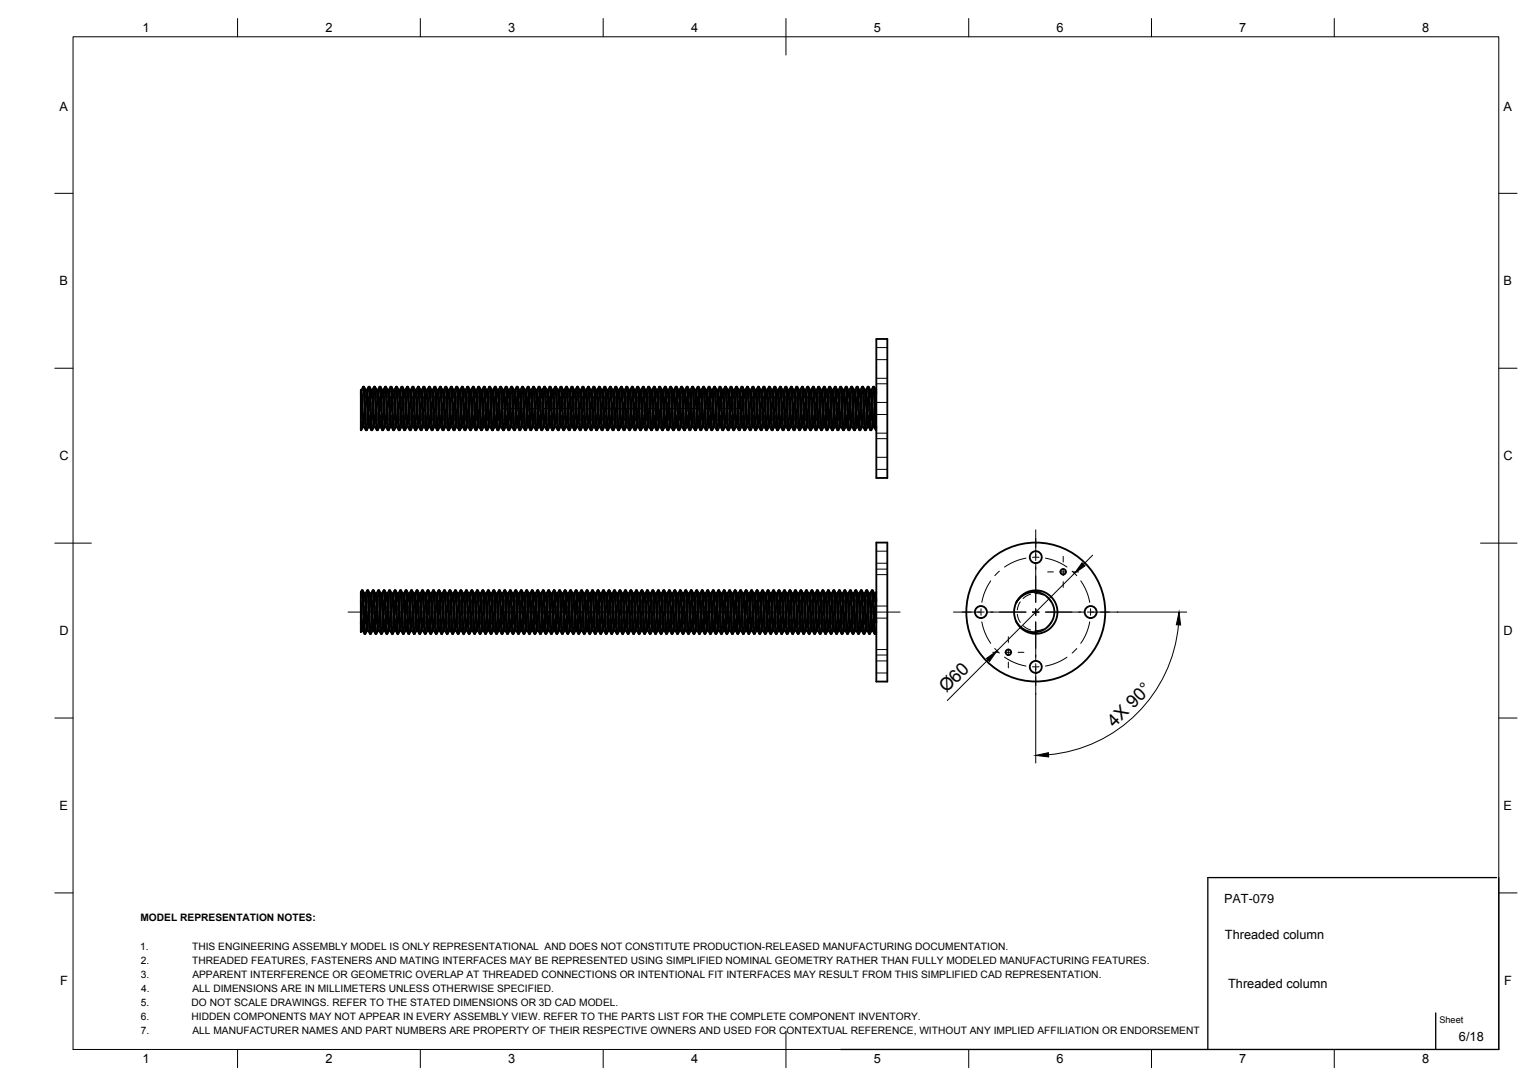
ISO-10303-21;
HEADER;
/* Generated by software containing ST-Developer
 * from STEP Tools, Inc. (www.steptools.com) 
 */

FILE_DESCRIPTION(
/* description */ ('Pipe clamp stand with threaded column'),
/* implementation_level */ '2;1');

FILE_NAME(
/* name */ 'Threaded column.step',
/* time_stamp */ '2026-10-27T10:55:48-07:00',
/* author */ (''),
/* organization */ (''),
/* preprocessor_version */ 'ST-DEVELOPER v20.2',
/* originating_system */ 'Autodesk Translation Framework v15.17.0.0',
/* authorisation */ '');

FILE_SCHEMA (('AUTOMOTIVE_DESIGN { 1 0 10303 214 3 1 1 }'));
ENDSEC;

DATA;
#10=MECHANICAL_DESIGN_GEOMETRIC_PRESENTATION_REPRESENTATION('',(#742),#34433);
#207=B_SPLINE_SURFACE_WITH_KNOTS('',3,3,((#22386,#22387,#22388,#22389,#22390,
#22391,#22392,#22393,#22394,#22395,#22396,#22397,#22398,#22399,#22400,#22401,
#22402,#22403,#22404,#22405,#22406,#22407,#22408,#22409,#22410,#22411,#22412,
#22413,#22414,#22415,#22416,#22417,#22418,#22419,#22420,#22421,#22422,#22423,
#22424,#22425,#22426,#22427,#22428,#22429,#22430,#22431,#22432,#22433,#22434,
#22435,#22436,#22437,#22438,#22439,#22440,#22441,#22442,#22443,#22444,#22445,
#22446,#22447,#22448,#22449,#22450,#22451,#22452,#22453,#22454,#22455,#22456,
#22457,#22458,#22459,#22460,#22461,#22462,#22463,#22464,#22465,#22466,#22467,
#22468,#22469,#22470,#22471,#22472,#22473,#22474,#22475,#22476,#22477,#22478,
#22479,#22480,#22481,#22482,#22483,#22484,#22485,#22486,#22487,#22488,#22489,
#22490,#22491,#22492,#22493,#22494,#22495,#22496,#22497,#22498,#22499,#22500,
#22501,#22502,#22503,#22504,#22505,#22506,#22507,#22508,#22509,#22510,#22511,
#22512,#22513,#22514,#22515,#22516,#22517,#22518,#22519,#22520,#22521,#22522,
#22523,#22524,#22525,#22526,#22527,#22528,#22529,#22530,#22531,#22532,#22533,
#22534,#22535,#22536,#22537,#22538,#22539,#22540,#22541,#22542,#22543,#22544,
#22545,#22546,#22547,#22548,#22549,#22550,#22551,#22552,#22553,#22554,#22555,
#22556,#22557,#22558,#22559,#22560,#22561,#22562,#22563,#22564,#22565,#22566,
#22567,#22568,#22569,#22570,#22571,#22572,#22573,#22574,#22575,#22576,#22577,
#22578,#22579,#22580,#22581,#22582,#22583,#22584,#22585,#22586,#22587,#22588,
#22589,#22590,#22591,#22592,#22593,#22594,#22595,#22596,#22597,#22598,#22599,
#22600,#22601,#22602,#22603,#22604,#22605,#22606,#22607,#22608,#22609,#22610,
#22611,#22612,#22613,#22614,#22615,#22616,#22617,#22618,#22619,#22620,#22621,
#22622,#22623,#22624,#22625,#22626,#22627,#22628,#22629,#22630,#22631,#22632,
#22633,#22634,#22635,#22636,#22637,#22638,#22639,#22640,#22641,#22642,#22643,
#22644,#22645,#22646,#22647,#22648,#22649,#22650,#22651,#22652,#22653,#22654,
#22655,#22656,#22657,#22658,#22659,#22660,#22661,#22662,#22663,#22664,#22665,
#22666,#22667,#22668,#22669,#22670,#22671,#22672,#22673,#22674,#22675,#22676,
#22677,#22678,#22679,#22680,#22681,#22682,#22683,#22684,#22685,#22686,#22687,
#22688,#22689,#22690,#22691,#22692,#22693,#22694,#22695,#22696,#22697,#22698,
#22699,#22700,#22701,#22702,#22703,#22704,#22705,#22706,#22707,#22708,#22709,
#22710,#22711,#22712,#22713,#22714,#22715,#22716,#22717,#22718,#22719,#22720,
#22721,#22722,#22723,#22724,#22725,#22726,#22727,#22728,#22729,#22730,#22731,
#22732,#22733,#22734,#22735,#22736,#22737,#22738,#22739,#22740,#22741,#22742,
#22743,#22744,#22745,#22746,#22747,#22748,#22749,#22750,#22751,#22752,#22753,
#22754,#22755,#22756,#22757,#22758,#22759,#22760,#22761,#22762,#22763,#22764,
#22765,#22766,#22767,#22768,#22769,#22770,#22771,#22772,#22773,#22774,#22775,
#22776,#22777,#22778,#22779,#22780,#22781,#22782,#22783,#22784,#22785,#22786,
#22787,#22788,#22789,#22790,#22791,#22792,#22793,#22794,#22795,#22796,#22797,
#22798,#22799,#22800,#22801,#22802,#22803,#22804,#22805,#22806,#22807,#22808,
#22809,#22810,#22811,#22812,#22813,#22814,#22815,#22816,#22817,#22818,#22819,
#22820,#22821,#22822,#22823,#22824,#22825,#22826,#22827,#22828,#22829,#22830,
#22831,#22832,#22833,#22834,#22835,#22836,#22837,#22838,#22839,#22840,#22841,
#22842,#22843,#22844,#22845,#22846,#22847,#22848,#22849,#22850,#22851,#22852,
#22853,#22854,#22855,#22856,#22857,#22858,#22859,#22860,#22861,#22862,#22863,
#22864,#22865,#22866,#22867,#22868,#22869,#22870,#22871,#22872,#22873,#22874,
#22875,#22876,#22877,#22878,#22879,#22880,#22881,#22882,#22883,#22884,#22885,
#22886,#22887,#22888,#22889,#22890,#22891,#22892,#22893,#22894,#22895,#22896,
#22897,#22898,#22899,#22900,#22901,#22902,#22903,#22904,#22905,#22906,#22907,
#22908,#22909,#22910,#22911,#22912,#22913,#22914,#22915,#22916,#22917,#22918,
#22919,#22920,#22921,#22922,#22923,#22924,#22925,#22926,#22927,#22928,#22929,
#22930,#22931,#22932,#22933,#22934,#22935,#22936,#22937,#22938,#22939,#22940,
#22941,#22942,#22943,#22944,#22945,#22946,#22947,#22948,#22949,#22950,#22951,
#22952,#22953,#22954,#22955,#22956,#22957,#22958,#22959,#22960,#22961,#22962,
#22963,#22964,#22965,#22966,#22967,#22968,#22969,#22970,#22971,#22972,#22973,
#22974,#22975,#22976,#22977,#22978,#22979,#22980,#22981,#22982,#22983,#22984,
#22985,#22986,#22987,#22988,#22989,#22990,#22991,#22992,#22993,#22994,#22995,
#22996,#22997,#22998,#22999,#23000,#23001,#23002,#23003,#23004,#23005,#23006,
#23007,#23008,#23009,#23010,#23011,#23012,#23013,#23014,#23015,#23016,#23017,
#23018,#23019,#23020,#23021,#23022,#23023,#23024,#23025,#23026,#23027,#23028,
#23029,#23030,#23031,#23032,#23033,#23034,#23035,#23036,#23037,#23038,#23039,
#23040,#23041,#23042,#23043,#23044,#23045,#23046,#23047,#23048,#23049,#23050,
#23051,#23052,#23053,#23054,#23055,#23056,#23057,#23058,#23059,#23060,#23061,
#23062,#23063,#23064,#23065,#23066,#23067),(#23068,#23069,#23070,#23071,
#23072,#23073,#23074,#23075,#23076,#23077,#23078,#23079,#23080,#23081,#23082,
#23083,#23084,#23085,#23086,#23087,#23088,#23089,#23090,#23091,#23092,#23093,
#23094,#23095,#23096,#23097,#23098,#23099,#23100,#23101,#23102,#23103,#23104,
#23105,#23106,#23107,#23108,#23109,#23110,#23111,#23112,#23113,#23114,#23115,
#23116,#23117,#23118,#23119,#23120,#23121,#23122,#23123,#23124,#23125,#23126,
#23127,#23128,#23129,#23130,#23131,#23132,#23133,#23134,#23135,#23136,#23137,
#23138,#23139,#23140,#23141,#23142,#23143,#23144,#23145,#23146,#23147,#23148,
#23149,#23150,#23151,#23152,#23153,#23154,#23155,#23156,#23157,#23158,#23159,
#23160,#23161,#23162,#23163,#23164,#23165,#23166,#23167,#23168,#23169,#23170,
#23171,#23172,#23173,#23174,#23175,#23176,#23177,#23178,#23179,#23180,#23181,
#23182,#23183,#23184,#23185,#23186,#23187,#23188,#23189,#23190,#23191,#23192,
#23193,#23194,#23195,#23196,#23197,#23198,#23199,#23200,#23201,#23202,#23203,
#23204,#23205,#23206,#23207,#23208,#23209,#23210,#23211,#23212,#23213,#23214,
#23215,#23216,#23217,#23218,#23219,#23220,#23221,#23222,#23223,#23224,#23225,
#23226,#23227,#23228,#23229,#23230,#23231,#23232,#23233,#23234,#23235,#23236,
#23237,#23238,#23239,#23240,#23241,#23242,#23243,#23244,#23245,#23246,#23247,
#23248,#23249,#23250,#23251,#23252,#23253,#23254,#23255,#23256,#23257,#23258,
#23259,#23260,#23261,#23262,#23263,#23264,#23265,#23266,#23267,#23268,#23269,
#23270,#23271,#23272,#23273,#23274,#23275,#23276,#23277,#23278,#23279,#23280,
#23281,#23282,#23283,#23284,#23285,#23286,#23287,#23288,#23289,#23290,#23291,
#23292,#23293,#23294,#23295,#23296,#23297,#23298,#23299,#23300,#23301,#23302,
#23303,#23304,#23305,#23306,#23307,#23308,#23309,#23310,#23311,#23312,#23313,
#23314,#23315,#23316,#23317,#23318,#23319,#23320,#23321,#23322,#23323,#23324,
#23325,#23326,#23327,#23328,#23329,#23330,#23331,#23332,#23333,#23334,#23335,
#23336,#23337,#23338,#23339,#23340,#23341,#23342,#23343,#23344,#23345,#23346,
#23347,#23348,#23349,#23350,#23351,#23352,#23353,#23354,#23355,#23356,#23357,
#23358,#23359,#23360,#23361,#23362,#23363,#23364,#23365,#23366,#23367,#23368,
#23369,#23370,#23371,#23372,#23373,#23374,#23375,#23376,#23377,#23378,#23379,
#23380,#23381,#23382,#23383,#23384,#23385,#23386,#23387,#23388,#23389,#23390,
#23391,#23392,#23393,#23394,#23395,#23396,#23397,#23398,#23399,#23400,#23401,
#23402,#23403,#23404,#23405,#23406,#23407,#23408,#23409,#23410,#23411,#23412,
#23413,#23414,#23415,#23416,#23417,#23418,#23419,#23420,#23421,#23422,#23423,
#23424,#23425,#23426,#23427,#23428,#23429,#23430,#23431,#23432,#23433,#23434,
#23435,#23436,#23437,#23438,#23439,#23440,#23441,#23442,#23443,#23444,#23445,
#23446,#23447,#23448,#23449,#23450,#23451,#23452,#23453,#23454,#23455,#23456,
#23457,#23458,#23459,#23460,#23461,#23462,#23463,#23464,#23465,#23466,#23467,
#23468,#23469,#23470,#23471,#23472,#23473,#23474,#23475,#23476,#23477,#23478,
#23479,#23480,#23481,#23482,#23483,#23484,#23485,#23486,#23487,#23488,#23489,
#23490,#23491,#23492,#23493,#23494,#23495,#23496,#23497,#23498,#23499,#23500,
#23501,#23502,#23503,#23504,#23505,#23506,#23507,#23508,#23509,#23510,#23511,
#23512,#23513,#23514,#23515,#23516,#23517,#23518,#23519,#23520,#23521,#23522,
#23523,#23524,#23525,#23526,#23527,#23528,#23529,#23530,#23531,#23532,#23533,
#23534,#23535,#23536,#23537,#23538,#23539,#23540,#23541,#23542,#23543,#23544,
#23545,#23546,#23547,#23548,#23549,#23550,#23551,#23552,#23553,#23554,#23555,
#23556,#23557,#23558,#23559,#23560,#23561,#23562,#23563,#23564,#23565,#23566,
#23567,#23568,#23569,#23570,#23571,#23572,#23573,#23574,#23575,#23576,#23577,
#23578,#23579,#23580,#23581,#23582,#23583,#23584,#23585,#23586,#23587,#23588,
#23589,#23590,#23591,#23592,#23593,#23594,#23595,#23596,#23597,#23598,#23599,
#23600,#23601,#23602,#23603,#23604,#23605,#23606,#23607,#23608,#23609,#23610,
#23611,#23612,#23613,#23614,#23615,#23616,#23617,#23618,#23619,#23620,#23621,
#23622,#23623,#23624,#23625,#23626,#23627,#23628,#23629,#23630,#23631,#23632,
#23633,#23634,#23635,#23636,#23637,#23638,#23639,#23640,#23641,#23642,#23643,
#23644,#23645,#23646,#23647,#23648,#23649,#23650,#23651,#23652,#23653,#23654,
#23655,#23656,#23657,#23658,#23659,#23660,#23661,#23662,#23663,#23664,#23665,
#23666,#23667,#23668,#23669,#23670,#23671,#23672,#23673,#23674,#23675,#23676,
#23677,#23678,#23679,#23680,#23681,#23682,#23683,#23684,#23685,#23686,#23687,
#23688,#23689,#23690,#23691,#23692,#23693,#23694,#23695,#23696,#23697,#23698,
#23699,#23700,#23701,#23702,#23703,#23704,#23705,#23706,#23707,#23708,#23709,
#23710,#23711,#23712,#23713,#23714,#23715,#23716,#23717,#23718,#23719,#23720,
#23721,#23722,#23723,#23724,#23725,#23726,#23727,#23728,#23729,#23730,#23731,
#23732,#23733,#23734,#23735,#23736,#23737,#23738,#23739,#23740,#23741,#23742,
#23743,#23744,#23745,#23746,#23747,#23748,#23749),(#23750,#23751,#23752,
#23753,#23754,#23755,#23756,#23757,#23758,#23759,#23760,#23761,#23762,#23763,
#23764,#23765,#23766,#23767,#23768,#23769,#23770,#23771,#23772,#23773,#23774,
#23775,#23776,#23777,#23778,#23779,#23780,#23781,#23782,#23783,#23784,#23785,
#23786,#23787,#23788,#23789,#23790,#23791,#23792,#23793,#23794,#23795,#23796,
#23797,#23798,#23799,#23800,#23801,#23802,#23803,#23804,#23805,#23806,#23807,
#23808,#23809,#23810,#23811,#23812,#23813,#23814,#23815,#23816,#23817,#23818,
#23819,#23820,#23821,#23822,#23823,#23824,#23825,#23826,#23827,#23828,#23829,
#23830,#23831,#23832,#23833,#23834,#23835,#23836,#23837,#23838,#23839,#23840,
#23841,#23842,#23843,#23844,#23845,#23846,#23847,#23848,#23849,#23850,#23851,
#23852,#23853,#23854,#23855,#23856,#23857,#23858,#23859,#23860,#23861,#23862,
#23863,#23864,#23865,#23866,#23867,#23868,#23869,#23870,#23871,#23872,#23873,
#23874,#23875,#23876,#23877,#23878,#23879,#23880,#23881,#23882,#23883,#23884,
#23885,#23886,#23887,#23888,#23889,#23890,#23891,#23892,#23893,#23894,#23895,
#23896,#23897,#23898,#23899,#23900,#23901,#23902,#23903,#23904,#23905,#23906,
#23907,#23908,#23909,#23910,#23911,#23912,#23913,#23914,#23915,#23916,#23917,
#23918,#23919,#23920,#23921,#23922,#23923,#23924,#23925,#23926,#23927,#23928,
#23929,#23930,#23931,#23932,#23933,#23934,#23935,#23936,#23937,#23938,#23939,
#23940,#23941,#23942,#23943,#23944,#23945,#23946,#23947,#23948,#23949,#23950,
#23951,#23952,#23953,#23954,#23955,#23956,#23957,#23958,#23959,#23960,#23961,
#23962,#23963,#23964,#23965,#23966,#23967,#23968,#23969,#23970,#23971,#23972,
#23973,#23974,#23975,#23976,#23977,#23978,#23979,#23980,#23981,#23982,#23983,
#23984,#23985,#23986,#23987,#23988,#23989,#23990,#23991,#23992,#23993,#23994,
#23995,#23996,#23997,#23998,#23999,#24000,#24001,#24002,#24003,#24004,#24005,
#24006,#24007,#24008,#24009,#24010,#24011,#24012,#24013,#24014,#24015,#24016,
#24017,#24018,#24019,#24020,#24021,#24022,#24023,#24024,#24025,#24026,#24027,
#24028,#24029,#24030,#24031,#24032,#24033,#24034,#24035,#24036,#24037,#24038,
#24039,#24040,#24041,#24042,#24043,#24044,#24045,#24046,#24047,#24048,#24049,
#24050,#24051,#24052,#24053,#24054,#24055,#24056,#24057,#24058,#24059,#24060,
#24061,#24062,#24063,#24064,#24065,#24066,#24067,#24068,#24069,#24070,#24071,
#24072,#24073,#24074,#24075,#24076,#24077,#24078,#24079,#24080,#24081,#24082,
#24083,#24084,#24085,#24086,#24087,#24088,#24089,#24090,#24091,#24092,#24093,
#24094,#24095,#24096,#24097,#24098,#24099,#24100,#24101,#24102,#24103,#24104,
#24105,#24106,#24107,#24108,#24109,#24110,#24111,#24112,#24113,#24114,#24115,
#24116,#24117,#24118,#24119,#24120,#24121,#24122,#24123,#24124,#24125,#24126,
#24127,#24128,#24129,#24130,#24131,#24132,#24133,#24134,#24135,#24136,#24137,
#24138,#24139,#24140,#24141,#24142,#24143,#24144,#24145,#24146,#24147,#24148,
#24149,#24150,#24151,#24152,#24153,#24154,#24155,#24156,#24157,#24158,#24159,
#24160,#24161,#24162,#24163,#24164,#24165,#24166,#24167,#24168,#24169,#24170,
#24171,#24172,#24173,#24174,#24175,#24176,#24177,#24178,#24179,#24180,#24181,
#24182,#24183,#24184,#24185,#24186,#24187,#24188,#24189,#24190,#24191,#24192,
#24193,#24194,#24195,#24196,#24197,#24198,#24199,#24200,#24201,#24202,#24203,
#24204,#24205,#24206,#24207,#24208,#24209,#24210,#24211,#24212,#24213,#24214,
#24215,#24216,#24217,#24218,#24219,#24220,#24221,#24222,#24223,#24224,#24225,
#24226,#24227,#24228,#24229,#24230,#24231,#24232,#24233,#24234,#24235,#24236,
#24237,#24238,#24239,#24240,#24241,#24242,#24243,#24244,#24245,#24246,#24247,
#24248,#24249,#24250,#24251,#24252,#24253,#24254,#24255,#24256,#24257,#24258,
#24259,#24260,#24261,#24262,#24263,#24264,#24265,#24266,#24267,#24268,#24269,
#24270,#24271,#24272,#24273,#24274,#24275,#24276,#24277,#24278,#24279,#24280,
#24281,#24282,#24283,#24284,#24285,#24286,#24287,#24288,#24289,#24290,#24291,
#24292,#24293,#24294,#24295,#24296,#24297,#24298,#24299,#24300,#24301,#24302,
#24303,#24304,#24305,#24306,#24307,#24308,#24309,#24310,#24311,#24312,#24313,
#24314,#24315,#24316,#24317,#24318,#24319,#24320,#24321,#24322,#24323,#24324,
#24325,#24326,#24327,#24328,#24329,#24330,#24331,#24332,#24333,#24334,#24335,
#24336,#24337,#24338,#24339,#24340,#24341,#24342,#24343,#24344,#24345,#24346,
#24347,#24348,#24349,#24350,#24351,#24352,#24353,#24354,#24355,#24356,#24357,
#24358,#24359,#24360,#24361,#24362,#24363,#24364,#24365,#24366,#24367,#24368,
#24369,#24370,#24371,#24372,#24373,#24374,#24375,#24376,#24377,#24378,#24379,
#24380,#24381,#24382,#24383,#24384,#24385,#24386,#24387,#24388,#24389,#24390,
#24391,#24392,#24393,#24394,#24395,#24396,#24397,#24398,#24399,#24400,#24401,
#24402,#24403,#24404,#24405,#24406,#24407,#24408,#24409,#24410,#24411,#24412,
#24413,#24414,#24415,#24416,#24417,#24418,#24419,#24420,#24421,#24422,#24423,
#24424,#24425,#24426,#24427,#24428,#24429,#24430,#24431),(#24432,#24433,
#24434,#24435,#24436,#24437,#24438,#24439,#24440,#24441,#24442,#24443,#24444,
#24445,#24446,#24447,#24448,#24449,#24450,#24451,#24452,#24453,#24454,#24455,
#24456,#24457,#24458,#24459,#24460,#24461,#24462,#24463,#24464,#24465,#24466,
#24467,#24468,#24469,#24470,#24471,#24472,#24473,#24474,#24475,#24476,#24477,
#24478,#24479,#24480,#24481,#24482,#24483,#24484,#24485,#24486,#24487,#24488,
#24489,#24490,#24491,#24492,#24493,#24494,#24495,#24496,#24497,#24498,#24499,
#24500,#24501,#24502,#24503,#24504,#24505,#24506,#24507,#24508,#24509,#24510,
#24511,#24512,#24513,#24514,#24515,#24516,#24517,#24518,#24519,#24520,#24521,
#24522,#24523,#24524,#24525,#24526,#24527,#24528,#24529,#24530,#24531,#24532,
#24533,#24534,#24535,#24536,#24537,#24538,#24539,#24540,#24541,#24542,#24543,
#24544,#24545,#24546,#24547,#24548,#24549,#24550,#24551,#24552,#24553,#24554,
#24555,#24556,#24557,#24558,#24559,#24560,#24561,#24562,#24563,#24564,#24565,
#24566,#24567,#24568,#24569,#24570,#24571,#24572,#24573,#24574,#24575,#24576,
#24577,#24578,#24579,#24580,#24581,#24582,#24583,#24584,#24585,#24586,#24587,
#24588,#24589,#24590,#24591,#24592,#24593,#24594,#24595,#24596,#24597,#24598,
#24599,#24600,#24601,#24602,#24603,#24604,#24605,#24606,#24607,#24608,#24609,
#24610,#24611,#24612,#24613,#24614,#24615,#24616,#24617,#24618,#24619,#24620,
#24621,#24622,#24623,#24624,#24625,#24626,#24627,#24628,#24629,#24630,#24631,
#24632,#24633,#24634,#24635,#24636,#24637,#24638,#24639,#24640,#24641,#24642,
#24643,#24644,#24645,#24646,#24647,#24648,#24649,#24650,#24651,#24652,#24653,
#24654,#24655,#24656,#24657,#24658,#24659,#24660,#24661,#24662,#24663,#24664,
#24665,#24666,#24667,#24668,#24669,#24670,#24671,#24672,#24673,#24674,#24675,
#24676,#24677,#24678,#24679,#24680,#24681,#24682,#24683,#24684,#24685,#24686,
#24687,#24688,#24689,#24690,#24691,#24692,#24693,#24694,#24695,#24696,#24697,
#24698,#24699,#24700,#24701,#24702,#24703,#24704,#24705,#24706,#24707,#24708,
#24709,#24710,#24711,#24712,#24713,#24714,#24715,#24716,#24717,#24718,#24719,
#24720,#24721,#24722,#24723,#24724,#24725,#24726,#24727,#24728,#24729,#24730,
#24731,#24732,#24733,#24734,#24735,#24736,#24737,#24738,#24739,#24740,#24741,
#24742,#24743,#24744,#24745,#24746,#24747,#24748,#24749,#24750,#24751,#24752,
#24753,#24754,#24755,#24756,#24757,#24758,#24759,#24760,#24761,#24762,#24763,
#24764,#24765,#24766,#24767,#24768,#24769,#24770,#24771,#24772,#24773,#24774,
#24775,#24776,#24777,#24778,#24779,#24780,#24781,#24782,#24783,#24784,#24785,
#24786,#24787,#24788,#24789,#24790,#24791,#24792,#24793,#24794,#24795,#24796,
#24797,#24798,#24799,#24800,#24801,#24802,#24803,#24804,#24805,#24806,#24807,
#24808,#24809,#24810,#24811,#24812,#24813,#24814,#24815,#24816,#24817,#24818,
#24819,#24820,#24821,#24822,#24823,#24824,#24825,#24826,#24827,#24828,#24829,
#24830,#24831,#24832,#24833,#24834,#24835,#24836,#24837,#24838,#24839,#24840,
#24841,#24842,#24843,#24844,#24845,#24846,#24847,#24848,#24849,#24850,#24851,
#24852,#24853,#24854,#24855,#24856,#24857,#24858,#24859,#24860,#24861,#24862,
#24863,#24864,#24865,#24866,#24867,#24868,#24869,#24870,#24871,#24872,#24873,
#24874,#24875,#24876,#24877,#24878,#24879,#24880,#24881,#24882,#24883,#24884,
#24885,#24886,#24887,#24888,#24889,#24890,#24891,#24892,#24893,#24894,#24895,
#24896,#24897,#24898,#24899,#24900,#24901,#24902,#24903,#24904,#24905,#24906,
#24907,#24908,#24909,#24910,#24911,#24912,#24913,#24914,#24915,#24916,#24917,
#24918,#24919,#24920,#24921,#24922,#24923,#24924,#24925,#24926,#24927,#24928,
#24929,#24930,#24931,#24932,#24933,#24934,#24935,#24936,#24937,#24938,#24939,
#24940,#24941,#24942,#24943,#24944,#24945,#24946,#24947,#24948,#24949,#24950,
#24951,#24952,#24953,#24954,#24955,#24956,#24957,#24958,#24959,#24960,#24961,
#24962,#24963,#24964,#24965,#24966,#24967,#24968,#24969,#24970,#24971,#24972,
#24973,#24974,#24975,#24976,#24977,#24978,#24979,#24980,#24981,#24982,#24983,
#24984,#24985,#24986,#24987,#24988,#24989,#24990,#24991,#24992,#24993,#24994,
#24995,#24996,#24997,#24998,#24999,#25000,#25001,#25002,#25003,#25004,#25005,
#25006,#25007,#25008,#25009,#25010,#25011,#25012,#25013,#25014,#25015,#25016,
#25017,#25018,#25019,#25020,#25021,#25022,#25023,#25024,#25025,#25026,#25027,
#25028,#25029,#25030,#25031,#25032,#25033,#25034,#25035,#25036,#25037,#25038,
#25039,#25040,#25041,#25042,#25043,#25044,#25045,#25046,#25047,#25048,#25049,
#25050,#25051,#25052,#25053,#25054,#25055,#25056,#25057,#25058,#25059,#25060,
#25061,#25062,#25063,#25064,#25065,#25066,#25067,#25068,#25069,#25070,#25071,
#25072,#25073,#25074,#25075,#25076,#25077,#25078,#25079,#25080,#25081,#25082,
#25083,#25084,#25085,#25086,#25087,#25088,#25089,#25090,#25091,#25092,#25093,
#25094,#25095,#25096,#25097,#25098,#25099,#25100,#25101,#25102,#25103,#25104,
#25105,#25106,#25107,#25108,#25109,#25110,#25111,#25112,#25113)),
 .UNSPECIFIED.,.F.,.F.,.F.,(4,4),(4,1,1,1,1,1,1,1,1,1,1,1,1,1,1,1,1,1,1,
1,1,1,1,1,1,1,1,1,1,1,1,1,1,1,1,1,1,1,1,1,1,1,1,1,1,1,1,1,1,1,1,1,1,1,1,
1,1,1,1,1,1,1,1,1,1,1,1,1,1,1,1,1,1,1,1,1,1,1,1,1,1,1,1,1,1,1,1,1,1,1,1,
1,1,1,1,1,1,1,1,1,1,1,1,1,1,1,1,1,1,1,1,1,1,1,1,1,1,1,1,1,1,1,1,1,1,1,1,
1,1,1,1,1,1,1,1,1,1,1,1,1,1,1,1,1,1,1,1,1,1,1,1,1,1,1,1,1,1,1,1,1,1,1,1,
1,1,1,1,1,1,1,1,1,1,1,1,1,1,1,1,1,1,1,1,1,1,1,1,1,1,1,1,1,1,1,1,1,1,1,1,
1,1,1,1,1,1,1,1,1,1,1,1,1,1,1,1,1,1,1,1,1,1,1,1,1,1,1,1,1,1,1,1,1,1,1,1,
1,1,1,1,1,1,1,1,1,1,1,1,1,1,1,1,1,1,1,1,1,1,1,1,1,1,1,1,1,1,1,1,1,1,1,1,
1,1,1,1,1,1,1,1,1,1,1,1,1,1,1,1,1,1,1,1,1,1,1,1,1,1,1,1,1,1,1,1,1,1,1,1,
1,1,1,1,1,1,1,1,1,1,1,1,1,1,1,1,1,1,1,1,1,1,1,1,1,1,1,1,1,1,1,1,1,1,1,1,
1,1,1,1,1,1,1,1,1,1,1,1,1,1,1,1,1,1,1,1,1,1,1,1,1,1,1,1,1,1,1,1,1,1,1,1,
1,1,1,1,1,1,1,1,1,1,1,1,1,1,1,1,1,1,1,1,1,1,1,1,1,1,1,1,1,1,1,1,1,1,1,1,
1,1,1,1,1,1,1,1,1,1,1,1,1,1,1,1,1,1,1,1,1,1,1,1,1,1,1,1,1,1,1,1,1,1,1,1,
1,1,1,1,1,1,1,1,1,1,1,1,1,1,1,1,1,1,1,1,1,1,1,1,1,1,1,1,1,1,1,1,1,1,1,1,
1,1,1,1,1,1,1,1,1,1,1,1,1,1,1,1,1,1,1,1,1,1,1,1,1,1,1,1,1,1,1,1,1,1,1,1,
1,1,1,1,1,1,1,1,1,1,1,1,1,1,1,1,1,1,1,1,1,1,1,1,1,1,1,1,1,1,1,1,1,1,1,1,
1,1,1,1,1,1,1,1,1,1,1,1,1,1,1,1,1,1,1,1,1,1,1,1,1,1,1,1,1,1,1,1,1,1,1,1,
1,1,1,1,1,1,1,1,1,1,1,1,1,1,1,1,1,1,1,1,1,1,1,1,1,1,1,1,1,1,1,1,1,1,1,1,
1,1,1,1,1,1,1,1,1,1,1,1,1,1,1,1,1,1,1,1,1,1,1,1,1,1,1,1,1,1,1,1,1,1,1,1,
1,1,1,1,1,1,1,1,1,1,1,1,4),(0.,0.198319817466637),(8.29931545526329,8.79905931626407,
9.29880317726486,10.2982908992664,11.297778621268,12.2972663432696,12.7970102042703,
13.2967540652711,14.2962417872727,15.2957295092743,16.2952172312758,17.2947049532774,
18.294192675279,18.7939365362798,19.2936803972805,20.2931681192821,21.2926558412837,
22.2921435632852,23.2916312852868,24.2911190072884,25.2906067292899,25.7903505902907,
26.2900944512915,27.2895821732931,28.2890698952946,29.2885576172962,30.2880453392978,
31.2875330612993,32.2870207833009,32.7867646443017,33.2865085053025,34.2859962273041,
35.2854839493056,36.2849716713072,37.2844593933088,38.2839471153103,39.2834348373119,
39.7831786983127,40.2829225593135,41.282410281315,42.2818980033166,43.2813857253182,
44.2808734473197,45.2803611693213,46.2798488913229,46.7795927523237,47.2793366133244,
48.278824335326,49.2783120573276,50.2777997793291,51.2772875013307,52.2767752233323,
53.2762629453338,53.7760068063346,54.2757506673354,55.275238389337,56.2747261113385,
57.2742138333401,58.2737015553417,59.2731892773432,60.2726769993448,60.7724208603456,
61.2721647213464,62.2716524433479,63.2711401653495,64.2706278873511,65.2701156093526,
66.2696033313542,67.2690910533558,67.7688349143566,68.2685787753574,69.2680664973589,
70.2675542193605,71.2670419413621,72.2665296633636,73.2660173853652,74.2655051073667,
74.7652489683675,75.2649928293683,76.2644805513699,77.2639682733715,78.263455995373,
79.2629437173746,80.2624314393762,81.2619191613777,81.7616630223785,82.2614068833793,
83.2608946053809,84.2603823273824,85.259870049384,86.2593577713856,87.2588454933872,
88.2583332153887,88.7580770763895,89.2578209373903,90.2573086593918,91.2567963813934,
92.256284103395,93.2557718253966,94.2552595473981,95.2547472693997,95.7544911304005,
96.2542349914013,97.2537227134028,98.2532104354044,99.2526981574059,100.252185879408,
101.251673601409,102.251161323411,102.750905184411,103.250649045412,104.250136767414,
105.249624489415,106.249112211417,107.248599933418,108.24808765542,109.247575377422,
109.747319238422,110.247063099423,111.246550821425,112.246038543426,113.245526265428,
114.245013987429,115.244501709431,116.243989431433,116.743733292433,117.243477153434,
118.242964875436,119.242452597437,120.241940319439,121.24142804144,122.240915763442,
123.240403485444,123.740147346444,124.239891207445,125.239378929447,126.238866651448,
127.23835437345,128.237842095451,129.237329817453,130.236817539455,130.736561400455,
131.236305261456,132.235792983458,133.235280705459,134.234768427461,135.234256149462,
136.233743871464,137.233231593466,137.732975454466,138.232719315467,139.232207037469,
140.23169475947,141.231182481472,142.230670203473,143.230157925475,144.229645647477,
144.729389508477,145.229133369478,146.22862109148,147.228108813481,148.227596535483,
149.227084257484,150.226571979486,151.226059701487,151.725803562488,152.225547423489,
153.225035145491,154.224522867492,155.224010589494,156.223498311495,157.222986033497,
158.222473755498,158.722217616499,159.2219614775,160.221449199502,161.220936921503,
162.220424643505,163.219912365506,164.219400087508,165.218887809509,165.71863167051,
166.218375531511,167.217863253513,168.217350975514,169.216838697516,170.216326419517,
171.215814141519,172.21530186352,172.715045724521,173.214789585522,174.214277307524,
175.213765029525,176.213252751527,177.212740473528,178.21222819553,179.211715917531,
179.711459778532,180.211203639533,181.210691361535,182.210179083536,183.209666805538,
184.209154527539,185.208642249541,186.208129971542,186.707873832543,187.207617693544,
188.207105415545,189.206593137547,190.206080859549,191.20556858155,192.205056303552,
193.204544025553,193.704287886554,194.204031747555,195.203519469556,196.203007191558,
197.20249491356,198.201982635561,199.201470357563,200.200958079564,200.700701940565,
201.200445801566,202.199933523567,203.199421245569,204.198908967571,205.198396689572,
206.197884411574,207.197372133575,207.697115994576,208.196859855577,209.196347577578,
210.19583529958,211.195323021582,212.194810743583,213.194298465585,214.193786187586,
214.693530048587,215.193273909588,216.192761631589,217.192249353591,218.191737075593,
219.191224797594,220.190712519596,221.190200241597,221.689944102598,222.189687963599,
223.1891756856,224.188663407602,225.188151129604,226.187638851605,227.187126573607,
228.186614295608,228.686358156609,229.18610201761,230.185589739611,231.185077461613,
232.184565183614,233.184052905616,234.183540627618,235.183028349619,235.68277221062,
236.182516071621,237.182003793622,238.181491515624,239.180979237625,240.180466959627,
241.179954681629,242.17944240363,242.679186264631,243.178930125632,244.178417847633,
245.177905569635,246.177393291636,247.176881013638,248.17636873564,249.175856457641,
249.675600318642,250.175344179643,251.174831901644,252.174319623646,253.173807345647,
254.173295067649,255.172782789651,256.172270511652,256.672014372653,257.171758233654,
258.171245955655,259.170733677657,260.170221399658,261.16970912166,262.169196843661,
263.168684565663,263.668428426664,264.168172287665,265.167660009666,266.167147731668,
267.166635453669,268.166123175671,269.165610897672,270.165098619674,270.664842480675,
271.164586341676,272.164074063677,273.163561785679,274.16304950768,275.162537229682,
276.162024951683,277.161512673685,277.661256534686,278.161000395687,279.160488117688,
280.15997583969,281.159463561691,282.158951283693,283.158439005694,284.157926727696,
284.657670588697,285.157414449698,286.156902171699,287.156389893701,288.155877615702,
289.155365337704,290.154853059705,291.154340781707,291.654084642708,292.153828503709,
293.15331622571,294.152803947712,295.152291669713,296.151779391715,297.151267113716,
298.150754835718,298.650498696719,299.15024255772,300.149730279721,301.149218001723,
302.148705723724,303.148193445726,304.147681167727,305.147168889729,306.146656611731,
307.146144333732,308.145632055734,309.145119777735,310.144607499737,310.644351360738,
311.144095221738,312.14358294374,313.143070665741,314.142558387743,315.142046109745,
316.141533831746,317.141021553748,317.640765414749,318.140509275749,319.139996997751,
320.139484719752,321.138972441754,322.138460163756,323.137947885757,324.137435607759,
324.63717946876,325.13692332976,326.136411051762,327.135898773763,328.135386495765,
329.134874217767,330.134361939768,331.13384966177,331.63359352277,332.133337383771,
333.132825105773,334.132312827774,335.131800549776,336.131288271778,337.130775993779,
338.130263715781,338.630007576781,339.129751437782,340.129239159784,341.128726881785,
342.128214603787,343.127702325789,344.12719004779,345.126677769792,345.626421630792,
346.126165491793,347.125653213795,348.125140935796,349.124628657798,350.124116379799,
351.123604101801,352.123091823803,352.622835684803,353.122579545804,354.122067267806,
355.121554989807,356.121042711809,357.12053043381,358.120018155812,359.119505877814,
359.619249738814,360.118993599815,361.118481321817,362.117969043818,363.11745676582,
364.116944487821,365.116432209823,366.115919931825,366.615663792825,367.115407653826,
368.114895375828,369.114383097829,370.113870819831,371.113358541832,372.112846263834,
373.112333985836,373.612077846836,374.111821707837,375.111309429839,376.11079715184,
377.110284873842,378.109772595843,379.109260317845,380.108748039846,380.608491900847,
381.108235761848,382.10772348385,383.107211205851,384.106698927853,385.106186649854,
386.105674371856,387.105162093857,387.604905954858,388.104649815859,389.104137537861,
390.103625259862,391.103112981864,392.102600703865,393.102088425867,394.101576147868,
394.601320008869,395.10106386987,396.100551591872,397.100039313873,398.099527035875,
399.099014757876,400.098502479878,401.097990201879,401.59773406288,402.097477923881,
403.096965645883,404.096453367884,405.095941089886,406.095428811887,407.094916533889,
408.09440425589,408.594148116891,409.093891977892,410.093379699894,411.092867421895,
412.092355143897,413.091842865898,414.0913305879,415.090818309901,415.590562170902,
416.090306031903,417.089793753905,418.089281475906,419.088769197908,420.088256919909,
421.087744641911,422.087232363912,422.586976224913,423.086720085914,424.086207807916,
425.085695529917,426.085183251919,427.08467097392,428.084158695922,429.083646417923,
429.583390278924,430.083134139925,431.082621861926,432.082109583928,433.08159730593,
434.081085027931,435.080572749933,436.080060471934,436.579804332935,437.079548193936,
438.079035915937,439.078523637939,440.078011359941,441.077499081942,442.076986803944,
443.076474525945,443.576218386946,444.075962247947,445.075449969948,446.07493769195,
447.074425413952,448.073913135953,449.073400857955,450.072888579956,450.572632440957,
451.072376301958,452.071864023959,453.071351745961,454.070839467963,455.070327189964,
456.069814911966,457.069302633967,457.569046494968,458.068790355969,459.06827807797,
460.067765799972,461.067253521973,462.066741243975,463.066228965977,464.065716687978,
464.565460548979,465.06520440998,466.064692131981,467.064179853983,468.063667575984,
469.063155297986,470.062643019988,471.062130741989,471.56187460299,472.061618463991,
473.061106185992,474.060593907994,475.060081629995,476.059569351997,477.059057073999,
478.058544796,478.558288657001,479.058032518002,480.057520240003,481.057007962005,
482.056495684006,483.055983406008,484.05547112801,485.054958850011,485.554702711012,
486.054446572013,487.053934294014,488.053422016016,489.052909738017,490.052397460019,
491.051885182021,492.051372904022,492.551116765023,493.050860626024,494.050348348025,
495.049836070027,496.049323792028,497.04881151403,498.048299236031,499.047786958033,
499.547530819034,500.047274680035,501.046762402036,502.046250124038,503.045737846039,
504.045225568041,505.044713290042,506.044201012044,506.543944873045,507.043688734046,
508.043176456047,509.042664178049,510.04215190005,511.041639622052,512.041127344053,
513.040615066055,513.540358927056,514.040102788057,515.039590510058,516.03907823206,
517.038565954061,518.038053676063,519.037541398064,520.037029120066,520.536772981067,
521.036516842067,522.036004564069,523.035492286071,524.034980008072,525.034467730074,
526.033955452075,527.033443174077,527.533187035078,528.032930896078,529.03241861808,
530.031906340082,531.031394062083,532.030881784085,533.030369506086,534.029857228088,
534.529601089089,535.029344950089,536.028832672091,537.028320394093,538.027808116094,
539.027295838096,540.026783560097,541.026271282099,541.5260151431,542.0257590041,
543.025246726102,544.024734448104,545.024222170105,546.023709892107,547.023197614108,
548.02268533611,548.522429197111,549.022173058111,550.021660780113,551.021148502115,
552.020636224116,553.020123946118,554.019611668119,555.019099390121,555.518843251122,
556.018587112122,557.018074834124,558.017562556126,559.017050278127,560.016538000129,
561.01602572213,562.015513444132,562.515257305133,563.015001166133,564.014488888135,
565.013976610137,566.013464332138,567.01295205414,568.012439776141,569.011927498143,
569.511671359144,570.011415220144,571.010902942146,572.010390664148,573.009878386149,
574.009366108151,575.008853830152,576.008341552154,576.508085413155,577.007829274155,
578.007316996157,579.006804718158,580.00629244016,581.005780162162,582.005267884163,
583.004755606165,583.504499467165,584.004243328166,585.003731050168,586.003218772169,
587.002706494171,588.002194216173,589.001681938174,590.001169660176,590.500913521176,
591.000657382177,592.000145104179,592.99963282618,593.999120548182,594.998608270183,
595.998095992185,596.497839853186,596.997583714187,597.997071436188,598.99655915819,
599.996046880191,600.495790741192,600.995534602193),.UNSPECIFIED.);
#208=B_SPLINE_SURFACE_WITH_KNOTS('',3,3,((#25249,#25250,#25251,#25252,#25253,
#25254,#25255,#25256,#25257,#25258,#25259,#25260,#25261,#25262,#25263,#25264,
#25265,#25266,#25267,#25268,#25269,#25270,#25271,#25272,#25273,#25274,#25275,
#25276,#25277,#25278,#25279,#25280,#25281,#25282,#25283,#25284,#25285,#25286,
#25287,#25288,#25289,#25290,#25291,#25292,#25293,#25294,#25295,#25296,#25297,
#25298,#25299,#25300,#25301,#25302,#25303,#25304,#25305,#25306,#25307,#25308,
#25309,#25310,#25311,#25312,#25313,#25314,#25315,#25316,#25317,#25318,#25319,
#25320,#25321,#25322,#25323,#25324,#25325,#25326,#25327,#25328,#25329,#25330,
#25331,#25332,#25333,#25334,#25335,#25336,#25337,#25338,#25339,#25340,#25341,
#25342,#25343,#25344,#25345,#25346,#25347,#25348,#25349,#25350,#25351,#25352,
#25353,#25354,#25355,#25356,#25357,#25358,#25359,#25360,#25361,#25362,#25363,
#25364,#25365,#25366,#25367,#25368,#25369,#25370,#25371,#25372,#25373,#25374,
#25375,#25376,#25377,#25378,#25379,#25380,#25381,#25382,#25383,#25384,#25385,
#25386,#25387,#25388,#25389,#25390,#25391,#25392,#25393,#25394,#25395,#25396,
#25397,#25398,#25399,#25400,#25401,#25402,#25403,#25404,#25405,#25406,#25407,
#25408,#25409,#25410,#25411,#25412,#25413,#25414,#25415,#25416,#25417,#25418,
#25419,#25420,#25421,#25422,#25423,#25424,#25425,#25426,#25427,#25428,#25429,
#25430,#25431,#25432,#25433,#25434,#25435,#25436,#25437,#25438,#25439,#25440,
#25441,#25442,#25443,#25444,#25445,#25446,#25447,#25448,#25449,#25450,#25451,
#25452,#25453,#25454,#25455,#25456,#25457,#25458,#25459,#25460,#25461,#25462,
#25463,#25464,#25465,#25466,#25467,#25468,#25469,#25470,#25471,#25472,#25473,
#25474,#25475,#25476,#25477,#25478,#25479,#25480,#25481,#25482,#25483,#25484,
#25485,#25486,#25487,#25488,#25489,#25490,#25491,#25492,#25493,#25494,#25495,
#25496,#25497,#25498,#25499,#25500,#25501,#25502,#25503,#25504,#25505,#25506,
#25507,#25508,#25509,#25510,#25511,#25512,#25513,#25514,#25515,#25516,#25517,
#25518,#25519,#25520,#25521,#25522,#25523,#25524,#25525,#25526,#25527,#25528,
#25529,#25530,#25531,#25532,#25533,#25534,#25535,#25536,#25537,#25538,#25539,
#25540,#25541,#25542,#25543,#25544,#25545,#25546,#25547,#25548,#25549,#25550,
#25551,#25552,#25553,#25554,#25555,#25556,#25557,#25558,#25559,#25560,#25561,
#25562,#25563,#25564,#25565,#25566,#25567,#25568,#25569,#25570,#25571,#25572,
#25573,#25574,#25575,#25576,#25577,#25578,#25579,#25580,#25581,#25582,#25583,
#25584,#25585,#25586,#25587,#25588,#25589,#25590,#25591,#25592,#25593,#25594,
#25595,#25596,#25597,#25598,#25599,#25600,#25601,#25602,#25603,#25604,#25605,
#25606,#25607,#25608,#25609,#25610,#25611,#25612,#25613,#25614,#25615,#25616,
#25617,#25618,#25619,#25620,#25621,#25622,#25623,#25624,#25625,#25626,#25627,
#25628,#25629,#25630,#25631,#25632,#25633,#25634,#25635,#25636,#25637,#25638,
#25639,#25640,#25641,#25642,#25643,#25644,#25645,#25646,#25647,#25648,#25649,
#25650,#25651,#25652,#25653,#25654,#25655,#25656,#25657,#25658,#25659,#25660,
#25661,#25662,#25663,#25664,#25665,#25666,#25667,#25668,#25669,#25670,#25671,
#25672,#25673,#25674,#25675,#25676,#25677,#25678,#25679,#25680,#25681,#25682,
#25683,#25684,#25685,#25686,#25687,#25688,#25689,#25690,#25691,#25692,#25693,
#25694,#25695,#25696,#25697,#25698,#25699,#25700,#25701,#25702,#25703,#25704,
#25705,#25706,#25707,#25708,#25709,#25710,#25711,#25712,#25713,#25714,#25715,
#25716,#25717,#25718,#25719,#25720,#25721,#25722,#25723,#25724,#25725,#25726,
#25727,#25728,#25729,#25730,#25731,#25732,#25733,#25734,#25735,#25736,#25737,
#25738,#25739,#25740,#25741,#25742,#25743,#25744,#25745,#25746,#25747,#25748,
#25749,#25750,#25751,#25752,#25753,#25754,#25755,#25756,#25757,#25758,#25759,
#25760,#25761,#25762,#25763,#25764,#25765,#25766,#25767,#25768,#25769,#25770,
#25771,#25772,#25773,#25774,#25775,#25776,#25777,#25778,#25779,#25780,#25781,
#25782,#25783,#25784,#25785,#25786,#25787,#25788,#25789,#25790,#25791,#25792,
#25793,#25794,#25795,#25796,#25797,#25798,#25799,#25800,#25801,#25802,#25803,
#25804,#25805,#25806,#25807,#25808,#25809,#25810,#25811,#25812,#25813,#25814,
#25815,#25816,#25817,#25818,#25819,#25820,#25821,#25822,#25823,#25824,#25825,
#25826,#25827,#25828,#25829,#25830,#25831,#25832,#25833,#25834,#25835,#25836,
#25837,#25838,#25839,#25840,#25841,#25842,#25843,#25844,#25845,#25846,#25847,
#25848,#25849,#25850,#25851,#25852,#25853,#25854,#25855,#25856,#25857,#25858,
#25859,#25860,#25861,#25862,#25863,#25864,#25865,#25866,#25867,#25868,#25869,
#25870,#25871,#25872,#25873,#25874,#25875,#25876,#25877,#25878,#25879,#25880,
#25881,#25882,#25883,#25884,#25885,#25886,#25887,#25888,#25889,#25890,#25891,
#25892,#25893,#25894,#25895,#25896,#25897,#25898,#25899,#25900,#25901,#25902,
#25903,#25904,#25905,#25906,#25907,#25908,#25909,#25910,#25911,#25912,#25913,
#25914,#25915,#25916,#25917,#25918,#25919,#25920,#25921,#25922,#25923,#25924,
#25925,#25926,#25927,#25928,#25929,#25930),(#25931,#25932,#25933,#25934,
#25935,#25936,#25937,#25938,#25939,#25940,#25941,#25942,#25943,#25944,#25945,
#25946,#25947,#25948,#25949,#25950,#25951,#25952,#25953,#25954,#25955,#25956,
#25957,#25958,#25959,#25960,#25961,#25962,#25963,#25964,#25965,#25966,#25967,
#25968,#25969,#25970,#25971,#25972,#25973,#25974,#25975,#25976,#25977,#25978,
#25979,#25980,#25981,#25982,#25983,#25984,#25985,#25986,#25987,#25988,#25989,
#25990,#25991,#25992,#25993,#25994,#25995,#25996,#25997,#25998,#25999,#26000,
#26001,#26002,#26003,#26004,#26005,#26006,#26007,#26008,#26009,#26010,#26011,
#26012,#26013,#26014,#26015,#26016,#26017,#26018,#26019,#26020,#26021,#26022,
#26023,#26024,#26025,#26026,#26027,#26028,#26029,#26030,#26031,#26032,#26033,
#26034,#26035,#26036,#26037,#26038,#26039,#26040,#26041,#26042,#26043,#26044,
#26045,#26046,#26047,#26048,#26049,#26050,#26051,#26052,#26053,#26054,#26055,
#26056,#26057,#26058,#26059,#26060,#26061,#26062,#26063,#26064,#26065,#26066,
#26067,#26068,#26069,#26070,#26071,#26072,#26073,#26074,#26075,#26076,#26077,
#26078,#26079,#26080,#26081,#26082,#26083,#26084,#26085,#26086,#26087,#26088,
#26089,#26090,#26091,#26092,#26093,#26094,#26095,#26096,#26097,#26098,#26099,
#26100,#26101,#26102,#26103,#26104,#26105,#26106,#26107,#26108,#26109,#26110,
#26111,#26112,#26113,#26114,#26115,#26116,#26117,#26118,#26119,#26120,#26121,
#26122,#26123,#26124,#26125,#26126,#26127,#26128,#26129,#26130,#26131,#26132,
#26133,#26134,#26135,#26136,#26137,#26138,#26139,#26140,#26141,#26142,#26143,
#26144,#26145,#26146,#26147,#26148,#26149,#26150,#26151,#26152,#26153,#26154,
#26155,#26156,#26157,#26158,#26159,#26160,#26161,#26162,#26163,#26164,#26165,
#26166,#26167,#26168,#26169,#26170,#26171,#26172,#26173,#26174,#26175,#26176,
#26177,#26178,#26179,#26180,#26181,#26182,#26183,#26184,#26185,#26186,#26187,
#26188,#26189,#26190,#26191,#26192,#26193,#26194,#26195,#26196,#26197,#26198,
#26199,#26200,#26201,#26202,#26203,#26204,#26205,#26206,#26207,#26208,#26209,
#26210,#26211,#26212,#26213,#26214,#26215,#26216,#26217,#26218,#26219,#26220,
#26221,#26222,#26223,#26224,#26225,#26226,#26227,#26228,#26229,#26230,#26231,
#26232,#26233,#26234,#26235,#26236,#26237,#26238,#26239,#26240,#26241,#26242,
#26243,#26244,#26245,#26246,#26247,#26248,#26249,#26250,#26251,#26252,#26253,
#26254,#26255,#26256,#26257,#26258,#26259,#26260,#26261,#26262,#26263,#26264,
#26265,#26266,#26267,#26268,#26269,#26270,#26271,#26272,#26273,#26274,#26275,
#26276,#26277,#26278,#26279,#26280,#26281,#26282,#26283,#26284,#26285,#26286,
#26287,#26288,#26289,#26290,#26291,#26292,#26293,#26294,#26295,#26296,#26297,
#26298,#26299,#26300,#26301,#26302,#26303,#26304,#26305,#26306,#26307,#26308,
#26309,#26310,#26311,#26312,#26313,#26314,#26315,#26316,#26317,#26318,#26319,
#26320,#26321,#26322,#26323,#26324,#26325,#26326,#26327,#26328,#26329,#26330,
#26331,#26332,#26333,#26334,#26335,#26336,#26337,#26338,#26339,#26340,#26341,
#26342,#26343,#26344,#26345,#26346,#26347,#26348,#26349,#26350,#26351,#26352,
#26353,#26354,#26355,#26356,#26357,#26358,#26359,#26360,#26361,#26362,#26363,
#26364,#26365,#26366,#26367,#26368,#26369,#26370,#26371,#26372,#26373,#26374,
#26375,#26376,#26377,#26378,#26379,#26380,#26381,#26382,#26383,#26384,#26385,
#26386,#26387,#26388,#26389,#26390,#26391,#26392,#26393,#26394,#26395,#26396,
#26397,#26398,#26399,#26400,#26401,#26402,#26403,#26404,#26405,#26406,#26407,
#26408,#26409,#26410,#26411,#26412,#26413,#26414,#26415,#26416,#26417,#26418,
#26419,#26420,#26421,#26422,#26423,#26424,#26425,#26426,#26427,#26428,#26429,
#26430,#26431,#26432,#26433,#26434,#26435,#26436,#26437,#26438,#26439,#26440,
#26441,#26442,#26443,#26444,#26445,#26446,#26447,#26448,#26449,#26450,#26451,
#26452,#26453,#26454,#26455,#26456,#26457,#26458,#26459,#26460,#26461,#26462,
#26463,#26464,#26465,#26466,#26467,#26468,#26469,#26470,#26471,#26472,#26473,
#26474,#26475,#26476,#26477,#26478,#26479,#26480,#26481,#26482,#26483,#26484,
#26485,#26486,#26487,#26488,#26489,#26490,#26491,#26492,#26493,#26494,#26495,
#26496,#26497,#26498,#26499,#26500,#26501,#26502,#26503,#26504,#26505,#26506,
#26507,#26508,#26509,#26510,#26511,#26512,#26513,#26514,#26515,#26516,#26517,
#26518,#26519,#26520,#26521,#26522,#26523,#26524,#26525,#26526,#26527,#26528,
#26529,#26530,#26531,#26532,#26533,#26534,#26535,#26536,#26537,#26538,#26539,
#26540,#26541,#26542,#26543,#26544,#26545,#26546,#26547,#26548,#26549,#26550,
#26551,#26552,#26553,#26554,#26555,#26556,#26557,#26558,#26559,#26560,#26561,
#26562,#26563,#26564,#26565,#26566,#26567,#26568,#26569,#26570,#26571,#26572,
#26573,#26574,#26575,#26576,#26577,#26578,#26579,#26580,#26581,#26582,#26583,
#26584,#26585,#26586,#26587,#26588,#26589,#26590,#26591,#26592,#26593,#26594,
#26595,#26596,#26597,#26598,#26599,#26600,#26601,#26602,#26603,#26604,#26605,
#26606,#26607,#26608,#26609,#26610,#26611,#26612),(#26613,#26614,#26615,
#26616,#26617,#26618,#26619,#26620,#26621,#26622,#26623,#26624,#26625,#26626,
#26627,#26628,#26629,#26630,#26631,#26632,#26633,#26634,#26635,#26636,#26637,
#26638,#26639,#26640,#26641,#26642,#26643,#26644,#26645,#26646,#26647,#26648,
#26649,#26650,#26651,#26652,#26653,#26654,#26655,#26656,#26657,#26658,#26659,
#26660,#26661,#26662,#26663,#26664,#26665,#26666,#26667,#26668,#26669,#26670,
#26671,#26672,#26673,#26674,#26675,#26676,#26677,#26678,#26679,#26680,#26681,
#26682,#26683,#26684,#26685,#26686,#26687,#26688,#26689,#26690,#26691,#26692,
#26693,#26694,#26695,#26696,#26697,#26698,#26699,#26700,#26701,#26702,#26703,
#26704,#26705,#26706,#26707,#26708,#26709,#26710,#26711,#26712,#26713,#26714,
#26715,#26716,#26717,#26718,#26719,#26720,#26721,#26722,#26723,#26724,#26725,
#26726,#26727,#26728,#26729,#26730,#26731,#26732,#26733,#26734,#26735,#26736,
#26737,#26738,#26739,#26740,#26741,#26742,#26743,#26744,#26745,#26746,#26747,
#26748,#26749,#26750,#26751,#26752,#26753,#26754,#26755,#26756,#26757,#26758,
#26759,#26760,#26761,#26762,#26763,#26764,#26765,#26766,#26767,#26768,#26769,
#26770,#26771,#26772,#26773,#26774,#26775,#26776,#26777,#26778,#26779,#26780,
#26781,#26782,#26783,#26784,#26785,#26786,#26787,#26788,#26789,#26790,#26791,
#26792,#26793,#26794,#26795,#26796,#26797,#26798,#26799,#26800,#26801,#26802,
#26803,#26804,#26805,#26806,#26807,#26808,#26809,#26810,#26811,#26812,#26813,
#26814,#26815,#26816,#26817,#26818,#26819,#26820,#26821,#26822,#26823,#26824,
#26825,#26826,#26827,#26828,#26829,#26830,#26831,#26832,#26833,#26834,#26835,
#26836,#26837,#26838,#26839,#26840,#26841,#26842,#26843,#26844,#26845,#26846,
#26847,#26848,#26849,#26850,#26851,#26852,#26853,#26854,#26855,#26856,#26857,
#26858,#26859,#26860,#26861,#26862,#26863,#26864,#26865,#26866,#26867,#26868,
#26869,#26870,#26871,#26872,#26873,#26874,#26875,#26876,#26877,#26878,#26879,
#26880,#26881,#26882,#26883,#26884,#26885,#26886,#26887,#26888,#26889,#26890,
#26891,#26892,#26893,#26894,#26895,#26896,#26897,#26898,#26899,#26900,#26901,
#26902,#26903,#26904,#26905,#26906,#26907,#26908,#26909,#26910,#26911,#26912,
#26913,#26914,#26915,#26916,#26917,#26918,#26919,#26920,#26921,#26922,#26923,
#26924,#26925,#26926,#26927,#26928,#26929,#26930,#26931,#26932,#26933,#26934,
#26935,#26936,#26937,#26938,#26939,#26940,#26941,#26942,#26943,#26944,#26945,
#26946,#26947,#26948,#26949,#26950,#26951,#26952,#26953,#26954,#26955,#26956,
#26957,#26958,#26959,#26960,#26961,#26962,#26963,#26964,#26965,#26966,#26967,
#26968,#26969,#26970,#26971,#26972,#26973,#26974,#26975,#26976,#26977,#26978,
#26979,#26980,#26981,#26982,#26983,#26984,#26985,#26986,#26987,#26988,#26989,
#26990,#26991,#26992,#26993,#26994,#26995,#26996,#26997,#26998,#26999,#27000,
#27001,#27002,#27003,#27004,#27005,#27006,#27007,#27008,#27009,#27010,#27011,
#27012,#27013,#27014,#27015,#27016,#27017,#27018,#27019,#27020,#27021,#27022,
#27023,#27024,#27025,#27026,#27027,#27028,#27029,#27030,#27031,#27032,#27033,
#27034,#27035,#27036,#27037,#27038,#27039,#27040,#27041,#27042,#27043,#27044,
#27045,#27046,#27047,#27048,#27049,#27050,#27051,#27052,#27053,#27054,#27055,
#27056,#27057,#27058,#27059,#27060,#27061,#27062,#27063,#27064,#27065,#27066,
#27067,#27068,#27069,#27070,#27071,#27072,#27073,#27074,#27075,#27076,#27077,
#27078,#27079,#27080,#27081,#27082,#27083,#27084,#27085,#27086,#27087,#27088,
#27089,#27090,#27091,#27092,#27093,#27094,#27095,#27096,#27097,#27098,#27099,
#27100,#27101,#27102,#27103,#27104,#27105,#27106,#27107,#27108,#27109,#27110,
#27111,#27112,#27113,#27114,#27115,#27116,#27117,#27118,#27119,#27120,#27121,
#27122,#27123,#27124,#27125,#27126,#27127,#27128,#27129,#27130,#27131,#27132,
#27133,#27134,#27135,#27136,#27137,#27138,#27139,#27140,#27141,#27142,#27143,
#27144,#27145,#27146,#27147,#27148,#27149,#27150,#27151,#27152,#27153,#27154,
#27155,#27156,#27157,#27158,#27159,#27160,#27161,#27162,#27163,#27164,#27165,
#27166,#27167,#27168,#27169,#27170,#27171,#27172,#27173,#27174,#27175,#27176,
#27177,#27178,#27179,#27180,#27181,#27182,#27183,#27184,#27185,#27186,#27187,
#27188,#27189,#27190,#27191,#27192,#27193,#27194,#27195,#27196,#27197,#27198,
#27199,#27200,#27201,#27202,#27203,#27204,#27205,#27206,#27207,#27208,#27209,
#27210,#27211,#27212,#27213,#27214,#27215,#27216,#27217,#27218,#27219,#27220,
#27221,#27222,#27223,#27224,#27225,#27226,#27227,#27228,#27229,#27230,#27231,
#27232,#27233,#27234,#27235,#27236,#27237,#27238,#27239,#27240,#27241,#27242,
#27243,#27244,#27245,#27246,#27247,#27248,#27249,#27250,#27251,#27252,#27253,
#27254,#27255,#27256,#27257,#27258,#27259,#27260,#27261,#27262,#27263,#27264,
#27265,#27266,#27267,#27268,#27269,#27270,#27271,#27272,#27273,#27274,#27275,
#27276,#27277,#27278,#27279,#27280,#27281,#27282,#27283,#27284,#27285,#27286,
#27287,#27288,#27289,#27290,#27291,#27292,#27293,#27294),(#27295,#27296,
#27297,#27298,#27299,#27300,#27301,#27302,#27303,#27304,#27305,#27306,#27307,
#27308,#27309,#27310,#27311,#27312,#27313,#27314,#27315,#27316,#27317,#27318,
#27319,#27320,#27321,#27322,#27323,#27324,#27325,#27326,#27327,#27328,#27329,
#27330,#27331,#27332,#27333,#27334,#27335,#27336,#27337,#27338,#27339,#27340,
#27341,#27342,#27343,#27344,#27345,#27346,#27347,#27348,#27349,#27350,#27351,
#27352,#27353,#27354,#27355,#27356,#27357,#27358,#27359,#27360,#27361,#27362,
#27363,#27364,#27365,#27366,#27367,#27368,#27369,#27370,#27371,#27372,#27373,
#27374,#27375,#27376,#27377,#27378,#27379,#27380,#27381,#27382,#27383,#27384,
#27385,#27386,#27387,#27388,#27389,#27390,#27391,#27392,#27393,#27394,#27395,
#27396,#27397,#27398,#27399,#27400,#27401,#27402,#27403,#27404,#27405,#27406,
#27407,#27408,#27409,#27410,#27411,#27412,#27413,#27414,#27415,#27416,#27417,
#27418,#27419,#27420,#27421,#27422,#27423,#27424,#27425,#27426,#27427,#27428,
#27429,#27430,#27431,#27432,#27433,#27434,#27435,#27436,#27437,#27438,#27439,
#27440,#27441,#27442,#27443,#27444,#27445,#27446,#27447,#27448,#27449,#27450,
#27451,#27452,#27453,#27454,#27455,#27456,#27457,#27458,#27459,#27460,#27461,
#27462,#27463,#27464,#27465,#27466,#27467,#27468,#27469,#27470,#27471,#27472,
#27473,#27474,#27475,#27476,#27477,#27478,#27479,#27480,#27481,#27482,#27483,
#27484,#27485,#27486,#27487,#27488,#27489,#27490,#27491,#27492,#27493,#27494,
#27495,#27496,#27497,#27498,#27499,#27500,#27501,#27502,#27503,#27504,#27505,
#27506,#27507,#27508,#27509,#27510,#27511,#27512,#27513,#27514,#27515,#27516,
#27517,#27518,#27519,#27520,#27521,#27522,#27523,#27524,#27525,#27526,#27527,
#27528,#27529,#27530,#27531,#27532,#27533,#27534,#27535,#27536,#27537,#27538,
#27539,#27540,#27541,#27542,#27543,#27544,#27545,#27546,#27547,#27548,#27549,
#27550,#27551,#27552,#27553,#27554,#27555,#27556,#27557,#27558,#27559,#27560,
#27561,#27562,#27563,#27564,#27565,#27566,#27567,#27568,#27569,#27570,#27571,
#27572,#27573,#27574,#27575,#27576,#27577,#27578,#27579,#27580,#27581,#27582,
#27583,#27584,#27585,#27586,#27587,#27588,#27589,#27590,#27591,#27592,#27593,
#27594,#27595,#27596,#27597,#27598,#27599,#27600,#27601,#27602,#27603,#27604,
#27605,#27606,#27607,#27608,#27609,#27610,#27611,#27612,#27613,#27614,#27615,
#27616,#27617,#27618,#27619,#27620,#27621,#27622,#27623,#27624,#27625,#27626,
#27627,#27628,#27629,#27630,#27631,#27632,#27633,#27634,#27635,#27636,#27637,
#27638,#27639,#27640,#27641,#27642,#27643,#27644,#27645,#27646,#27647,#27648,
#27649,#27650,#27651,#27652,#27653,#27654,#27655,#27656,#27657,#27658,#27659,
#27660,#27661,#27662,#27663,#27664,#27665,#27666,#27667,#27668,#27669,#27670,
#27671,#27672,#27673,#27674,#27675,#27676,#27677,#27678,#27679,#27680,#27681,
#27682,#27683,#27684,#27685,#27686,#27687,#27688,#27689,#27690,#27691,#27692,
#27693,#27694,#27695,#27696,#27697,#27698,#27699,#27700,#27701,#27702,#27703,
#27704,#27705,#27706,#27707,#27708,#27709,#27710,#27711,#27712,#27713,#27714,
#27715,#27716,#27717,#27718,#27719,#27720,#27721,#27722,#27723,#27724,#27725,
#27726,#27727,#27728,#27729,#27730,#27731,#27732,#27733,#27734,#27735,#27736,
#27737,#27738,#27739,#27740,#27741,#27742,#27743,#27744,#27745,#27746,#27747,
#27748,#27749,#27750,#27751,#27752,#27753,#27754,#27755,#27756,#27757,#27758,
#27759,#27760,#27761,#27762,#27763,#27764,#27765,#27766,#27767,#27768,#27769,
#27770,#27771,#27772,#27773,#27774,#27775,#27776,#27777,#27778,#27779,#27780,
#27781,#27782,#27783,#27784,#27785,#27786,#27787,#27788,#27789,#27790,#27791,
#27792,#27793,#27794,#27795,#27796,#27797,#27798,#27799,#27800,#27801,#27802,
#27803,#27804,#27805,#27806,#27807,#27808,#27809,#27810,#27811,#27812,#27813,
#27814,#27815,#27816,#27817,#27818,#27819,#27820,#27821,#27822,#27823,#27824,
#27825,#27826,#27827,#27828,#27829,#27830,#27831,#27832,#27833,#27834,#27835,
#27836,#27837,#27838,#27839,#27840,#27841,#27842,#27843,#27844,#27845,#27846,
#27847,#27848,#27849,#27850,#27851,#27852,#27853,#27854,#27855,#27856,#27857,
#27858,#27859,#27860,#27861,#27862,#27863,#27864,#27865,#27866,#27867,#27868,
#27869,#27870,#27871,#27872,#27873,#27874,#27875,#27876,#27877,#27878,#27879,
#27880,#27881,#27882,#27883,#27884,#27885,#27886,#27887,#27888,#27889,#27890,
#27891,#27892,#27893,#27894,#27895,#27896,#27897,#27898,#27899,#27900,#27901,
#27902,#27903,#27904,#27905,#27906,#27907,#27908,#27909,#27910,#27911,#27912,
#27913,#27914,#27915,#27916,#27917,#27918,#27919,#27920,#27921,#27922,#27923,
#27924,#27925,#27926,#27927,#27928,#27929,#27930,#27931,#27932,#27933,#27934,
#27935,#27936,#27937,#27938,#27939,#27940,#27941,#27942,#27943,#27944,#27945,
#27946,#27947,#27948,#27949,#27950,#27951,#27952,#27953,#27954,#27955,#27956,
#27957,#27958,#27959,#27960,#27961,#27962,#27963,#27964,#27965,#27966,#27967,
#27968,#27969,#27970,#27971,#27972,#27973,#27974,#27975,#27976)),
 .UNSPECIFIED.,.F.,.F.,.F.,(4,4),(4,1,1,1,1,1,1,1,1,1,1,1,1,1,1,1,1,1,1,
1,1,1,1,1,1,1,1,1,1,1,1,1,1,1,1,1,1,1,1,1,1,1,1,1,1,1,1,1,1,1,1,1,1,1,1,
1,1,1,1,1,1,1,1,1,1,1,1,1,1,1,1,1,1,1,1,1,1,1,1,1,1,1,1,1,1,1,1,1,1,1,1,
1,1,1,1,1,1,1,1,1,1,1,1,1,1,1,1,1,1,1,1,1,1,1,1,1,1,1,1,1,1,1,1,1,1,1,1,
1,1,1,1,1,1,1,1,1,1,1,1,1,1,1,1,1,1,1,1,1,1,1,1,1,1,1,1,1,1,1,1,1,1,1,1,
1,1,1,1,1,1,1,1,1,1,1,1,1,1,1,1,1,1,1,1,1,1,1,1,1,1,1,1,1,1,1,1,1,1,1,1,
1,1,1,1,1,1,1,1,1,1,1,1,1,1,1,1,1,1,1,1,1,1,1,1,1,1,1,1,1,1,1,1,1,1,1,1,
1,1,1,1,1,1,1,1,1,1,1,1,1,1,1,1,1,1,1,1,1,1,1,1,1,1,1,1,1,1,1,1,1,1,1,1,
1,1,1,1,1,1,1,1,1,1,1,1,1,1,1,1,1,1,1,1,1,1,1,1,1,1,1,1,1,1,1,1,1,1,1,1,
1,1,1,1,1,1,1,1,1,1,1,1,1,1,1,1,1,1,1,1,1,1,1,1,1,1,1,1,1,1,1,1,1,1,1,1,
1,1,1,1,1,1,1,1,1,1,1,1,1,1,1,1,1,1,1,1,1,1,1,1,1,1,1,1,1,1,1,1,1,1,1,1,
1,1,1,1,1,1,1,1,1,1,1,1,1,1,1,1,1,1,1,1,1,1,1,1,1,1,1,1,1,1,1,1,1,1,1,1,
1,1,1,1,1,1,1,1,1,1,1,1,1,1,1,1,1,1,1,1,1,1,1,1,1,1,1,1,1,1,1,1,1,1,1,1,
1,1,1,1,1,1,1,1,1,1,1,1,1,1,1,1,1,1,1,1,1,1,1,1,1,1,1,1,1,1,1,1,1,1,1,1,
1,1,1,1,1,1,1,1,1,1,1,1,1,1,1,1,1,1,1,1,1,1,1,1,1,1,1,1,1,1,1,1,1,1,1,1,
1,1,1,1,1,1,1,1,1,1,1,1,1,1,1,1,1,1,1,1,1,1,1,1,1,1,1,1,1,1,1,1,1,1,1,1,
1,1,1,1,1,1,1,1,1,1,1,1,1,1,1,1,1,1,1,1,1,1,1,1,1,1,1,1,1,1,1,1,1,1,1,1,
1,1,1,1,1,1,1,1,1,1,1,1,1,1,1,1,1,1,1,1,1,1,1,1,1,1,1,1,1,1,1,1,1,1,1,1,
1,1,1,1,1,1,1,1,1,1,1,1,1,1,1,1,1,1,1,1,1,1,1,1,1,1,1,1,1,1,1,1,1,1,1,1,
1,1,1,1,1,1,1,1,1,1,1,1,4),(0.,0.198319817466637),(11.6150328478198,12.1147767088206,
12.6145205698214,13.614008291823,14.6134960138245,15.6129837358261,16.1127275968269,
16.6124714578277,17.6119591798292,18.6114469018308,19.6109346238324,20.6104223458339,
21.6099100678355,22.1096539288363,22.6093977898371,23.6088855118386,24.6083732338402,
25.6078609558418,26.6073486778433,27.6068363998449,28.6063241218465,29.1060679828472,
29.605811843848,30.6052995658496,31.6047872878512,32.6042750098527,33.6037627318543,
34.6032504538559,35.6027381758574,36.1024820368582,36.602225897859,37.6017136198606,
38.6012013418621,39.6006890638637,40.6001767858653,41.5996645078668,42.5991522298684,
43.0988960908692,43.59863995187,44.5981276738715,45.5976153958731,46.5971031178747,
47.5965908398762,48.5960785618778,49.5955662838794,50.0953101448802,50.5950540058809,
51.5945417278825,52.5940294498841,53.5935171718856,54.5930048938872,55.5924926158888,
56.5919803378903,57.0917241988911,57.5914680598919,58.5909557818935,59.590443503895,
60.5899312258966,61.5894189478982,62.5889066698997,63.5883943919013,64.0881382529021,
64.5878821139029,65.5873698359044,66.586857557906,67.5863452799076,68.5858330019091,
69.5853207239107,70.5848084459123,71.0845523069131,71.5842961679138,72.5837838899154,
73.583271611917,74.5827593339185,75.5822470559201,76.5817347779217,77.5812224999232,
78.080966360924,78.5807102219248,79.5801979439264,80.5796856659279,81.5791733879295,
82.5786611099311,83.5781488319326,84.5776365539342,85.077380414935,85.5771242759358,
86.5766119979373,87.5760997199389,88.5755874419405,89.575075163942,90.5745628859436,
91.5740506079452,92.073794468946,92.5735383299467,93.5730260519483,94.5725137739499,
95.5720014959514,96.571489217953,97.5709769399546,98.5704646619562,99.0702085229569,
99.5699523839577,100.569440105959,101.568927827961,102.568415549962,103.567903271964,
104.567390993966,105.566878715967,106.066622576968,106.566366437969,107.56585415997,
108.565341881972,109.564829603973,110.564317325975,111.563805047977,112.563292769978,
113.063036630979,113.56278049198,114.562268213981,115.561755935983,116.561243657984,
117.560731379986,118.560219101987,119.559706823989,120.05945068499,120.559194545991,
121.558682267992,122.558169989994,123.557657711995,124.557145433997,125.556633155998,
126.556120878,127.055864739001,127.555608600002,128.555096322003,129.554584044005,
130.554071766006,131.553559488008,132.553047210009,133.552534932011,134.052278793012,
134.552022654013,135.551510376014,136.550998098016,137.550485820017,138.549973542019,
139.54946126402,140.548948986022,141.048692847023,141.548436708024,142.547924430025,
143.547412152027,144.546899874028,145.54638759603,146.545875318031,147.545363040033,
148.045106901034,148.544850762035,149.544338484036,150.543826206038,151.543313928039,
152.542801650041,153.542289372042,154.541777094044,155.041520955045,155.541264816045,
156.540752538047,157.540240260049,158.53972798205,159.539215704052,160.538703426053,
161.538191148055,162.037935009056,162.537678870056,163.537166592058,164.53665431406,
165.536142036061,166.535629758063,167.535117480064,168.534605202066,169.034349063067,
169.534092924067,170.533580646069,171.533068368071,172.532556090072,173.532043812074,
174.531531534075,175.531019256077,176.030763117078,176.530506978078,177.52999470008,
178.529482422082,179.528970144083,180.528457866085,181.527945588086,182.527433310088,
183.027177171089,183.526921032089,184.526408754091,185.525896476092,186.525384198094,
187.524871920096,188.524359642097,189.523847364099,190.0235912251,190.5233350861,
191.522822808102,192.522310530103,193.521798252105,194.521285974107,195.520773696108,
196.52026141811,197.020005279111,197.519749140111,198.519236862113,199.518724584114,
200.518212306116,201.517700028118,202.517187750119,203.516675472121,204.016419333121,
204.516163194122,205.515650916124,206.515138638125,207.514626360127,208.514114082129,
209.51360180413,210.513089526132,211.012833387132,211.512577248133,212.512064970135,
213.511552692136,214.511040414138,215.510528136139,216.510015858141,217.509503580143,
218.009247441143,218.508991302144,219.508479024146,220.507966746147,221.507454468149,
222.50694219015,223.506429912152,224.505917634154,225.005661495154,225.505405356155,
226.504893078157,227.504380800158,228.50386852216,229.503356244161,230.502843966163,
231.502331688165,232.002075549165,232.501819410166,233.501307132168,234.500794854169,
235.500282576171,236.499770298172,237.499258020174,238.498745742176,238.998489603176,
239.498233464177,240.497721186179,241.49720890818,242.496696630182,243.496184352183,
244.495672074185,245.495159796186,245.994903657187,246.494647518188,247.49413524019,
248.493622962191,249.493110684193,250.492598406194,251.492086128196,252.491573850197,
252.991317711198,253.491061572199,254.490549294201,255.490037016202,256.489524738204,
257.489012460205,258.488500182207,259.487987904208,259.987731765209,260.48747562621,
261.486963348212,262.486451070213,263.485938792215,264.485426514216,265.484914236218,
266.484401958219,266.98414581922,267.483889680221,268.483377402223,269.482865124224,
270.482352846226,271.481840568227,272.481328290229,273.48081601223,273.980559873231,
274.480303734232,275.479791456233,276.479279178235,277.478766900237,278.478254622238,
279.47774234424,280.477230066241,280.976973927242,281.476717788243,282.476205510244,
283.475693232246,284.475180954248,285.474668676249,286.474156398251,287.473644120252,
287.973387981253,288.473131842254,289.472619564255,290.472107286257,291.471595008259,
292.47108273026,293.470570452262,294.470058174263,294.969802035264,295.469545896265,
296.469033618266,297.468521340268,298.46800906227,299.467496784271,300.466984506273,
301.466472228274,301.966216089275,302.465959950276,303.465447672277,304.464935394279,
305.46442311628,306.463910838282,307.463398560284,308.462886282285,309.462374004287,
310.461861726288,311.46134944829,312.460837170291,313.460324892293,313.960068753294,
314.459812614295,315.459300336296,316.458788058298,317.458275780299,318.457763502301,
319.457251224302,320.456738946304,320.956482807305,321.456226668306,322.455714390307,
323.455202112309,324.45468983431,325.454177556312,326.453665278313,327.453153000315,
327.952896861316,328.452640722317,329.452128444318,330.45161616632,331.451103888321,
332.450591610323,333.450079332324,334.449567054326,334.949310915327,335.449054776328,
336.448542498329,337.448030220331,338.447517942332,339.447005664334,340.446493386335,
341.445981108337,341.945724969338,342.445468830338,343.44495655234,344.444444274342,
345.443931996343,346.443419718345,347.442907440346,348.442395162348,348.942139023349,
349.441882884349,350.441370606351,351.440858328353,352.440346050354,353.439833772356,
354.439321494357,355.438809216359,355.93855307736,356.43829693836,357.437784660362,
358.437272382364,359.436760104365,360.436247826367,361.435735548368,362.43522327037,
362.934967131371,363.434710992371,364.434198714373,365.433686436375,366.433174158376,
367.432661880378,368.432149602379,369.431637324381,369.931381185382,370.431125046382,
371.430612768384,372.430100490385,373.429588212387,374.429075934389,375.42856365639,
376.428051378392,376.927795239393,377.427539100393,378.427026822395,379.426514544396,
380.426002266398,381.4254899884,382.424977710401,383.424465432403,383.924209293403,
384.423953154404,385.423440876406,386.422928598407,387.422416320409,388.421904042411,
389.421391764412,390.420879486414,390.920623347414,391.420367208415,392.419854930417,
393.419342652418,394.41883037442,395.418318096422,396.417805818423,397.417293540425,
397.917037401425,398.416781262426,399.416268984428,400.415756706429,401.415244428431,
402.414732150432,403.414219872434,404.413707594436,404.913451455436,405.413195316437,
406.412683038439,407.41217076044,408.411658482442,409.411146204443,410.410633926445,
411.410121648447,411.909865509447,412.409609370448,413.40909709245,414.408584814451,
415.408072536453,416.407560258454,417.407047980456,418.406535702458,418.906279563458,
419.406023424459,420.405511146461,421.404998868462,422.404486590464,423.403974312465,
424.403462034467,425.402949756469,425.902693617469,426.40243747847,427.401925200472,
428.401412922473,429.400900644475,430.400388366476,431.399876088478,432.399363810479,
432.89910767148,433.398851532481,434.398339254483,435.397826976484,436.397314698486,
437.396802420487,438.396290142489,439.39577786449,439.895521725491,440.395265586492,
441.394753308494,442.394241030495,443.393728752497,444.393216474498,445.3927041965,
446.392191918501,446.891935779502,447.391679640503,448.391167362505,449.390655084506,
450.390142806508,451.389630528509,452.389118250511,453.388605972512,453.888349833513,
454.388093694514,455.387581416516,456.387069138517,457.386556860519,458.38604458252,
459.385532304522,460.385020026523,460.884763887524,461.384507748525,462.383995470527,
463.383483192528,464.38297091453,465.382458636531,466.381946358533,467.381434080534,
467.881177941535,468.380921802536,469.380409524537,470.379897246539,471.379384968541,
472.378872690542,473.378360412544,474.377848134545,474.877591995546,475.377335856547,
476.376823578548,477.37631130055,478.375799022552,479.375286744553,480.374774466555,
481.374262188556,481.874006049557,482.373749910558,483.373237632559,484.372725354561,
485.372213076563,486.371700798564,487.371188520566,488.370676242567,488.870420103568,
489.370163964569,490.36965168657,491.369139408572,492.368627130574,493.368114852575,
494.367602574577,495.367090296578,495.866834157579,496.36657801858,497.366065740581,
498.365553462583,499.365041184584,500.364528906586,501.364016628588,502.363504350589,
502.86324821159,503.362992072591,504.362479794592,505.361967516594,506.361455238595,
507.360942960597,508.360430682599,509.3599184046,509.859662265601,510.359406126602,
511.358893848603,512.358381570605,513.357869292606,514.357357014608,515.35684473661,
516.356332458611,516.856076319612,517.355820180613,518.355307902614,519.354795624616,
520.354283346617,521.353771068619,522.353258790621,523.352746512622,523.852490373623,
524.352234234624,525.351721956625,526.351209678627,527.350697400628,528.35018512263,
529.349672844632,530.349160566633,530.848904427634,531.348648288635,532.348136010636,
533.347623732638,534.347111454639,535.346599176641,536.346086898643,537.345574620644,
537.845318481645,538.345062342646,539.344550064647,540.344037786649,541.34352550865,
542.343013230652,543.342500952653,544.341988674655,544.841732535656,545.341476396657,
546.340964118658,547.34045184066,548.339939562661,549.339427284663,550.338915006664,
551.338402728666,551.838146589667,552.337890450668,553.337378172669,554.336865894671,
555.336353616672,556.335841338674,557.335329060675,558.334816782677,558.834560643678,
559.334304504679,560.33379222668,561.333279948682,562.332767670683,563.332255392685,
564.331743114686,565.331230836688,565.830974697689,566.33071855869,567.330206280691,
568.329694002693,569.329181724694,570.328669446696,571.328157168697,572.327644890699,
572.8273887517,573.327132612701,574.326620334702,575.326108056704,576.325595778705,
577.325083500707,578.324571222708,579.32405894471,579.823802805711,580.323546666712,
581.323034388713,582.322522110715,583.322009832716,584.321497554718,585.320985276719,
586.320472998721,586.820216859722,587.319960720722,588.319448442724,589.318936164726,
590.318423886727,591.317911608729,592.31739933073,593.316887052732,593.816630913733,
594.316374774733,595.315862496735,596.315350218737,597.314837940738,598.31432566274,
599.313813384741,599.813557245742,600.313301106743,601.312788828744,602.312276550746,
603.311764272747,603.811508133748,604.311251994749),.UNSPECIFIED.);
#217=B_SPLINE_CURVE_WITH_KNOTS('',3,(#11779,#11780,#11781,#11782,#11783,
#11784,#11785,#11786,#11787,#11788),.UNSPECIFIED.,.F.,.F.,(4,3,3,4),(-4.09293042013064,
-3.3387479513909,-2.58456548265116,-2.07680027204819),.UNSPECIFIED.);
#218=B_SPLINE_CURVE_WITH_KNOTS('',3,(#11791,#11792,#11793,#11794,#11795,
#11796,#11797,#11798,#11799,#11800),.UNSPECIFIED.,.F.,.F.,(4,3,3,4),(0.,
0.49974386100078,0.99948772200156,1.12546250550931),.UNSPECIFIED.);
#219=B_SPLINE_CURVE_WITH_KNOTS('',3,(#11805,#11806,#11807,#11808,#11809,
#11810,#11811,#11812,#11813,#11814,#11815,#11816,#11817,#11818,#11819,#11820,
#11821,#11822,#11823,#11824,#11825,#11826,#11827,#11828,#11829),
 .UNSPECIFIED.,.F.,.F.,(4,3,3,3,3,3,3,3,4),(-10.3761157273102,-9.99487722001567,
-8.9953894980141,-7.99590177601253,-6.99641405401097,-5.9969263320094,-4.99743861000784,
-4.49769474900705,-4.09293042013064),.UNSPECIFIED.);
#220=B_SPLINE_CURVE_WITH_KNOTS('',3,(#11830,#11831,#11832,#11833,#11834,
#11835,#11836,#11837,#11838,#11839,#11840,#11841,#11842,#11843,#11844,#11845,
#11846,#11847,#11848,#11849,#11850,#11851,#11852,#11853,#11854),
 .UNSPECIFIED.,.F.,.F.,(4,3,3,3,3,3,3,3,4),(1.12546250550931,1.99897544400314,
2.99846316600472,3.99795088800629,4.49769474900708,4.99743861000787,5.99692633200945,
6.99641405401103,7.4086478126889),.UNSPECIFIED.);
#221=B_SPLINE_CURVE_WITH_KNOTS('',3,(#11859,#11860,#11861,#11862,#11863,
#11864,#11865,#11866,#11867,#11868,#11869,#11870,#11871,#11872,#11873,#11874,
#11875,#11876,#11877,#11878,#11879,#11880,#11881,#11882,#11883,#11884,#11885,
#11886),.UNSPECIFIED.,.F.,.F.,(4,3,3,3,3,3,3,3,3,4),(-16.6593010344898,
-15.9051185657501,-15.1509360970104,-14.3967536282706,-13.6425711595309,
-12.8883886907912,-12.1342062220514,-11.3800237533117,-10.625841284572,
-10.3761157273102),.UNSPECIFIED.);
#222=B_SPLINE_CURVE_WITH_KNOTS('',3,(#11887,#11888,#11889,#11890,#11891,
#11892,#11893,#11894,#11895,#11896,#11897,#11898,#11899,#11900,#11901,#11902,
#11903,#11904,#11905,#11906,#11907,#11908,#11909,#11910,#11911,#11912,#11913,
#11914),.UNSPECIFIED.,.F.,.F.,(4,3,3,3,3,3,3,3,3,4),(7.4086478126889,8.16283028142863,
8.91701275016836,9.67119521890809,10.4253776876478,11.1795601563876,11.9337426251273,
12.687925093867,13.4421075626068,13.6918331198685),.UNSPECIFIED.);
#223=B_SPLINE_CURVE_WITH_KNOTS('',3,(#11919,#11920,#11921,#11922,#11923,
#11924,#11925,#11926,#11927,#11928,#11929,#11930,#11931,#11932,#11933,#11934,
#11935,#11936,#11937,#11938,#11939,#11940,#11941,#11942,#11943,#11944,#11945,
#11946),.UNSPECIFIED.,.F.,.F.,(4,3,3,3,3,3,3,3,3,4),(-22.9424863416694,
-22.1883038729297,-21.4341214041899,-20.6799389354502,-19.9257564667105,
-19.1715739979707,-18.417391529231,-17.6632090604913,-16.9090265917515,
-16.6593010344898),.UNSPECIFIED.);
#224=B_SPLINE_CURVE_WITH_KNOTS('',3,(#11947,#11948,#11949,#11950,#11951,
#11952,#11953,#11954,#11955,#11956,#11957,#11958,#11959,#11960,#11961,#11962,
#11963,#11964,#11965,#11966,#11967,#11968,#11969,#11970,#11971),
 .UNSPECIFIED.,.F.,.F.,(4,3,3,3,3,3,3,3,4),(13.6918331198685,13.9928281080218,
14.9923158300234,15.991803552025,16.9912912740266,17.4910351350274,17.9907789960282,
18.9902667180298,19.9750184270481),.UNSPECIFIED.);
#225=B_SPLINE_CURVE_WITH_KNOTS('',3,(#11976,#11977,#11978,#11979,#11980,
#11981,#11982,#11983,#11984,#11985,#11986,#11987,#11988,#11989,#11990,#11991,
#11992,#11993,#11994,#11995,#11996,#11997,#11998,#11999,#12000,#12001,#12002,
#12003),.UNSPECIFIED.,.F.,.F.,(4,3,3,3,3,3,3,3,3,4),(-29.225671648849,-28.4714891801093,
-27.7173067113695,-26.9631242426298,-26.2089417738901,-25.4547593051504,
-24.7005768364106,-23.9463943676709,-23.1922118989312,-22.9424863416694),
 .UNSPECIFIED.);
#226=B_SPLINE_CURVE_WITH_KNOTS('',3,(#12004,#12005,#12006,#12007,#12008,
#12009,#12010,#12011,#12012,#12013,#12014,#12015,#12016,#12017,#12018,#12019,
#12020,#12021,#12022,#12023,#12024,#12025,#12026,#12027,#12028,#12029,#12030,
#12031),.UNSPECIFIED.,.F.,.F.,(4,3,3,3,3,3,3,3,3,4),(19.9750184270481,20.7292008957878,
21.4833833645275,22.2375658332673,22.991748302007,23.7459307707468,24.5001132394865,
25.2542957082262,26.008478176966,26.2582037342277),.UNSPECIFIED.);
#227=B_SPLINE_CURVE_WITH_KNOTS('',3,(#12036,#12037,#12038,#12039,#12040,
#12041,#12042,#12043,#12044,#12045,#12046,#12047,#12048,#12049,#12050,#12051,
#12052,#12053,#12054,#12055,#12056,#12057,#12058,#12059,#12060,#12061,#12062,
#12063),.UNSPECIFIED.,.F.,.F.,(4,3,3,3,3,3,3,3,3,4),(-35.5088569560286,
-34.7546744872888,-34.0004920185491,-33.2463095498094,-32.4921270810696,
-31.7379446123299,-30.9837621435901,-30.2295796748504,-29.4753972061106,
-29.225671648849),.UNSPECIFIED.);
#228=B_SPLINE_CURVE_WITH_KNOTS('',3,(#12064,#12065,#12066,#12067,#12068,
#12069,#12070,#12071,#12072,#12073,#12074,#12075,#12076,#12077,#12078,#12079,
#12080,#12081,#12082,#12083,#12084,#12085,#12086,#12087,#12088,#12089,#12090,
#12091),.UNSPECIFIED.,.F.,.F.,(4,3,3,3,3,3,3,3,3,4),(26.2582037342277,27.0123862029674,
27.7665686717072,28.5207511404469,29.2749336091866,30.0291160779264,30.7832985466661,
31.5374810154059,32.2916634841456,32.5413890414072),.UNSPECIFIED.);
#229=B_SPLINE_CURVE_WITH_KNOTS('',3,(#12096,#12097,#12098,#12099,#12100,
#12101,#12102,#12103,#12104,#12105,#12106,#12107,#12108,#12109,#12110,#12111,
#12112,#12113,#12114,#12115,#12116,#12117,#12118,#12119,#12120),
 .UNSPECIFIED.,.F.,.F.,(4,3,3,3,3,3,3,3,4),(-41.7920422632082,-40.9789966020643,
-39.9795088800627,-38.9800211580611,-38.4802772970603,-37.9805334360596,
-36.981045714058,-35.9815579920564,-35.5088569560286),.UNSPECIFIED.);
#230=B_SPLINE_CURVE_WITH_KNOTS('',3,(#12121,#12122,#12123,#12124,#12125,
#12126,#12127,#12128,#12129,#12130,#12131,#12132,#12133,#12134,#12135,#12136,
#12137,#12138,#12139,#12140,#12141,#12142,#12143,#12144,#12145,#12146,#12147,
#12148),.UNSPECIFIED.,.F.,.F.,(4,3,3,3,3,3,3,3,3,4),(32.5413890414072,33.295571510147,
34.0497539788867,34.8039364476264,35.5581189163662,36.3123013851059,37.0664838538456,
37.8206663225853,38.5748487913251,38.8245743485868),.UNSPECIFIED.);
#231=B_SPLINE_CURVE_WITH_KNOTS('',3,(#12153,#12154,#12155,#12156,#12157,
#12158,#12159,#12160,#12161,#12162,#12163,#12164,#12165,#12166,#12167,#12168,
#12169,#12170,#12171,#12172,#12173,#12174,#12175,#12176,#12177,#12178,#12179,
#12180),.UNSPECIFIED.,.F.,.F.,(4,3,3,3,3,3,3,3,3,4),(-48.0752275703878,
-47.321045101648,-46.5668626329083,-45.8126801641685,-45.0584976954288,
-44.304315226689,-43.5501327579493,-42.7959502892096,-42.0417678204698,
-41.7920422632082),.UNSPECIFIED.);
#232=B_SPLINE_CURVE_WITH_KNOTS('',3,(#12181,#12182,#12183,#12184,#12185,
#12186,#12187,#12188,#12189,#12190,#12191,#12192,#12193,#12194,#12195,#12196,
#12197,#12198,#12199,#12200,#12201,#12202,#12203,#12204,#12205,#12206,#12207,
#12208),.UNSPECIFIED.,.F.,.F.,(4,3,3,3,3,3,3,3,3,4),(38.8245743485868,39.5787568173266,
40.3329392860663,41.087121754806,41.8413042235457,42.5954866922855,43.3496691610252,
44.1038516297649,44.8580340985047,45.1077596557664),.UNSPECIFIED.);
#233=B_SPLINE_CURVE_WITH_KNOTS('',3,(#12213,#12214,#12215,#12216,#12217,
#12218,#12219,#12220,#12221,#12222,#12223,#12224,#12225,#12226,#12227,#12228,
#12229,#12230,#12231,#12232,#12233,#12234,#12235,#12236,#12237,#12238,#12239,
#12240),.UNSPECIFIED.,.F.,.F.,(4,3,3,3,3,3,3,3,3,4),(-54.3584128775674,
-53.6042304088276,-52.8500479400879,-52.0958654713482,-51.3416830026084,
-50.5875005338687,-49.833318065129,-49.0791355963893,-48.3249531276495,
-48.0752275703878),.UNSPECIFIED.);
#234=B_SPLINE_CURVE_WITH_KNOTS('',3,(#12241,#12242,#12243,#12244,#12245,
#12246,#12247,#12248,#12249,#12250,#12251,#12252,#12253,#12254,#12255,#12256,
#12257,#12258,#12259,#12260,#12261,#12262,#12263,#12264,#12265,#12266,#12267,
#12268),.UNSPECIFIED.,.F.,.F.,(4,3,3,3,3,3,3,3,3,4),(45.1077596557664,45.8619421245062,
46.6161245932459,47.3703070619856,48.1244895307253,48.8786719994651,49.6328544682048,
50.3870369369445,51.1412194056842,51.390944962946),.UNSPECIFIED.);
#235=B_SPLINE_CURVE_WITH_KNOTS('',3,(#12273,#12274,#12275,#12276,#12277,
#12278,#12279,#12280,#12281,#12282,#12283,#12284,#12285,#12286,#12287,#12288,
#12289,#12290,#12291,#12292,#12293,#12294,#12295,#12296,#12297,#12298,#12299,
#12300),.UNSPECIFIED.,.F.,.F.,(4,3,3,3,3,3,3,3,3,4),(-60.6415981847469,
-59.8874157160072,-59.1332332472675,-58.3790507785277,-57.624868309788,
-56.8706858410483,-56.1165033723085,-55.3623209035688,-54.6081384348291,
-54.3584128775674),.UNSPECIFIED.);
#236=B_SPLINE_CURVE_WITH_KNOTS('',3,(#12301,#12302,#12303,#12304,#12305,
#12306,#12307,#12308,#12309,#12310,#12311,#12312,#12313,#12314,#12315,#12316,
#12317,#12318,#12319,#12320,#12321,#12322,#12323,#12324,#12325,#12326,#12327,
#12328),.UNSPECIFIED.,.F.,.F.,(4,3,3,3,3,3,3,3,3,4),(51.390944962946,52.1451274316857,
52.8993099004255,53.6534923691652,54.4076748379049,55.1618573066447,55.9160397753844,
56.6702222441241,57.4244047128638,57.6741302701256),.UNSPECIFIED.);
#237=B_SPLINE_CURVE_WITH_KNOTS('',3,(#12333,#12334,#12335,#12336,#12337,
#12338,#12339,#12340,#12341,#12342,#12343,#12344,#12345,#12346,#12347,#12348,
#12349,#12350,#12351,#12352,#12353,#12354,#12355,#12356,#12357,#12358,#12359,
#12360),.UNSPECIFIED.,.F.,.F.,(4,3,3,3,3,3,3,3,3,4),(-66.9247834919265,
-66.1706010231868,-65.4164185544471,-64.6622360857073,-63.9080536169676,
-63.1538711482279,-62.3996886794882,-61.6455062107484,-60.8913237420087,
-60.6415981847469),.UNSPECIFIED.);
#238=B_SPLINE_CURVE_WITH_KNOTS('',3,(#12361,#12362,#12363,#12364,#12365,
#12366,#12367,#12368,#12369,#12370,#12371,#12372,#12373,#12374,#12375,#12376,
#12377,#12378,#12379,#12380,#12381,#12382,#12383,#12384,#12385,#12386,#12387,
#12388),.UNSPECIFIED.,.F.,.F.,(4,3,3,3,3,3,3,3,3,4),(57.6741302701256,58.4283127388654,
59.1824952076051,59.9366776763448,60.6908601450845,61.4450426138243,62.199225082564,
62.9534075513037,63.7075900200434,63.9573155773052),.UNSPECIFIED.);
#239=B_SPLINE_CURVE_WITH_KNOTS('',3,(#12393,#12394,#12395,#12396,#12397,
#12398,#12399,#12400,#12401,#12402,#12403,#12404,#12405,#12406,#12407,#12408,
#12409,#12410,#12411,#12412,#12413,#12414,#12415,#12416,#12417,#12418,#12419,
#12420),.UNSPECIFIED.,.F.,.F.,(4,3,3,3,3,3,3,3,3,4),(-73.2079687991061,
-72.4537863303664,-71.6996038616266,-70.9454213928869,-70.1912389241472,
-69.4370564554074,-68.6828739866677,-67.9286915179279,-67.1745090491882,
-66.9247834919265),.UNSPECIFIED.);
#240=B_SPLINE_CURVE_WITH_KNOTS('',3,(#12421,#12422,#12423,#12424,#12425,
#12426,#12427,#12428,#12429,#12430,#12431,#12432,#12433,#12434,#12435,#12436,
#12437,#12438,#12439,#12440,#12441,#12442,#12443,#12444,#12445,#12446,#12447,
#12448),.UNSPECIFIED.,.F.,.F.,(4,3,3,3,3,3,3,3,3,4),(63.9573155773052,63.9672142081004,
64.9667019301019,65.9661896521034,66.4659335131042,66.965677374105,67.9651650961065,
68.9646528181081,69.9641405401096,70.2405008844848),.UNSPECIFIED.);
#241=B_SPLINE_CURVE_WITH_KNOTS('',3,(#12453,#12454,#12455,#12456,#12457,
#12458,#12459,#12460,#12461,#12462,#12463,#12464,#12465,#12466,#12467,#12468,
#12469,#12470,#12471,#12472,#12473,#12474,#12475,#12476,#12477,#12478,#12479,
#12480),.UNSPECIFIED.,.F.,.F.,(4,3,3,3,3,3,3,3,3,4),(-79.4911541062857,
-78.736971637546,-77.9827891688063,-77.2286067000665,-76.4744242313268,
-75.7202417625871,-74.9660592938474,-74.2118768251076,-73.4576943563679,
-73.2079687991061),.UNSPECIFIED.);
#242=B_SPLINE_CURVE_WITH_KNOTS('',3,(#12481,#12482,#12483,#12484,#12485,
#12486,#12487,#12488,#12489,#12490,#12491,#12492,#12493,#12494,#12495,#12496,
#12497,#12498,#12499,#12500,#12501,#12502,#12503,#12504,#12505),
 .UNSPECIFIED.,.F.,.F.,(4,3,3,3,3,3,3,3,4),(70.2405008844848,70.9636282621112,
71.9631159841128,72.9626037061144,73.4623475671152,73.962091428116,74.9615791501176,
75.9610668721191,76.5236861916644),.UNSPECIFIED.);
#243=B_SPLINE_CURVE_WITH_KNOTS('',3,(#12510,#12511,#12512,#12513,#12514,
#12515,#12516,#12517,#12518,#12519,#12520,#12521,#12522,#12523,#12524,#12525,
#12526,#12527,#12528,#12529,#12530,#12531,#12532,#12533,#12534,#12535,#12536,
#12537),.UNSPECIFIED.,.F.,.F.,(4,3,3,3,3,3,3,3,3,4),(-85.7743394134653,
-85.0201569447256,-84.2659744759859,-83.5117920072462,-82.7576095385065,
-82.0034270697667,-81.249244601027,-80.4950621322873,-79.7408796635476,
-79.4911541062857),.UNSPECIFIED.);
#244=B_SPLINE_CURVE_WITH_KNOTS('',3,(#12538,#12539,#12540,#12541,#12542,
#12543,#12544,#12545,#12546,#12547,#12548,#12549,#12550,#12551,#12552,#12553,
#12554,#12555,#12556,#12557,#12558,#12559,#12560,#12561,#12562,#12563,#12564,
#12565),.UNSPECIFIED.,.F.,.F.,(4,3,3,3,3,3,3,3,3,4),(76.5236861916644,77.2778686604041,
78.0320511291438,78.7862335978835,79.5404160666232,80.2945985353629,81.0487810041027,
81.8029634728424,82.5571459415821,82.806871498844),.UNSPECIFIED.);
#245=B_SPLINE_CURVE_WITH_KNOTS('',3,(#12570,#12571,#12572,#12573,#12574,
#12575,#12576,#12577,#12578,#12579,#12580,#12581,#12582,#12583,#12584,#12585,
#12586,#12587,#12588,#12589,#12590,#12591,#12592,#12593,#12594,#12595,#12596,
#12597),.UNSPECIFIED.,.F.,.F.,(4,3,3,3,3,3,3,3,3,4),(-92.0575247206449,
-91.3033422519052,-90.5491597831655,-89.7949773144257,-89.040794845686,
-88.2866123769463,-87.5324299082066,-86.7782474394668,-86.0240649707271,
-85.7743394134653),.UNSPECIFIED.);
#246=B_SPLINE_CURVE_WITH_KNOTS('',3,(#12598,#12599,#12600,#12601,#12602,
#12603,#12604,#12605,#12606,#12607,#12608,#12609,#12610,#12611,#12612,#12613,
#12614,#12615,#12616,#12617,#12618,#12619,#12620,#12621,#12622,#12623,#12624,
#12625),.UNSPECIFIED.,.F.,.F.,(4,3,3,3,3,3,3,3,3,4),(82.806871498844,83.5610539675837,
84.3152364363234,85.0694189050632,85.8236013738029,86.5777838425426,87.3319663112823,
88.0861487800221,88.8403312487618,89.0900568060236),.UNSPECIFIED.);
#247=B_SPLINE_CURVE_WITH_KNOTS('',3,(#12630,#12631,#12632,#12633,#12634,
#12635,#12636,#12637,#12638,#12639,#12640,#12641,#12642,#12643,#12644,#12645,
#12646,#12647,#12648,#12649,#12650,#12651,#12652,#12653,#12654,#12655,#12656,
#12657),.UNSPECIFIED.,.F.,.F.,(4,3,3,3,3,3,3,3,3,4),(-98.3407100278245,
-97.5865275590848,-96.832345090345,-96.0781626216053,-95.3239801528655,
-94.5697976841258,-93.8156152153861,-93.0614327466463,-92.3072502779066,
-92.0575247206449),.UNSPECIFIED.);
#248=B_SPLINE_CURVE_WITH_KNOTS('',3,(#12658,#12659,#12660,#12661,#12662,
#12663,#12664,#12665,#12666,#12667,#12668,#12669,#12670,#12671,#12672,#12673,
#12674,#12675,#12676,#12677,#12678,#12679,#12680,#12681,#12682,#12683,#12684,
#12685),.UNSPECIFIED.,.F.,.F.,(4,3,3,3,3,3,3,3,3,4),(89.0900568060236,89.8442392747633,
90.598421743503,91.3526042122428,92.1067866809825,92.8609691497222,93.615151618462,
94.3693340872017,95.1235165559414,95.3732421132032),.UNSPECIFIED.);
#249=B_SPLINE_CURVE_WITH_KNOTS('',3,(#12690,#12691,#12692,#12693,#12694,
#12695,#12696,#12697,#12698,#12699,#12700,#12701,#12702,#12703,#12704,#12705,
#12706,#12707,#12708,#12709,#12710,#12711,#12712,#12713,#12714,#12715,#12716,
#12717),.UNSPECIFIED.,.F.,.F.,(4,3,3,3,3,3,3,3,3,4),(-104.623895335004,
-103.869712866264,-103.115530397525,-102.361347928785,-101.607165460045,
-100.852982991305,-100.098800522566,-99.344618053826,-98.5904355850863,
-98.3407100278245),.UNSPECIFIED.);
#250=B_SPLINE_CURVE_WITH_KNOTS('',3,(#12718,#12719,#12720,#12721,#12722,
#12723,#12724,#12725,#12726,#12727,#12728,#12729,#12730,#12731,#12732,#12733,
#12734,#12735,#12736,#12737,#12738,#12739,#12740,#12741,#12742,#12743,#12744,
#12745),.UNSPECIFIED.,.F.,.F.,(4,3,3,3,3,3,3,3,3,4),(95.3732421132032,96.1274245819429,
96.8816070506826,97.6357895194223,98.389971988162,99.1441544569017,99.8983369256415,
100.652519394381,101.406701863121,101.656427420383),.UNSPECIFIED.);
#251=B_SPLINE_CURVE_WITH_KNOTS('',3,(#12750,#12751,#12752,#12753,#12754,
#12755,#12756,#12757,#12758,#12759,#12760,#12761,#12762,#12763,#12764,#12765,
#12766,#12767,#12768,#12769,#12770,#12771,#12772,#12773,#12774),
 .UNSPECIFIED.,.F.,.F.,(4,3,3,3,3,3,3,3,4),(-110.907080642184,-109.943649420172,
-108.944161698171,-108.44441783717,-107.944673976169,-106.945186254168,
-105.945698532166,-104.946210810165,-104.623895335004),.UNSPECIFIED.);
#252=B_SPLINE_CURVE_WITH_KNOTS('',3,(#12775,#12776,#12777,#12778,#12779,
#12780,#12781,#12782,#12783,#12784,#12785,#12786,#12787,#12788,#12789,#12790,
#12791,#12792,#12793,#12794,#12795,#12796,#12797,#12798,#12799,#12800,#12801,
#12802),.UNSPECIFIED.,.F.,.F.,(4,3,3,3,3,3,3,3,3,4),(101.656427420383,102.410609889122,
103.164792357862,103.918974826602,104.673157295342,105.427339764081,106.181522232821,
106.935704701561,107.689887170301,107.939612727562),.UNSPECIFIED.);
#253=B_SPLINE_CURVE_WITH_KNOTS('',3,(#12807,#12808,#12809,#12810,#12811,
#12812,#12813,#12814,#12815,#12816,#12817,#12818,#12819,#12820,#12821,#12822,
#12823,#12824,#12825,#12826,#12827,#12828,#12829,#12830,#12831,#12832,#12833,
#12834),.UNSPECIFIED.,.F.,.F.,(4,3,3,3,3,3,3,3,3,4),(-117.190265949363,
-116.436083480624,-115.681901011884,-114.927718543144,-114.173536074404,
-113.419353605665,-112.665171136925,-111.910988668185,-111.156806199445,
-110.907080642184),.UNSPECIFIED.);
#254=B_SPLINE_CURVE_WITH_KNOTS('',3,(#12835,#12836,#12837,#12838,#12839,
#12840,#12841,#12842,#12843,#12844,#12845,#12846,#12847,#12848,#12849,#12850,
#12851,#12852,#12853,#12854,#12855,#12856,#12857,#12858,#12859,#12860,#12861,
#12862),.UNSPECIFIED.,.F.,.F.,(4,3,3,3,3,3,3,3,3,4),(107.939612727562,108.693795196302,
109.447977665042,110.202160133782,110.956342602521,111.710525071261,112.464707540001,
113.21889000874,113.97307247748,114.222798034742),.UNSPECIFIED.);
#255=B_SPLINE_CURVE_WITH_KNOTS('',3,(#12867,#12868,#12869,#12870,#12871,
#12872,#12873,#12874,#12875,#12876,#12877,#12878,#12879,#12880,#12881,#12882,
#12883,#12884,#12885,#12886,#12887,#12888,#12889,#12890,#12891,#12892,#12893,
#12894),.UNSPECIFIED.,.F.,.F.,(4,3,3,3,3,3,3,3,3,4),(-123.473451256543,
-122.719268787803,-121.965086319063,-121.210903850324,-120.456721381584,
-119.702538912844,-118.948356444104,-118.194173975365,-117.439991506625,
-117.190265949363),.UNSPECIFIED.);
#256=B_SPLINE_CURVE_WITH_KNOTS('',3,(#12895,#12896,#12897,#12898,#12899,
#12900,#12901,#12902,#12903,#12904,#12905,#12906,#12907,#12908,#12909,#12910,
#12911,#12912,#12913,#12914,#12915,#12916,#12917,#12918,#12919,#12920,#12921,
#12922),.UNSPECIFIED.,.F.,.F.,(4,3,3,3,3,3,3,3,3,4),(114.222798034742,114.976980503482,
115.731162972221,116.485345440961,117.239527909701,117.993710378441,118.74789284718,
119.50207531592,120.25625778466,120.505983341922),.UNSPECIFIED.);
#257=B_SPLINE_CURVE_WITH_KNOTS('',3,(#12927,#12928,#12929,#12930,#12931,
#12932,#12933,#12934,#12935,#12936,#12937,#12938,#12939,#12940,#12941,#12942,
#12943,#12944,#12945,#12946,#12947,#12948,#12949,#12950,#12951,#12952,#12953,
#12954),.UNSPECIFIED.,.F.,.F.,(4,3,3,3,3,3,3,3,3,4),(-129.756636563722,
-129.002454094983,-128.248271626243,-127.494089157503,-126.739906688764,
-125.985724220024,-125.231541751284,-124.477359282544,-123.723176813805,
-123.473451256543),.UNSPECIFIED.);
#258=B_SPLINE_CURVE_WITH_KNOTS('',3,(#12955,#12956,#12957,#12958,#12959,
#12960,#12961,#12962,#12963,#12964,#12965,#12966,#12967,#12968,#12969,#12970,
#12971,#12972,#12973,#12974,#12975,#12976,#12977,#12978,#12979,#12980,#12981,
#12982),.UNSPECIFIED.,.F.,.F.,(4,3,3,3,3,3,3,3,3,4),(120.505983341922,121.260165810661,
122.014348279401,122.768530748141,123.52271321688,124.27689568562,125.03107815436,
125.7852606231,126.539443091839,126.789168649101),.UNSPECIFIED.);
#259=B_SPLINE_CURVE_WITH_KNOTS('',3,(#12987,#12988,#12989,#12990,#12991,
#12992,#12993,#12994,#12995,#12996,#12997,#12998,#12999,#13000,#13001,#13002,
#13003,#13004,#13005,#13006,#13007,#13008,#13009,#13010,#13011,#13012,#13013,
#13014),.UNSPECIFIED.,.F.,.F.,(4,3,3,3,3,3,3,3,3,4),(-136.039821870902,
-135.285639402162,-134.531456933423,-133.777274464683,-133.023091995943,
-132.268909527203,-131.514727058464,-130.760544589724,-130.006362120984,
-129.756636563722),.UNSPECIFIED.);
#260=B_SPLINE_CURVE_WITH_KNOTS('',3,(#13015,#13016,#13017,#13018,#13019,
#13020,#13021,#13022,#13023,#13024,#13025,#13026,#13027,#13028,#13029,#13030,
#13031,#13032,#13033,#13034,#13035,#13036,#13037,#13038,#13039,#13040,#13041,
#13042),.UNSPECIFIED.,.F.,.F.,(4,3,3,3,3,3,3,3,3,4),(126.789168649101,127.543351117841,
128.297533586581,129.05171605532,129.80589852406,130.5600809928,131.31426346154,
132.068445930279,132.822628399019,133.072353956281),.UNSPECIFIED.);
#261=B_SPLINE_CURVE_WITH_KNOTS('',3,(#13047,#13048,#13049,#13050,#13051,
#13052,#13053,#13054,#13055,#13056,#13057,#13058,#13059,#13060,#13061,#13062,
#13063,#13064,#13065,#13066,#13067,#13068,#13069,#13070,#13071),
 .UNSPECIFIED.,.F.,.F.,(4,3,3,3,3,3,3,3,4),(-142.323007178082,-141.927256524223,
-140.927768802221,-139.928281080219,-138.928793358218,-137.929305636216,
-136.929817914215,-136.430074053214,-136.039821870902),.UNSPECIFIED.);
#262=B_SPLINE_CURVE_WITH_KNOTS('',3,(#13072,#13073,#13074,#13075,#13076,
#13077,#13078,#13079,#13080,#13081,#13082,#13083,#13084,#13085,#13086,#13087,
#13088,#13089,#13090,#13091,#13092,#13093,#13094,#13095,#13096),
 .UNSPECIFIED.,.F.,.F.,(4,3,3,3,3,3,3,3,4),(133.072353956281,133.93135474821,
134.930842470212,135.930330192213,136.430074053214,136.929817914215,137.929305636216,
138.928793358218,139.35553926346),.UNSPECIFIED.);
#263=B_SPLINE_CURVE_WITH_KNOTS('',3,(#13101,#13102,#13103,#13104,#13105,
#13106,#13107,#13108,#13109,#13110,#13111,#13112,#13113,#13114,#13115,#13116,
#13117,#13118,#13119,#13120,#13121,#13122,#13123,#13124,#13125,#13126,#13127,
#13128),.UNSPECIFIED.,.F.,.F.,(4,3,3,3,3,3,3,3,3,4),(-148.606192485261,
-147.852010016521,-147.097827547782,-146.343645079042,-145.589462610302,
-144.835280141562,-144.081097672823,-143.326915204083,-142.572732735343,
-142.323007178082),.UNSPECIFIED.);
#264=B_SPLINE_CURVE_WITH_KNOTS('',3,(#13129,#13130,#13131,#13132,#13133,
#13134,#13135,#13136,#13137,#13138,#13139,#13140,#13141,#13142,#13143,#13144,
#13145,#13146,#13147,#13148,#13149,#13150,#13151,#13152,#13153,#13154,#13155,
#13156),.UNSPECIFIED.,.F.,.F.,(4,3,3,3,3,3,3,3,3,4),(139.35553926346,140.1097217322,
140.86390420094,141.61808666968,142.372269138419,143.126451607159,143.880634075899,
144.634816544639,145.388999013378,145.63872457064),.UNSPECIFIED.);
#265=B_SPLINE_CURVE_WITH_KNOTS('',3,(#13161,#13162,#13163,#13164,#13165,
#13166,#13167,#13168,#13169,#13170,#13171,#13172,#13173,#13174,#13175,#13176,
#13177,#13178,#13179,#13180,#13181,#13182,#13183,#13184,#13185,#13186,#13187,
#13188),.UNSPECIFIED.,.F.,.F.,(4,3,3,3,3,3,3,3,3,4),(-154.889377792441,
-154.135195323701,-153.381012854961,-152.626830386222,-151.872647917482,
-151.118465448742,-150.364282980002,-149.610100511263,-148.855918042523,
-148.606192485261),.UNSPECIFIED.);
#266=B_SPLINE_CURVE_WITH_KNOTS('',3,(#13189,#13190,#13191,#13192,#13193,
#13194,#13195,#13196,#13197,#13198,#13199,#13200,#13201,#13202,#13203,#13204,
#13205,#13206,#13207,#13208,#13209,#13210,#13211,#13212,#13213,#13214,#13215,
#13216),.UNSPECIFIED.,.F.,.F.,(4,3,3,3,3,3,3,3,3,4),(145.63872457064,146.39290703938,
147.147089508119,147.901271976859,148.655454445599,149.409636914339,150.163819383078,
150.918001851818,151.672184320558,151.921909877819),.UNSPECIFIED.);
#267=B_SPLINE_CURVE_WITH_KNOTS('',3,(#13221,#13222,#13223,#13224,#13225,
#13226,#13227,#13228,#13229,#13230,#13231,#13232,#13233,#13234,#13235,#13236,
#13237,#13238,#13239,#13240,#13241,#13242,#13243,#13244,#13245,#13246,#13247,
#13248),.UNSPECIFIED.,.F.,.F.,(4,3,3,3,3,3,3,3,3,4),(-161.17256309962,-160.418380630881,
-159.664198162141,-158.910015693401,-158.155833224661,-157.401650755922,
-156.647468287182,-155.893285818442,-155.139103349702,-154.889377792441),
 .UNSPECIFIED.);
#268=B_SPLINE_CURVE_WITH_KNOTS('',3,(#13249,#13250,#13251,#13252,#13253,
#13254,#13255,#13256,#13257,#13258,#13259,#13260,#13261,#13262,#13263,#13264,
#13265,#13266,#13267,#13268,#13269,#13270,#13271,#13272,#13273,#13274,#13275,
#13276),.UNSPECIFIED.,.F.,.F.,(4,3,3,3,3,3,3,3,3,4),(151.921909877819,152.676092346559,
153.430274815299,154.184457284039,154.938639752778,155.692822221518,156.447004690258,
157.201187158998,157.955369627737,158.205095184999),.UNSPECIFIED.);
#269=B_SPLINE_CURVE_WITH_KNOTS('',3,(#13281,#13282,#13283,#13284,#13285,
#13286,#13287,#13288,#13289,#13290,#13291,#13292,#13293,#13294,#13295,#13296,
#13297,#13298,#13299,#13300,#13301,#13302,#13303,#13304,#13305),
 .UNSPECIFIED.,.F.,.F.,(4,3,3,3,3,3,3,3,4),(-167.4557484068,-166.914449574262,
-165.91496185226,-164.915474130259,-164.415730269258,-163.915986408257,
-162.916498686255,-161.917010964254,-161.17256309962),.UNSPECIFIED.);
#270=B_SPLINE_CURVE_WITH_KNOTS('',3,(#13306,#13307,#13308,#13309,#13310,
#13311,#13312,#13313,#13314,#13315,#13316,#13317,#13318,#13319,#13320,#13321,
#13322,#13323,#13324,#13325,#13326,#13327,#13328,#13329,#13330,#13331,#13332,
#13333),.UNSPECIFIED.,.F.,.F.,(4,3,3,3,3,3,3,3,3,4),(158.205095184999,158.959277653739,
159.713460122478,160.467642591218,161.221825059958,161.976007528697,162.730189997437,
163.484372466177,164.238554934916,164.488280492179),.UNSPECIFIED.);
#271=B_SPLINE_CURVE_WITH_KNOTS('',3,(#13338,#13339,#13340,#13341,#13342,
#13343,#13344,#13345,#13346,#13347,#13348,#13349,#13350,#13351,#13352,#13353,
#13354,#13355,#13356,#13357,#13358,#13359,#13360,#13361,#13362,#13363,#13364,
#13365),.UNSPECIFIED.,.F.,.F.,(4,3,3,3,3,3,3,3,3,4),(-173.738933713979,
-172.98475124524,-172.2305687765,-171.47638630776,-170.72220383902,-169.968021370281,
-169.213838901541,-168.459656432801,-167.705473964061,-167.4557484068),
 .UNSPECIFIED.);
#272=B_SPLINE_CURVE_WITH_KNOTS('',3,(#13366,#13367,#13368,#13369,#13370,
#13371,#13372,#13373,#13374,#13375,#13376,#13377,#13378,#13379,#13380,#13381,
#13382,#13383,#13384,#13385,#13386,#13387,#13388,#13389,#13390,#13391,#13392,
#13393),.UNSPECIFIED.,.F.,.F.,(4,3,3,3,3,3,3,3,3,4),(164.488280492179,165.242462960918,
165.996645429658,166.750827898398,167.505010367137,168.259192835877,169.013375304617,
169.767557773357,170.521740242096,170.771465799358),.UNSPECIFIED.);
#273=B_SPLINE_CURVE_WITH_KNOTS('',3,(#13398,#13399,#13400,#13401,#13402,
#13403,#13404,#13405,#13406,#13407,#13408,#13409,#13410,#13411,#13412,#13413,
#13414,#13415,#13416,#13417,#13418,#13419,#13420,#13421,#13422,#13423,#13424,
#13425),.UNSPECIFIED.,.F.,.F.,(4,3,3,3,3,3,3,3,3,4),(-180.022119021159,
-179.267936552419,-178.513754083679,-177.75957161494,-177.0053891462,-176.25120667746,
-175.497024208721,-174.742841739981,-173.988659271241,-173.738933713979),
 .UNSPECIFIED.);
#274=B_SPLINE_CURVE_WITH_KNOTS('',3,(#13426,#13427,#13428,#13429,#13430,
#13431,#13432,#13433,#13434,#13435,#13436,#13437,#13438,#13439,#13440,#13441,
#13442,#13443,#13444,#13445,#13446,#13447,#13448,#13449,#13450,#13451,#13452,
#13453),.UNSPECIFIED.,.F.,.F.,(4,3,3,3,3,3,3,3,3,4),(170.771465799358,171.525648268098,
172.279830736838,173.034013205577,173.788195674317,174.542378143057,175.296560611797,
176.050743080536,176.804925549276,177.054651106538),.UNSPECIFIED.);
#275=B_SPLINE_CURVE_WITH_KNOTS('',3,(#13458,#13459,#13460,#13461,#13462,
#13463,#13464,#13465,#13466,#13467,#13468,#13469,#13470,#13471,#13472,#13473,
#13474,#13475,#13476,#13477,#13478,#13479,#13480,#13481,#13482,#13483,#13484,
#13485),.UNSPECIFIED.,.F.,.F.,(4,3,3,3,3,3,3,3,3,4),(-186.305304328339,
-185.551121859599,-184.796939390859,-184.042756922119,-183.28857445338,
-182.53439198464,-181.7802095159,-181.026027047161,-180.271844578421,-180.022119021159),
 .UNSPECIFIED.);
#276=B_SPLINE_CURVE_WITH_KNOTS('',3,(#13486,#13487,#13488,#13489,#13490,
#13491,#13492,#13493,#13494,#13495,#13496,#13497,#13498,#13499,#13500,#13501,
#13502,#13503,#13504,#13505,#13506,#13507,#13508,#13509,#13510,#13511,#13512,
#13513),.UNSPECIFIED.,.F.,.F.,(4,3,3,3,3,3,3,3,3,4),(177.054651106538,177.808833575277,
178.563016044017,179.317198512757,180.071380981497,180.825563450236,181.579745918976,
182.333928387716,183.088110856456,183.337836413717),.UNSPECIFIED.);
#277=B_SPLINE_CURVE_WITH_KNOTS('',3,(#13518,#13519,#13520,#13521,#13522,
#13523,#13524,#13525,#13526,#13527,#13528,#13529,#13530,#13531,#13532,#13533,
#13534,#13535,#13536,#13537,#13538,#13539,#13540,#13541,#13542,#13543,#13544,
#13545),.UNSPECIFIED.,.F.,.F.,(4,3,3,3,3,3,3,3,3,4),(-192.588489635518,
-191.834307166778,-191.080124698039,-190.325942229299,-189.571759760559,
-188.817577291819,-188.06339482308,-187.30921235434,-186.5550298856,-186.305304328339),
 .UNSPECIFIED.);
#278=B_SPLINE_CURVE_WITH_KNOTS('',3,(#13546,#13547,#13548,#13549,#13550,
#13551,#13552,#13553,#13554,#13555,#13556,#13557,#13558,#13559,#13560,#13561,
#13562,#13563,#13564,#13565,#13566,#13567,#13568,#13569,#13570,#13571,#13572,
#13573),.UNSPECIFIED.,.F.,.F.,(4,3,3,3,3,3,3,3,3,4),(183.337836413717,184.092018882457,
184.846201351197,185.600383819936,186.354566288676,187.108748757416,187.862931226156,
188.617113694895,189.371296163635,189.621021720897),.UNSPECIFIED.);
#279=B_SPLINE_CURVE_WITH_KNOTS('',3,(#13578,#13579,#13580,#13581,#13582,
#13583,#13584,#13585,#13586,#13587,#13588,#13589,#13590,#13591,#13592,#13593,
#13594,#13595,#13596,#13597,#13598,#13599,#13600,#13601,#13602,#13603,#13604,
#13605),.UNSPECIFIED.,.F.,.F.,(4,3,3,3,3,3,3,3,3,4),(-198.871674942698,
-198.117492473958,-197.363310005218,-196.609127536478,-195.854945067739,
-195.100762598999,-194.346580130259,-193.592397661519,-192.83821519278,
-192.588489635518),.UNSPECIFIED.);
#280=B_SPLINE_CURVE_WITH_KNOTS('',3,(#13606,#13607,#13608,#13609,#13610,
#13611,#13612,#13613,#13614,#13615,#13616,#13617,#13618,#13619,#13620,#13621,
#13622,#13623,#13624,#13625,#13626,#13627,#13628,#13629,#13630,#13631,#13632,
#13633),.UNSPECIFIED.,.F.,.F.,(4,3,3,3,3,3,3,3,3,4),(189.621021720897,190.375204189637,
191.129386658376,191.883569127116,192.637751595856,193.391934064595,194.146116533335,
194.900299002075,195.654481470815,195.904207028076),.UNSPECIFIED.);
#281=B_SPLINE_CURVE_WITH_KNOTS('',3,(#13638,#13639,#13640,#13641,#13642,
#13643,#13644,#13645,#13646,#13647,#13648,#13649,#13650,#13651,#13652,#13653,
#13654,#13655,#13656,#13657,#13658,#13659,#13660,#13661,#13662,#13663,#13664,
#13665),.UNSPECIFIED.,.F.,.F.,(4,3,3,3,3,3,3,3,3,4),(-205.154860249877,
-204.400677781137,-203.646495312398,-202.892312843658,-202.138130374918,
-201.383947906178,-200.629765437439,-199.875582968699,-199.121400499959,
-198.871674942698),.UNSPECIFIED.);
#282=B_SPLINE_CURVE_WITH_KNOTS('',3,(#13666,#13667,#13668,#13669,#13670,
#13671,#13672,#13673,#13674,#13675,#13676,#13677,#13678,#13679,#13680,#13681,
#13682,#13683,#13684,#13685,#13686,#13687,#13688,#13689,#13690,#13691,#13692,
#13693),.UNSPECIFIED.,.F.,.F.,(4,3,3,3,3,3,3,3,3,4),(195.904207028076,196.658389496816,
197.412571965556,198.166754434296,198.920936903035,199.675119371775,200.429301840515,
201.183484309255,201.937666777995,202.187392335256),.UNSPECIFIED.);
#283=B_SPLINE_CURVE_WITH_KNOTS('',3,(#13698,#13699,#13700,#13701,#13702,
#13703,#13704,#13705,#13706,#13707,#13708,#13709,#13710,#13711,#13712,#13713,
#13714,#13715,#13716,#13717,#13718,#13719,#13720,#13721,#13722,#13723,#13724,
#13725),.UNSPECIFIED.,.F.,.F.,(4,3,3,3,3,3,3,3,3,4),(-211.438045557057,
-210.683863088317,-209.929680619577,-209.175498150838,-208.421315682098,
-207.667133213358,-206.912950744618,-206.158768275878,-205.404585807139,
-205.154860249877),.UNSPECIFIED.);
#284=B_SPLINE_CURVE_WITH_KNOTS('',3,(#13726,#13727,#13728,#13729,#13730,
#13731,#13732,#13733,#13734,#13735,#13736,#13737,#13738,#13739,#13740,#13741,
#13742,#13743,#13744,#13745,#13746,#13747,#13748,#13749,#13750,#13751,#13752,
#13753),.UNSPECIFIED.,.F.,.F.,(4,3,3,3,3,3,3,3,3,4),(202.187392335256,202.941574803996,
203.695757272735,204.449939741475,205.204122210215,205.958304678955,206.712487147694,
207.466669616434,208.220852085174,208.470577642436),.UNSPECIFIED.);
#285=B_SPLINE_CURVE_WITH_KNOTS('',3,(#13758,#13759,#13760,#13761,#13762,
#13763,#13764,#13765,#13766,#13767,#13768,#13769,#13770,#13771,#13772,#13773,
#13774,#13775,#13776,#13777,#13778,#13779,#13780,#13781,#13782,#13783,#13784,
#13785),.UNSPECIFIED.,.F.,.F.,(4,3,3,3,3,3,3,3,3,4),(-217.721230864236,
-216.967048395497,-216.212865926757,-215.458683458017,-214.704500989278,
-213.950318520538,-213.196136051798,-212.441953583058,-211.687771114319,
-211.438045557057),.UNSPECIFIED.);
#286=B_SPLINE_CURVE_WITH_KNOTS('',3,(#13786,#13787,#13788,#13789,#13790,
#13791,#13792,#13793,#13794,#13795,#13796,#13797,#13798,#13799,#13800,#13801,
#13802,#13803,#13804,#13805,#13806,#13807,#13808,#13809,#13810,#13811,#13812,
#13813),.UNSPECIFIED.,.F.,.F.,(4,3,3,3,3,3,3,3,3,4),(208.470577642436,209.224760111175,
209.978942579915,210.733125048655,211.487307517394,212.241489986134,212.995672454874,
213.749854923614,214.504037392353,214.753762949615),.UNSPECIFIED.);
#287=B_SPLINE_CURVE_WITH_KNOTS('',3,(#13818,#13819,#13820,#13821,#13822,
#13823,#13824,#13825,#13826,#13827,#13828,#13829,#13830,#13831,#13832,#13833,
#13834,#13835,#13836,#13837,#13838,#13839,#13840,#13841,#13842,#13843,#13844,
#13845),.UNSPECIFIED.,.F.,.F.,(4,3,3,3,3,3,3,3,3,4),(-224.004416171416,
-223.250233702676,-222.496051233936,-221.741868765197,-220.987686296457,
-220.233503827717,-219.479321358978,-218.725138890238,-217.970956421498,
-217.721230864236),.UNSPECIFIED.);
#288=B_SPLINE_CURVE_WITH_KNOTS('',3,(#13846,#13847,#13848,#13849,#13850,
#13851,#13852,#13853,#13854,#13855,#13856,#13857,#13858,#13859,#13860,#13861,
#13862,#13863,#13864,#13865,#13866,#13867,#13868,#13869,#13870,#13871,#13872,
#13873),.UNSPECIFIED.,.F.,.F.,(4,3,3,3,3,3,3,3,3,4),(214.753762949615,215.507945418355,
216.262127887095,217.016310355834,217.770492824574,218.524675293314,219.278857762054,
220.033040230793,220.787222699533,221.036948256795),.UNSPECIFIED.);
#289=B_SPLINE_CURVE_WITH_KNOTS('',3,(#13878,#13879,#13880,#13881,#13882,
#13883,#13884,#13885,#13886,#13887,#13888,#13889,#13890,#13891,#13892,#13893,
#13894,#13895,#13896,#13897,#13898,#13899,#13900,#13901,#13902),
 .UNSPECIFIED.,.F.,.F.,(4,3,3,3,3,3,3,3,4),(-230.287601478596,-229.88217606036,
-228.882688338359,-227.883200616357,-227.383456755357,-226.883712894356,
-225.884225172354,-224.884737450353,-224.004416171416),.UNSPECIFIED.);
#290=B_SPLINE_CURVE_WITH_KNOTS('',3,(#13903,#13904,#13905,#13906,#13907,
#13908,#13909,#13910,#13911,#13912,#13913,#13914,#13915,#13916,#13917,#13918,
#13919,#13920,#13921,#13922,#13923,#13924,#13925,#13926,#13927,#13928,#13929,
#13930),.UNSPECIFIED.,.F.,.F.,(4,3,3,3,3,3,3,3,3,4),(221.036948256795,221.791130725534,
222.545313194274,223.299495663014,224.053678131754,224.807860600493,225.562043069233,
226.316225537973,227.070408006713,227.320133563974),.UNSPECIFIED.);
#291=B_SPLINE_CURVE_WITH_KNOTS('',3,(#13935,#13936,#13937,#13938,#13939,
#13940,#13941,#13942,#13943,#13944,#13945,#13946,#13947,#13948,#13949,#13950,
#13951,#13952,#13953,#13954,#13955,#13956,#13957,#13958,#13959,#13960,#13961,
#13962),.UNSPECIFIED.,.F.,.F.,(4,3,3,3,3,3,3,3,3,4),(-236.570786785775,
-235.816604317035,-235.062421848296,-234.308239379556,-233.554056910816,
-232.799874442076,-232.045691973336,-231.291509504597,-230.537327035857,
-230.287601478596),.UNSPECIFIED.);
#292=B_SPLINE_CURVE_WITH_KNOTS('',3,(#13963,#13964,#13965,#13966,#13967,
#13968,#13969,#13970,#13971,#13972,#13973,#13974,#13975,#13976,#13977,#13978,
#13979,#13980,#13981,#13982,#13983,#13984,#13985,#13986,#13987,#13988,#13989,
#13990),.UNSPECIFIED.,.F.,.F.,(4,3,3,3,3,3,3,3,3,4),(227.320133563974,228.074316032714,
228.828498501454,229.582680970193,230.336863438933,231.091045907673,231.845228376413,
232.599410845153,233.353593313892,233.603318871154),.UNSPECIFIED.);
#293=B_SPLINE_CURVE_WITH_KNOTS('',3,(#13995,#13996,#13997,#13998,#13999,
#14000,#14001,#14002,#14003,#14004,#14005,#14006,#14007,#14008,#14009,#14010,
#14011,#14012,#14013,#14014,#14015,#14016,#14017,#14018,#14019,#14020,#14021,
#14022),.UNSPECIFIED.,.F.,.F.,(4,3,3,3,3,3,3,3,3,4),(-242.853972092955,
-242.099789624215,-241.345607155475,-240.591424686735,-239.837242217996,
-239.083059749256,-238.328877280516,-237.574694811776,-236.820512343037,
-236.570786785775),.UNSPECIFIED.);
#294=B_SPLINE_CURVE_WITH_KNOTS('',3,(#14023,#14024,#14025,#14026,#14027,
#14028,#14029,#14030,#14031,#14032,#14033,#14034,#14035,#14036,#14037,#14038,
#14039,#14040,#14041,#14042,#14043,#14044,#14045,#14046,#14047,#14048,#14049,
#14050),.UNSPECIFIED.,.F.,.F.,(4,3,3,3,3,3,3,3,3,4),(233.603318871154,234.357501339894,
235.111683808633,235.865866277373,236.620048746113,237.374231214852,238.128413683592,
238.882596152332,239.636778621072,239.886504178333),.UNSPECIFIED.);
#295=B_SPLINE_CURVE_WITH_KNOTS('',3,(#14055,#14056,#14057,#14058,#14059,
#14060,#14061,#14062,#14063,#14064,#14065,#14066,#14067,#14068,#14069,#14070,
#14071,#14072,#14073,#14074,#14075,#14076,#14077,#14078,#14079,#14080,#14081,
#14082),.UNSPECIFIED.,.F.,.F.,(4,3,3,3,3,3,3,3,3,4),(-249.137157400134,
-248.382974931394,-247.628792462655,-246.874609993915,-246.120427525175,
-245.366245056435,-244.612062587695,-243.857880118956,-243.103697650216,
-242.853972092955),.UNSPECIFIED.);
#296=B_SPLINE_CURVE_WITH_KNOTS('',3,(#14083,#14084,#14085,#14086,#14087,
#14088,#14089,#14090,#14091,#14092,#14093,#14094,#14095,#14096,#14097,#14098,
#14099,#14100,#14101,#14102,#14103,#14104,#14105,#14106,#14107,#14108,#14109,
#14110),.UNSPECIFIED.,.F.,.F.,(4,3,3,3,3,3,3,3,3,4),(239.886504178333,240.640686647073,
241.394869115813,242.149051584552,242.903234053292,243.657416522032,244.411598990772,
245.165781459511,245.919963928251,246.169689485513),.UNSPECIFIED.);
#297=B_SPLINE_CURVE_WITH_KNOTS('',3,(#14115,#14116,#14117,#14118,#14119,
#14120,#14121,#14122,#14123,#14124,#14125,#14126,#14127,#14128,#14129,#14130,
#14131,#14132,#14133,#14134,#14135,#14136,#14137,#14138,#14139,#14140,#14141,
#14142),.UNSPECIFIED.,.F.,.F.,(4,3,3,3,3,3,3,3,3,4),(-255.420342707314,
-254.666160238574,-253.911977769834,-253.157795301094,-252.403612832355,
-251.649430363615,-250.895247894875,-250.141065426135,-249.386882957396,
-249.137157400134),.UNSPECIFIED.);
#298=B_SPLINE_CURVE_WITH_KNOTS('',3,(#14143,#14144,#14145,#14146,#14147,
#14148,#14149,#14150,#14151,#14152,#14153,#14154,#14155,#14156,#14157,#14158,
#14159,#14160,#14161,#14162,#14163,#14164,#14165,#14166,#14167,#14168,#14169,
#14170),.UNSPECIFIED.,.F.,.F.,(4,3,3,3,3,3,3,3,3,4),(246.169689485513,246.923871954253,
247.678054422992,248.432236891732,249.186419360471,249.940601829211,250.694784297951,
251.44896676669,252.20314923543,252.452874792692),.UNSPECIFIED.);
#299=B_SPLINE_CURVE_WITH_KNOTS('',3,(#14175,#14176,#14177,#14178,#14179,
#14180,#14181,#14182,#14183,#14184,#14185,#14186,#14187,#14188,#14189,#14190,
#14191,#14192,#14193,#14194,#14195,#14196,#14197,#14198,#14199,#14200,#14201,
#14202),.UNSPECIFIED.,.F.,.F.,(4,3,3,3,3,3,3,3,3,4),(-261.703528014493,
-260.949345545754,-260.195163077014,-259.440980608274,-258.686798139535,
-257.932615670795,-257.178433202055,-256.424250733315,-255.670068264576,
-255.420342707314),.UNSPECIFIED.);
#300=B_SPLINE_CURVE_WITH_KNOTS('',3,(#14203,#14204,#14205,#14206,#14207,
#14208,#14209,#14210,#14211,#14212,#14213,#14214,#14215,#14216,#14217,#14218,
#14219,#14220,#14221,#14222,#14223,#14224,#14225,#14226,#14227),
 .UNSPECIFIED.,.F.,.F.,(4,3,3,3,3,3,3,3,4),(252.452874792692,252.870393666397,
253.869881388398,254.8693691104,255.369112971401,255.868856832401,256.868344554403,
257.867832276404,258.736060099872),.UNSPECIFIED.);
#301=B_SPLINE_CURVE_WITH_KNOTS('',3,(#14232,#14233,#14234,#14235,#14236,
#14237,#14238,#14239,#14240,#14241,#14242,#14243,#14244,#14245,#14246,#14247,
#14248,#14249,#14250,#14251,#14252,#14253,#14254,#14255,#14256,#14257,#14258,
#14259),.UNSPECIFIED.,.F.,.F.,(4,3,3,3,3,3,3,3,3,4),(-267.986713321673,
-267.232530852933,-266.478348384194,-265.724165915454,-264.969983446714,
-264.215800977974,-263.461618509235,-262.707436040495,-261.953253571755,
-261.703528014493),.UNSPECIFIED.);
#302=B_SPLINE_CURVE_WITH_KNOTS('',3,(#14260,#14261,#14262,#14263,#14264,
#14265,#14266,#14267,#14268,#14269,#14270,#14271,#14272,#14273,#14274,#14275,
#14276,#14277,#14278,#14279,#14280,#14281,#14282,#14283,#14284,#14285,#14286,
#14287),.UNSPECIFIED.,.F.,.F.,(4,3,3,3,3,3,3,3,3,4),(258.736060099872,259.490242568612,
260.244425037352,260.998607506091,261.752789974831,262.506972443571,263.261154912311,
264.01533738105,264.76951984979,265.019245407052),.UNSPECIFIED.);
#303=B_SPLINE_CURVE_WITH_KNOTS('',3,(#14292,#14293,#14294,#14295,#14296,
#14297,#14298,#14299,#14300,#14301,#14302,#14303,#14304,#14305,#14306,#14307,
#14308,#14309,#14310,#14311,#14312,#14313,#14314,#14315,#14316,#14317,#14318,
#14319),.UNSPECIFIED.,.F.,.F.,(4,3,3,3,3,3,3,3,3,4),(-274.269898628852,
-273.515716160113,-272.761533691373,-272.007351222633,-271.253168753893,
-270.498986285153,-269.744803816413,-268.990621347674,-268.236438878934,
-267.986713321673),.UNSPECIFIED.);
#304=B_SPLINE_CURVE_WITH_KNOTS('',3,(#14320,#14321,#14322,#14323,#14324,
#14325,#14326,#14327,#14328,#14329,#14330,#14331,#14332,#14333,#14334,#14335,
#14336,#14337,#14338,#14339,#14340,#14341,#14342,#14343,#14344,#14345,#14346,
#14347),.UNSPECIFIED.,.F.,.F.,(4,3,3,3,3,3,3,3,3,4),(265.019245407052,265.773427875791,
266.527610344531,267.281792813271,268.03597528201,268.79015775075,269.54434021949,
270.29852268823,271.052705156969,271.302430714231),.UNSPECIFIED.);
#305=B_SPLINE_CURVE_WITH_KNOTS('',3,(#14352,#14353,#14354,#14355,#14356,
#14357,#14358,#14359,#14360,#14361,#14362,#14363,#14364,#14365,#14366,#14367,
#14368,#14369,#14370,#14371,#14372,#14373,#14374,#14375,#14376,#14377,#14378,
#14379),.UNSPECIFIED.,.F.,.F.,(4,3,3,3,3,3,3,3,3,4),(-280.553083936032,
-279.798901467292,-279.044718998553,-278.290536529813,-277.536354061073,
-276.782171592333,-276.027989123593,-275.273806654854,-274.519624186114,
-274.269898628852),.UNSPECIFIED.);
#306=B_SPLINE_CURVE_WITH_KNOTS('',3,(#14380,#14381,#14382,#14383,#14384,
#14385,#14386,#14387,#14388,#14389,#14390,#14391,#14392,#14393,#14394,#14395,
#14396,#14397,#14398,#14399,#14400,#14401,#14402,#14403,#14404,#14405,#14406,
#14407),.UNSPECIFIED.,.F.,.F.,(4,3,3,3,3,3,3,3,3,4),(271.302430714231,272.056613182971,
272.810795651711,273.56497812045,274.31916058919,275.07334305793,275.82752552667,
276.58170799541,277.335890464149,277.585616021411),.UNSPECIFIED.);
#307=B_SPLINE_CURVE_WITH_KNOTS('',3,(#14412,#14413,#14414,#14415,#14416,
#14417,#14418,#14419,#14420,#14421,#14422,#14423,#14424,#14425,#14426,#14427,
#14428,#14429,#14430,#14431,#14432,#14433,#14434,#14435,#14436,#14437,#14438,
#14439),.UNSPECIFIED.,.F.,.F.,(4,3,3,3,3,3,3,3,3,4),(-286.836269243212,
-286.082086774472,-285.327904305732,-284.573721836992,-283.819539368252,
-283.065356899512,-282.311174430773,-281.556991962033,-280.802809493293,
-280.553083936032),.UNSPECIFIED.);
#308=B_SPLINE_CURVE_WITH_KNOTS('',3,(#14440,#14441,#14442,#14443,#14444,
#14445,#14446,#14447,#14448,#14449,#14450,#14451,#14452,#14453,#14454,#14455,
#14456,#14457,#14458,#14459,#14460,#14461,#14462,#14463,#14464,#14465,#14466,
#14467),.UNSPECIFIED.,.F.,.F.,(4,3,3,3,3,3,3,3,3,4),(277.585616021411,278.33979849015,
279.09398095889,279.84816342763,280.60234589637,281.356528365109,282.110710833849,
282.864893302589,283.619075771328,283.86880132859),.UNSPECIFIED.);
#309=B_SPLINE_CURVE_WITH_KNOTS('',3,(#14472,#14473,#14474,#14475,#14476,
#14477,#14478,#14479,#14480,#14481,#14482,#14483,#14484,#14485,#14486,#14487,
#14488,#14489,#14490,#14491,#14492,#14493,#14494,#14495,#14496,#14497,#14498,
#14499),.UNSPECIFIED.,.F.,.F.,(4,3,3,3,3,3,3,3,3,4),(-293.119454550391,
-292.365272081651,-291.611089612912,-290.856907144172,-290.102724675432,
-289.348542206692,-288.594359737953,-287.840177269213,-287.085994800473,
-286.836269243212),.UNSPECIFIED.);
#310=B_SPLINE_CURVE_WITH_KNOTS('',3,(#14500,#14501,#14502,#14503,#14504,
#14505,#14506,#14507,#14508,#14509,#14510,#14511,#14512,#14513,#14514,#14515,
#14516,#14517,#14518,#14519,#14520,#14521,#14522,#14523,#14524,#14525,#14526,
#14527),.UNSPECIFIED.,.F.,.F.,(4,3,3,3,3,3,3,3,3,4),(283.86880132859,284.62298379733,
285.37716626607,286.131348734809,286.885531203549,287.639713672289,288.393896141029,
289.148078609768,289.902261078508,290.15198663577),.UNSPECIFIED.);
#311=B_SPLINE_CURVE_WITH_KNOTS('',3,(#14532,#14533,#14534,#14535,#14536,
#14537,#14538,#14539,#14540,#14541,#14542,#14543,#14544,#14545,#14546,#14547,
#14548,#14549,#14550,#14551,#14552,#14553,#14554,#14555,#14556,#14557,#14558,
#14559),.UNSPECIFIED.,.F.,.F.,(4,3,3,3,3,3,3,3,3,4),(-299.402639857571,
-298.648457388831,-297.894274920091,-297.140092451352,-296.385909982612,
-295.631727513872,-294.877545045133,-294.123362576393,-293.369180107653,
-293.119454550391),.UNSPECIFIED.);
#312=B_SPLINE_CURVE_WITH_KNOTS('',3,(#14560,#14561,#14562,#14563,#14564,
#14565,#14566,#14567,#14568,#14569,#14570,#14571,#14572,#14573,#14574,#14575,
#14576,#14577,#14578,#14579,#14580,#14581,#14582,#14583,#14584,#14585,#14586,
#14587),.UNSPECIFIED.,.F.,.F.,(4,3,3,3,3,3,3,3,3,4),(290.15198663577,290.90616910451,
291.660351573249,292.414534041989,293.168716510729,293.922898979468,294.677081448208,
295.431263916948,296.185446385687,296.435171942949),.UNSPECIFIED.);
#313=B_SPLINE_CURVE_WITH_KNOTS('',3,(#14592,#14593,#14594,#14595,#14596,
#14597,#14598,#14599,#14600,#14601,#14602,#14603,#14604,#14605,#14606,#14607,
#14608,#14609,#14610,#14611,#14612,#14613,#14614,#14615,#14616),
 .UNSPECIFIED.,.F.,.F.,(4,3,3,3,3,3,3,3,4),(-305.68582516475,-304.843755210478,
-303.844267488476,-302.844779766475,-302.345035905474,-301.845292044473,
-300.845804322472,-299.84631660047,-299.402639857571),.UNSPECIFIED.);
#314=B_SPLINE_CURVE_WITH_KNOTS('',3,(#14617,#14618,#14619,#14620,#14621,
#14622,#14623,#14624,#14625,#14626,#14627,#14628,#14629,#14630,#14631,#14632,
#14633,#14634,#14635,#14636,#14637,#14638,#14639,#14640,#14641,#14642,#14643,
#14644),.UNSPECIFIED.,.F.,.F.,(4,3,3,3,3,3,3,3,3,4),(296.435171942949,297.189354411689,
297.943536880429,298.697719349169,299.451901817908,300.206084286648,300.960266755388,
301.714449224128,302.468631692868,302.718357250129),.UNSPECIFIED.);
#315=B_SPLINE_CURVE_WITH_KNOTS('',3,(#14649,#14650,#14651,#14652,#14653,
#14654,#14655,#14656,#14657,#14658,#14659,#14660,#14661,#14662,#14663,#14664,
#14665,#14666,#14667,#14668,#14669,#14670,#14671,#14672,#14673,#14674,#14675,
#14676),.UNSPECIFIED.,.F.,.F.,(4,3,3,3,3,3,3,3,3,4),(-311.96901047193,-311.21482800319,
-310.46064553445,-309.706463065711,-308.952280596971,-308.198098128231,
-307.443915659491,-306.689733190751,-305.935550722012,-305.68582516475),
 .UNSPECIFIED.);
#316=B_SPLINE_CURVE_WITH_KNOTS('',3,(#14677,#14678,#14679,#14680,#14681,
#14682,#14683,#14684,#14685,#14686,#14687,#14688,#14689,#14690,#14691,#14692,
#14693,#14694,#14695,#14696,#14697,#14698,#14699,#14700,#14701,#14702,#14703,
#14704),.UNSPECIFIED.,.F.,.F.,(4,3,3,3,3,3,3,3,3,4),(302.718357250129,303.472539718869,
304.226722187608,304.980904656348,305.735087125088,306.489269593828,307.243452062567,
307.997634531307,308.751817000047,309.001542557308),.UNSPECIFIED.);
#317=B_SPLINE_CURVE_WITH_KNOTS('',3,(#14709,#14710,#14711,#14712,#14713,
#14714,#14715,#14716,#14717,#14718,#14719,#14720,#14721,#14722,#14723,#14724,
#14725,#14726,#14727,#14728,#14729,#14730,#14731,#14732,#14733,#14734,#14735,
#14736),.UNSPECIFIED.,.F.,.F.,(4,3,3,3,3,3,3,3,3,4),(-318.25219577911,-317.49801331037,
-316.74383084163,-315.98964837289,-315.23546590415,-314.481283435411,-313.727100966671,
-312.972918497931,-312.218736029191,-311.96901047193),.UNSPECIFIED.);
#318=B_SPLINE_CURVE_WITH_KNOTS('',3,(#14737,#14738,#14739,#14740,#14741,
#14742,#14743,#14744,#14745,#14746,#14747,#14748,#14749,#14750,#14751,#14752,
#14753,#14754,#14755,#14756,#14757,#14758,#14759,#14760,#14761,#14762,#14763,
#14764),.UNSPECIFIED.,.F.,.F.,(4,3,3,3,3,3,3,3,3,4),(309.001542557308,309.755725026048,
310.509907494788,311.264089963528,312.018272432267,312.772454901007,313.526637369747,
314.280819838486,315.035002307226,315.284727864488),.UNSPECIFIED.);
#319=B_SPLINE_CURVE_WITH_KNOTS('',3,(#14769,#14770,#14771,#14772,#14773,
#14774,#14775,#14776,#14777,#14778,#14779,#14780,#14781,#14782,#14783,#14784,
#14785,#14786,#14787,#14788,#14789,#14790,#14791,#14792,#14793,#14794,#14795,
#14796),.UNSPECIFIED.,.F.,.F.,(4,3,3,3,3,3,3,3,3,4),(-324.535381086289,
-323.781198617549,-323.027016148809,-322.27283368007,-321.51865121133,-320.76446874259,
-320.01028627385,-319.256103805111,-318.501921336371,-318.25219577911),
 .UNSPECIFIED.);
#320=B_SPLINE_CURVE_WITH_KNOTS('',3,(#14797,#14798,#14799,#14800,#14801,
#14802,#14803,#14804,#14805,#14806,#14807,#14808,#14809,#14810,#14811,#14812,
#14813,#14814,#14815,#14816,#14817,#14818,#14819,#14820,#14821,#14822,#14823,
#14824),.UNSPECIFIED.,.F.,.F.,(4,3,3,3,3,3,3,3,3,4),(315.284727864488,316.038910333228,
316.793092801967,317.547275270707,318.301457739447,319.055640208187,319.809822676926,
320.564005145666,321.318187614406,321.567913171668),.UNSPECIFIED.);
#321=B_SPLINE_CURVE_WITH_KNOTS('',3,(#14829,#14830,#14831,#14832,#14833,
#14834,#14835,#14836,#14837,#14838,#14839,#14840,#14841,#14842,#14843,#14844,
#14845,#14846,#14847,#14848,#14849,#14850,#14851,#14852,#14853,#14854,#14855,
#14856),.UNSPECIFIED.,.F.,.F.,(4,3,3,3,3,3,3,3,3,4),(-330.818566393469,
-330.064383924729,-329.310201455989,-328.556018987249,-327.80183651851,
-327.04765404977,-326.29347158103,-325.539289112291,-324.785106643551,-324.535381086289),
 .UNSPECIFIED.);
#322=B_SPLINE_CURVE_WITH_KNOTS('',3,(#14857,#14858,#14859,#14860,#14861,
#14862,#14863,#14864,#14865,#14866,#14867,#14868,#14869,#14870,#14871,#14872,
#14873,#14874,#14875,#14876,#14877,#14878,#14879,#14880,#14881,#14882,#14883,
#14884),.UNSPECIFIED.,.F.,.F.,(4,3,3,3,3,3,3,3,3,4),(321.567913171668,322.322095640407,
323.076278109147,323.830460577887,324.584643046626,325.338825515366,326.093007984106,
326.847190452846,327.601372921585,327.851098478847),.UNSPECIFIED.);
#323=B_SPLINE_CURVE_WITH_KNOTS('',3,(#14889,#14890,#14891,#14892,#14893,
#14894,#14895,#14896,#14897,#14898,#14899,#14900,#14901,#14902,#14903,#14904,
#14905,#14906,#14907,#14908,#14909,#14910,#14911,#14912,#14913,#14914,#14915,
#14916),.UNSPECIFIED.,.F.,.F.,(4,3,3,3,3,3,3,3,3,4),(-337.101751700648,
-336.347569231908,-335.593386763168,-334.839204294429,-334.085021825689,
-333.330839356949,-332.576656888209,-331.822474419469,-331.06829195073,
-330.818566393469),.UNSPECIFIED.);
#324=B_SPLINE_CURVE_WITH_KNOTS('',3,(#14917,#14918,#14919,#14920,#14921,
#14922,#14923,#14924,#14925,#14926,#14927,#14928,#14929,#14930,#14931,#14932,
#14933,#14934,#14935,#14936,#14937,#14938,#14939,#14940,#14941),
 .UNSPECIFIED.,.F.,.F.,(4,3,3,3,3,3,3,3,4),(327.851098478847,328.831460538516,
329.830948260517,330.330692121518,330.830435982519,331.829923704521,332.829411426522,
333.828899148524,334.134283786027),.UNSPECIFIED.);
#325=B_SPLINE_CURVE_WITH_KNOTS('',3,(#14946,#14947,#14948,#14949,#14950,
#14951,#14952,#14953,#14954,#14955,#14956,#14957,#14958,#14959,#14960,#14961,
#14962,#14963,#14964,#14965,#14966,#14967,#14968,#14969,#14970,#14971,#14972,
#14973),.UNSPECIFIED.,.F.,.F.,(4,3,3,3,3,3,3,3,3,4),(-343.384937007828,
-342.630754539088,-341.876572070348,-341.122389601608,-340.368207132869,
-339.614024664129,-338.859842195389,-338.105659726649,-337.351477257909,
-337.101751700648),.UNSPECIFIED.);
#326=B_SPLINE_CURVE_WITH_KNOTS('',3,(#14974,#14975,#14976,#14977,#14978,
#14979,#14980,#14981,#14982,#14983,#14984,#14985,#14986,#14987,#14988,#14989,
#14990,#14991,#14992,#14993,#14994,#14995,#14996,#14997,#14998,#14999,#15000,
#15001),.UNSPECIFIED.,.F.,.F.,(4,3,3,3,3,3,3,3,3,4),(334.134283786027,334.888466254766,
335.642648723506,336.396831192246,337.151013660986,337.905196129725,338.659378598465,
339.413561067205,340.167743535944,340.417469093206),.UNSPECIFIED.);
#327=B_SPLINE_CURVE_WITH_KNOTS('',3,(#15006,#15007,#15008,#15009,#15010,
#15011,#15012,#15013,#15014,#15015,#15016,#15017,#15018,#15019,#15020,#15021,
#15022,#15023,#15024,#15025,#15026,#15027,#15028,#15029,#15030,#15031,#15032,
#15033),.UNSPECIFIED.,.F.,.F.,(4,3,3,3,3,3,3,3,3,4),(-349.668122315007,
-348.913939846268,-348.159757377528,-347.405574908788,-346.651392440048,
-345.897209971308,-345.143027502569,-344.388845033829,-343.634662565089,
-343.384937007828),.UNSPECIFIED.);
#328=B_SPLINE_CURVE_WITH_KNOTS('',3,(#15034,#15035,#15036,#15037,#15038,
#15039,#15040,#15041,#15042,#15043,#15044,#15045,#15046,#15047,#15048,#15049,
#15050,#15051,#15052,#15053,#15054,#15055,#15056,#15057,#15058,#15059,#15060,
#15061),.UNSPECIFIED.,.F.,.F.,(4,3,3,3,3,3,3,3,3,4),(340.417469093206,341.171651561946,
341.925834030686,342.680016499426,343.434198968165,344.188381436905,344.942563905645,
345.696746374385,346.450928843124,346.700654400386),.UNSPECIFIED.);
#329=B_SPLINE_CURVE_WITH_KNOTS('',3,(#15066,#15067,#15068,#15069,#15070,
#15071,#15072,#15073,#15074,#15075,#15076,#15077,#15078,#15079,#15080,#15081,
#15082,#15083,#15084,#15085,#15086,#15087,#15088,#15089,#15090,#15091,#15092,
#15093),.UNSPECIFIED.,.F.,.F.,(4,3,3,3,3,3,3,3,3,4),(-355.951307622187,
-355.197125153447,-354.442942684707,-353.688760215967,-352.934577747228,
-352.180395278488,-351.426212809748,-350.672030341008,-349.917847872269,
-349.668122315007),.UNSPECIFIED.);
#330=B_SPLINE_CURVE_WITH_KNOTS('',3,(#15094,#15095,#15096,#15097,#15098,
#15099,#15100,#15101,#15102,#15103,#15104,#15105,#15106,#15107,#15108,#15109,
#15110,#15111,#15112,#15113,#15114,#15115,#15116,#15117,#15118,#15119,#15120,
#15121),.UNSPECIFIED.,.F.,.F.,(4,3,3,3,3,3,3,3,3,4),(346.700654400386,347.454836869126,
348.209019337865,348.963201806605,349.717384275345,350.471566744084,351.225749212824,
351.979931681564,352.734114150304,352.983839707566),.UNSPECIFIED.);
#331=B_SPLINE_CURVE_WITH_KNOTS('',3,(#15126,#15127,#15128,#15129,#15130,
#15131,#15132,#15133,#15134,#15135,#15136,#15137,#15138,#15139,#15140,#15141,
#15142,#15143,#15144,#15145,#15146,#15147,#15148,#15149,#15150,#15151,#15152,
#15153),.UNSPECIFIED.,.F.,.F.,(4,3,3,3,3,3,3,3,3,4),(-362.234492929366,
-361.480310460627,-360.726127991887,-359.971945523147,-359.217763054408,
-358.463580585668,-357.709398116928,-356.955215648188,-356.201033179449,
-355.951307622187),.UNSPECIFIED.);
#332=B_SPLINE_CURVE_WITH_KNOTS('',3,(#15154,#15155,#15156,#15157,#15158,
#15159,#15160,#15161,#15162,#15163,#15164,#15165,#15166,#15167,#15168,#15169,
#15170,#15171,#15172,#15173,#15174,#15175,#15176,#15177,#15178,#15179,#15180,
#15181),.UNSPECIFIED.,.F.,.F.,(4,3,3,3,3,3,3,3,3,4),(352.983839707566,353.738022176305,
354.492204645045,355.246387113785,356.000569582525,356.754752051264,357.508934520004,
358.263116988744,359.017299457484,359.267025014745),.UNSPECIFIED.);
#333=B_SPLINE_CURVE_WITH_KNOTS('',3,(#15186,#15187,#15188,#15189,#15190,
#15191,#15192,#15193,#15194,#15195,#15196,#15197,#15198,#15199,#15200,#15201,
#15202,#15203,#15204,#15205,#15206,#15207,#15208,#15209,#15210,#15211,#15212,
#15213),.UNSPECIFIED.,.F.,.F.,(4,3,3,3,3,3,3,3,3,4),(-368.517678236546,
-367.763495767806,-367.009313299066,-366.255130830327,-365.500948361587,
-364.746765892847,-363.992583424108,-363.238400955368,-362.484218486628,
-362.234492929366),.UNSPECIFIED.);
#334=B_SPLINE_CURVE_WITH_KNOTS('',3,(#15214,#15215,#15216,#15217,#15218,
#15219,#15220,#15221,#15222,#15223,#15224,#15225,#15226,#15227,#15228,#15229,
#15230,#15231,#15232,#15233,#15234,#15235,#15236,#15237,#15238,#15239,#15240,
#15241),.UNSPECIFIED.,.F.,.F.,(4,3,3,3,3,3,3,3,3,4),(359.267025014745,360.021207483485,
360.775389952225,361.529572420964,362.283754889704,363.037937358444,363.792119827184,
364.546302295924,365.300484764664,365.550210321925),.UNSPECIFIED.);
#335=B_SPLINE_CURVE_WITH_KNOTS('',3,(#15246,#15247,#15248,#15249,#15250,
#15251,#15252,#15253,#15254,#15255,#15256,#15257,#15258,#15259,#15260,#15261,
#15262,#15263,#15264,#15265,#15266,#15267,#15268,#15269,#15270),
 .UNSPECIFIED.,.F.,.F.,(4,3,3,3,3,3,3,3,4),(-374.800863543725,-373.808408028586,
-372.808920306584,-372.309176445584,-371.809432584583,-370.809944862581,
-369.81045714058,-368.810969418578,-368.517678236546),.UNSPECIFIED.);
#336=B_SPLINE_CURVE_WITH_KNOTS('',3,(#15271,#15272,#15273,#15274,#15275,
#15276,#15277,#15278,#15279,#15280,#15281,#15282,#15283,#15284,#15285,#15286,
#15287,#15288,#15289,#15290,#15291,#15292,#15293,#15294,#15295,#15296,#15297,
#15298),.UNSPECIFIED.,.F.,.F.,(4,3,3,3,3,3,3,3,3,4),(365.550210321925,366.304392790664,
367.058575259404,367.812757728144,368.566940196884,369.321122665623,370.075305134363,
370.829487603103,371.583670071843,371.833395629104),.UNSPECIFIED.);
#337=B_SPLINE_CURVE_WITH_KNOTS('',3,(#15303,#15304,#15305,#15306,#15307,
#15308,#15309,#15310,#15311,#15312,#15313,#15314,#15315,#15316,#15317,#15318,
#15319,#15320,#15321,#15322,#15323,#15324,#15325,#15326,#15327,#15328,#15329,
#15330),.UNSPECIFIED.,.F.,.F.,(4,3,3,3,3,3,3,3,3,4),(-381.084048850905,
-380.329866382165,-379.575683913426,-378.821501444686,-378.067318975946,
-377.313136507206,-376.558954038467,-375.804771569727,-375.050589100987,
-374.800863543725),.UNSPECIFIED.);
#338=B_SPLINE_CURVE_WITH_KNOTS('',3,(#15331,#15332,#15333,#15334,#15335,
#15336,#15337,#15338,#15339,#15340,#15341,#15342,#15343,#15344,#15345,#15346,
#15347,#15348,#15349,#15350,#15351,#15352,#15353,#15354,#15355,#15356,#15357,
#15358),.UNSPECIFIED.,.F.,.F.,(4,3,3,3,3,3,3,3,3,4),(371.833395629104,372.587578097844,
373.341760566584,374.095943035323,374.850125504063,375.604307972803,376.358490441542,
377.112672910282,377.866855379022,378.116580936284),.UNSPECIFIED.);
#339=B_SPLINE_CURVE_WITH_KNOTS('',3,(#15363,#15364,#15365,#15366,#15367,
#15368,#15369,#15370,#15371,#15372,#15373,#15374,#15375,#15376,#15377,#15378,
#15379,#15380,#15381,#15382,#15383,#15384,#15385,#15386,#15387,#15388,#15389,
#15390),.UNSPECIFIED.,.F.,.F.,(4,3,3,3,3,3,3,3,3,4),(-387.367234158085,
-386.613051689345,-385.858869220605,-385.104686751865,-384.350504283126,
-383.596321814386,-382.842139345646,-382.087956876907,-381.333774408167,
-381.084048850905),.UNSPECIFIED.);
#340=B_SPLINE_CURVE_WITH_KNOTS('',3,(#15391,#15392,#15393,#15394,#15395,
#15396,#15397,#15398,#15399,#15400,#15401,#15402,#15403,#15404,#15405,#15406,
#15407,#15408,#15409,#15410,#15411,#15412,#15413,#15414,#15415,#15416,#15417,
#15418),.UNSPECIFIED.,.F.,.F.,(4,3,3,3,3,3,3,3,3,4),(378.116580936284,378.870763405023,
379.624945873763,380.379128342503,381.133310811243,381.887493279982,382.641675748722,
383.395858217462,384.150040686201,384.399766243463),.UNSPECIFIED.);
#341=B_SPLINE_CURVE_WITH_KNOTS('',3,(#15423,#15424,#15425,#15426,#15427,
#15428,#15429,#15430,#15431,#15432,#15433,#15434,#15435,#15436,#15437,#15438,
#15439,#15440,#15441,#15442,#15443,#15444,#15445,#15446,#15447,#15448,#15449,
#15450),.UNSPECIFIED.,.F.,.F.,(4,3,3,3,3,3,3,3,3,4),(-393.650419465264,
-392.896236996525,-392.142054527785,-391.387872059045,-390.633689590305,
-389.879507121566,-389.125324652826,-388.371142184086,-387.616959715347,
-387.367234158085),.UNSPECIFIED.);
#342=B_SPLINE_CURVE_WITH_KNOTS('',3,(#15451,#15452,#15453,#15454,#15455,
#15456,#15457,#15458,#15459,#15460,#15461,#15462,#15463,#15464,#15465,#15466,
#15467,#15468,#15469,#15470,#15471,#15472,#15473,#15474,#15475,#15476,#15477,
#15478),.UNSPECIFIED.,.F.,.F.,(4,3,3,3,3,3,3,3,3,4),(384.399766243463,385.153948712203,
385.908131180943,386.662313649683,387.416496118422,388.170678587162,388.924861055902,
389.679043524642,390.433225993381,390.682951550643),.UNSPECIFIED.);
#343=B_SPLINE_CURVE_WITH_KNOTS('',3,(#15483,#15484,#15485,#15486,#15487,
#15488,#15489,#15490,#15491,#15492,#15493,#15494,#15495,#15496,#15497,#15498,
#15499,#15500,#15501,#15502,#15503,#15504,#15505,#15506,#15507,#15508,#15509,
#15510),.UNSPECIFIED.,.F.,.F.,(4,3,3,3,3,3,3,3,3,4),(-399.933604772444,
-399.179422303704,-398.425239834964,-397.671057366224,-396.916874897485,
-396.162692428745,-395.408509960005,-394.654327491265,-393.900145022526,
-393.650419465264),.UNSPECIFIED.);
#344=B_SPLINE_CURVE_WITH_KNOTS('',3,(#15511,#15512,#15513,#15514,#15515,
#15516,#15517,#15518,#15519,#15520,#15521,#15522,#15523,#15524,#15525,#15526,
#15527,#15528,#15529,#15530,#15531,#15532,#15533,#15534,#15535,#15536,#15537,
#15538),.UNSPECIFIED.,.F.,.F.,(4,3,3,3,3,3,3,3,3,4),(390.682951550643,391.437134019383,
392.191316488122,392.945498956862,393.699681425602,394.453863894341,395.208046363081,
395.962228831821,396.716411300561,396.966136857822),.UNSPECIFIED.);
#345=B_SPLINE_CURVE_WITH_KNOTS('',3,(#15543,#15544,#15545,#15546,#15547,
#15548,#15549,#15550,#15551,#15552,#15553,#15554,#15555,#15556,#15557,#15558,
#15559,#15560,#15561,#15562,#15563,#15564,#15565,#15566,#15567,#15568,#15569,
#15570),.UNSPECIFIED.,.F.,.F.,(4,3,3,3,3,3,3,3,3,4),(-406.216790079623,
-405.462607610884,-404.708425142144,-403.954242673404,-403.200060204664,
-402.445877735925,-401.691695267185,-400.937512798445,-400.183330329705,
-399.933604772444),.UNSPECIFIED.);
#346=B_SPLINE_CURVE_WITH_KNOTS('',3,(#15571,#15572,#15573,#15574,#15575,
#15576,#15577,#15578,#15579,#15580,#15581,#15582,#15583,#15584,#15585,#15586,
#15587,#15588,#15589,#15590,#15591,#15592,#15593,#15594,#15595),
 .UNSPECIFIED.,.F.,.F.,(4,3,3,3,3,3,3,3,4),(396.966136857822,397.796113356624,
398.795601078626,399.795088800627,400.294832661628,400.794576522629,401.79406424463,
402.793551966632,403.249322165002),.UNSPECIFIED.);
#347=B_SPLINE_CURVE_WITH_KNOTS('',3,(#15600,#15601,#15602,#15603,#15604,
#15605,#15606,#15607,#15608,#15609,#15610,#15611,#15612,#15613,#15614,#15615,
#15616,#15617,#15618,#15619,#15620,#15621,#15622,#15623,#15624,#15625,#15626,
#15627),.UNSPECIFIED.,.F.,.F.,(4,3,3,3,3,3,3,3,3,4),(-412.499975386803,
-411.745792918063,-410.991610449323,-410.237427980584,-409.483245511844,
-408.729063043104,-407.974880574364,-407.220698105624,-406.466515636885,
-406.216790079623),.UNSPECIFIED.);
#348=B_SPLINE_CURVE_WITH_KNOTS('',3,(#15628,#15629,#15630,#15631,#15632,
#15633,#15634,#15635,#15636,#15637,#15638,#15639,#15640,#15641,#15642,#15643,
#15644,#15645,#15646,#15647,#15648,#15649,#15650,#15651,#15652,#15653,#15654,
#15655),.UNSPECIFIED.,.F.,.F.,(4,3,3,3,3,3,3,3,3,4),(403.249322165002,404.003504633742,
404.757687102482,405.511869571221,406.266052039961,407.020234508701,407.774416977441,
408.52859944618,409.28278191492,409.532507472182),.UNSPECIFIED.);
#349=B_SPLINE_CURVE_WITH_KNOTS('',3,(#15660,#15661,#15662,#15663,#15664,
#15665,#15666,#15667,#15668,#15669,#15670,#15671,#15672,#15673,#15674,#15675,
#15676,#15677,#15678,#15679,#15680,#15681,#15682,#15683,#15684,#15685,#15686,
#15687),.UNSPECIFIED.,.F.,.F.,(4,3,3,3,3,3,3,3,3,4),(-418.783160693982,
-418.028978225243,-417.274795756503,-416.520613287763,-415.766430819024,
-415.012248350284,-414.258065881544,-413.503883412804,-412.749700944065,
-412.499975386803),.UNSPECIFIED.);
#350=B_SPLINE_CURVE_WITH_KNOTS('',3,(#15688,#15689,#15690,#15691,#15692,
#15693,#15694,#15695,#15696,#15697,#15698,#15699,#15700,#15701,#15702,#15703,
#15704,#15705,#15706,#15707,#15708,#15709,#15710,#15711,#15712,#15713,#15714,
#15715),.UNSPECIFIED.,.F.,.F.,(4,3,3,3,3,3,3,3,3,4),(409.532507472182,410.286689940921,
411.040872409661,411.795054878401,412.54923734714,413.30341981588,414.05760228462,
414.81178475336,415.565967222099,415.815692779361),.UNSPECIFIED.);
#351=B_SPLINE_CURVE_WITH_KNOTS('',3,(#15720,#15721,#15722,#15723,#15724,
#15725,#15726,#15727,#15728,#15729,#15730,#15731,#15732,#15733,#15734,#15735,
#15736,#15737,#15738,#15739,#15740,#15741,#15742,#15743,#15744,#15745,#15746,
#15747),.UNSPECIFIED.,.F.,.F.,(4,3,3,3,3,3,3,3,3,4),(-425.066346001162,
-424.782281850666,-423.782794128664,-422.783306406663,-421.783818684661,
-421.28407482366,-420.78433096266,-419.784843240658,-418.785355518657,-418.783160693982),
 .UNSPECIFIED.);
#352=B_SPLINE_CURVE_WITH_KNOTS('',3,(#15748,#15749,#15750,#15751,#15752,
#15753,#15754,#15755,#15756,#15757,#15758,#15759,#15760,#15761,#15762,#15763,
#15764,#15765,#15766,#15767,#15768,#15769,#15770,#15771,#15772,#15773,#15774,
#15775),.UNSPECIFIED.,.F.,.F.,(4,3,3,3,3,3,3,3,3,4),(415.815692779361,416.569875248101,
417.324057716841,418.07824018558,418.83242265432,419.58660512306,420.340787591799,
421.094970060539,421.849152529279,422.098878086541),.UNSPECIFIED.);
#353=B_SPLINE_CURVE_WITH_KNOTS('',3,(#15780,#15781,#15782,#15783,#15784,
#15785,#15786,#15787,#15788,#15789,#15790,#15791,#15792,#15793,#15794,#15795,
#15796,#15797,#15798,#15799,#15800,#15801,#15802,#15803,#15804),
 .UNSPECIFIED.,.F.,.F.,(4,3,3,3,3,3,3,3,4),(-431.349531308342,-430.779208182675,
-429.779720460674,-428.780232738672,-428.280488877671,-427.780745016671,
-426.781257294669,-425.781769572668,-425.066346001162),.UNSPECIFIED.);
#354=B_SPLINE_CURVE_WITH_KNOTS('',3,(#15805,#15806,#15807,#15808,#15809,
#15810,#15811,#15812,#15813,#15814,#15815,#15816,#15817,#15818,#15819,#15820,
#15821,#15822,#15823,#15824,#15825,#15826,#15827,#15828,#15829,#15830,#15831,
#15832),.UNSPECIFIED.,.F.,.F.,(4,3,3,3,3,3,3,3,3,4),(422.098878086541,422.85306055528,
423.60724302402,424.36142549276,425.1156079615,425.86979043024,426.623972898979,
427.378155367719,428.132337836459,428.38206339372),.UNSPECIFIED.);
#355=B_SPLINE_CURVE_WITH_KNOTS('',3,(#15837,#15838,#15839,#15840,#15841,
#15842,#15843,#15844,#15845,#15846,#15847,#15848,#15849,#15850,#15851,#15852,
#15853,#15854,#15855,#15856,#15857,#15858,#15859,#15860,#15861,#15862,#15863,
#15864),.UNSPECIFIED.,.F.,.F.,(4,3,3,3,3,3,3,3,3,4),(-437.632716615521,
-436.878534146781,-436.124351678042,-435.370169209302,-434.615986740562,
-433.861804271822,-433.107621803083,-432.353439334343,-431.599256865603,
-431.349531308342),.UNSPECIFIED.);
#356=B_SPLINE_CURVE_WITH_KNOTS('',3,(#15865,#15866,#15867,#15868,#15869,
#15870,#15871,#15872,#15873,#15874,#15875,#15876,#15877,#15878,#15879,#15880,
#15881,#15882,#15883,#15884,#15885,#15886,#15887,#15888,#15889,#15890,#15891,
#15892),.UNSPECIFIED.,.F.,.F.,(4,3,3,3,3,3,3,3,3,4),(428.38206339372,429.13624586246,
429.8904283312,430.644610799939,431.398793268679,432.152975737419,432.907158206158,
433.661340674898,434.415523143638,434.6652487009),.UNSPECIFIED.);
#357=B_SPLINE_CURVE_WITH_KNOTS('',3,(#15897,#15898,#15899,#15900,#15901,
#15902,#15903,#15904,#15905,#15906,#15907,#15908,#15909,#15910,#15911,#15912,
#15913,#15914,#15915,#15916,#15917,#15918,#15919,#15920,#15921,#15922,#15923,
#15924),.UNSPECIFIED.,.F.,.F.,(4,3,3,3,3,3,3,3,3,4),(-443.915901922701,
-443.161719453961,-442.407536985222,-441.653354516482,-440.899172047743,
-440.144989579003,-439.390807110263,-438.636624641524,-437.882442172784,
-437.632716615521),.UNSPECIFIED.);
#358=B_SPLINE_CURVE_WITH_KNOTS('',3,(#15925,#15926,#15927,#15928,#15929,
#15930,#15931,#15932,#15933,#15934,#15935,#15936,#15937,#15938,#15939,#15940,
#15941,#15942,#15943,#15944,#15945,#15946,#15947,#15948,#15949,#15950,#15951,
#15952),.UNSPECIFIED.,.F.,.F.,(4,3,3,3,3,3,3,3,3,4),(434.6652487009,435.41943116964,
436.173613638379,436.927796107119,437.681978575859,438.436161044599,439.190343513339,
439.944525982079,440.698708450818,440.948434008079),.UNSPECIFIED.);
#359=B_SPLINE_CURVE_WITH_KNOTS('',3,(#15957,#15958,#15959,#15960,#15961,
#15962,#15963,#15964,#15965,#15966,#15967,#15968,#15969,#15970,#15971,#15972,
#15973,#15974,#15975,#15976,#15977,#15978,#15979,#15980,#15981,#15982,#15983,
#15984),.UNSPECIFIED.,.F.,.F.,(4,3,3,3,3,3,3,3,3,4),(-450.19908722988,-449.44490476114,
-448.690722292401,-447.936539823661,-447.182357354921,-446.428174886181,
-445.673992417442,-444.919809948702,-444.165627479962,-443.915901922701),
 .UNSPECIFIED.);
#360=B_SPLINE_CURVE_WITH_KNOTS('',3,(#15985,#15986,#15987,#15988,#15989,
#15990,#15991,#15992,#15993,#15994,#15995,#15996,#15997,#15998,#15999,#16000,
#16001,#16002,#16003,#16004,#16005,#16006,#16007,#16008,#16009,#16010,#16011,
#16012),.UNSPECIFIED.,.F.,.F.,(4,3,3,3,3,3,3,3,3,4),(440.948434008079,441.702616476819,
442.456798945559,443.210981414299,443.965163883038,444.719346351778,445.473528820518,
446.227711289257,446.981893757997,447.231619315259),.UNSPECIFIED.);
#361=B_SPLINE_CURVE_WITH_KNOTS('',3,(#16017,#16018,#16019,#16020,#16021,
#16022,#16023,#16024,#16025,#16026,#16027,#16028,#16029,#16030,#16031,#16032,
#16033,#16034,#16035,#16036,#16037,#16038,#16039,#16040,#16041,#16042,#16043,
#16044),.UNSPECIFIED.,.F.,.F.,(4,3,3,3,3,3,3,3,3,4),(-456.48227253706,-455.72809006832,
-454.97390759958,-454.219725130841,-453.465542662101,-452.711360193361,
-451.957177724622,-451.202995255882,-450.448812787142,-450.19908722988),
 .UNSPECIFIED.);
#362=B_SPLINE_CURVE_WITH_KNOTS('',3,(#16045,#16046,#16047,#16048,#16049,
#16050,#16051,#16052,#16053,#16054,#16055,#16056,#16057,#16058,#16059,#16060,
#16061,#16062,#16063,#16064,#16065,#16066,#16067,#16068,#16069,#16070,#16071,
#16072),.UNSPECIFIED.,.F.,.F.,(4,3,3,3,3,3,3,3,3,4),(447.231619315259,447.985801783999,
448.739984252738,449.494166721478,450.248349190217,451.002531658957,451.756714127697,
452.510896596436,453.265079065176,453.514804622438),.UNSPECIFIED.);
#363=B_SPLINE_CURVE_WITH_KNOTS('',3,(#16077,#16078,#16079,#16080,#16081,
#16082,#16083,#16084,#16085,#16086,#16087,#16088,#16089,#16090,#16091,#16092,
#16093,#16094,#16095,#16096,#16097,#16098,#16099,#16100,#16101,#16102,#16103,
#16104),.UNSPECIFIED.,.F.,.F.,(4,3,3,3,3,3,3,3,3,4),(-462.765457844239,
-462.0112753755,-461.25709290676,-460.50291043802,-459.74872796928,-458.99454550054,
-458.240363031801,-457.486180563061,-456.731998094321,-456.48227253706),
 .UNSPECIFIED.);
#364=B_SPLINE_CURVE_WITH_KNOTS('',3,(#16105,#16106,#16107,#16108,#16109,
#16110,#16111,#16112,#16113,#16114,#16115,#16116,#16117,#16118,#16119,#16120,
#16121,#16122,#16123,#16124,#16125,#16126,#16127,#16128,#16129,#16130,#16131,
#16132),.UNSPECIFIED.,.F.,.F.,(4,3,3,3,3,3,3,3,3,4),(453.514804622438,454.268987091178,
455.023169559918,455.777352028658,456.531534497398,457.285716966138,458.039899434877,
458.794081903617,459.548264372357,459.797989929618),.UNSPECIFIED.);
#365=B_SPLINE_CURVE_WITH_KNOTS('',3,(#16137,#16138,#16139,#16140,#16141,
#16142,#16143,#16144,#16145,#16146,#16147,#16148,#16149,#16150,#16151,#16152,
#16153,#16154,#16155,#16156,#16157,#16158,#16159,#16160,#16161,#16162,#16163,
#16164),.UNSPECIFIED.,.F.,.F.,(4,3,3,3,3,3,3,3,3,4),(-469.048643151419,
-468.294460682679,-467.54027821394,-466.7860957452,-466.03191327646,-465.277730807721,
-464.523548338981,-463.769365870241,-463.015183401502,-462.765457844239),
 .UNSPECIFIED.);
#366=B_SPLINE_CURVE_WITH_KNOTS('',3,(#16165,#16166,#16167,#16168,#16169,
#16170,#16171,#16172,#16173,#16174,#16175,#16176,#16177,#16178,#16179,#16180,
#16181,#16182,#16183,#16184,#16185,#16186,#16187,#16188,#16189,#16190,#16191,
#16192),.UNSPECIFIED.,.F.,.F.,(4,3,3,3,3,3,3,3,3,4),(459.797989929618,460.552172398358,
461.306354867097,462.060537335837,462.814719804577,463.568902273316,464.323084742056,
465.077267210796,465.831449679535,466.081175236798),.UNSPECIFIED.);
#367=B_SPLINE_CURVE_WITH_KNOTS('',3,(#16197,#16198,#16199,#16200,#16201,
#16202,#16203,#16204,#16205,#16206,#16207,#16208,#16209,#16210,#16211,#16212,
#16213,#16214,#16215,#16216,#16217,#16218,#16219,#16220,#16221,#16222,#16223,
#16224),.UNSPECIFIED.,.F.,.F.,(4,3,3,3,3,3,3,3,3,4),(-475.331828458599,
-474.577645989859,-473.823463521119,-473.069281052379,-472.31509858364,
-471.5609161149,-470.80673364616,-470.052551177421,-469.298368708681,-469.048643151419),
 .UNSPECIFIED.);
#368=B_SPLINE_CURVE_WITH_KNOTS('',3,(#16225,#16226,#16227,#16228,#16229,
#16230,#16231,#16232,#16233,#16234,#16235,#16236,#16237,#16238,#16239,#16240,
#16241,#16242,#16243,#16244,#16245,#16246,#16247,#16248,#16249,#16250,#16251,
#16252),.UNSPECIFIED.,.F.,.F.,(4,3,3,3,3,3,3,3,3,4),(466.081175236798,466.835357705537,
467.589540174277,468.343722643017,469.097905111756,469.852087580496,470.606270049236,
471.360452517975,472.114634986715,472.364360543977),.UNSPECIFIED.);
#369=B_SPLINE_CURVE_WITH_KNOTS('',3,(#16257,#16258,#16259,#16260,#16261,
#16262,#16263,#16264,#16265,#16266,#16267,#16268,#16269,#16270,#16271,#16272,
#16273,#16274,#16275,#16276,#16277,#16278,#16279,#16280,#16281,#16282,#16283,
#16284),.UNSPECIFIED.,.F.,.F.,(4,3,3,3,3,3,3,3,3,4),(-481.615013765778,
-480.860831297038,-480.106648828299,-479.352466359559,-478.598283890819,
-477.844101422079,-477.08991895334,-476.3357364846,-475.58155401586,-475.331828458599),
 .UNSPECIFIED.);
#370=B_SPLINE_CURVE_WITH_KNOTS('',3,(#16285,#16286,#16287,#16288,#16289,
#16290,#16291,#16292,#16293,#16294,#16295,#16296,#16297,#16298,#16299,#16300,
#16301,#16302,#16303,#16304,#16305,#16306,#16307,#16308,#16309,#16310,#16311,
#16312),.UNSPECIFIED.,.F.,.F.,(4,3,3,3,3,3,3,3,3,4),(472.364360543977,473.118543012717,
473.872725481457,474.626907950196,475.381090418936,476.135272887676,476.889455356416,
477.643637825155,478.397820293895,478.647545851157),.UNSPECIFIED.);
#371=B_SPLINE_CURVE_WITH_KNOTS('',3,(#16317,#16318,#16319,#16320,#16321,
#16322,#16323,#16324,#16325,#16326,#16327,#16328,#16329,#16330,#16331,#16332,
#16333,#16334,#16335,#16336,#16337,#16338,#16339,#16340,#16341,#16342,#16343,
#16344),.UNSPECIFIED.,.F.,.F.,(4,3,3,3,3,3,3,3,3,4),(-487.898199072958,
-487.144016604218,-486.389834135478,-485.635651666738,-484.881469197999,
-484.127286729259,-483.373104260519,-482.618921791779,-481.86473932304,
-481.615013765778),.UNSPECIFIED.);
#372=B_SPLINE_CURVE_WITH_KNOTS('',3,(#16345,#16346,#16347,#16348,#16349,
#16350,#16351,#16352,#16353,#16354,#16355,#16356,#16357,#16358,#16359,#16360,
#16361,#16362,#16363,#16364,#16365,#16366,#16367,#16368,#16369,#16370,#16371,
#16372),.UNSPECIFIED.,.F.,.F.,(4,3,3,3,3,3,3,3,3,4),(478.647545851157,479.401728319896,
480.155910788636,480.910093257376,481.664275726116,482.418458194855,483.172640663595,
483.926823132335,484.681005601074,484.930731158336),.UNSPECIFIED.);
#373=B_SPLINE_CURVE_WITH_KNOTS('',3,(#16377,#16378,#16379,#16380,#16381,
#16382,#16383,#16384,#16385,#16386,#16387,#16388,#16389,#16390,#16391,#16392,
#16393,#16394,#16395,#16396,#16397,#16398,#16399,#16400,#16401),
 .UNSPECIFIED.,.F.,.F.,(4,3,3,3,3,3,3,3,4),(-494.181384380137,-493.746934668774,
-492.747446946773,-491.747959224771,-491.24821536377,-490.748471502769,
-489.748983780768,-488.749496058766,-487.898199072958),.UNSPECIFIED.);
#374=B_SPLINE_CURVE_WITH_KNOTS('',3,(#16402,#16403,#16404,#16405,#16406,
#16407,#16408,#16409,#16410,#16411,#16412,#16413,#16414,#16415,#16416,#16417,
#16418,#16419,#16420,#16421,#16422,#16423,#16424,#16425,#16426,#16427,#16428,
#16429),.UNSPECIFIED.,.F.,.F.,(4,3,3,3,3,3,3,3,3,4),(484.930731158336,485.684913627076,
486.439096095816,487.193278564555,487.947461033295,488.701643502035,489.455825970775,
490.210008439514,490.964190908254,491.213916465516),.UNSPECIFIED.);
#375=B_SPLINE_CURVE_WITH_KNOTS('',3,(#16434,#16435,#16436,#16437,#16438,
#16439,#16440,#16441,#16442,#16443,#16444,#16445,#16446,#16447,#16448,#16449,
#16450,#16451,#16452,#16453,#16454,#16455,#16456,#16457,#16458,#16459,#16460,
#16461),.UNSPECIFIED.,.F.,.F.,(4,3,3,3,3,3,3,3,3,4),(-500.464569687317,
-499.710387218577,-498.956204749837,-498.202022281097,-497.447839812357,
-496.693657343618,-495.939474874878,-495.185292406138,-494.431109937398,
-494.181384380137),.UNSPECIFIED.);
#376=B_SPLINE_CURVE_WITH_KNOTS('',3,(#16462,#16463,#16464,#16465,#16466,
#16467,#16468,#16469,#16470,#16471,#16472,#16473,#16474,#16475,#16476,#16477,
#16478,#16479,#16480,#16481,#16482,#16483,#16484,#16485,#16486,#16487,#16488,
#16489),.UNSPECIFIED.,.F.,.F.,(4,3,3,3,3,3,3,3,3,4),(491.213916465516,491.968098934256,
492.722281402995,493.476463871735,494.230646340475,494.984828809214,495.739011277954,
496.493193746694,497.247376215433,497.497101772695),.UNSPECIFIED.);
#377=B_SPLINE_CURVE_WITH_KNOTS('',3,(#16494,#16495,#16496,#16497,#16498,
#16499,#16500,#16501,#16502,#16503,#16504,#16505,#16506,#16507,#16508,#16509,
#16510,#16511,#16512,#16513,#16514,#16515,#16516,#16517,#16518,#16519,#16520,
#16521),.UNSPECIFIED.,.F.,.F.,(4,3,3,3,3,3,3,3,3,4),(-506.747754994496,
-505.993572525757,-505.239390057017,-504.485207588277,-503.731025119538,
-502.976842650798,-502.222660182058,-501.468477713319,-500.714295244579,
-500.464569687317),.UNSPECIFIED.);
#378=B_SPLINE_CURVE_WITH_KNOTS('',3,(#16522,#16523,#16524,#16525,#16526,
#16527,#16528,#16529,#16530,#16531,#16532,#16533,#16534,#16535,#16536,#16537,
#16538,#16539,#16540,#16541,#16542,#16543,#16544,#16545,#16546,#16547,#16548,
#16549),.UNSPECIFIED.,.F.,.F.,(4,3,3,3,3,3,3,3,3,4),(497.497101772695,498.251284241435,
499.005466710175,499.759649178915,500.513831647655,501.268014116394,502.022196585134,
502.776379053874,503.530561522614,503.780287079875),.UNSPECIFIED.);
#379=B_SPLINE_CURVE_WITH_KNOTS('',3,(#16554,#16555,#16556,#16557,#16558,
#16559,#16560,#16561,#16562,#16563,#16564,#16565,#16566,#16567,#16568,#16569,
#16570,#16571,#16572,#16573,#16574,#16575,#16576,#16577,#16578,#16579,#16580,
#16581),.UNSPECIFIED.,.F.,.F.,(4,3,3,3,3,3,3,3,3,4),(-513.030940301676,
-512.276757832936,-511.522575364197,-510.768392895457,-510.014210426717,
-509.260027957977,-508.505845489238,-507.751663020498,-506.997480551758,
-506.747754994496),.UNSPECIFIED.);
#380=B_SPLINE_CURVE_WITH_KNOTS('',3,(#16582,#16583,#16584,#16585,#16586,
#16587,#16588,#16589,#16590,#16591,#16592,#16593,#16594,#16595,#16596,#16597,
#16598,#16599,#16600,#16601,#16602,#16603,#16604,#16605,#16606,#16607,#16608,
#16609),.UNSPECIFIED.,.F.,.F.,(4,3,3,3,3,3,3,3,3,4),(503.780287079875,504.534469548615,
505.288652017355,506.042834486094,506.797016954834,507.551199423574,508.305381892314,
509.059564361054,509.813746829794,510.063472387055),.UNSPECIFIED.);
#381=B_SPLINE_CURVE_WITH_KNOTS('',3,(#16614,#16615,#16616,#16617,#16618,
#16619,#16620,#16621,#16622,#16623,#16624,#16625,#16626,#16627,#16628,#16629,
#16630,#16631,#16632,#16633,#16634,#16635,#16636,#16637,#16638,#16639,#16640,
#16641),.UNSPECIFIED.,.F.,.F.,(4,3,3,3,3,3,3,3,3,4),(-519.314125608855,
-518.559943140116,-517.805760671376,-517.051578202637,-516.297395733897,
-515.543213265157,-514.789030796418,-514.034848327678,-513.280665858939,
-513.030940301676),.UNSPECIFIED.);
#382=B_SPLINE_CURVE_WITH_KNOTS('',3,(#16642,#16643,#16644,#16645,#16646,
#16647,#16648,#16649,#16650,#16651,#16652,#16653,#16654,#16655,#16656,#16657,
#16658,#16659,#16660,#16661,#16662,#16663,#16664,#16665,#16666,#16667,#16668,
#16669),.UNSPECIFIED.,.F.,.F.,(4,3,3,3,3,3,3,3,3,4),(510.063472387055,510.817654855794,
511.571837324534,512.326019793273,513.080202262013,513.834384730752,514.588567199492,
515.342749668232,516.096932136971,516.346657694234),.UNSPECIFIED.);
#383=B_SPLINE_CURVE_WITH_KNOTS('',3,(#16674,#16675,#16676,#16677,#16678,
#16679,#16680,#16681,#16682,#16683,#16684,#16685,#16686,#16687,#16688,#16689,
#16690,#16691,#16692,#16693,#16694,#16695,#16696,#16697,#16698,#16699,#16700,
#16701),.UNSPECIFIED.,.F.,.F.,(4,3,3,3,3,3,3,3,3,4),(-525.597310916035,
-524.843128447295,-524.088945978556,-523.334763509816,-522.580581041076,
-521.826398572337,-521.072216103597,-520.318033634857,-519.563851166117,
-519.314125608855),.UNSPECIFIED.);
#384=B_SPLINE_CURVE_WITH_KNOTS('',3,(#16702,#16703,#16704,#16705,#16706,
#16707,#16708,#16709,#16710,#16711,#16712,#16713,#16714,#16715,#16716,#16717,
#16718,#16719,#16720,#16721,#16722,#16723,#16724,#16725,#16726),
 .UNSPECIFIED.,.F.,.F.,(4,3,3,3,3,3,3,3,4),(516.346657694234,516.735152274811,
517.734639996812,518.734127718814,519.233871579814,519.733615440815,520.733103162817,
521.732590884818,522.629843001414),.UNSPECIFIED.);
#385=B_SPLINE_CURVE_WITH_KNOTS('',3,(#16731,#16732,#16733,#16734,#16735,
#16736,#16737,#16738,#16739,#16740,#16741,#16742,#16743,#16744,#16745,#16746,
#16747,#16748,#16749,#16750,#16751,#16752,#16753,#16754,#16755,#16756,#16757,
#16758),.UNSPECIFIED.,.F.,.F.,(4,3,3,3,3,3,3,3,3,4),(-531.880496223215,
-531.126313754475,-530.372131285735,-529.617948816995,-528.863766348255,
-528.109583879515,-527.355401410776,-526.601218942036,-525.847036473296,
-525.597310916035),.UNSPECIFIED.);
#386=B_SPLINE_CURVE_WITH_KNOTS('',3,(#16759,#16760,#16761,#16762,#16763,
#16764,#16765,#16766,#16767,#16768,#16769,#16770,#16771,#16772,#16773,#16774,
#16775,#16776,#16777,#16778,#16779,#16780,#16781,#16782,#16783,#16784,#16785,
#16786),.UNSPECIFIED.,.F.,.F.,(4,3,3,3,3,3,3,3,3,4),(522.629843001414,523.384025470153,
524.138207938893,524.892390407633,525.646572876373,526.400755345113,527.154937813853,
527.909120282592,528.663302751332,528.913028308593),.UNSPECIFIED.);
#387=B_SPLINE_CURVE_WITH_KNOTS('',3,(#16791,#16792,#16793,#16794,#16795,
#16796,#16797,#16798,#16799,#16800,#16801,#16802,#16803,#16804,#16805,#16806,
#16807,#16808,#16809,#16810,#16811,#16812,#16813,#16814,#16815,#16816,#16817,
#16818),.UNSPECIFIED.,.F.,.F.,(4,3,3,3,3,3,3,3,3,4),(-538.163681530394,
-537.409499061655,-536.655316592915,-535.901134124175,-535.146951655435,
-534.392769186696,-533.638586717956,-532.884404249216,-532.130221780477,
-531.880496223215),.UNSPECIFIED.);
#388=B_SPLINE_CURVE_WITH_KNOTS('',3,(#16819,#16820,#16821,#16822,#16823,
#16824,#16825,#16826,#16827,#16828,#16829,#16830,#16831,#16832,#16833,#16834,
#16835,#16836,#16837,#16838,#16839,#16840,#16841,#16842,#16843,#16844,#16845,
#16846),.UNSPECIFIED.,.F.,.F.,(4,3,3,3,3,3,3,3,3,4),(528.913028308593,529.667210777333,
530.421393246073,531.175575714812,531.929758183552,532.683940652292,533.438123121032,
534.192305589771,534.946488058511,535.196213615773),.UNSPECIFIED.);
#389=B_SPLINE_CURVE_WITH_KNOTS('',3,(#16851,#16852,#16853,#16854,#16855,
#16856,#16857,#16858,#16859,#16860,#16861,#16862,#16863,#16864,#16865,#16866,
#16867,#16868,#16869,#16870,#16871,#16872,#16873,#16874,#16875,#16876,#16877,
#16878),.UNSPECIFIED.,.F.,.F.,(4,3,3,3,3,3,3,3,3,4),(-544.446866837574,
-543.692684368834,-542.938501900094,-542.184319431355,-541.430136962615,
-540.675954493875,-539.921772025136,-539.167589556396,-538.413407087656,
-538.163681530394),.UNSPECIFIED.);
#390=B_SPLINE_CURVE_WITH_KNOTS('',3,(#16879,#16880,#16881,#16882,#16883,
#16884,#16885,#16886,#16887,#16888,#16889,#16890,#16891,#16892,#16893,#16894,
#16895,#16896,#16897,#16898,#16899,#16900,#16901,#16902,#16903,#16904,#16905,
#16906),.UNSPECIFIED.,.F.,.F.,(4,3,3,3,3,3,3,3,3,4),(535.196213615773,535.950396084513,
536.704578553252,537.458761021992,538.212943490732,538.967125959471,539.721308428211,
540.475490896951,541.229673365691,541.479398922952),.UNSPECIFIED.);
#391=B_SPLINE_CURVE_WITH_KNOTS('',3,(#16911,#16912,#16913,#16914,#16915,
#16916,#16917,#16918,#16919,#16920,#16921,#16922,#16923,#16924,#16925,#16926,
#16927,#16928,#16929,#16930,#16931,#16932,#16933,#16934,#16935,#16936,#16937,
#16938),.UNSPECIFIED.,.F.,.F.,(4,3,3,3,3,3,3,3,3,4),(-550.730052144753,
-549.975869676014,-549.221687207274,-548.467504738534,-547.713322269795,
-546.959139801055,-546.204957332315,-545.450774863575,-544.696592394836,
-544.446866837574),.UNSPECIFIED.);
#392=B_SPLINE_CURVE_WITH_KNOTS('',3,(#16939,#16940,#16941,#16942,#16943,
#16944,#16945,#16946,#16947,#16948,#16949,#16950,#16951,#16952,#16953,#16954,
#16955,#16956,#16957,#16958,#16959,#16960,#16961,#16962,#16963,#16964,#16965,
#16966),.UNSPECIFIED.,.F.,.F.,(4,3,3,3,3,3,3,3,3,4),(541.479398922952,542.233581391692,
542.987763860432,543.741946329171,544.496128797911,545.250311266651,546.004493735391,
546.75867620413,547.51285867287,547.762584230132),.UNSPECIFIED.);
#393=B_SPLINE_CURVE_WITH_KNOTS('',3,(#16971,#16972,#16973,#16974,#16975,
#16976,#16977,#16978,#16979,#16980,#16981,#16982,#16983,#16984,#16985,#16986,
#16987,#16988,#16989,#16990,#16991,#16992,#16993,#16994,#16995,#16996,#16997,
#16998),.UNSPECIFIED.,.F.,.F.,(4,3,3,3,3,3,3,3,3,4),(-557.013237451933,
-556.259054983193,-555.504872514453,-554.750690045713,-553.996507576973,
-553.242325108234,-552.488142639494,-551.733960170754,-550.979777702014,
-550.730052144753),.UNSPECIFIED.);
#394=B_SPLINE_CURVE_WITH_KNOTS('',3,(#16999,#17000,#17001,#17002,#17003,
#17004,#17005,#17006,#17007,#17008,#17009,#17010,#17011,#17012,#17013,#17014,
#17015,#17016,#17017,#17018,#17019,#17020,#17021,#17022,#17023,#17024,#17025,
#17026),.UNSPECIFIED.,.F.,.F.,(4,3,3,3,3,3,3,3,3,4),(547.762584230132,548.516766698872,
549.270949167611,550.025131636351,550.779314105091,551.533496573831,552.28767904257,
553.04186151131,553.79604398005,554.045769537312),.UNSPECIFIED.);
#395=B_SPLINE_CURVE_WITH_KNOTS('',3,(#17031,#17032,#17033,#17034,#17035,
#17036,#17037,#17038,#17039,#17040,#17041,#17042,#17043,#17044,#17045,#17046,
#17047,#17048,#17049,#17050,#17051,#17052,#17053,#17054,#17055,#17056,#17057,
#17058),.UNSPECIFIED.,.F.,.F.,(4,3,3,3,3,3,3,3,3,4),(-563.296422759112,
-562.542240290373,-561.788057821633,-561.033875352894,-560.279692884154,
-559.525510415414,-558.771327946675,-558.017145477935,-557.262963009196,
-557.013237451933),.UNSPECIFIED.);
#396=B_SPLINE_CURVE_WITH_KNOTS('',3,(#17059,#17060,#17061,#17062,#17063,
#17064,#17065,#17066,#17067,#17068,#17069,#17070,#17071,#17072,#17073,#17074,
#17075,#17076,#17077,#17078,#17079,#17080,#17081,#17082,#17083,#17084,#17085,
#17086),.UNSPECIFIED.,.F.,.F.,(4,3,3,3,3,3,3,3,3,4),(554.045769537312,554.799952006051,
555.554134474791,556.308316943531,557.062499412271,557.816681881011,558.570864349751,
559.32504681849,560.07922928723,560.328954844491),.UNSPECIFIED.);
#397=B_SPLINE_CURVE_WITH_KNOTS('',3,(#17091,#17092,#17093,#17094,#17095,
#17096,#17097,#17098,#17099,#17100,#17101,#17102,#17103,#17104,#17105,#17106,
#17107,#17108,#17109,#17110,#17111,#17112,#17113,#17114,#17115,#17116,#17117,
#17118),.UNSPECIFIED.,.F.,.F.,(4,3,3,3,3,3,3,3,3,4),(-569.579608066292,
-568.825425597552,-568.071243128813,-567.317060660073,-566.562878191334,
-565.808695722594,-565.054513253854,-564.300330785115,-563.546148316375,
-563.296422759112),.UNSPECIFIED.);
#398=B_SPLINE_CURVE_WITH_KNOTS('',3,(#17119,#17120,#17121,#17122,#17123,
#17124,#17125,#17126,#17127,#17128,#17129,#17130,#17131,#17132,#17133,#17134,
#17135,#17136,#17137,#17138,#17139,#17140,#17141,#17142,#17143,#17144,#17145,
#17146),.UNSPECIFIED.,.F.,.F.,(4,3,3,3,3,3,3,3,3,4),(560.328954844491,561.083137313231,
561.837319781971,562.59150225071,563.34568471945,564.09986718819,564.854049656929,
565.608232125669,566.362414594409,566.612140151671),.UNSPECIFIED.);
#399=B_SPLINE_CURVE_WITH_KNOTS('',3,(#17151,#17152,#17153,#17154,#17155,
#17156,#17157,#17158,#17159,#17160,#17161,#17162,#17163,#17164,#17165,#17166,
#17167,#17168,#17169,#17170,#17171,#17172,#17173,#17174,#17175,#17176,#17177,
#17178),.UNSPECIFIED.,.F.,.F.,(4,3,3,3,3,3,3,3,3,4),(-575.862793373472,
-575.108610904732,-574.354428435992,-573.600245967253,-572.846063498513,
-572.091881029774,-571.337698561034,-570.583516092294,-569.829333623555,
-569.579608066292),.UNSPECIFIED.);
#400=B_SPLINE_CURVE_WITH_KNOTS('',3,(#17179,#17180,#17181,#17182,#17183,
#17184,#17185,#17186,#17187,#17188,#17189,#17190,#17191,#17192,#17193,#17194,
#17195,#17196,#17197,#17198,#17199,#17200,#17201,#17202,#17203,#17204,#17205,
#17206),.UNSPECIFIED.,.F.,.F.,(4,3,3,3,3,3,3,3,3,4),(566.612140151671,567.36632262041,
568.12050508915,568.87468755789,569.62887002663,570.383052495369,571.137234964109,
571.891417432849,572.645599901588,572.89532545885),.UNSPECIFIED.);
#401=B_SPLINE_CURVE_WITH_KNOTS('',3,(#17211,#17212,#17213,#17214,#17215,
#17216,#17217,#17218,#17219,#17220,#17221,#17222,#17223,#17224,#17225,#17226,
#17227,#17228,#17229,#17230,#17231,#17232,#17233,#17234,#17235,#17236,#17237,
#17238),.UNSPECIFIED.,.F.,.F.,(4,3,3,3,3,3,3,3,3,4),(-582.145978680651,
-581.391796211912,-580.637613743172,-579.883431274432,-579.129248805693,
-578.375066336953,-577.620883868214,-576.866701399474,-576.112518930734,
-575.862793373472),.UNSPECIFIED.);
#402=B_SPLINE_CURVE_WITH_KNOTS('',3,(#17239,#17240,#17241,#17242,#17243,
#17244,#17245,#17246,#17247,#17248,#17249,#17250,#17251,#17252,#17253,#17254,
#17255,#17256,#17257,#17258,#17259,#17260,#17261,#17262,#17263,#17264,#17265,
#17266),.UNSPECIFIED.,.F.,.F.,(4,3,3,3,3,3,3,3,3,4),(572.89532545885,573.64950792759,
574.40369039633,575.157872865069,575.912055333809,576.666237802549,577.420420271289,
578.174602740028,578.928785208768,579.17851076603),.UNSPECIFIED.);
#403=B_SPLINE_CURVE_WITH_KNOTS('',3,(#17271,#17272,#17273,#17274,#17275,
#17276,#17277,#17278,#17279,#17280,#17281,#17282,#17283,#17284,#17285,#17286,
#17287,#17288,#17289,#17290,#17291,#17292,#17293,#17294,#17295,#17296,#17297,
#17298),.UNSPECIFIED.,.F.,.F.,(4,3,3,3,3,3,3,3,3,4),(-588.429163987831,
-587.674981519091,-586.920799050352,-586.166616581612,-585.412434112872,
-584.658251644133,-583.904069175393,-583.149886706654,-582.395704237914,
-582.145978680651),.UNSPECIFIED.);
#404=B_SPLINE_CURVE_WITH_KNOTS('',3,(#17299,#17300,#17301,#17302,#17303,
#17304,#17305,#17306,#17307,#17308,#17309,#17310,#17311,#17312,#17313,#17314,
#17315,#17316,#17317,#17318,#17319,#17320,#17321,#17322,#17323),
 .UNSPECIFIED.,.F.,.F.,(4,3,3,3,3,3,3,3,4),(579.17851076603,579.702878760909,
580.702366482911,581.701854204912,582.201598065913,582.701341926914,583.700829648916,
584.700317370917,585.461696073209),.UNSPECIFIED.);
#405=B_SPLINE_CURVE_WITH_KNOTS('',3,(#17329,#17330,#17331,#17332,#17333,
#17334,#17335,#17336,#17337,#17338),.UNSPECIFIED.,.F.,.F.,(4,3,3,4),(600.04419683565,
600.828396999699,601.612597163748,602.234451722701),.UNSPECIFIED.);
#406=B_SPLINE_CURVE_WITH_KNOTS('',3,(#17341,#17342,#17343,#17344,#17345),
 .UNSPECIFIED.,.F.,.F.,(4,1,4),(600.04419683565,600.495790741192,600.995534602193),
 .UNSPECIFIED.);
#407=B_SPLINE_CURVE_WITH_KNOTS('',3,(#17350,#17351,#17352,#17353,#17354,
#17355,#17356,#17357,#17358,#17359,#17360,#17361,#17362,#17363,#17364,#17365,
#17366,#17367,#17368,#17369,#17370,#17371,#17372,#17373,#17374,#17375,#17376,
#17377),.UNSPECIFIED.,.F.,.F.,(4,3,3,3,3,3,3,3,3,4),(593.761011528471,594.54521169252,
595.329411856569,596.113612020618,596.897812184667,597.682012348716,598.466212512766,
599.250412676815,600.034612840864,600.04419683565),.UNSPECIFIED.);
#408=B_SPLINE_CURVE_WITH_KNOTS('',3,(#17378,#17379,#17380,#17381,#17382,
#17383,#17384,#17385,#17386,#17387,#17388,#17389,#17390,#17391,#17392,#17393,
#17394,#17395,#17396,#17397,#17398,#17399,#17400,#17401,#17402,#17403,#17404,
#17405),.UNSPECIFIED.,.F.,.F.,(4,3,3,3,3,3,3,3,3,4),(593.761011528471,594.54521169252,
595.329411856569,596.113612020618,596.897812184667,597.682012348717,598.466212512766,
599.250412676815,600.034612840864,600.04419683565),.UNSPECIFIED.);
#409=B_SPLINE_CURVE_WITH_KNOTS('',3,(#17410,#17411,#17412,#17413,#17414,
#17415,#17416,#17417,#17418,#17419,#17420,#17421,#17422,#17423,#17424,#17425,
#17426,#17427,#17428,#17429,#17430,#17431,#17432,#17433,#17434,#17435,#17436,
#17437),.UNSPECIFIED.,.F.,.F.,(4,3,3,3,3,3,3,3,3,4),(587.477826221291,588.26202638534,
589.046226549389,589.830426713438,590.614626877487,591.398827041536,592.183027205585,
592.967227369634,593.751427533683,593.761011528471),.UNSPECIFIED.);
#410=B_SPLINE_CURVE_WITH_KNOTS('',3,(#17438,#17439,#17440,#17441,#17442,
#17443,#17444,#17445,#17446,#17447,#17448,#17449,#17450,#17451,#17452,#17453,
#17454,#17455,#17456,#17457,#17458,#17459,#17460,#17461,#17462),
 .UNSPECIFIED.,.F.,.F.,(4,3,3,3,3,3,3,3,4),(587.477826221291,588.002194216173,
589.001681938174,590.001169660176,590.500913521176,591.000657382177,592.000145104179,
592.99963282618,593.761011528471),.UNSPECIFIED.);
#411=B_SPLINE_CURVE_WITH_KNOTS('',3,(#17467,#17468,#17469,#17470,#17471,
#17472,#17473,#17474,#17475,#17476,#17477,#17478,#17479,#17480,#17481,#17482,
#17483,#17484,#17485,#17486,#17487,#17488,#17489,#17490,#17491,#17492,#17493,
#17494),.UNSPECIFIED.,.F.,.F.,(4,3,3,3,3,3,3,3,3,4),(581.194640914112,581.978841078161,
582.76304124221,583.54724140626,584.331441570309,585.115641734358,585.899841898408,
586.684042062457,587.468242226507,587.477826221291),.UNSPECIFIED.);
#412=B_SPLINE_CURVE_WITH_KNOTS('',3,(#17495,#17496,#17497,#17498,#17499,
#17500,#17501,#17502,#17503,#17504,#17505,#17506,#17507,#17508,#17509,#17510,
#17511,#17512,#17513,#17514,#17515,#17516,#17517,#17518,#17519,#17520,#17521,
#17522),.UNSPECIFIED.,.F.,.F.,(4,3,3,3,3,3,3,3,3,4),(581.194640914112,581.978841078161,
582.763041242211,583.54724140626,584.331441570309,585.115641734359,585.899841898408,
586.684042062457,587.468242226507,587.477826221291),.UNSPECIFIED.);
#413=B_SPLINE_CURVE_WITH_KNOTS('',3,(#17527,#17528,#17529,#17530,#17531,
#17532,#17533,#17534,#17535,#17536,#17537,#17538,#17539,#17540,#17541,#17542,
#17543,#17544,#17545,#17546,#17547,#17548,#17549,#17550,#17551,#17552,#17553,
#17554),.UNSPECIFIED.,.F.,.F.,(4,3,3,3,3,3,3,3,3,4),(574.911455606932,575.695655770981,
576.47985593503,577.264056099079,578.048256263128,578.832456427178,579.616656591227,
580.400856755276,581.185056919325,581.194640914112),.UNSPECIFIED.);
#414=B_SPLINE_CURVE_WITH_KNOTS('',3,(#17555,#17556,#17557,#17558,#17559,
#17560,#17561,#17562,#17563,#17564,#17565,#17566,#17567,#17568,#17569,#17570,
#17571,#17572,#17573,#17574,#17575,#17576,#17577,#17578,#17579,#17580,#17581,
#17582),.UNSPECIFIED.,.F.,.F.,(4,3,3,3,3,3,3,3,3,4),(574.911455606932,575.695655770981,
576.479855935031,577.26405609908,578.048256263129,578.832456427178,579.616656591227,
580.400856755276,581.185056919325,581.194640914112),.UNSPECIFIED.);
#415=B_SPLINE_CURVE_WITH_KNOTS('',3,(#17587,#17588,#17589,#17590,#17591,
#17592,#17593,#17594,#17595,#17596,#17597,#17598,#17599,#17600,#17601,#17602,
#17603,#17604,#17605,#17606,#17607,#17608,#17609,#17610,#17611,#17612,#17613,
#17614),.UNSPECIFIED.,.F.,.F.,(4,3,3,3,3,3,3,3,3,4),(568.628270299752,569.412470463802,
570.196670627851,570.9808707919,571.765070955949,572.549271119999,573.333471284048,
574.117671448097,574.901871612146,574.911455606932),.UNSPECIFIED.);
#416=B_SPLINE_CURVE_WITH_KNOTS('',3,(#17615,#17616,#17617,#17618,#17619,
#17620,#17621,#17622,#17623,#17624,#17625),.UNSPECIFIED.,.F.,.F.,(4,1,1,
1,1,1,1,1,4),(568.628270299753,569.011927498143,569.511671359144,570.011415220144,
571.010902942146,572.010390664148,573.009878386149,574.009366108151,574.911455606932),
 .UNSPECIFIED.);
#417=B_SPLINE_CURVE_WITH_KNOTS('',3,(#17630,#17631,#17632,#17633,#17634,
#17635,#17636,#17637,#17638,#17639,#17640),.UNSPECIFIED.,.F.,.F.,(4,1,1,
1,1,1,1,1,4),(562.345084992573,563.332255392685,564.331743114686,565.331230836688,
565.830974697689,566.33071855869,567.330206280691,568.329694002693,568.628270299752),
 .UNSPECIFIED.);
#418=B_SPLINE_CURVE_WITH_KNOTS('',3,(#17641,#17642,#17643,#17644,#17645,
#17646,#17647,#17648,#17649,#17650,#17651,#17652,#17653,#17654,#17655,#17656,
#17657,#17658,#17659,#17660,#17661,#17662,#17663,#17664,#17665,#17666,#17667,
#17668),.UNSPECIFIED.,.F.,.F.,(4,3,3,3,3,3,3,3,3,4),(562.345084992573,563.129285156622,
563.913485320671,564.69768548472,565.48188564877,566.266085812819,567.050285976868,
567.834486140917,568.618686304966,568.628270299753),.UNSPECIFIED.);
#419=B_SPLINE_CURVE_WITH_KNOTS('',3,(#17673,#17674,#17675,#17676,#17677,
#17678,#17679,#17680,#17681,#17682,#17683,#17684,#17685,#17686,#17687,#17688,
#17689,#17690,#17691,#17692,#17693,#17694,#17695,#17696,#17697,#17698,#17699,
#17700),.UNSPECIFIED.,.F.,.F.,(4,3,3,3,3,3,3,3,3,4),(556.061899685393,556.846099849442,
557.630300013492,558.414500177541,559.19870034159,559.982900505639,560.767100669689,
561.551300833738,562.335500997787,562.345084992573),.UNSPECIFIED.);
#420=B_SPLINE_CURVE_WITH_KNOTS('',3,(#17701,#17702,#17703,#17704,#17705,
#17706,#17707,#17708,#17709,#17710),.UNSPECIFIED.,.F.,.F.,(4,1,1,1,1,1,
1,4),(556.061899685393,557.018074834124,558.017562556126,559.017050278127,
560.016538000129,561.01602572213,562.015513444132,562.345084992573),
 .UNSPECIFIED.);
#421=B_SPLINE_CURVE_WITH_KNOTS('',3,(#17715,#17716,#17717,#17718,#17719,
#17720,#17721,#17722,#17723,#17724,#17725,#17726,#17727,#17728,#17729,#17730,
#17731,#17732,#17733,#17734,#17735,#17736,#17737,#17738,#17739,#17740,#17741,
#17742),.UNSPECIFIED.,.F.,.F.,(4,3,3,3,3,3,3,3,3,4),(549.778714378214,550.562914542263,
551.347114706312,552.131314870362,552.915515034411,553.699715198461,554.48391536251,
555.268115526559,556.052315690609,556.061899685393),.UNSPECIFIED.);
#422=B_SPLINE_CURVE_WITH_KNOTS('',3,(#17743,#17744,#17745,#17746,#17747,
#17748,#17749,#17750,#17751,#17752,#17753,#17754,#17755,#17756,#17757,#17758,
#17759,#17760,#17761,#17762,#17763,#17764,#17765,#17766,#17767,#17768,#17769,
#17770),.UNSPECIFIED.,.F.,.F.,(4,3,3,3,3,3,3,3,3,4),(549.778714378214,550.562914542263,
551.347114706312,552.131314870362,552.915515034411,553.69971519846,554.483915362509,
555.268115526559,556.052315690608,556.061899685393),.UNSPECIFIED.);
#423=B_SPLINE_CURVE_WITH_KNOTS('',3,(#17775,#17776,#17777,#17778,#17779,
#17780,#17781,#17782,#17783,#17784,#17785,#17786,#17787,#17788,#17789,#17790,
#17791,#17792,#17793,#17794,#17795,#17796,#17797,#17798,#17799,#17800,#17801,
#17802),.UNSPECIFIED.,.F.,.F.,(4,3,3,3,3,3,3,3,3,4),(543.495529071034,544.279729235084,
545.063929399133,545.848129563182,546.632329727232,547.416529891281,548.20073005533,
548.98493021938,549.769130383429,549.778714378214),.UNSPECIFIED.);
#424=B_SPLINE_CURVE_WITH_KNOTS('',3,(#17803,#17804,#17805,#17806,#17807,
#17808,#17809,#17810,#17811,#17812,#17813,#17814,#17815,#17816,#17817,#17818,
#17819,#17820,#17821,#17822,#17823,#17824,#17825,#17826,#17827,#17828,#17829,
#17830),.UNSPECIFIED.,.F.,.F.,(4,3,3,3,3,3,3,3,3,4),(543.495529071034,544.279729235084,
545.063929399133,545.848129563183,546.632329727232,547.416529891281,548.200730055331,
548.98493021938,549.769130383429,549.778714378214),.UNSPECIFIED.);
#425=B_SPLINE_CURVE_WITH_KNOTS('',3,(#17835,#17836,#17837,#17838,#17839,
#17840,#17841,#17842,#17843,#17844,#17845,#17846,#17847,#17848,#17849,#17850,
#17851,#17852,#17853,#17854,#17855,#17856,#17857,#17858,#17859,#17860,#17861,
#17862),.UNSPECIFIED.,.F.,.F.,(4,3,3,3,3,3,3,3,3,4),(537.212343763855,537.996543927904,
538.780744091952,539.564944256001,540.34914442005,541.133344584099,541.917544748148,
542.701744912197,543.485945076246,543.495529071034),.UNSPECIFIED.);
#426=B_SPLINE_CURVE_WITH_KNOTS('',3,(#17863,#17864,#17865,#17866,#17867,
#17868,#17869,#17870,#17871,#17872,#17873,#17874,#17875,#17876,#17877,#17878,
#17879,#17880,#17881,#17882,#17883,#17884,#17885,#17886,#17887,#17888,#17889,
#17890),.UNSPECIFIED.,.F.,.F.,(4,3,3,3,3,3,3,3,3,4),(537.212343763855,537.996543927904,
538.780744091953,539.564944256002,540.349144420051,541.1333445841,541.917544748149,
542.701744912198,543.485945076247,543.495529071034),.UNSPECIFIED.);
#427=B_SPLINE_CURVE_WITH_KNOTS('',3,(#17895,#17896,#17897,#17898,#17899,
#17900,#17901,#17902,#17903,#17904,#17905,#17906,#17907,#17908,#17909,#17910,
#17911,#17912,#17913,#17914,#17915,#17916,#17917,#17918,#17919,#17920,#17921,
#17922),.UNSPECIFIED.,.F.,.F.,(4,3,3,3,3,3,3,3,3,4),(530.929158456675,531.713358620724,
532.497558784773,533.281758948822,534.065959112871,534.85015927692,535.634359440969,
536.418559605018,537.202759769067,537.212343763855),.UNSPECIFIED.);
#428=B_SPLINE_CURVE_WITH_KNOTS('',3,(#17923,#17924,#17925,#17926,#17927,
#17928,#17929,#17930,#17931,#17932,#17933,#17934,#17935,#17936,#17937,#17938,
#17939,#17940,#17941,#17942,#17943,#17944,#17945,#17946,#17947,#17948,#17949,
#17950),.UNSPECIFIED.,.F.,.F.,(4,3,3,3,3,3,3,3,3,4),(530.929158456675,531.713358620725,
532.497558784774,533.281758948823,534.065959112872,534.850159276922,535.634359440971,
536.41855960502,537.202759769069,537.212343763855),.UNSPECIFIED.);
#429=B_SPLINE_CURVE_WITH_KNOTS('',3,(#17955,#17956,#17957,#17958,#17959,
#17960,#17961,#17962,#17963,#17964,#17965,#17966,#17967,#17968,#17969,#17970,
#17971,#17972,#17973,#17974,#17975,#17976,#17977,#17978,#17979,#17980,#17981,
#17982),.UNSPECIFIED.,.F.,.F.,(4,3,3,3,3,3,3,3,3,4),(524.645973149495,525.430173313545,
526.214373477594,526.998573641643,527.782773805692,528.566973969742,529.351174133791,
530.13537429784,530.91957446189,530.929158456675),.UNSPECIFIED.);
#430=B_SPLINE_CURVE_WITH_KNOTS('',3,(#17983,#17984,#17985,#17986,#17987,
#17988,#17989,#17990,#17991,#17992,#17993),.UNSPECIFIED.,.F.,.F.,(4,1,1,
1,1,1,1,1,4),(524.645973149496,525.034467730074,526.033955452075,527.033443174077,
527.533187035078,528.032930896078,529.03241861808,530.031906340082,530.929158456675),
 .UNSPECIFIED.);
#431=B_SPLINE_CURVE_WITH_KNOTS('',3,(#17998,#17999,#18000,#18001,#18002,
#18003,#18004,#18005,#18006,#18007,#18008,#18009,#18010,#18011,#18012,#18013,
#18014,#18015,#18016,#18017,#18018,#18019,#18020,#18021,#18022,#18023,#18024,
#18025),.UNSPECIFIED.,.F.,.F.,(4,3,3,3,3,3,3,3,3,4),(518.362787842316,519.146988006365,
519.931188170414,520.715388334463,521.499588498512,522.283788662561,523.06798882661,
523.852188990659,524.636389154708,524.645973149495),.UNSPECIFIED.);
#432=B_SPLINE_CURVE_WITH_KNOTS('',3,(#18026,#18027,#18028,#18029,#18030,
#18031,#18032,#18033,#18034,#18035,#18036,#18037,#18038,#18039,#18040,#18041,
#18042,#18043,#18044,#18045,#18046,#18047,#18048,#18049,#18050,#18051,#18052,
#18053),.UNSPECIFIED.,.F.,.F.,(4,3,3,3,3,3,3,3,3,4),(518.362787842316,519.146988006365,
519.931188170415,520.715388334464,521.499588498513,522.283788662562,523.067988826612,
523.852188990661,524.63638915471,524.645973149496),.UNSPECIFIED.);
#433=B_SPLINE_CURVE_WITH_KNOTS('',3,(#18058,#18059,#18060,#18061,#18062,
#18063,#18064,#18065,#18066,#18067,#18068,#18069,#18070,#18071,#18072,#18073,
#18074,#18075,#18076,#18077,#18078,#18079,#18080,#18081,#18082,#18083,#18084,
#18085),.UNSPECIFIED.,.F.,.F.,(4,3,3,3,3,3,3,3,3,4),(512.079602535136,512.863802699186,
513.648002863235,514.432203027284,515.216403191333,516.000603355383,516.784803519432,
517.569003683481,518.35320384753,518.362787842316),.UNSPECIFIED.);
#434=B_SPLINE_CURVE_WITH_KNOTS('',3,(#18086,#18087,#18088,#18089,#18090,
#18091,#18092,#18093,#18094,#18095,#18096,#18097,#18098,#18099,#18100,#18101,
#18102,#18103,#18104,#18105,#18106,#18107,#18108,#18109,#18110,#18111,#18112,
#18113),.UNSPECIFIED.,.F.,.F.,(4,3,3,3,3,3,3,3,3,4),(512.079602535137,512.863802699186,
513.648002863235,514.432203027285,515.216403191334,516.000603355383,516.784803519433,
517.569003683482,518.353203847532,518.362787842316),.UNSPECIFIED.);
#435=B_SPLINE_CURVE_WITH_KNOTS('',3,(#18118,#18119,#18120,#18121,#18122,
#18123,#18124,#18125,#18126,#18127,#18128,#18129,#18130,#18131,#18132,#18133,
#18134,#18135,#18136,#18137,#18138,#18139,#18140,#18141,#18142,#18143,#18144,
#18145),.UNSPECIFIED.,.F.,.F.,(4,3,3,3,3,3,3,3,3,4),(505.796417227957,506.580617392006,
507.364817556055,508.149017720104,508.933217884153,509.717418048202,510.501618212252,
511.285818376301,512.07001854035,512.079602535136),.UNSPECIFIED.);
#436=B_SPLINE_CURVE_WITH_KNOTS('',3,(#18146,#18147,#18148,#18149,#18150,
#18151,#18152,#18153,#18154,#18155,#18156,#18157,#18158,#18159,#18160,#18161,
#18162,#18163,#18164,#18165,#18166,#18167,#18168,#18169,#18170,#18171,#18172,
#18173),.UNSPECIFIED.,.F.,.F.,(4,3,3,3,3,3,3,3,3,4),(505.796417227957,506.580617392006,
507.364817556056,508.149017720105,508.933217884154,509.717418048203,510.501618212253,
511.285818376302,512.070018540351,512.079602535137),.UNSPECIFIED.);
#437=B_SPLINE_CURVE_WITH_KNOTS('',3,(#18178,#18179,#18180,#18181,#18182,
#18183,#18184,#18185,#18186,#18187,#18188),.UNSPECIFIED.,.F.,.F.,(4,1,1,
1,1,1,1,1,4),(499.513231920777,500.364528906586,501.364016628588,502.363504350589,
502.86324821159,503.362992072591,504.362479794592,505.361967516594,505.796417227957),
 .UNSPECIFIED.);
#438=B_SPLINE_CURVE_WITH_KNOTS('',3,(#18189,#18190,#18191,#18192,#18193,
#18194,#18195,#18196,#18197,#18198,#18199,#18200,#18201,#18202,#18203,#18204,
#18205,#18206,#18207,#18208,#18209,#18210,#18211,#18212,#18213,#18214,#18215,
#18216),.UNSPECIFIED.,.F.,.F.,(4,3,3,3,3,3,3,3,3,4),(499.513231920777,500.297432084827,
501.081632248876,501.865832412925,502.650032576974,503.434232741023,504.218432905073,
505.002633069122,505.786833233171,505.796417227957),.UNSPECIFIED.);
#439=B_SPLINE_CURVE_WITH_KNOTS('',3,(#18221,#18222,#18223,#18224,#18225,
#18226,#18227,#18228,#18229,#18230,#18231,#18232,#18233,#18234,#18235,#18236,
#18237,#18238,#18239,#18240,#18241,#18242,#18243,#18244,#18245,#18246,#18247,
#18248),.UNSPECIFIED.,.F.,.F.,(4,3,3,3,3,3,3,3,3,4),(493.230046613598,494.014246777647,
494.798446941696,495.582647105745,496.366847269795,497.151047433844,497.935247597893,
498.719447761942,499.503647925992,499.513231920777),.UNSPECIFIED.);
#440=B_SPLINE_CURVE_WITH_KNOTS('',3,(#18249,#18250,#18251,#18252,#18253,
#18254,#18255,#18256,#18257,#18258,#18259,#18260,#18261,#18262,#18263,#18264,
#18265,#18266,#18267,#18268,#18269,#18270,#18271,#18272,#18273,#18274,#18275,
#18276),.UNSPECIFIED.,.F.,.F.,(4,3,3,3,3,3,3,3,3,4),(493.230046613598,494.014246777647,
494.798446941696,495.582647105745,496.366847269794,497.151047433844,497.935247597893,
498.719447761942,499.503647925991,499.513231920777),.UNSPECIFIED.);
#441=B_SPLINE_CURVE_WITH_KNOTS('',3,(#18281,#18282,#18283,#18284,#18285,
#18286,#18287,#18288,#18289,#18290,#18291,#18292,#18293,#18294,#18295,#18296,
#18297,#18298,#18299,#18300,#18301,#18302,#18303,#18304,#18305,#18306,#18307,
#18308),.UNSPECIFIED.,.F.,.F.,(4,3,3,3,3,3,3,3,3,4),(486.946861306418,487.731061470467,
488.515261634516,489.299461798566,490.083661962615,490.867862126664,491.652062290713,
492.436262454762,493.220462618811,493.230046613598),.UNSPECIFIED.);
#442=B_SPLINE_CURVE_WITH_KNOTS('',3,(#18309,#18310,#18311,#18312,#18313,
#18314,#18315,#18316,#18317,#18318,#18319,#18320,#18321,#18322,#18323,#18324,
#18325,#18326,#18327,#18328,#18329,#18330,#18331,#18332,#18333,#18334,#18335,
#18336),.UNSPECIFIED.,.F.,.F.,(4,3,3,3,3,3,3,3,3,4),(486.946861306418,487.731061470467,
488.515261634517,489.299461798566,490.083661962615,490.867862126664,491.652062290713,
492.436262454762,493.220462618811,493.230046613598),.UNSPECIFIED.);
#443=B_SPLINE_CURVE_WITH_KNOTS('',3,(#18341,#18342,#18343,#18344,#18345,
#18346,#18347,#18348,#18349,#18350,#18351,#18352,#18353,#18354,#18355,#18356,
#18357,#18358,#18359,#18360,#18361,#18362,#18363,#18364,#18365,#18366,#18367,
#18368),.UNSPECIFIED.,.F.,.F.,(4,3,3,3,3,3,3,3,3,4),(480.663675999239,481.447876163288,
482.232076327337,483.016276491386,483.800476655435,484.584676819484,485.368876983533,
486.153077147583,486.937277311632,486.946861306418),.UNSPECIFIED.);
#444=B_SPLINE_CURVE_WITH_KNOTS('',3,(#18369,#18370,#18371,#18372,#18373,
#18374,#18375,#18376,#18377,#18378,#18379,#18380,#18381,#18382,#18383,#18384,
#18385,#18386,#18387,#18388,#18389,#18390,#18391,#18392,#18393,#18394,#18395,
#18396),.UNSPECIFIED.,.F.,.F.,(4,3,3,3,3,3,3,3,3,4),(480.663675999239,481.447876163288,
482.232076327337,483.016276491386,483.800476655435,484.584676819485,485.368876983534,
486.153077147583,486.937277311632,486.946861306418),.UNSPECIFIED.);
#445=B_SPLINE_CURVE_WITH_KNOTS('',3,(#18401,#18402,#18403,#18404,#18405,
#18406,#18407,#18408,#18409,#18410,#18411,#18412,#18413,#18414,#18415,#18416,
#18417,#18418,#18419,#18420,#18421,#18422,#18423,#18424,#18425,#18426,#18427,
#18428),.UNSPECIFIED.,.F.,.F.,(4,3,3,3,3,3,3,3,3,4),(474.380490692059,475.164690856108,
475.948891020157,476.733091184207,477.517291348256,478.301491512305,479.085691676354,
479.869891840403,480.654092004453,480.663675999239),.UNSPECIFIED.);
#446=B_SPLINE_CURVE_WITH_KNOTS('',3,(#18429,#18430,#18431,#18432,#18433,
#18434,#18435,#18436,#18437,#18438,#18439,#18440,#18441,#18442,#18443,#18444,
#18445,#18446,#18447,#18448,#18449,#18450,#18451,#18452,#18453,#18454,#18455,
#18456),.UNSPECIFIED.,.F.,.F.,(4,3,3,3,3,3,3,3,3,4),(474.380490692059,475.164690856108,
475.948891020158,476.733091184207,477.517291348256,478.301491512305,479.085691676354,
479.869891840404,480.654092004453,480.663675999239),.UNSPECIFIED.);
#447=B_SPLINE_CURVE_WITH_KNOTS('',3,(#18461,#18462,#18463,#18464,#18465,
#18466,#18467,#18468,#18469,#18470,#18471,#18472,#18473,#18474,#18475,#18476,
#18477,#18478,#18479,#18480,#18481,#18482,#18483,#18484,#18485,#18486,#18487,
#18488),.UNSPECIFIED.,.F.,.F.,(4,3,3,3,3,3,3,3,3,4),(468.097305384879,468.881505548929,
469.665705712978,470.449905877027,471.234106041076,472.018306205126,472.802506369175,
473.586706533224,474.370906697273,474.380490692059),.UNSPECIFIED.);
#448=B_SPLINE_CURVE_WITH_KNOTS('',3,(#18489,#18490,#18491,#18492,#18493,
#18494,#18495,#18496,#18497,#18498,#18499),.UNSPECIFIED.,.F.,.F.,(4,1,1,
1,1,1,1,1,4),(468.09730538488,469.063155297986,470.062643019988,471.062130741989,
471.56187460299,472.061618463991,473.061106185992,474.060593907994,474.380490692059),
 .UNSPECIFIED.);
#449=B_SPLINE_CURVE_WITH_KNOTS('',3,(#18504,#18505,#18506,#18507,#18508,
#18509,#18510,#18511,#18512,#18513,#18514,#18515,#18516,#18517,#18518,#18519,
#18520,#18521,#18522,#18523,#18524,#18525,#18526,#18527,#18528,#18529,#18530,
#18531),.UNSPECIFIED.,.F.,.F.,(4,3,3,3,3,3,3,3,3,4),(461.8141200777,462.598320241749,
463.382520405798,464.166720569848,464.950920733897,465.735120897946,466.519321061995,
467.303521226045,468.087721390094,468.097305384879),.UNSPECIFIED.);
#450=B_SPLINE_CURVE_WITH_KNOTS('',3,(#18532,#18533,#18534,#18535,#18536,
#18537,#18538,#18539,#18540,#18541,#18542,#18543,#18544,#18545,#18546,#18547,
#18548,#18549,#18550,#18551,#18552,#18553,#18554,#18555,#18556,#18557,#18558,
#18559),.UNSPECIFIED.,.F.,.F.,(4,3,3,3,3,3,3,3,3,4),(461.8141200777,462.598320241749,
463.382520405798,464.166720569848,464.950920733897,465.735120897946,466.519321061995,
467.303521226044,468.087721390094,468.09730538488),.UNSPECIFIED.);
#451=B_SPLINE_CURVE_WITH_KNOTS('',3,(#18564,#18565,#18566,#18567,#18568,
#18569,#18570,#18571,#18572,#18573,#18574,#18575,#18576,#18577,#18578,#18579,
#18580,#18581,#18582,#18583,#18584,#18585,#18586,#18587,#18588,#18589,#18590,
#18591),.UNSPECIFIED.,.F.,.F.,(4,3,3,3,3,3,3,3,3,4),(455.53093477052,456.31513493457,
457.099335098619,457.883535262668,458.667735426717,459.451935590767,460.236135754816,
461.020335918865,461.804536082914,461.8141200777),.UNSPECIFIED.);
#452=B_SPLINE_CURVE_WITH_KNOTS('',3,(#18592,#18593,#18594,#18595,#18596,
#18597,#18598,#18599,#18600,#18601,#18602,#18603,#18604,#18605,#18606,#18607,
#18608,#18609,#18610,#18611,#18612,#18613,#18614,#18615,#18616,#18617,#18618,
#18619),.UNSPECIFIED.,.F.,.F.,(4,3,3,3,3,3,3,3,3,4),(455.53093477052,456.31513493457,
457.099335098619,457.883535262668,458.667735426717,459.451935590766,460.236135754816,
461.020335918865,461.804536082914,461.8141200777),.UNSPECIFIED.);
#453=B_SPLINE_CURVE_WITH_KNOTS('',3,(#18624,#18625,#18626,#18627,#18628,
#18629,#18630,#18631,#18632,#18633,#18634,#18635,#18636,#18637,#18638,#18639,
#18640,#18641,#18642,#18643,#18644,#18645,#18646,#18647,#18648,#18649,#18650,
#18651),.UNSPECIFIED.,.F.,.F.,(4,3,3,3,3,3,3,3,3,4),(449.247749463341,450.03194962739,
450.816149791439,451.600349955488,452.384550119537,453.168750283587,453.952950447636,
454.737150611685,455.521350775734,455.53093477052),.UNSPECIFIED.);
#454=B_SPLINE_CURVE_WITH_KNOTS('',3,(#18652,#18653,#18654,#18655,#18656,
#18657,#18658,#18659,#18660,#18661,#18662,#18663,#18664,#18665,#18666,#18667,
#18668,#18669,#18670,#18671,#18672,#18673,#18674,#18675,#18676,#18677,#18678,
#18679),.UNSPECIFIED.,.F.,.F.,(4,3,3,3,3,3,3,3,3,4),(449.247749463341,450.03194962739,
450.816149791439,451.600349955488,452.384550119538,453.168750283587,453.952950447636,
454.737150611685,455.521350775734,455.53093477052),.UNSPECIFIED.);
#455=B_SPLINE_CURVE_WITH_KNOTS('',3,(#18684,#18685,#18686,#18687,#18688,
#18689,#18690,#18691,#18692,#18693,#18694,#18695,#18696,#18697,#18698,#18699,
#18700,#18701,#18702,#18703,#18704,#18705,#18706,#18707,#18708,#18709,#18710,
#18711),.UNSPECIFIED.,.F.,.F.,(4,3,3,3,3,3,3,3,3,4),(442.964564156161,443.74876432021,
444.532964484259,445.317164648309,446.101364812358,446.885564976407,447.669765140456,
448.453965304505,449.238165468555,449.247749463341),.UNSPECIFIED.);
#456=B_SPLINE_CURVE_WITH_KNOTS('',3,(#18712,#18713,#18714,#18715,#18716,
#18717,#18718,#18719,#18720,#18721,#18722,#18723,#18724,#18725,#18726,#18727,
#18728,#18729,#18730,#18731,#18732,#18733,#18734,#18735,#18736,#18737,#18738,
#18739),.UNSPECIFIED.,.F.,.F.,(4,3,3,3,3,3,3,3,3,4),(442.964564156161,443.748764320211,
444.53296448426,445.317164648309,446.101364812358,446.885564976407,447.669765140457,
448.453965304506,449.238165468555,449.247749463341),.UNSPECIFIED.);
#457=B_SPLINE_CURVE_WITH_KNOTS('',3,(#18744,#18745,#18746,#18747,#18748,
#18749,#18750,#18751,#18752,#18753,#18754),.UNSPECIFIED.,.F.,.F.,(4,1,1,
1,1,1,1,1,4),(436.681378848981,437.396802420487,438.396290142489,439.39577786449,
439.895521725491,440.395265586492,441.394753308494,442.394241030495,442.964564156161),
 .UNSPECIFIED.);
#458=B_SPLINE_CURVE_WITH_KNOTS('',3,(#18755,#18756,#18757,#18758,#18759,
#18760,#18761,#18762,#18763,#18764),.UNSPECIFIED.,.F.,.F.,(4,1,1,1,1,1,
1,4),(436.681378848982,437.079548193936,438.079035915937,439.078523637939,
440.078011359941,441.077499081942,442.076986803944,442.964564156161),
 .UNSPECIFIED.);
#459=B_SPLINE_CURVE_WITH_KNOTS('',3,(#18769,#18770,#18771,#18772,#18773,
#18774,#18775,#18776,#18777,#18778,#18779,#18780),.UNSPECIFIED.,.F.,.F.,
(4,1,1,1,1,1,1,1,1,4),(430.398193541802,430.400388366476,431.399876088478,
432.399363810479,432.89910767148,433.398851532481,434.398339254483,435.397826976484,
436.397314698486,436.681378848981),.UNSPECIFIED.);
#460=B_SPLINE_CURVE_WITH_KNOTS('',3,(#18781,#18782,#18783,#18784,#18785,
#18786,#18787,#18788,#18789,#18790,#18791,#18792,#18793,#18794,#18795,#18796,
#18797,#18798,#18799,#18800,#18801,#18802,#18803,#18804,#18805,#18806,#18807,
#18808),.UNSPECIFIED.,.F.,.F.,(4,3,3,3,3,3,3,3,3,4),(430.398193541802,431.182393705851,
431.966593869901,432.75079403395,433.534994197999,434.319194362049,435.103394526098,
435.887594690147,436.671794854196,436.681378848982),.UNSPECIFIED.);
#461=B_SPLINE_CURVE_WITH_KNOTS('',3,(#18813,#18814,#18815,#18816,#18817,
#18818,#18819,#18820,#18821,#18822,#18823,#18824,#18825,#18826,#18827,#18828,
#18829,#18830,#18831,#18832,#18833,#18834,#18835,#18836,#18837,#18838,#18839,
#18840),.UNSPECIFIED.,.F.,.F.,(4,3,3,3,3,3,3,3,3,4),(424.115008234622,424.899208398672,
425.683408562721,426.46760872677,427.251808890819,428.036009054868,428.820209218918,
429.604409382967,430.388609547016,430.398193541802),.UNSPECIFIED.);
#462=B_SPLINE_CURVE_WITH_KNOTS('',3,(#18841,#18842,#18843,#18844,#18845,
#18846,#18847,#18848,#18849,#18850,#18851,#18852,#18853,#18854,#18855,#18856,
#18857,#18858,#18859,#18860,#18861,#18862,#18863,#18864,#18865,#18866,#18867,
#18868),.UNSPECIFIED.,.F.,.F.,(4,3,3,3,3,3,3,3,3,4),(424.115008234623,424.899208398672,
425.683408562721,426.46760872677,427.25180889082,428.036009054869,428.820209218918,
429.604409382967,430.388609547017,430.398193541802),.UNSPECIFIED.);
#463=B_SPLINE_CURVE_WITH_KNOTS('',3,(#18873,#18874,#18875,#18876,#18877,
#18878,#18879,#18880,#18881,#18882,#18883,#18884,#18885,#18886,#18887,#18888,
#18889,#18890,#18891,#18892,#18893,#18894,#18895,#18896,#18897,#18898,#18899,
#18900),.UNSPECIFIED.,.F.,.F.,(4,3,3,3,3,3,3,3,3,4),(417.831822927443,418.616023091492,
419.400223255541,420.18442341959,420.968623583639,421.752823747689,422.537023911738,
423.321224075787,424.105424239836,424.115008234622),.UNSPECIFIED.);
#464=B_SPLINE_CURVE_WITH_KNOTS('',3,(#18901,#18902,#18903,#18904,#18905,
#18906,#18907,#18908,#18909,#18910,#18911,#18912,#18913,#18914,#18915,#18916,
#18917,#18918,#18919,#18920,#18921,#18922,#18923,#18924,#18925,#18926,#18927,
#18928),.UNSPECIFIED.,.F.,.F.,(4,3,3,3,3,3,3,3,3,4),(417.831822927443,418.616023091492,
419.400223255541,420.184423419591,420.96862358364,421.752823747689,422.537023911738,
423.321224075787,424.105424239836,424.115008234623),.UNSPECIFIED.);
#465=B_SPLINE_CURVE_WITH_KNOTS('',3,(#18933,#18934,#18935,#18936,#18937,
#18938,#18939,#18940,#18941,#18942,#18943),.UNSPECIFIED.,.F.,.F.,(4,1,1,
1,1,1,1,1,4),(411.548637620263,411.909865509447,412.409609370448,413.40909709245,
414.408584814451,415.408072536453,416.407560258454,417.407047980456,417.831822927443),
 .UNSPECIFIED.);
#466=B_SPLINE_CURVE_WITH_KNOTS('',3,(#18944,#18945,#18946,#18947,#18948,
#18949,#18950,#18951,#18952,#18953,#18954,#18955,#18956,#18957,#18958,#18959,
#18960,#18961,#18962,#18963,#18964,#18965,#18966,#18967,#18968,#18969,#18970,
#18971),.UNSPECIFIED.,.F.,.F.,(4,3,3,3,3,3,3,3,3,4),(411.548637620263,412.332837784313,
413.117037948362,413.901238112411,414.68543827646,415.469638440509,416.253838604559,
417.038038768608,417.822238932657,417.831822927443),.UNSPECIFIED.);
#467=B_SPLINE_CURVE_WITH_KNOTS('',3,(#18976,#18977,#18978,#18979,#18980,
#18981,#18982,#18983,#18984,#18985,#18986,#18987,#18988,#18989,#18990,#18991,
#18992,#18993,#18994,#18995,#18996,#18997,#18998,#18999,#19000,#19001,#19002,
#19003),.UNSPECIFIED.,.F.,.F.,(4,3,3,3,3,3,3,3,3,4),(405.265452313084,406.049652477133,
406.833852641182,407.618052805231,408.40225296928,409.186453133329,409.970653297379,
410.754853461428,411.539053625477,411.548637620263),.UNSPECIFIED.);
#468=B_SPLINE_CURVE_WITH_KNOTS('',3,(#19004,#19005,#19006,#19007,#19008,
#19009,#19010,#19011,#19012,#19013,#19014),.UNSPECIFIED.,.F.,.F.,(4,1,1,
1,1,1,1,1,4),(405.265452313084,406.095428811887,407.094916533889,408.09440425589,
408.594148116891,409.093891977892,410.093379699894,411.092867421895,411.548637620263),
 .UNSPECIFIED.);
#469=B_SPLINE_CURVE_WITH_KNOTS('',3,(#19019,#19020,#19021,#19022,#19023,
#19024,#19025,#19026,#19027,#19028,#19029),.UNSPECIFIED.,.F.,.F.,(4,1,1,
1,1,1,1,1,4),(398.982267005904,399.416268984428,400.415756706429,401.415244428431,
402.414732150432,403.414219872434,404.413707594436,404.913451455436,405.265452313084),
 .UNSPECIFIED.);
#470=B_SPLINE_CURVE_WITH_KNOTS('',3,(#19030,#19031,#19032,#19033,#19034,
#19035,#19036,#19037,#19038,#19039,#19040,#19041,#19042,#19043,#19044,#19045,
#19046,#19047,#19048,#19049,#19050,#19051,#19052,#19053,#19054,#19055,#19056,
#19057),.UNSPECIFIED.,.F.,.F.,(4,3,3,3,3,3,3,3,3,4),(398.982267005904,399.766467169954,
400.550667334003,401.334867498052,402.119067662101,402.903267826151,403.6874679902,
404.471668154249,405.255868318298,405.265452313084),.UNSPECIFIED.);
#471=B_SPLINE_CURVE_WITH_KNOTS('',3,(#19062,#19063,#19064,#19065,#19066,
#19067,#19068,#19069,#19070,#19071,#19072,#19073,#19074,#19075,#19076,#19077,
#19078,#19079,#19080,#19081,#19082,#19083,#19084,#19085,#19086,#19087,#19088,
#19089),.UNSPECIFIED.,.F.,.F.,(4,3,3,3,3,3,3,3,3,4),(392.699081698725,393.483281862774,
394.267482026823,395.051682190872,395.835882354922,396.620082518971,397.40428268302,
398.188482847069,398.972683011119,398.982267005904),.UNSPECIFIED.);
#472=B_SPLINE_CURVE_WITH_KNOTS('',3,(#19090,#19091,#19092,#19093,#19094,
#19095,#19096,#19097,#19098,#19099,#19100,#19101,#19102,#19103,#19104,#19105,
#19106,#19107,#19108,#19109,#19110,#19111,#19112,#19113,#19114,#19115,#19116,
#19117),.UNSPECIFIED.,.F.,.F.,(4,3,3,3,3,3,3,3,3,4),(392.699081698725,393.483281862774,
394.267482026823,395.051682190872,395.835882354921,396.620082518971,397.40428268302,
398.188482847069,398.972683011118,398.982267005904),.UNSPECIFIED.);
#473=B_SPLINE_CURVE_WITH_KNOTS('',3,(#19122,#19123,#19124,#19125,#19126,
#19127,#19128,#19129,#19130,#19131,#19132,#19133,#19134,#19135,#19136,#19137,
#19138,#19139,#19140,#19141,#19142,#19143,#19144,#19145,#19146,#19147,#19148,
#19149),.UNSPECIFIED.,.F.,.F.,(4,3,3,3,3,3,3,3,3,4),(386.415896391545,387.200096555594,
387.984296719643,388.768496883693,389.552697047742,390.336897211791,391.12109737584,
391.905297539889,392.689497703939,392.699081698725),.UNSPECIFIED.);
#474=B_SPLINE_CURVE_WITH_KNOTS('',3,(#19150,#19151,#19152,#19153,#19154,
#19155,#19156,#19157,#19158,#19159,#19160,#19161,#19162,#19163,#19164,#19165,
#19166,#19167,#19168,#19169,#19170,#19171,#19172,#19173,#19174,#19175,#19176,
#19177),.UNSPECIFIED.,.F.,.F.,(4,3,3,3,3,3,3,3,3,4),(386.415896391545,387.200096555594,
387.984296719644,388.768496883693,389.552697047742,390.336897211791,391.12109737584,
391.90529753989,392.689497703939,392.699081698725),.UNSPECIFIED.);
#475=B_SPLINE_CURVE_WITH_KNOTS('',3,(#19182,#19183,#19184,#19185,#19186,
#19187,#19188,#19189,#19190,#19191,#19192),.UNSPECIFIED.,.F.,.F.,(4,1,1,
1,1,1,1,1,4),(380.132711084365,380.426002266398,381.4254899884,382.424977710401,
383.424465432403,383.924209293403,384.423953154404,385.423440876406,386.415896391545),
 .UNSPECIFIED.);
#476=B_SPLINE_CURVE_WITH_KNOTS('',3,(#19193,#19194,#19195,#19196,#19197,
#19198,#19199,#19200,#19201,#19202,#19203,#19204,#19205,#19206,#19207,#19208,
#19209,#19210,#19211,#19212,#19213,#19214,#19215,#19216,#19217,#19218,#19219,
#19220),.UNSPECIFIED.,.F.,.F.,(4,3,3,3,3,3,3,3,3,4),(380.132711084366,380.916911248415,
381.701111412464,382.485311576513,383.269511740562,384.053711904611,384.837912068661,
385.62211223271,386.406312396759,386.415896391545),.UNSPECIFIED.);
#477=B_SPLINE_CURVE_WITH_KNOTS('',3,(#19225,#19226,#19227,#19228,#19229,
#19230,#19231,#19232,#19233,#19234,#19235),.UNSPECIFIED.,.F.,.F.,(4,1,1,
1,1,1,1,1,4),(373.849525777186,374.429075934389,375.42856365639,376.428051378392,
376.927795239393,377.427539100393,378.427026822395,379.426514544396,380.132711084365),
 .UNSPECIFIED.);
#478=B_SPLINE_CURVE_WITH_KNOTS('',3,(#19236,#19237,#19238,#19239,#19240,
#19241,#19242,#19243,#19244,#19245,#19246,#19247,#19248,#19249,#19250,#19251,
#19252,#19253,#19254,#19255,#19256,#19257,#19258,#19259,#19260,#19261,#19262,
#19263),.UNSPECIFIED.,.F.,.F.,(4,3,3,3,3,3,3,3,3,4),(373.849525777186,374.633725941235,
375.417926105284,376.202126269334,376.986326433383,377.770526597432,378.554726761481,
379.33892692553,380.12312708958,380.132711084366),.UNSPECIFIED.);
#479=B_SPLINE_CURVE_WITH_KNOTS('',3,(#19268,#19269,#19270,#19271,#19272,
#19273,#19274,#19275,#19276,#19277,#19278,#19279,#19280,#19281,#19282,#19283,
#19284,#19285,#19286,#19287,#19288,#19289,#19290,#19291,#19292,#19293,#19294,
#19295),.UNSPECIFIED.,.F.,.F.,(4,3,3,3,3,3,3,3,3,4),(367.566340470006,368.350540634056,
369.134740798105,369.918940962154,370.703141126203,371.487341290252,372.271541454301,
373.055741618351,373.8399417824,373.849525777186),.UNSPECIFIED.);
#480=B_SPLINE_CURVE_WITH_KNOTS('',3,(#19296,#19297,#19298,#19299,#19300,
#19301,#19302,#19303,#19304,#19305,#19306,#19307,#19308,#19309,#19310,#19311,
#19312,#19313,#19314,#19315,#19316,#19317,#19318,#19319,#19320,#19321,#19322,
#19323),.UNSPECIFIED.,.F.,.F.,(4,3,3,3,3,3,3,3,3,4),(367.566340470007,368.350540634056,
369.134740798105,369.918940962155,370.703141126204,371.487341290253,372.271541454302,
373.055741618352,373.839941782401,373.849525777186),.UNSPECIFIED.);
#481=B_SPLINE_CURVE_WITH_KNOTS('',3,(#19328,#19329,#19330,#19331,#19332,
#19333,#19334,#19335,#19336,#19337,#19338,#19339,#19340,#19341,#19342,#19343,
#19344,#19345,#19346,#19347,#19348,#19349,#19350,#19351,#19352,#19353,#19354,
#19355),.UNSPECIFIED.,.F.,.F.,(4,3,3,3,3,3,3,3,3,4),(361.283155162827,362.067355326876,
362.851555490925,363.635755654975,364.419955819024,365.204155983073,365.988356147122,
366.772556311172,367.556756475221,367.566340470006),.UNSPECIFIED.);
#482=B_SPLINE_CURVE_WITH_KNOTS('',3,(#19356,#19357,#19358,#19359,#19360,
#19361,#19362,#19363,#19364,#19365,#19366,#19367,#19368,#19369,#19370,#19371,
#19372,#19373,#19374,#19375,#19376,#19377,#19378,#19379,#19380,#19381,#19382,
#19383),.UNSPECIFIED.,.F.,.F.,(4,3,3,3,3,3,3,3,3,4),(361.283155162827,362.067355326876,
362.851555490926,363.635755654975,364.419955819024,365.204155983073,365.988356147123,
366.772556311172,367.556756475221,367.566340470007),.UNSPECIFIED.);
#483=B_SPLINE_CURVE_WITH_KNOTS('',3,(#19388,#19389,#19390,#19391,#19392,
#19393,#19394,#19395,#19396,#19397,#19398,#19399,#19400,#19401,#19402,#19403,
#19404,#19405,#19406,#19407,#19408,#19409,#19410,#19411,#19412,#19413,#19414,
#19415),.UNSPECIFIED.,.F.,.F.,(4,3,3,3,3,3,3,3,3,4),(354.999969855647,355.784170019696,
356.568370183746,357.352570347795,358.136770511844,358.920970675893,359.705170839943,
360.489371003992,361.273571168041,361.283155162827),.UNSPECIFIED.);
#484=B_SPLINE_CURVE_WITH_KNOTS('',3,(#19416,#19417,#19418,#19419,#19420,
#19421,#19422,#19423,#19424,#19425,#19426,#19427,#19428,#19429,#19430,#19431,
#19432,#19433,#19434,#19435,#19436,#19437,#19438,#19439,#19440,#19441,#19442,
#19443),.UNSPECIFIED.,.F.,.F.,(4,3,3,3,3,3,3,3,3,4),(354.999969855647,355.784170019697,
356.568370183746,357.352570347795,358.136770511844,358.920970675893,359.705170839943,
360.489371003992,361.273571168041,361.283155162827),.UNSPECIFIED.);
#485=B_SPLINE_CURVE_WITH_KNOTS('',3,(#19448,#19449,#19450,#19451,#19452,
#19453,#19454,#19455,#19456,#19457,#19458,#19459,#19460,#19461,#19462,#19463,
#19464,#19465,#19466,#19467,#19468,#19469,#19470,#19471,#19472,#19473,#19474,
#19475),.UNSPECIFIED.,.F.,.F.,(4,3,3,3,3,3,3,3,3,4),(348.716784548468,349.500984712517,
350.285184876566,351.069385040616,351.853585204665,352.637785368714,353.421985532763,
354.206185696813,354.990385860862,354.999969855647),.UNSPECIFIED.);
#486=B_SPLINE_CURVE_WITH_KNOTS('',3,(#19476,#19477,#19478,#19479,#19480,
#19481,#19482,#19483,#19484,#19485,#19486,#19487,#19488,#19489,#19490,#19491,
#19492,#19493,#19494,#19495,#19496,#19497,#19498,#19499,#19500,#19501,#19502,
#19503),.UNSPECIFIED.,.F.,.F.,(4,3,3,3,3,3,3,3,3,4),(348.716784548468,349.500984712517,
350.285184876566,351.069385040615,351.853585204664,352.637785368713,353.421985532762,
354.206185696811,354.990385860861,354.999969855647),.UNSPECIFIED.);
#487=B_SPLINE_CURVE_WITH_KNOTS('',3,(#19508,#19509,#19510,#19511,#19512,
#19513,#19514,#19515,#19516,#19517,#19518,#19519,#19520,#19521,#19522,#19523,
#19524,#19525,#19526,#19527,#19528,#19529,#19530,#19531,#19532,#19533,#19534,
#19535),.UNSPECIFIED.,.F.,.F.,(4,3,3,3,3,3,3,3,3,4),(342.433599241288,343.217799405337,
344.001999569386,344.786199733435,345.570399897485,346.354600061534,347.138800225583,
347.923000389632,348.707200553681,348.716784548468),.UNSPECIFIED.);
#488=B_SPLINE_CURVE_WITH_KNOTS('',3,(#19536,#19537,#19538,#19539,#19540,
#19541,#19542,#19543,#19544,#19545,#19546),.UNSPECIFIED.,.F.,.F.,(4,1,1,
1,1,1,1,1,4),(342.433599241288,343.127702325789,344.12719004779,345.126677769792,
345.626421630792,346.126165491793,347.125653213795,348.125140935796,348.716784548468),
 .UNSPECIFIED.);
#489=B_SPLINE_CURVE_WITH_KNOTS('',3,(#19551,#19552,#19553,#19554,#19555,
#19556,#19557,#19558,#19559,#19560,#19561,#19562,#19563,#19564,#19565,#19566,
#19567,#19568,#19569,#19570,#19571,#19572,#19573,#19574,#19575,#19576,#19577,
#19578),.UNSPECIFIED.,.F.,.F.,(4,3,3,3,3,3,3,3,3,4),(336.150413934109,336.934614098158,
337.718814262207,338.503014426256,339.287214590305,340.071414754354,340.855614918403,
341.639815082453,342.424015246502,342.433599241288),.UNSPECIFIED.);
#490=B_SPLINE_CURVE_WITH_KNOTS('',3,(#19579,#19580,#19581,#19582,#19583,
#19584,#19585,#19586,#19587,#19588,#19589),.UNSPECIFIED.,.F.,.F.,(4,1,1,
1,1,1,1,1,4),(336.150413934109,337.130775993779,338.130263715781,338.630007576781,
339.129751437782,340.129239159784,341.128726881785,342.128214603787,342.433599241288),
 .UNSPECIFIED.);
#491=B_SPLINE_CURVE_WITH_KNOTS('',3,(#19594,#19595,#19596,#19597,#19598,
#19599,#19600,#19601,#19602,#19603,#19604,#19605,#19606,#19607,#19608,#19609,
#19610,#19611,#19612,#19613,#19614,#19615,#19616,#19617,#19618,#19619,#19620,
#19621),.UNSPECIFIED.,.F.,.F.,(4,3,3,3,3,3,3,3,3,4),(329.867228626929,330.651428790978,
331.435628955027,332.219829119077,333.004029283126,333.788229447175,334.572429611224,
335.356629775273,336.140829939323,336.150413934109),.UNSPECIFIED.);
#492=B_SPLINE_CURVE_WITH_KNOTS('',3,(#19622,#19623,#19624,#19625,#19626,
#19627,#19628,#19629,#19630,#19631,#19632,#19633,#19634,#19635,#19636,#19637,
#19638,#19639,#19640,#19641,#19642,#19643,#19644,#19645,#19646,#19647,#19648,
#19649),.UNSPECIFIED.,.F.,.F.,(4,3,3,3,3,3,3,3,3,4),(329.867228626929,330.651428790978,
331.435628955028,332.219829119077,333.004029283126,333.788229447175,334.572429611224,
335.356629775274,336.140829939323,336.150413934109),.UNSPECIFIED.);
#493=B_SPLINE_CURVE_WITH_KNOTS('',3,(#19654,#19655,#19656,#19657,#19658,
#19659,#19660,#19661,#19662,#19663,#19664,#19665,#19666,#19667,#19668,#19669,
#19670,#19671,#19672,#19673,#19674,#19675,#19676,#19677,#19678,#19679,#19680,
#19681),.UNSPECIFIED.,.F.,.F.,(4,3,3,3,3,3,3,3,3,4),(323.584043319749,324.368243483799,
325.152443647848,325.936643811897,326.720843975946,327.505044139995,328.289244304045,
329.073444468094,329.857644632143,329.867228626929),.UNSPECIFIED.);
#494=B_SPLINE_CURVE_WITH_KNOTS('',3,(#19682,#19683,#19684,#19685,#19686,
#19687,#19688,#19689,#19690,#19691,#19692,#19693,#19694,#19695,#19696,#19697,
#19698,#19699,#19700,#19701,#19702,#19703,#19704,#19705,#19706,#19707,#19708,
#19709),.UNSPECIFIED.,.F.,.F.,(4,3,3,3,3,3,3,3,3,4),(323.58404331975,324.368243483799,
325.152443647848,325.936643811897,326.720843975946,327.505044139996,328.289244304045,
329.073444468094,329.857644632143,329.867228626929),.UNSPECIFIED.);
#495=B_SPLINE_CURVE_WITH_KNOTS('',3,(#19714,#19715,#19716,#19717,#19718,
#19719,#19720,#19721,#19722,#19723,#19724,#19725,#19726,#19727,#19728,#19729,
#19730,#19731,#19732,#19733,#19734,#19735,#19736,#19737,#19738,#19739,#19740,
#19741),.UNSPECIFIED.,.F.,.F.,(4,3,3,3,3,3,3,3,3,4),(317.30085801257,318.085058176619,
318.869258340668,319.653458504718,320.437658668767,321.221858832816,322.006058996865,
322.790259160915,323.574459324964,323.584043319749),.UNSPECIFIED.);
#496=B_SPLINE_CURVE_WITH_KNOTS('',3,(#19742,#19743,#19744,#19745,#19746,
#19747,#19748,#19749,#19750,#19751,#19752),.UNSPECIFIED.,.F.,.F.,(4,1,1,
1,1,1,1,1,4),(317.30085801257,317.640765414749,318.140509275749,319.139996997751,
320.139484719752,321.138972441754,322.138460163756,323.137947885757,323.58404331975),
 .UNSPECIFIED.);
#497=B_SPLINE_CURVE_WITH_KNOTS('',3,(#19757,#19758,#19759,#19760,#19761,
#19762,#19763,#19764,#19765,#19766,#19767),.UNSPECIFIED.,.F.,.F.,(4,1,1,
1,1,1,1,1,4),(311.01767270539,311.46134944829,312.460837170291,313.460324892293,
313.960068753294,314.459812614295,315.459300336296,316.458788058298,317.30085801257),
 .UNSPECIFIED.);
#498=B_SPLINE_CURVE_WITH_KNOTS('',3,(#19768,#19769,#19770,#19771,#19772,
#19773,#19774,#19775,#19776,#19777,#19778,#19779,#19780,#19781,#19782,#19783,
#19784,#19785,#19786,#19787,#19788,#19789,#19790,#19791,#19792,#19793,#19794,
#19795),.UNSPECIFIED.,.F.,.F.,(4,3,3,3,3,3,3,3,3,4),(311.01767270539,311.80187286944,
312.586073033489,313.370273197538,314.154473361587,314.938673525636,315.722873689685,
316.507073853734,317.291274017784,317.30085801257),.UNSPECIFIED.);
#499=B_SPLINE_CURVE_WITH_KNOTS('',3,(#19800,#19801,#19802,#19803,#19804,
#19805,#19806,#19807,#19808,#19809,#19810,#19811,#19812,#19813,#19814,#19815,
#19816,#19817,#19818,#19819,#19820,#19821,#19822,#19823,#19824,#19825,#19826,
#19827),.UNSPECIFIED.,.F.,.F.,(4,3,3,3,3,3,3,3,3,4),(304.734487398211,305.51868756226,
306.302887726309,307.087087890358,307.871288054408,308.655488218457,309.439688382506,
310.223888546555,311.008088710604,311.01767270539),.UNSPECIFIED.);
#500=B_SPLINE_CURVE_WITH_KNOTS('',3,(#19828,#19829,#19830,#19831,#19832,
#19833,#19834,#19835,#19836,#19837,#19838),.UNSPECIFIED.,.F.,.F.,(4,1,1,
1,1,1,1,1,4),(304.734487398211,305.147168889729,306.146656611731,307.146144333732,
308.145632055734,309.145119777735,310.144607499737,310.644351360738,311.01767270539),
 .UNSPECIFIED.);
#501=B_SPLINE_CURVE_WITH_KNOTS('',3,(#19843,#19844,#19845,#19846,#19847,
#19848,#19849,#19850,#19851,#19852,#19853,#19854,#19855,#19856,#19857,#19858,
#19859,#19860,#19861,#19862,#19863,#19864,#19865,#19866,#19867,#19868,#19869,
#19870),.UNSPECIFIED.,.F.,.F.,(4,3,3,3,3,3,3,3,3,4),(298.451302091031,299.23550225508,
300.019702419129,300.803902583179,301.588102747228,302.372302911277,303.156503075326,
303.940703239375,304.724903403425,304.734487398211),.UNSPECIFIED.);
#502=B_SPLINE_CURVE_WITH_KNOTS('',3,(#19871,#19872,#19873,#19874,#19875,
#19876,#19877,#19878,#19879,#19880,#19881,#19882,#19883,#19884,#19885,#19886,
#19887,#19888,#19889,#19890,#19891,#19892,#19893,#19894,#19895,#19896,#19897,
#19898),.UNSPECIFIED.,.F.,.F.,(4,3,3,3,3,3,3,3,3,4),(298.451302091031,299.235502255081,
300.01970241913,300.803902583179,301.588102747228,302.372302911278,303.156503075327,
303.940703239376,304.724903403425,304.734487398211),.UNSPECIFIED.);
#503=B_SPLINE_CURVE_WITH_KNOTS('',3,(#19903,#19904,#19905,#19906,#19907,
#19908,#19909,#19910,#19911,#19912,#19913),.UNSPECIFIED.,.F.,.F.,(4,1,1,
1,1,1,1,1,4),(292.168116783852,292.47108273026,293.470570452262,294.470058174263,
294.969802035264,295.469545896265,296.469033618266,297.468521340268,298.451302091031),
 .UNSPECIFIED.);
#504=B_SPLINE_CURVE_WITH_KNOTS('',3,(#19914,#19915,#19916,#19917,#19918,
#19919,#19920,#19921,#19922,#19923,#19924,#19925,#19926,#19927,#19928,#19929,
#19930,#19931,#19932,#19933,#19934,#19935,#19936,#19937,#19938,#19939,#19940,
#19941),.UNSPECIFIED.,.F.,.F.,(4,3,3,3,3,3,3,3,3,4),(292.168116783852,292.952316947901,
293.73651711195,294.520717276,295.304917440049,296.089117604098,296.873317768147,
297.657517932197,298.441718096246,298.451302091031),.UNSPECIFIED.);
#505=B_SPLINE_CURVE_WITH_KNOTS('',3,(#19946,#19947,#19948,#19949,#19950,
#19951,#19952,#19953,#19954,#19955,#19956,#19957,#19958,#19959,#19960,#19961,
#19962,#19963,#19964,#19965,#19966,#19967,#19968,#19969,#19970,#19971,#19972,
#19973),.UNSPECIFIED.,.F.,.F.,(4,3,3,3,3,3,3,3,3,4),(285.884931476672,286.669131640721,
287.45333180477,288.23753196882,289.021732132869,289.805932296918,290.590132460967,
291.374332625016,292.158532789066,292.168116783852),.UNSPECIFIED.);
#506=B_SPLINE_CURVE_WITH_KNOTS('',3,(#19974,#19975,#19976,#19977,#19978,
#19979,#19980,#19981,#19982,#19983,#19984,#19985,#19986,#19987,#19988,#19989,
#19990,#19991,#19992,#19993,#19994,#19995,#19996,#19997,#19998,#19999,#20000,
#20001),.UNSPECIFIED.,.F.,.F.,(4,3,3,3,3,3,3,3,3,4),(285.884931476672,286.669131640721,
287.453331804771,288.23753196882,289.021732132869,289.805932296918,290.590132460967,
291.374332625017,292.158532789066,292.168116783852),.UNSPECIFIED.);
#507=B_SPLINE_CURVE_WITH_KNOTS('',3,(#20006,#20007,#20008,#20009,#20010,
#20011,#20012,#20013,#20014,#20015,#20016,#20017,#20018,#20019,#20020,#20021,
#20022,#20023,#20024,#20025,#20026,#20027,#20028,#20029,#20030,#20031,#20032,
#20033),.UNSPECIFIED.,.F.,.F.,(4,3,3,3,3,3,3,3,3,4),(279.601746169492,280.385946333542,
281.170146497591,281.95434666164,282.738546825689,283.522746989739,284.306947153788,
285.091147317837,285.875347481886,285.884931476672),.UNSPECIFIED.);
#508=B_SPLINE_CURVE_WITH_KNOTS('',3,(#20034,#20035,#20036,#20037,#20038,
#20039,#20040,#20041,#20042,#20043,#20044,#20045,#20046,#20047,#20048,#20049,
#20050,#20051,#20052,#20053,#20054,#20055,#20056,#20057,#20058,#20059,#20060,
#20061),.UNSPECIFIED.,.F.,.F.,(4,3,3,3,3,3,3,3,3,4),(279.601746169493,280.385946333542,
281.170146497591,281.95434666164,282.738546825689,283.522746989739,284.306947153788,
285.091147317837,285.875347481886,285.884931476672),.UNSPECIFIED.);
#509=B_SPLINE_CURVE_WITH_KNOTS('',3,(#20066,#20067,#20068,#20069,#20070,
#20071,#20072,#20073,#20074,#20075,#20076,#20077,#20078,#20079,#20080,#20081,
#20082,#20083,#20084,#20085,#20086,#20087,#20088,#20089,#20090,#20091,#20092,
#20093),.UNSPECIFIED.,.F.,.F.,(4,3,3,3,3,3,3,3,3,4),(273.318560862313,274.102761026362,
274.886961190411,275.67116135446,276.45536151851,277.239561682559,278.023761846608,
278.807962010657,279.592162174706,279.601746169492),.UNSPECIFIED.);
#510=B_SPLINE_CURVE_WITH_KNOTS('',3,(#20094,#20095,#20096,#20097,#20098,
#20099,#20100,#20101,#20102,#20103,#20104,#20105,#20106,#20107,#20108,#20109,
#20110,#20111,#20112,#20113,#20114,#20115,#20116,#20117,#20118,#20119,#20120,
#20121),.UNSPECIFIED.,.F.,.F.,(4,3,3,3,3,3,3,3,3,4),(273.318560862313,274.102761026362,
274.886961190412,275.671161354461,276.45536151851,277.239561682559,278.023761846609,
278.807962010658,279.592162174707,279.601746169493),.UNSPECIFIED.);
#511=B_SPLINE_CURVE_WITH_KNOTS('',3,(#20126,#20127,#20128,#20129,#20130,
#20131,#20132,#20133,#20134,#20135,#20136,#20137,#20138,#20139,#20140,#20141,
#20142,#20143,#20144,#20145,#20146,#20147,#20148,#20149,#20150,#20151,#20152,
#20153),.UNSPECIFIED.,.F.,.F.,(4,3,3,3,3,3,3,3,3,4),(267.035375555133,267.819575719182,
268.603775883232,269.387976047281,270.17217621133,270.956376375379,271.740576539428,
272.524776703478,273.308976867527,273.318560862313),.UNSPECIFIED.);
#512=B_SPLINE_CURVE_WITH_KNOTS('',3,(#20154,#20155,#20156,#20157,#20158,
#20159,#20160,#20161,#20162,#20163,#20164,#20165,#20166,#20167,#20168,#20169,
#20170,#20171,#20172,#20173,#20174,#20175,#20176,#20177,#20178,#20179,#20180,
#20181),.UNSPECIFIED.,.F.,.F.,(4,3,3,3,3,3,3,3,3,4),(267.035375555134,267.819575719183,
268.603775883232,269.387976047281,270.17217621133,270.956376375379,271.740576539428,
272.524776703478,273.308976867527,273.318560862313),.UNSPECIFIED.);
#513=B_SPLINE_CURVE_WITH_KNOTS('',3,(#20186,#20187,#20188,#20189,#20190,
#20191,#20192,#20193,#20194,#20195,#20196,#20197,#20198,#20199,#20200,#20201,
#20202,#20203,#20204,#20205,#20206,#20207,#20208,#20209,#20210,#20211,#20212,
#20213),.UNSPECIFIED.,.F.,.F.,(4,3,3,3,3,3,3,3,3,4),(260.752190247954,261.536390412003,
262.320590576052,263.104790740101,263.888990904151,264.6731910682,265.457391232249,
266.241591396298,267.025791560347,267.035375555133),.UNSPECIFIED.);
#514=B_SPLINE_CURVE_WITH_KNOTS('',3,(#20214,#20215,#20216,#20217,#20218,
#20219,#20220,#20221,#20222,#20223,#20224),.UNSPECIFIED.,.F.,.F.,(4,1,1,
1,1,1,1,1,4),(260.752190247954,261.16970912166,262.169196843661,263.168684565663,
263.668428426664,264.168172287665,265.167660009666,266.167147731668,267.035375555134),
 .UNSPECIFIED.);
#515=B_SPLINE_CURVE_WITH_KNOTS('',3,(#20229,#20230,#20231,#20232,#20233,
#20234,#20235,#20236,#20237,#20238,#20239,#20240,#20241,#20242,#20243,#20244,
#20245,#20246,#20247,#20248,#20249,#20250,#20251,#20252,#20253,#20254,#20255,
#20256),.UNSPECIFIED.,.F.,.F.,(4,3,3,3,3,3,3,3,3,4),(254.469004940774,255.253205104823,
256.037405268872,256.821605432922,257.605805596971,258.39000576102,259.174205925069,
259.958406089118,260.742606253167,260.752190247954),.UNSPECIFIED.);
#516=B_SPLINE_CURVE_WITH_KNOTS('',3,(#20257,#20258,#20259,#20260,#20261,
#20262,#20263,#20264,#20265,#20266,#20267,#20268,#20269,#20270,#20271,#20272,
#20273,#20274,#20275,#20276,#20277,#20278,#20279,#20280,#20281,#20282,#20283,
#20284),.UNSPECIFIED.,.F.,.F.,(4,3,3,3,3,3,3,3,3,4),(254.469004940774,255.253205104824,
256.037405268873,256.821605432922,257.605805596971,258.39000576102,259.174205925069,
259.958406089118,260.742606253168,260.752190247954),.UNSPECIFIED.);
#517=B_SPLINE_CURVE_WITH_KNOTS('',3,(#20289,#20290,#20291,#20292,#20293,
#20294,#20295,#20296,#20297,#20298,#20299,#20300,#20301,#20302,#20303,#20304,
#20305,#20306,#20307,#20308,#20309,#20310,#20311,#20312,#20313,#20314,#20315,
#20316),.UNSPECIFIED.,.F.,.F.,(4,3,3,3,3,3,3,3,3,4),(248.185819633595,248.970019797644,
249.754219961693,250.538420125742,251.322620289791,252.10682045384,252.89102061789,
253.675220781939,254.459420945988,254.469004940774),.UNSPECIFIED.);
#518=B_SPLINE_CURVE_WITH_KNOTS('',3,(#20317,#20318,#20319,#20320,#20321,
#20322,#20323,#20324,#20325,#20326,#20327,#20328,#20329,#20330,#20331,#20332,
#20333,#20334,#20335,#20336,#20337,#20338,#20339,#20340,#20341,#20342,#20343,
#20344),.UNSPECIFIED.,.F.,.F.,(4,3,3,3,3,3,3,3,3,4),(248.185819633595,248.970019797644,
249.754219961693,250.538420125742,251.322620289792,252.106820453841,252.89102061789,
253.675220781939,254.459420945988,254.469004940774),.UNSPECIFIED.);
#519=B_SPLINE_CURVE_WITH_KNOTS('',3,(#20349,#20350,#20351,#20352,#20353,
#20354,#20355,#20356,#20357,#20358,#20359,#20360,#20361,#20362,#20363,#20364,
#20365,#20366,#20367,#20368,#20369,#20370,#20371,#20372,#20373,#20374,#20375,
#20376),.UNSPECIFIED.,.F.,.F.,(4,3,3,3,3,3,3,3,3,4),(241.902634326415,242.686834490464,
243.471034654513,244.255234818563,245.039434982612,245.823635146661,246.60783531071,
247.392035474759,248.176235638809,248.185819633595),.UNSPECIFIED.);
#520=B_SPLINE_CURVE_WITH_KNOTS('',3,(#20377,#20378,#20379,#20380,#20381,
#20382,#20383,#20384,#20385,#20386,#20387,#20388,#20389,#20390,#20391,#20392,
#20393,#20394,#20395,#20396,#20397,#20398,#20399,#20400,#20401,#20402,#20403,
#20404),.UNSPECIFIED.,.F.,.F.,(4,3,3,3,3,3,3,3,3,4),(241.902634326415,242.686834490465,
243.471034654514,244.255234818563,245.039434982612,245.823635146661,246.60783531071,
247.39203547476,248.176235638809,248.185819633595),.UNSPECIFIED.);
#521=B_SPLINE_CURVE_WITH_KNOTS('',3,(#20409,#20410,#20411,#20412,#20413,
#20414,#20415,#20416,#20417,#20418,#20419),.UNSPECIFIED.,.F.,.F.,(4,1,1,
1,1,1,1,1,4),(235.619449019236,236.499770298172,237.499258020174,238.498745742176,
238.998489603176,239.498233464177,240.497721186179,241.49720890818,241.902634326415),
 .UNSPECIFIED.);
#522=B_SPLINE_CURVE_WITH_KNOTS('',3,(#20420,#20421,#20422,#20423,#20424,
#20425,#20426,#20427,#20428,#20429,#20430,#20431,#20432,#20433,#20434,#20435,
#20436,#20437,#20438,#20439,#20440,#20441,#20442,#20443,#20444,#20445,#20446,
#20447),.UNSPECIFIED.,.F.,.F.,(4,3,3,3,3,3,3,3,3,4),(235.619449019236,236.403649183285,
237.187849347334,237.972049511383,238.756249675432,239.540449839482,240.324650003531,
241.10885016758,241.893050331629,241.902634326415),.UNSPECIFIED.);
#523=B_SPLINE_CURVE_WITH_KNOTS('',3,(#20452,#20453,#20454,#20455,#20456,
#20457,#20458,#20459,#20460,#20461,#20462,#20463,#20464,#20465,#20466,#20467,
#20468,#20469,#20470,#20471,#20472,#20473,#20474,#20475,#20476,#20477,#20478,
#20479),.UNSPECIFIED.,.F.,.F.,(4,3,3,3,3,3,3,3,3,4),(229.336263712056,230.120463876105,
230.904664040154,231.688864204203,232.473064368253,233.257264532302,234.041464696351,
234.8256648604,235.609865024449,235.619449019236),.UNSPECIFIED.);
#524=B_SPLINE_CURVE_WITH_KNOTS('',3,(#20480,#20481,#20482,#20483,#20484,
#20485,#20486,#20487,#20488,#20489,#20490,#20491,#20492,#20493,#20494,#20495,
#20496,#20497,#20498,#20499,#20500,#20501,#20502,#20503,#20504,#20505,#20506,
#20507),.UNSPECIFIED.,.F.,.F.,(4,3,3,3,3,3,3,3,3,4),(229.336263712056,230.120463876105,
230.904664040155,231.688864204204,232.473064368253,233.257264532302,234.041464696352,
234.825664860401,235.60986502445,235.619449019236),.UNSPECIFIED.);
#525=B_SPLINE_CURVE_WITH_KNOTS('',3,(#20512,#20513,#20514,#20515,#20516,
#20517,#20518,#20519,#20520,#20521,#20522,#20523,#20524,#20525,#20526,#20527,
#20528,#20529,#20530,#20531,#20532,#20533,#20534,#20535,#20536,#20537,#20538,
#20539),.UNSPECIFIED.,.F.,.F.,(4,3,3,3,3,3,3,3,3,4),(223.053078404876,223.837278568926,
224.621478732975,225.405678897024,226.189879061073,226.974079225123,227.758279389172,
228.542479553221,229.32667971727,229.336263712056),.UNSPECIFIED.);
#526=B_SPLINE_CURVE_WITH_KNOTS('',3,(#20540,#20541,#20542,#20543,#20544,
#20545,#20546,#20547,#20548,#20549,#20550,#20551,#20552,#20553,#20554,#20555,
#20556,#20557,#20558,#20559,#20560,#20561,#20562,#20563,#20564,#20565,#20566,
#20567),.UNSPECIFIED.,.F.,.F.,(4,3,3,3,3,3,3,3,3,4),(223.053078404877,223.837278568926,
224.621478732975,225.405678897024,226.189879061073,226.974079225123,227.758279389172,
228.542479553221,229.32667971727,229.336263712056),.UNSPECIFIED.);
#527=B_SPLINE_CURVE_WITH_KNOTS('',3,(#20572,#20573,#20574,#20575,#20576,
#20577,#20578,#20579,#20580,#20581,#20582,#20583,#20584,#20585,#20586,#20587,
#20588,#20589,#20590,#20591,#20592,#20593,#20594,#20595,#20596,#20597,#20598,
#20599),.UNSPECIFIED.,.F.,.F.,(4,3,3,3,3,3,3,3,3,4),(216.769893097697,217.554093261746,
218.338293425795,219.122493589844,219.906693753894,220.690893917943,221.475094081992,
222.259294246041,223.043494410091,223.053078404876),.UNSPECIFIED.);
#528=B_SPLINE_CURVE_WITH_KNOTS('',3,(#20600,#20601,#20602,#20603,#20604,
#20605,#20606,#20607,#20608,#20609,#20610,#20611,#20612,#20613,#20614,#20615,
#20616,#20617,#20618,#20619,#20620,#20621,#20622,#20623,#20624,#20625,#20626,
#20627),.UNSPECIFIED.,.F.,.F.,(4,3,3,3,3,3,3,3,3,4),(216.769893097697,217.554093261746,
218.338293425795,219.122493589845,219.906693753894,220.690893917943,221.475094081992,
222.259294246042,223.043494410091,223.053078404877),.UNSPECIFIED.);
#529=B_SPLINE_CURVE_WITH_KNOTS('',3,(#20632,#20633,#20634,#20635,#20636,
#20637,#20638,#20639,#20640,#20641,#20642,#20643,#20644,#20645,#20646,#20647,
#20648,#20649,#20650,#20651,#20652,#20653,#20654,#20655,#20656,#20657,#20658,
#20659),.UNSPECIFIED.,.F.,.F.,(4,3,3,3,3,3,3,3,3,4),(210.486707790517,211.270907954566,
212.055108118616,212.839308282665,213.623508446714,214.407708610763,215.191908774813,
215.976108938862,216.760309102911,216.769893097697),.UNSPECIFIED.);
#530=B_SPLINE_CURVE_WITH_KNOTS('',3,(#20660,#20661,#20662,#20663,#20664,
#20665,#20666,#20667,#20668,#20669,#20670,#20671,#20672,#20673,#20674,#20675,
#20676,#20677,#20678,#20679,#20680,#20681,#20682,#20683,#20684,#20685,#20686,
#20687),.UNSPECIFIED.,.F.,.F.,(4,3,3,3,3,3,3,3,3,4),(210.486707790517,211.270907954567,
212.055108118616,212.839308282665,213.623508446714,214.407708610764,215.191908774813,
215.976108938862,216.760309102911,216.769893097697),.UNSPECIFIED.);
#531=B_SPLINE_CURVE_WITH_KNOTS('',3,(#20692,#20693,#20694,#20695,#20696,
#20697,#20698,#20699,#20700,#20701),.UNSPECIFIED.,.F.,.F.,(4,1,1,1,1,1,
1,4),(204.203522483338,204.516163194122,205.515650916124,206.515138638125,
207.514626360127,208.514114082129,209.51360180413,210.486707790517),
 .UNSPECIFIED.);
#532=B_SPLINE_CURVE_WITH_KNOTS('',3,(#20702,#20703,#20704,#20705,#20706,
#20707,#20708,#20709,#20710,#20711,#20712,#20713,#20714,#20715,#20716,#20717,
#20718,#20719,#20720,#20721,#20722,#20723,#20724,#20725,#20726,#20727,#20728,
#20729),.UNSPECIFIED.,.F.,.F.,(4,3,3,3,3,3,3,3,3,4),(204.203522483338,204.987722647387,
205.771922811436,206.556122975485,207.340323139535,208.124523303584,208.908723467633,
209.692923631682,210.477123795732,210.486707790517),.UNSPECIFIED.);
#533=B_SPLINE_CURVE_WITH_KNOTS('',3,(#20734,#20735,#20736,#20737,#20738,
#20739,#20740,#20741,#20742,#20743,#20744,#20745,#20746,#20747,#20748,#20749,
#20750,#20751,#20752,#20753,#20754,#20755,#20756,#20757,#20758,#20759,#20760,
#20761),.UNSPECIFIED.,.F.,.F.,(4,3,3,3,3,3,3,3,3,4),(197.920337176158,198.704537340207,
199.488737504256,200.272937668306,201.057137832355,201.841337996404,202.625538160453,
203.409738324502,204.193938488552,204.203522483338),.UNSPECIFIED.);
#534=B_SPLINE_CURVE_WITH_KNOTS('',3,(#20762,#20763,#20764,#20765,#20766,
#20767,#20768,#20769,#20770,#20771,#20772,#20773,#20774,#20775,#20776,#20777,
#20778,#20779,#20780,#20781,#20782,#20783,#20784,#20785,#20786,#20787,#20788,
#20789),.UNSPECIFIED.,.F.,.F.,(4,3,3,3,3,3,3,3,3,4),(197.920337176158,198.704537340207,
199.488737504257,200.272937668306,201.057137832355,201.841337996404,202.625538160453,
203.409738324502,204.193938488552,204.203522483338),.UNSPECIFIED.);
#535=B_SPLINE_CURVE_WITH_KNOTS('',3,(#20794,#20795,#20796,#20797,#20798,
#20799,#20800,#20801,#20802,#20803,#20804),.UNSPECIFIED.,.F.,.F.,(4,1,1,
1,1,1,1,1,4),(191.637151868978,192.522310530103,193.521798252105,194.521285974107,
195.520773696108,196.52026141811,197.020005279111,197.519749140111,197.920337176158),
 .UNSPECIFIED.);
#536=B_SPLINE_CURVE_WITH_KNOTS('',3,(#20805,#20806,#20807,#20808,#20809,
#20810,#20811,#20812,#20813,#20814,#20815,#20816,#20817,#20818,#20819,#20820,
#20821,#20822,#20823,#20824,#20825,#20826,#20827,#20828,#20829,#20830,#20831,
#20832),.UNSPECIFIED.,.F.,.F.,(4,3,3,3,3,3,3,3,3,4),(191.637151868979,192.421352033028,
193.205552197077,193.989752361126,194.773952525176,195.558152689225,196.342352853274,
197.126553017323,197.910753181373,197.920337176158),.UNSPECIFIED.);
#537=B_SPLINE_CURVE_WITH_KNOTS('',3,(#20837,#20838,#20839,#20840,#20841,
#20842,#20843,#20844,#20845,#20846,#20847,#20848,#20849,#20850,#20851,#20852,
#20853,#20854,#20855,#20856,#20857,#20858,#20859,#20860,#20861,#20862,#20863,
#20864),.UNSPECIFIED.,.F.,.F.,(4,3,3,3,3,3,3,3,3,4),(185.353966561799,186.138166725848,
186.922366889897,187.706567053947,188.490767217996,189.274967382045,190.059167546094,
190.843367710144,191.627567874193,191.637151868979),.UNSPECIFIED.);
#538=B_SPLINE_CURVE_WITH_KNOTS('',3,(#20865,#20866,#20867,#20868,#20869,
#20870,#20871,#20872,#20873,#20874,#20875,#20876,#20877,#20878,#20879,#20880,
#20881,#20882,#20883,#20884,#20885,#20886,#20887,#20888,#20889,#20890,#20891,
#20892),.UNSPECIFIED.,.F.,.F.,(4,3,3,3,3,3,3,3,3,4),(185.353966561799,186.138166725848,
186.922366889898,187.706567053947,188.490767217996,189.274967382045,190.059167546095,
190.843367710144,191.627567874193,191.637151868979),.UNSPECIFIED.);
#539=B_SPLINE_CURVE_WITH_KNOTS('',3,(#20897,#20898,#20899,#20900,#20901,
#20902,#20903,#20904,#20905,#20906,#20907,#20908,#20909,#20910,#20911,#20912,
#20913,#20914,#20915,#20916,#20917,#20918,#20919,#20920,#20921,#20922,#20923,
#20924),.UNSPECIFIED.,.F.,.F.,(4,3,3,3,3,3,3,3,3,4),(179.070781254619,179.854981418669,
180.639181582718,181.423381746767,182.207581910816,182.991782074865,183.775982238915,
184.560182402964,185.344382567013,185.353966561799),.UNSPECIFIED.);
#540=B_SPLINE_CURVE_WITH_KNOTS('',3,(#20925,#20926,#20927,#20928,#20929,
#20930,#20931,#20932,#20933,#20934,#20935,#20936,#20937,#20938,#20939,#20940,
#20941,#20942,#20943,#20944,#20945,#20946,#20947,#20948,#20949,#20950,#20951,
#20952),.UNSPECIFIED.,.F.,.F.,(4,3,3,3,3,3,3,3,3,4),(179.07078125462,179.854981418669,
180.639181582718,181.423381746767,182.207581910816,182.991782074865,183.775982238915,
184.560182402964,185.344382567013,185.353966561799),.UNSPECIFIED.);
#541=B_SPLINE_CURVE_WITH_KNOTS('',3,(#20957,#20958,#20959,#20960,#20961,
#20962,#20963,#20964,#20965,#20966,#20967),.UNSPECIFIED.,.F.,.F.,(4,1,1,
1,1,1,1,1,4),(172.78759594744,173.532043812074,174.531531534075,175.531019256077,
176.030763117078,176.530506978078,177.52999470008,178.529482422082,179.070781254619),
 .UNSPECIFIED.);
#542=B_SPLINE_CURVE_WITH_KNOTS('',3,(#20968,#20969,#20970,#20971,#20972,
#20973,#20974,#20975,#20976,#20977,#20978,#20979,#20980,#20981,#20982,#20983,
#20984,#20985,#20986,#20987,#20988,#20989,#20990,#20991,#20992,#20993,#20994,
#20995),.UNSPECIFIED.,.F.,.F.,(4,3,3,3,3,3,3,3,3,4),(172.78759594744,173.571796111489,
174.355996275539,175.140196439588,175.924396603637,176.708596767686,177.492796931735,
178.276997095785,179.061197259834,179.07078125462),.UNSPECIFIED.);
#543=B_SPLINE_CURVE_WITH_KNOTS('',3,(#21000,#21001,#21002,#21003,#21004,
#21005,#21006,#21007,#21008,#21009,#21010,#21011),.UNSPECIFIED.,.F.,.F.,
(4,1,1,1,1,1,1,1,1,4),(166.50441064026,166.535629758063,167.535117480064,
168.534605202066,169.034349063067,169.534092924067,170.533580646069,171.533068368071,
172.532556090072,172.78759594744),.UNSPECIFIED.);
#544=B_SPLINE_CURVE_WITH_KNOTS('',3,(#21012,#21013,#21014,#21015,#21016,
#21017,#21018,#21019,#21020,#21021,#21022,#21023,#21024,#21025,#21026,#21027,
#21028,#21029,#21030,#21031,#21032,#21033,#21034,#21035,#21036,#21037,#21038,
#21039),.UNSPECIFIED.,.F.,.F.,(4,3,3,3,3,3,3,3,3,4),(166.50441064026,167.28861080431,
168.072810968359,168.857011132408,169.641211296457,170.425411460506,171.209611624556,
171.993811788605,172.778011952654,172.78759594744),.UNSPECIFIED.);
#545=B_SPLINE_CURVE_WITH_KNOTS('',3,(#21044,#21045,#21046,#21047,#21048,
#21049,#21050,#21051,#21052,#21053,#21054,#21055,#21056,#21057,#21058,#21059,
#21060,#21061,#21062,#21063,#21064,#21065,#21066,#21067,#21068,#21069,#21070,
#21071),.UNSPECIFIED.,.F.,.F.,(4,3,3,3,3,3,3,3,3,4),(160.221225333081,161.00542549713,
161.789625661179,162.573825825228,163.358025989277,164.142226153327,164.926426317376,
165.710626481425,166.494826645474,166.50441064026),.UNSPECIFIED.);
#546=B_SPLINE_CURVE_WITH_KNOTS('',3,(#21072,#21073,#21074,#21075,#21076,
#21077,#21078,#21079,#21080,#21081,#21082,#21083,#21084,#21085,#21086,#21087,
#21088,#21089,#21090,#21091,#21092,#21093,#21094,#21095,#21096,#21097,#21098,
#21099),.UNSPECIFIED.,.F.,.F.,(4,3,3,3,3,3,3,3,3,4),(160.221225333081,161.00542549713,
161.789625661179,162.573825825229,163.358025989278,164.142226153327,164.926426317376,
165.710626481425,166.494826645475,166.50441064026),.UNSPECIFIED.);
#547=B_SPLINE_CURVE_WITH_KNOTS('',3,(#21104,#21105,#21106,#21107,#21108,
#21109,#21110,#21111,#21112,#21113,#21114,#21115,#21116,#21117,#21118,#21119,
#21120,#21121,#21122,#21123,#21124,#21125,#21126,#21127,#21128,#21129,#21130,
#21131),.UNSPECIFIED.,.F.,.F.,(4,3,3,3,3,3,3,3,3,4),(153.938040025901,154.72224018995,
155.506440354,156.290640518049,157.074840682098,157.859040846147,158.643241010196,
159.427441174246,160.211641338295,160.221225333081),.UNSPECIFIED.);
#548=B_SPLINE_CURVE_WITH_KNOTS('',3,(#21132,#21133,#21134,#21135,#21136,
#21137,#21138,#21139,#21140,#21141,#21142,#21143,#21144,#21145,#21146,#21147,
#21148,#21149,#21150,#21151,#21152,#21153,#21154,#21155,#21156,#21157,#21158,
#21159),.UNSPECIFIED.,.F.,.F.,(4,3,3,3,3,3,3,3,3,4),(153.938040025901,154.722240189951,
155.506440354,156.290640518049,157.074840682098,157.859040846147,158.643241010197,
159.427441174246,160.211641338295,160.221225333081),.UNSPECIFIED.);
#549=B_SPLINE_CURVE_WITH_KNOTS('',3,(#21164,#21165,#21166,#21167,#21168,
#21169,#21170,#21171,#21172,#21173,#21174),.UNSPECIFIED.,.F.,.F.,(4,1,1,
1,1,1,1,1,4),(147.654854718722,148.045106901034,148.544850762035,149.544338484036,
150.543826206038,151.543313928039,152.542801650041,153.542289372042,153.938040025901),
 .UNSPECIFIED.);
#550=B_SPLINE_CURVE_WITH_KNOTS('',3,(#21175,#21176,#21177,#21178,#21179,
#21180,#21181,#21182,#21183,#21184,#21185,#21186,#21187,#21188,#21189,#21190,
#21191,#21192,#21193,#21194,#21195,#21196,#21197,#21198,#21199,#21200,#21201,
#21202),.UNSPECIFIED.,.F.,.F.,(4,3,3,3,3,3,3,3,3,4),(147.654854718722,148.439054882771,
149.22325504682,150.007455210869,150.791655374919,151.575855538968,152.360055703017,
153.144255867066,153.928456031116,153.938040025901),.UNSPECIFIED.);
#551=B_SPLINE_CURVE_WITH_KNOTS('',3,(#21207,#21208,#21209,#21210,#21211,
#21212,#21213,#21214,#21215,#21216,#21217,#21218,#21219,#21220,#21221,#21222,
#21223,#21224,#21225,#21226,#21227,#21228,#21229,#21230,#21231,#21232,#21233,
#21234),.UNSPECIFIED.,.F.,.F.,(4,3,3,3,3,3,3,3,3,4),(141.371669411542,142.155869575591,
142.94006973964,143.72426990369,144.508470067739,145.292670231788,146.076870395837,
146.861070559887,147.645270723936,147.654854718722),.UNSPECIFIED.);
#552=B_SPLINE_CURVE_WITH_KNOTS('',3,(#21235,#21236,#21237,#21238,#21239,
#21240,#21241,#21242,#21243,#21244,#21245),.UNSPECIFIED.,.F.,.F.,(4,1,1,
1,1,1,1,1,4),(141.371669411542,142.230670203473,143.230157925475,144.229645647477,
144.729389508477,145.229133369478,146.22862109148,147.228108813481,147.654854718722),
 .UNSPECIFIED.);
#553=B_SPLINE_CURVE_WITH_KNOTS('',3,(#21250,#21251,#21252,#21253,#21254,
#21255,#21256,#21257,#21258,#21259,#21260,#21261,#21262,#21263,#21264,#21265,
#21266,#21267,#21268,#21269,#21270,#21271,#21272,#21273,#21274,#21275,#21276,
#21277),.UNSPECIFIED.,.F.,.F.,(4,3,3,3,3,3,3,3,3,4),(135.088484104362,135.872684268412,
136.656884432461,137.44108459651,138.225284760559,139.009484924609,139.793685088658,
140.577885252707,141.362085416756,141.371669411542),.UNSPECIFIED.);
#554=B_SPLINE_CURVE_WITH_KNOTS('',3,(#21278,#21279,#21280,#21281,#21282,
#21283,#21284,#21285,#21286,#21287,#21288,#21289,#21290,#21291,#21292,#21293,
#21294,#21295,#21296,#21297,#21298,#21299,#21300,#21301,#21302,#21303,#21304,
#21305),.UNSPECIFIED.,.F.,.F.,(4,3,3,3,3,3,3,3,3,4),(135.088484104363,135.872684268412,
136.656884432461,137.44108459651,138.225284760559,139.009484924609,139.793685088658,
140.577885252707,141.362085416756,141.371669411542),.UNSPECIFIED.);
#555=B_SPLINE_CURVE_WITH_KNOTS('',3,(#21310,#21311,#21312,#21313,#21314,
#21315,#21316,#21317,#21318,#21319,#21320,#21321,#21322,#21323,#21324,#21325,
#21326,#21327,#21328,#21329,#21330,#21331,#21332,#21333,#21334,#21335,#21336,
#21337),.UNSPECIFIED.,.F.,.F.,(4,3,3,3,3,3,3,3,3,4),(128.805298797183,129.589498961232,
130.373699125281,131.15789928933,131.94209945338,132.726299617429,133.510499781478,
134.294699945527,135.078900109576,135.088484104362),.UNSPECIFIED.);
#556=B_SPLINE_CURVE_WITH_KNOTS('',3,(#21338,#21339,#21340,#21341,#21342,
#21343,#21344,#21345,#21346,#21347,#21348,#21349,#21350,#21351,#21352,#21353,
#21354,#21355,#21356,#21357,#21358,#21359,#21360,#21361,#21362,#21363,#21364,
#21365),.UNSPECIFIED.,.F.,.F.,(4,3,3,3,3,3,3,3,3,4),(128.805298797183,129.589498961232,
130.373699125281,131.157899289331,131.94209945338,132.726299617429,133.510499781478,
134.294699945527,135.078900109576,135.088484104363),.UNSPECIFIED.);
#557=B_SPLINE_CURVE_WITH_KNOTS('',3,(#21370,#21371,#21372,#21373,#21374,
#21375,#21376,#21377,#21378,#21379,#21380,#21381,#21382,#21383,#21384,#21385,
#21386,#21387,#21388,#21389,#21390,#21391,#21392,#21393,#21394,#21395,#21396,
#21397),.UNSPECIFIED.,.F.,.F.,(4,3,3,3,3,3,3,3,3,4),(122.522113490003,123.306313654053,
124.090513818102,124.874713982151,125.6589141462,126.443114310249,127.227314474299,
128.011514638348,128.795714802397,128.805298797183),.UNSPECIFIED.);
#558=B_SPLINE_CURVE_WITH_KNOTS('',3,(#21398,#21399,#21400,#21401,#21402,
#21403,#21404,#21405,#21406,#21407,#21408,#21409,#21410,#21411,#21412,#21413,
#21414,#21415,#21416,#21417,#21418,#21419,#21420,#21421,#21422,#21423,#21424,
#21425),.UNSPECIFIED.,.F.,.F.,(4,3,3,3,3,3,3,3,3,4),(122.522113490004,123.306313654053,
124.090513818102,124.874713982151,125.6589141462,126.44311431025,127.227314474299,
128.011514638348,128.795714802397,128.805298797183),.UNSPECIFIED.);
#559=B_SPLINE_CURVE_WITH_KNOTS('',3,(#21430,#21431,#21432,#21433,#21434,
#21435,#21436,#21437,#21438,#21439,#21440),.UNSPECIFIED.,.F.,.F.,(4,1,1,
1,1,1,1,1,4),(116.238928182824,116.561243657984,117.560731379986,118.560219101987,
119.559706823989,120.05945068499,120.559194545991,121.558682267992,122.522113490003),
 .UNSPECIFIED.);
#560=B_SPLINE_CURVE_WITH_KNOTS('',3,(#21441,#21442,#21443,#21444,#21445,
#21446,#21447,#21448,#21449,#21450,#21451,#21452,#21453,#21454,#21455,#21456,
#21457,#21458,#21459,#21460,#21461,#21462,#21463,#21464,#21465,#21466,#21467,
#21468),.UNSPECIFIED.,.F.,.F.,(4,3,3,3,3,3,3,3,3,4),(116.238928182824,117.023128346873,
117.807328510922,118.591528674972,119.375728839021,120.15992900307,120.944129167119,
121.728329331169,122.512529495218,122.522113490004),.UNSPECIFIED.);
#561=B_SPLINE_CURVE_WITH_KNOTS('',3,(#21473,#21474,#21475,#21476,#21477,
#21478,#21479,#21480,#21481,#21482,#21483),.UNSPECIFIED.,.F.,.F.,(4,1,1,
1,1,1,1,1,4),(109.955742875644,110.564317325975,111.563805047977,112.563292769978,
113.063036630979,113.56278049198,114.562268213981,115.561755935983,116.238928182824),
 .UNSPECIFIED.);
#562=B_SPLINE_CURVE_WITH_KNOTS('',3,(#21484,#21485,#21486,#21487,#21488,
#21489,#21490,#21491,#21492,#21493,#21494,#21495,#21496,#21497,#21498,#21499,
#21500,#21501,#21502,#21503,#21504,#21505,#21506,#21507,#21508,#21509,#21510,
#21511),.UNSPECIFIED.,.F.,.F.,(4,3,3,3,3,3,3,3,3,4),(109.955742875644,110.739943039694,
111.524143203743,112.308343367792,113.092543531841,113.87674369589,114.66094385994,
115.445144023989,116.229344188038,116.238928182824),.UNSPECIFIED.);
#563=B_SPLINE_CURVE_WITH_KNOTS('',3,(#21516,#21517,#21518,#21519,#21520,
#21521,#21522,#21523,#21524,#21525,#21526,#21527,#21528,#21529,#21530,#21531,
#21532,#21533,#21534,#21535,#21536,#21537,#21538,#21539,#21540,#21541,#21542,
#21543),.UNSPECIFIED.,.F.,.F.,(4,3,3,3,3,3,3,3,3,4),(103.672557568465,104.456757732514,
105.240957896563,106.025158060612,106.809358224661,107.593558388711,108.37775855276,
109.161958716809,109.946158880858,109.955742875644),.UNSPECIFIED.);
#564=B_SPLINE_CURVE_WITH_KNOTS('',3,(#21544,#21545,#21546,#21547,#21548,
#21549,#21550,#21551,#21552,#21553,#21554,#21555,#21556,#21557,#21558,#21559,
#21560,#21561,#21562,#21563,#21564,#21565,#21566,#21567,#21568,#21569,#21570,
#21571),.UNSPECIFIED.,.F.,.F.,(4,3,3,3,3,3,3,3,3,4),(103.672557568465,104.456757732514,
105.240957896563,106.025158060612,106.809358224662,107.593558388711,108.37775855276,
109.161958716809,109.946158880859,109.955742875644),.UNSPECIFIED.);
#565=B_SPLINE_CURVE_WITH_KNOTS('',3,(#21576,#21577,#21578,#21579,#21580,
#21581,#21582,#21583,#21584,#21585,#21586,#21587,#21588,#21589,#21590,#21591,
#21592,#21593,#21594,#21595,#21596,#21597,#21598,#21599,#21600,#21601,#21602,
#21603),.UNSPECIFIED.,.F.,.F.,(4,3,3,3,3,3,3,3,3,4),(97.3893722612849,98.1735724253341,
98.9577725893833,99.7419727534325,100.526172917482,101.310373081531,102.09457324558,
102.878773409629,103.662973573678,103.672557568465),.UNSPECIFIED.);
#566=B_SPLINE_CURVE_WITH_KNOTS('',3,(#21604,#21605,#21606,#21607,#21608,
#21609,#21610,#21611,#21612,#21613,#21614,#21615,#21616,#21617,#21618,#21619,
#21620,#21621,#21622,#21623,#21624,#21625,#21626,#21627,#21628,#21629,#21630,
#21631),.UNSPECIFIED.,.F.,.F.,(4,3,3,3,3,3,3,3,3,4),(97.3893722612851,98.1735724253344,
98.9577725893836,99.7419727534328,100.526172917482,101.310373081531,102.09457324558,
102.87877340963,103.662973573679,103.672557568465),.UNSPECIFIED.);
#567=B_SPLINE_CURVE_WITH_KNOTS('',3,(#21636,#21637,#21638,#21639,#21640,
#21641,#21642,#21643,#21644,#21645,#21646,#21647,#21648,#21649,#21650,#21651,
#21652,#21653,#21654,#21655,#21656,#21657,#21658,#21659,#21660,#21661,#21662,
#21663),.UNSPECIFIED.,.F.,.F.,(4,3,3,3,3,3,3,3,3,4),(91.1061869541053,91.8903871181545,
92.6745872822037,93.458787446253,94.2429876103022,95.0271877743514,95.8113879384006,
96.5955881024498,97.379788266499,97.3893722612849),.UNSPECIFIED.);
#568=B_SPLINE_CURVE_WITH_KNOTS('',3,(#21664,#21665,#21666,#21667,#21668,
#21669,#21670,#21671,#21672,#21673,#21674,#21675,#21676,#21677,#21678,#21679,
#21680,#21681,#21682,#21683,#21684,#21685,#21686,#21687,#21688,#21689,#21690,
#21691),.UNSPECIFIED.,.F.,.F.,(4,3,3,3,3,3,3,3,3,4),(91.1061869541056,91.8903871181548,
92.674587282204,93.4587874462532,94.2429876103025,95.0271877743517,95.8113879384009,
96.5955881024501,97.3797882664994,97.3893722612851),.UNSPECIFIED.);
#569=B_SPLINE_CURVE_WITH_KNOTS('',3,(#21696,#21697,#21698,#21699,#21700,
#21701,#21702,#21703,#21704,#21705,#21706,#21707,#21708,#21709,#21710,#21711,
#21712,#21713,#21714,#21715,#21716,#21717,#21718,#21719,#21720,#21721,#21722,
#21723),.UNSPECIFIED.,.F.,.F.,(4,3,3,3,3,3,3,3,3,4),(84.8230016469257,85.6072018109749,
86.3914019750241,87.1756021390733,87.9598023031225,88.7440024671717,89.5282026312209,
90.3124027952701,91.0966029593193,91.1061869541053),.UNSPECIFIED.);
#570=B_SPLINE_CURVE_WITH_KNOTS('',3,(#21724,#21725,#21726,#21727,#21728,
#21729,#21730,#21731,#21732,#21733,#21734,#21735,#21736,#21737,#21738,#21739,
#21740,#21741,#21742,#21743,#21744,#21745,#21746,#21747,#21748,#21749,#21750,
#21751),.UNSPECIFIED.,.F.,.F.,(4,3,3,3,3,3,3,3,3,4),(84.823001646926,85.6072018109752,
86.3914019750244,87.1756021390736,87.9598023031228,88.744002467172,89.5282026312212,
90.3124027952704,91.0966029593196,91.1061869541056),.UNSPECIFIED.);
#571=B_SPLINE_CURVE_WITH_KNOTS('',3,(#21756,#21757,#21758,#21759,#21760,
#21761,#21762,#21763,#21764,#21765,#21766,#21767,#21768,#21769,#21770,#21771,
#21772,#21773,#21774,#21775,#21776,#21777,#21778,#21779,#21780,#21781,#21782,
#21783),.UNSPECIFIED.,.F.,.F.,(4,3,3,3,3,3,3,3,3,4),(78.5398163397462,79.3240165037953,
80.1082166678445,80.8924168318937,81.6766169959429,82.4608171599921,83.2450173240413,
84.0292174880905,84.8134176521397,84.8230016469257),.UNSPECIFIED.);
#572=B_SPLINE_CURVE_WITH_KNOTS('',3,(#21784,#21785,#21786,#21787,#21788,
#21789,#21790,#21791,#21792,#21793,#21794),.UNSPECIFIED.,.F.,.F.,(4,1,1,
1,1,1,1,1,4),(78.5398163397464,79.2629437173746,80.2624314393762,81.2619191613777,
81.7616630223785,82.2614068833793,83.2608946053809,84.2603823273824,84.823001646926),
 .UNSPECIFIED.);
#573=B_SPLINE_CURVE_WITH_KNOTS('',3,(#21799,#21800,#21801,#21802,#21803,
#21804,#21805,#21806,#21807,#21808,#21809),.UNSPECIFIED.,.F.,.F.,(4,1,1,
1,1,1,1,1,4),(72.2566310325665,72.5837838899154,73.583271611917,74.5827593339185,
75.5822470559201,76.5817347779217,77.5812224999232,78.080966360924,78.5398163397462),
 .UNSPECIFIED.);
#574=B_SPLINE_CURVE_WITH_KNOTS('',3,(#21810,#21811,#21812,#21813,#21814,
#21815,#21816,#21817,#21818,#21819,#21820,#21821),.UNSPECIFIED.,.F.,.F.,
(4,1,1,1,1,1,1,1,1,4),(72.2566310325668,72.2665296633636,73.2660173853652,
74.2655051073667,74.7652489683675,75.2649928293683,76.2644805513699,77.2639682733715,
78.263455995373,78.5398163397464),.UNSPECIFIED.);
#575=B_SPLINE_CURVE_WITH_KNOTS('',3,(#21826,#21827,#21828,#21829,#21830,
#21831,#21832,#21833,#21834,#21835,#21836,#21837,#21838,#21839,#21840,#21841,
#21842,#21843,#21844,#21845,#21846,#21847,#21848,#21849,#21850,#21851,#21852,
#21853),.UNSPECIFIED.,.F.,.F.,(4,3,3,3,3,3,3,3,3,4),(65.973445725387,66.7576458894362,
67.5418460534854,68.3260462175346,69.1102463815837,69.8944465456329,70.6786467096821,
71.4628468737313,72.2470470377805,72.2566310325665),.UNSPECIFIED.);
#576=B_SPLINE_CURVE_WITH_KNOTS('',3,(#21854,#21855,#21856,#21857,#21858,
#21859,#21860,#21861,#21862,#21863,#21864,#21865,#21866,#21867,#21868,#21869,
#21870,#21871,#21872,#21873,#21874,#21875,#21876,#21877,#21878,#21879,#21880,
#21881),.UNSPECIFIED.,.F.,.F.,(4,3,3,3,3,3,3,3,3,4),(65.9734457253872,66.7576458894364,
67.5418460534856,68.3260462175348,69.110246381584,69.8944465456332,70.6786467096824,
71.4628468737316,72.2470470377808,72.2566310325668),.UNSPECIFIED.);
#577=B_SPLINE_CURVE_WITH_KNOTS('',3,(#21886,#21887,#21888,#21889,#21890,
#21891,#21892,#21893,#21894,#21895,#21896),.UNSPECIFIED.,.F.,.F.,(4,1,1,
1,1,1,1,1,4),(59.6902604182074,60.5899312258966,61.5894189478982,62.5889066698997,
63.5883943919013,64.0881382529021,64.5878821139029,65.5873698359044,65.973445725387),
 .UNSPECIFIED.);
#578=B_SPLINE_CURVE_WITH_KNOTS('',3,(#21897,#21898,#21899,#21900,#21901,
#21902,#21903,#21904,#21905,#21906,#21907,#21908,#21909,#21910,#21911,#21912,
#21913,#21914,#21915,#21916,#21917,#21918,#21919,#21920,#21921,#21922,#21923,
#21924),.UNSPECIFIED.,.F.,.F.,(4,3,3,3,3,3,3,3,3,4),(59.6902604182076,60.4744605822568,
61.258660746306,62.0428609103552,62.8270610744044,63.6112612384536,64.3954614025028,
65.179661566552,65.9638617306012,65.9734457253872),.UNSPECIFIED.);
#579=B_SPLINE_CURVE_WITH_KNOTS('',3,(#21929,#21930,#21931,#21932,#21933,
#21934,#21935,#21936,#21937,#21938,#21939,#21940,#21941,#21942,#21943,#21944,
#21945,#21946,#21947,#21948,#21949,#21950,#21951,#21952,#21953,#21954,#21955,
#21956),.UNSPECIFIED.,.F.,.F.,(4,3,3,3,3,3,3,3,3,4),(53.4070751110278,54.191275275077,
54.9754754391262,55.7596756031754,56.5438757672245,57.3280759312737,58.1122760953229,
58.8964762593721,59.6806764234213,59.6902604182074),.UNSPECIFIED.);
#580=B_SPLINE_CURVE_WITH_KNOTS('',3,(#21957,#21958,#21959,#21960,#21961,
#21962,#21963,#21964,#21965,#21966,#21967),.UNSPECIFIED.,.F.,.F.,(4,1,1,
1,1,1,1,1,4),(53.407075111028,53.7760068063346,54.2757506673354,55.275238389337,
56.2747261113385,57.2742138333401,58.2737015553417,59.2731892773432,59.6902604182076),
 .UNSPECIFIED.);
#581=B_SPLINE_CURVE_WITH_KNOTS('',3,(#21972,#21973,#21974,#21975,#21976,
#21977,#21978,#21979,#21980,#21981,#21982),.UNSPECIFIED.,.F.,.F.,(4,1,1,
1,1,1,1,1,4),(47.1238898038482,47.5965908398762,48.5960785618778,49.5955662838794,
50.0953101448802,50.5950540058809,51.5945417278825,52.5940294498841,53.4070751110278),
 .UNSPECIFIED.);
#582=B_SPLINE_CURVE_WITH_KNOTS('',3,(#21983,#21984,#21985,#21986,#21987,
#21988,#21989,#21990,#21991,#21992,#21993,#21994,#21995,#21996,#21997,#21998,
#21999,#22000,#22001,#22002,#22003,#22004,#22005,#22006,#22007,#22008,#22009,
#22010),.UNSPECIFIED.,.F.,.F.,(4,3,3,3,3,3,3,3,3,4),(47.1238898038484,47.9080899678976,
48.6922901319468,49.4764902959961,50.2606904600453,51.0448906240945,51.8290907881437,
52.6132909521929,53.3974911162422,53.407075111028),.UNSPECIFIED.);
#583=B_SPLINE_CURVE_WITH_KNOTS('',3,(#22015,#22016,#22017,#22018,#22019,
#22020,#22021,#22022,#22023,#22024,#22025,#22026,#22027,#22028,#22029,#22030,
#22031,#22032,#22033,#22034,#22035,#22036,#22037,#22038,#22039,#22040,#22041,
#22042),.UNSPECIFIED.,.F.,.F.,(4,3,3,3,3,3,3,3,3,4),(40.8407044966686,41.6249046607178,
42.409104824767,43.1933049888162,43.9775051528655,44.7617053169147,45.5459054809639,
46.3301056450131,47.1143058090623,47.1238898038482),.UNSPECIFIED.);
#584=B_SPLINE_CURVE_WITH_KNOTS('',3,(#22043,#22044,#22045,#22046,#22047,
#22048,#22049,#22050,#22051,#22052,#22053),.UNSPECIFIED.,.F.,.F.,(4,1,1,
1,1,1,1,1,4),(40.8407044966688,41.282410281315,42.2818980033166,43.2813857253182,
44.2808734473197,45.2803611693213,46.2798488913229,46.7795927523237,47.1238898038484),
 .UNSPECIFIED.);
#585=B_SPLINE_CURVE_WITH_KNOTS('',3,(#22058,#22059,#22060,#22061,#22062,
#22063,#22064,#22065,#22066,#22067,#22068,#22069,#22070,#22071,#22072,#22073,
#22074,#22075,#22076,#22077,#22078,#22079,#22080,#22081,#22082,#22083,#22084,
#22085),.UNSPECIFIED.,.F.,.F.,(4,3,3,3,3,3,3,3,3,4),(34.557519189489,35.3417193535382,
36.1259195175874,36.9101196816366,37.6943198456858,38.478520009735,39.2627201737842,
40.0469203378334,40.8311205018826,40.8407044966686),.UNSPECIFIED.);
#586=B_SPLINE_CURVE_WITH_KNOTS('',3,(#22086,#22087,#22088,#22089,#22090,
#22091,#22092,#22093,#22094,#22095,#22096,#22097,#22098,#22099,#22100,#22101,
#22102,#22103,#22104,#22105,#22106,#22107,#22108,#22109,#22110,#22111,#22112,
#22113),.UNSPECIFIED.,.F.,.F.,(4,3,3,3,3,3,3,3,3,4),(34.5575191894892,35.3417193535384,
36.1259195175876,36.9101196816368,37.694319845686,38.4785200097352,39.2627201737844,
40.0469203378336,40.8311205018828,40.8407044966688),.UNSPECIFIED.);
#587=B_SPLINE_CURVE_WITH_KNOTS('',3,(#22118,#22119,#22120,#22121,#22122,
#22123,#22124,#22125,#22126,#22127,#22128,#22129,#22130,#22131,#22132,#22133,
#22134,#22135,#22136,#22137,#22138,#22139,#22140,#22141,#22142,#22143,#22144,
#22145),.UNSPECIFIED.,.F.,.F.,(4,3,3,3,3,3,3,3,3,4),(28.2743338823094,29.0585340463586,
29.8427342104078,30.6269343744571,31.4111345385063,32.1953347025555,32.9795348666047,
33.7637350306539,34.5479351947031,34.557519189489),.UNSPECIFIED.);
#588=B_SPLINE_CURVE_WITH_KNOTS('',3,(#22146,#22147,#22148,#22149,#22150,
#22151,#22152,#22153,#22154,#22155,#22156,#22157,#22158,#22159,#22160,#22161,
#22162,#22163,#22164,#22165,#22166,#22167,#22168,#22169,#22170,#22171,#22172,
#22173),.UNSPECIFIED.,.F.,.F.,(4,3,3,3,3,3,3,3,3,4),(28.2743338823096,29.0585340463588,
29.842734210408,30.6269343744572,31.4111345385064,32.1953347025557,32.9795348666049,
33.7637350306541,34.5479351947033,34.5575191894892),.UNSPECIFIED.);
#589=B_SPLINE_CURVE_WITH_KNOTS('',3,(#22178,#22179,#22180,#22181,#22182,
#22183,#22184,#22185,#22186,#22187,#22188,#22189,#22190,#22191,#22192,#22193,
#22194,#22195,#22196,#22197,#22198,#22199,#22200,#22201,#22202,#22203,#22204,
#22205),.UNSPECIFIED.,.F.,.F.,(4,3,3,3,3,3,3,3,3,4),(21.9911485751298,22.775348739179,
23.5595489032282,24.3437490672774,25.1279492313266,25.9121493953758,26.696349559425,
27.4805497234742,28.2647498875234,28.2743338823094),.UNSPECIFIED.);
#590=B_SPLINE_CURVE_WITH_KNOTS('',3,(#22206,#22207,#22208,#22209,#22210,
#22211,#22212,#22213,#22214,#22215,#22216),.UNSPECIFIED.,.F.,.F.,(4,1,1,
1,1,1,1,1,4),(21.99114857513,22.2921435632852,23.2916312852868,24.2911190072884,
25.2906067292899,25.7903505902907,26.2900944512915,27.2895821732931,28.2743338823096),
 .UNSPECIFIED.);
#591=B_SPLINE_CURVE_WITH_KNOTS('',3,(#22221,#22222,#22223,#22224,#22225,
#22226,#22227,#22228,#22229,#22230,#22231),.UNSPECIFIED.,.F.,.F.,(4,1,1,
1,1,1,1,1,4),(15.7079632679502,16.1127275968269,16.6124714578277,17.6119591798292,
18.6114469018308,19.6109346238324,20.6104223458339,21.6099100678355,21.9911485751298),
 .UNSPECIFIED.);
#592=B_SPLINE_CURVE_WITH_KNOTS('',3,(#22232,#22233,#22234,#22235,#22236,
#22237,#22238,#22239,#22240,#22241,#22242),.UNSPECIFIED.,.F.,.F.,(4,1,1,
1,1,1,1,1,4),(15.7079632679505,16.2952172312758,17.2947049532774,18.294192675279,
18.7939365362798,19.2936803972805,20.2931681192821,21.2926558412837,21.99114857513),
 .UNSPECIFIED.);
#593=B_SPLINE_CURVE_WITH_KNOTS('',3,(#22283,#22284,#22285,#22286,#22287,
#22288,#22289,#22290,#22291,#22292,#22293,#22294,#22295,#22296),
 .UNSPECIFIED.,.F.,.F.,(4,2,2,2,2,2,4),(0.,0.401864562314507,0.815996863195449,
1.24239114437787,1.68104169475581,1.98676350350074,2.29817876007995),
 .UNSPECIFIED.);
#594=B_SPLINE_CURVE_WITH_KNOTS('',3,(#22298,#22299,#22300,#22301,#22302,
#22303,#22304,#22305,#22306,#22307,#22308,#22309,#22310,#22311,#22312,#22313,
#22314,#22315,#22316,#22317,#22318,#22319,#22320,#22321,#22322,#22323,#22324,
#22325,#22326,#22327,#22328,#22329,#22330,#22331,#22332,#22333,#22334,#22335,
#22336,#22337,#22338,#22339,#22340,#22341,#22342,#22343,#22344,#22345,#22346,
#22347,#22348,#22349,#22350,#22351,#22352,#22353,#22354,#22355,#22356,#22357,
#22358,#22359,#22360,#22361,#22362,#22363,#22364,#22365,#22366,#22367,#22368,
#22369,#22370,#22371,#22372,#22373,#22374,#22375,#22376,#22377,#22378,#22379),
 .UNSPECIFIED.,.F.,.F.,(4,3,3,3,3,3,3,3,3,3,3,3,3,3,3,3,3,3,3,3,3,3,3,3,
3,3,3,4),(0.,0.0926102951683523,0.242481898243462,0.367224141810497,0.42570459697912,
0.455719969557024,0.483685835042882,0.631460986432984,0.783700701519674,
0.853497497696487,0.898154331254642,0.927522777398727,1.07095818631111,
1.21012247382799,1.24041984677974,1.31315875852148,1.35313933924437,1.49322196341175,
1.63841202124878,1.7110070501673,1.74549420777844,1.77435553121022,1.78360207908582,
1.91413601045329,2.0238902612264,2.05537001599445,2.18951620872001,2.3057378045557),
 .UNSPECIFIED.);
#595=B_SPLINE_CURVE_WITH_KNOTS('',3,(#25115,#25116,#25117,#25118,#25119,
#25120,#25121,#25122,#25123,#25124,#25125,#25126,#25127,#25128,#25129,#25130,
#25131,#25132,#25133,#25134,#25135,#25136,#25137,#25138,#25139,#25140,#25141,
#25142,#25143,#25144,#25145,#25146,#25147,#25148,#25149,#25150,#25151,#25152,
#25153,#25154,#25155,#25156,#25157,#25158,#25159,#25160,#25161,#25162,#25163,
#25164,#25165,#25166,#25167,#25168,#25169,#25170,#25171,#25172,#25173,#25174,
#25175,#25176,#25177,#25178,#25179,#25180,#25181,#25182,#25183,#25184,#25185,
#25186,#25187,#25188,#25189,#25190,#25191,#25192,#25193,#25194,#25195,#25196),
 .UNSPECIFIED.,.F.,.F.,(4,3,3,3,3,3,3,3,3,3,3,3,3,3,3,3,3,3,3,3,3,3,3,3,
3,3,3,4),(0.,0.0926102951686331,0.242481898248882,0.367224141815228,0.425704596969164,
0.455719969047205,0.48368583491359,0.631460986269685,0.783700701397176,
0.853497497532231,0.898154330267531,0.92752277734915,1.07095818632606,1.21012247381061,
1.24041984677965,1.31315875851436,1.35313933832513,1.49322196246626,1.63841202077606,
1.71100704993096,1.74549420694238,1.77435553196361,1.78360207908585,1.9141360104532,
2.02389026119983,2.05537001679799,2.18951620952033,2.30573780455522),
 .UNSPECIFIED.);
#596=B_SPLINE_CURVE_WITH_KNOTS('',3,(#25197,#25198,#25199,#25200,#25201,
#25202,#25203,#25204,#25205,#25206,#25207,#25208,#25209,#25210,#25211,#25212,
#25213,#25214,#25215,#25216,#25217,#25218),.UNSPECIFIED.,.F.,.F.,(4,3,3,
3,3,3,3,4),(585.461696073209,585.699805092919,586.69929281492,587.698780536922,
588.198524397923,588.698268258924,589.697755980925,590.619418874881),
 .UNSPECIFIED.);
#597=B_SPLINE_CURVE_WITH_KNOTS('',3,(#25219,#25220,#25221,#25222,#25223,
#25224,#25225,#25226,#25227,#25228),.UNSPECIFIED.,.F.,.F.,(4,1,1,1,1,1,
1,4),(10.3761157273117,11.297778621268,12.2972663432696,12.7970102042703,
13.2967540652711,14.2962417872727,15.2957295092743,15.7079632679505),
 .UNSPECIFIED.);
#598=B_SPLINE_CURVE_WITH_KNOTS('',3,(#25230,#25231,#25232,#25233,#25234,
#25235,#25236,#25237,#25238,#25239,#25240,#25241,#25242,#25243,#25244,#25245,
#25246,#25247,#25248),.UNSPECIFIED.,.F.,.F.,(4,3,3,3,3,3,4),(11.6150328478198,
12.399233011869,13.1834331759182,13.9676333399674,14.7518335040166,15.5360336680658,
15.7079632679502),.UNSPECIFIED.);
#599=B_SPLINE_CURVE_WITH_KNOTS('',3,(#27978,#27979,#27980,#27981,#27982,
#27983,#27984,#27985,#27986,#27987,#27988,#27989,#27990,#27991),
 .UNSPECIFIED.,.F.,.F.,(4,2,2,2,2,2,4),(0.,0.401864562314452,0.815996863195417,
1.2423911443779,1.68104169475587,1.98676350350112,2.29817876008015),
 .UNSPECIFIED.);
#600=B_SPLINE_CURVE_WITH_KNOTS('',3,(#27992,#27993,#27994,#27995,#27996,
#27997,#27998,#27999,#28000,#28001,#28002,#28003,#28004,#28005,#28006,#28007,
#28008,#28009,#28010),.UNSPECIFIED.,.F.,.F.,(4,3,3,3,3,3,4),(-592.696219146929,
-591.94203667819,-591.18785420945,-590.43367174071,-589.67948927197,-588.925306803231,
-588.429163987831),.UNSPECIFIED.);
#698=SHAPE_REPRESENTATION_RELATIONSHIP('SRR','None',#34540,#720);
#720=ADVANCED_BREP_SHAPE_REPRESENTATION('',(#772),#34408);
#742=STYLED_ITEM('',(#34757),#772);
#772=MANIFOLD_SOLID_BREP('Body1',#8769);
#809=FACE_BOUND('',#1750,.T.);
#810=FACE_BOUND('',#1751,.T.);
#811=FACE_BOUND('',#1752,.T.);
#812=FACE_BOUND('',#1753,.T.);
#813=FACE_BOUND('',#1754,.T.);
#814=FACE_BOUND('',#1755,.T.);
#815=FACE_BOUND('',#1756,.T.);
#816=FACE_BOUND('',#1759,.T.);
#817=FACE_BOUND('',#1760,.T.);
#818=FACE_BOUND('',#1761,.T.);
#819=FACE_BOUND('',#1762,.T.);
#820=FACE_BOUND('',#1763,.T.);
#821=FACE_BOUND('',#1764,.T.);
#865=PLANE('',#9281);
#866=PLANE('',#9286);
#867=PLANE('',#9288);
#1058=FACE_OUTER_BOUND('',#1555,.T.);
#1059=FACE_OUTER_BOUND('',#1556,.T.);
#1060=FACE_OUTER_BOUND('',#1557,.T.);
#1061=FACE_OUTER_BOUND('',#1558,.T.);
#1062=FACE_OUTER_BOUND('',#1559,.T.);
#1063=FACE_OUTER_BOUND('',#1560,.T.);
#1064=FACE_OUTER_BOUND('',#1561,.T.);
#1065=FACE_OUTER_BOUND('',#1562,.T.);
#1066=FACE_OUTER_BOUND('',#1563,.T.);
#1067=FACE_OUTER_BOUND('',#1564,.T.);
#1068=FACE_OUTER_BOUND('',#1565,.T.);
#1069=FACE_OUTER_BOUND('',#1566,.T.);
#1070=FACE_OUTER_BOUND('',#1567,.T.);
#1071=FACE_OUTER_BOUND('',#1568,.T.);
#1072=FACE_OUTER_BOUND('',#1569,.T.);
#1073=FACE_OUTER_BOUND('',#1570,.T.);
#1074=FACE_OUTER_BOUND('',#1571,.T.);
#1075=FACE_OUTER_BOUND('',#1572,.T.);
#1076=FACE_OUTER_BOUND('',#1573,.T.);
#1077=FACE_OUTER_BOUND('',#1574,.T.);
#1078=FACE_OUTER_BOUND('',#1575,.T.);
#1079=FACE_OUTER_BOUND('',#1576,.T.);
#1080=FACE_OUTER_BOUND('',#1577,.T.);
#1081=FACE_OUTER_BOUND('',#1578,.T.);
#1082=FACE_OUTER_BOUND('',#1579,.T.);
#1083=FACE_OUTER_BOUND('',#1580,.T.);
#1084=FACE_OUTER_BOUND('',#1581,.T.);
#1085=FACE_OUTER_BOUND('',#1582,.T.);
#1086=FACE_OUTER_BOUND('',#1583,.T.);
#1087=FACE_OUTER_BOUND('',#1584,.T.);
#1088=FACE_OUTER_BOUND('',#1585,.T.);
#1089=FACE_OUTER_BOUND('',#1586,.T.);
#1090=FACE_OUTER_BOUND('',#1587,.T.);
#1091=FACE_OUTER_BOUND('',#1588,.T.);
#1092=FACE_OUTER_BOUND('',#1589,.T.);
#1093=FACE_OUTER_BOUND('',#1590,.T.);
#1094=FACE_OUTER_BOUND('',#1591,.T.);
#1095=FACE_OUTER_BOUND('',#1592,.T.);
#1096=FACE_OUTER_BOUND('',#1593,.T.);
#1097=FACE_OUTER_BOUND('',#1594,.T.);
#1098=FACE_OUTER_BOUND('',#1595,.T.);
#1099=FACE_OUTER_BOUND('',#1596,.T.);
#1100=FACE_OUTER_BOUND('',#1597,.T.);
#1101=FACE_OUTER_BOUND('',#1598,.T.);
#1102=FACE_OUTER_BOUND('',#1599,.T.);
#1103=FACE_OUTER_BOUND('',#1600,.T.);
#1104=FACE_OUTER_BOUND('',#1601,.T.);
#1105=FACE_OUTER_BOUND('',#1602,.T.);
#1106=FACE_OUTER_BOUND('',#1603,.T.);
#1107=FACE_OUTER_BOUND('',#1604,.T.);
#1108=FACE_OUTER_BOUND('',#1605,.T.);
#1109=FACE_OUTER_BOUND('',#1606,.T.);
#1110=FACE_OUTER_BOUND('',#1607,.T.);
#1111=FACE_OUTER_BOUND('',#1608,.T.);
#1112=FACE_OUTER_BOUND('',#1609,.T.);
#1113=FACE_OUTER_BOUND('',#1610,.T.);
#1114=FACE_OUTER_BOUND('',#1611,.T.);
#1115=FACE_OUTER_BOUND('',#1612,.T.);
#1116=FACE_OUTER_BOUND('',#1613,.T.);
#1117=FACE_OUTER_BOUND('',#1614,.T.);
#1118=FACE_OUTER_BOUND('',#1615,.T.);
#1119=FACE_OUTER_BOUND('',#1616,.T.);
#1120=FACE_OUTER_BOUND('',#1617,.T.);
#1121=FACE_OUTER_BOUND('',#1618,.T.);
#1122=FACE_OUTER_BOUND('',#1619,.T.);
#1123=FACE_OUTER_BOUND('',#1620,.T.);
#1124=FACE_OUTER_BOUND('',#1621,.T.);
#1125=FACE_OUTER_BOUND('',#1622,.T.);
#1126=FACE_OUTER_BOUND('',#1623,.T.);
#1127=FACE_OUTER_BOUND('',#1624,.T.);
#1128=FACE_OUTER_BOUND('',#1625,.T.);
#1129=FACE_OUTER_BOUND('',#1626,.T.);
#1130=FACE_OUTER_BOUND('',#1627,.T.);
#1131=FACE_OUTER_BOUND('',#1628,.T.);
#1132=FACE_OUTER_BOUND('',#1629,.T.);
#1133=FACE_OUTER_BOUND('',#1630,.T.);
#1134=FACE_OUTER_BOUND('',#1631,.T.);
#1135=FACE_OUTER_BOUND('',#1632,.T.);
#1136=FACE_OUTER_BOUND('',#1633,.T.);
#1137=FACE_OUTER_BOUND('',#1634,.T.);
#1138=FACE_OUTER_BOUND('',#1635,.T.);
#1139=FACE_OUTER_BOUND('',#1636,.T.);
#1140=FACE_OUTER_BOUND('',#1637,.T.);
#1141=FACE_OUTER_BOUND('',#1638,.T.);
#1142=FACE_OUTER_BOUND('',#1639,.T.);
#1143=FACE_OUTER_BOUND('',#1640,.T.);
#1144=FACE_OUTER_BOUND('',#1641,.T.);
#1145=FACE_OUTER_BOUND('',#1642,.T.);
#1146=FACE_OUTER_BOUND('',#1643,.T.);
#1147=FACE_OUTER_BOUND('',#1644,.T.);
#1148=FACE_OUTER_BOUND('',#1645,.T.);
#1149=FACE_OUTER_BOUND('',#1646,.T.);
#1150=FACE_OUTER_BOUND('',#1647,.T.);
#1151=FACE_OUTER_BOUND('',#1648,.T.);
#1152=FACE_OUTER_BOUND('',#1649,.T.);
#1153=FACE_OUTER_BOUND('',#1650,.T.);
#1154=FACE_OUTER_BOUND('',#1651,.T.);
#1155=FACE_OUTER_BOUND('',#1652,.T.);
#1156=FACE_OUTER_BOUND('',#1653,.T.);
#1157=FACE_OUTER_BOUND('',#1654,.T.);
#1158=FACE_OUTER_BOUND('',#1655,.T.);
#1159=FACE_OUTER_BOUND('',#1656,.T.);
#1160=FACE_OUTER_BOUND('',#1657,.T.);
#1161=FACE_OUTER_BOUND('',#1658,.T.);
#1162=FACE_OUTER_BOUND('',#1659,.T.);
#1163=FACE_OUTER_BOUND('',#1660,.T.);
#1164=FACE_OUTER_BOUND('',#1661,.T.);
#1165=FACE_OUTER_BOUND('',#1662,.T.);
#1166=FACE_OUTER_BOUND('',#1663,.T.);
#1167=FACE_OUTER_BOUND('',#1664,.T.);
#1168=FACE_OUTER_BOUND('',#1665,.T.);
#1169=FACE_OUTER_BOUND('',#1666,.T.);
#1170=FACE_OUTER_BOUND('',#1667,.T.);
#1171=FACE_OUTER_BOUND('',#1668,.T.);
#1172=FACE_OUTER_BOUND('',#1669,.T.);
#1173=FACE_OUTER_BOUND('',#1670,.T.);
#1174=FACE_OUTER_BOUND('',#1671,.T.);
#1175=FACE_OUTER_BOUND('',#1672,.T.);
#1176=FACE_OUTER_BOUND('',#1673,.T.);
#1177=FACE_OUTER_BOUND('',#1674,.T.);
#1178=FACE_OUTER_BOUND('',#1675,.T.);
#1179=FACE_OUTER_BOUND('',#1676,.T.);
#1180=FACE_OUTER_BOUND('',#1677,.T.);
#1181=FACE_OUTER_BOUND('',#1678,.T.);
#1182=FACE_OUTER_BOUND('',#1679,.T.);
#1183=FACE_OUTER_BOUND('',#1680,.T.);
#1184=FACE_OUTER_BOUND('',#1681,.T.);
#1185=FACE_OUTER_BOUND('',#1682,.T.);
#1186=FACE_OUTER_BOUND('',#1683,.T.);
#1187=FACE_OUTER_BOUND('',#1684,.T.);
#1188=FACE_OUTER_BOUND('',#1685,.T.);
#1189=FACE_OUTER_BOUND('',#1686,.T.);
#1190=FACE_OUTER_BOUND('',#1687,.T.);
#1191=FACE_OUTER_BOUND('',#1688,.T.);
#1192=FACE_OUTER_BOUND('',#1689,.T.);
#1193=FACE_OUTER_BOUND('',#1690,.T.);
#1194=FACE_OUTER_BOUND('',#1691,.T.);
#1195=FACE_OUTER_BOUND('',#1692,.T.);
#1196=FACE_OUTER_BOUND('',#1693,.T.);
#1197=FACE_OUTER_BOUND('',#1694,.T.);
#1198=FACE_OUTER_BOUND('',#1695,.T.);
#1199=FACE_OUTER_BOUND('',#1696,.T.);
#1200=FACE_OUTER_BOUND('',#1697,.T.);
#1201=FACE_OUTER_BOUND('',#1698,.T.);
#1202=FACE_OUTER_BOUND('',#1699,.T.);
#1203=FACE_OUTER_BOUND('',#1700,.T.);
#1204=FACE_OUTER_BOUND('',#1701,.T.);
#1205=FACE_OUTER_BOUND('',#1702,.T.);
#1206=FACE_OUTER_BOUND('',#1703,.T.);
#1207=FACE_OUTER_BOUND('',#1704,.T.);
#1208=FACE_OUTER_BOUND('',#1705,.T.);
#1209=FACE_OUTER_BOUND('',#1706,.T.);
#1210=FACE_OUTER_BOUND('',#1707,.T.);
#1211=FACE_OUTER_BOUND('',#1708,.T.);
#1212=FACE_OUTER_BOUND('',#1709,.T.);
#1213=FACE_OUTER_BOUND('',#1710,.T.);
#1214=FACE_OUTER_BOUND('',#1711,.T.);
#1215=FACE_OUTER_BOUND('',#1712,.T.);
#1216=FACE_OUTER_BOUND('',#1713,.T.);
#1217=FACE_OUTER_BOUND('',#1714,.T.);
#1218=FACE_OUTER_BOUND('',#1715,.T.);
#1219=FACE_OUTER_BOUND('',#1716,.T.);
#1220=FACE_OUTER_BOUND('',#1717,.T.);
#1221=FACE_OUTER_BOUND('',#1718,.T.);
#1222=FACE_OUTER_BOUND('',#1719,.T.);
#1223=FACE_OUTER_BOUND('',#1720,.T.);
#1224=FACE_OUTER_BOUND('',#1721,.T.);
#1225=FACE_OUTER_BOUND('',#1722,.T.);
#1226=FACE_OUTER_BOUND('',#1723,.T.);
#1227=FACE_OUTER_BOUND('',#1724,.T.);
#1228=FACE_OUTER_BOUND('',#1725,.T.);
#1229=FACE_OUTER_BOUND('',#1726,.T.);
#1230=FACE_OUTER_BOUND('',#1727,.T.);
#1231=FACE_OUTER_BOUND('',#1728,.T.);
#1232=FACE_OUTER_BOUND('',#1729,.T.);
#1233=FACE_OUTER_BOUND('',#1730,.T.);
#1234=FACE_OUTER_BOUND('',#1731,.T.);
#1235=FACE_OUTER_BOUND('',#1732,.T.);
#1236=FACE_OUTER_BOUND('',#1733,.T.);
#1237=FACE_OUTER_BOUND('',#1734,.T.);
#1238=FACE_OUTER_BOUND('',#1735,.T.);
#1239=FACE_OUTER_BOUND('',#1736,.T.);
#1240=FACE_OUTER_BOUND('',#1737,.T.);
#1241=FACE_OUTER_BOUND('',#1738,.T.);
#1242=FACE_OUTER_BOUND('',#1739,.T.);
#1243=FACE_OUTER_BOUND('',#1740,.T.);
#1244=FACE_OUTER_BOUND('',#1741,.T.);
#1245=FACE_OUTER_BOUND('',#1742,.T.);
#1246=FACE_OUTER_BOUND('',#1743,.T.);
#1247=FACE_OUTER_BOUND('',#1744,.T.);
#1248=FACE_OUTER_BOUND('',#1745,.T.);
#1249=FACE_OUTER_BOUND('',#1746,.T.);
#1250=FACE_OUTER_BOUND('',#1747,.T.);
#1251=FACE_OUTER_BOUND('',#1748,.T.);
#1252=FACE_OUTER_BOUND('',#1749,.T.);
#1253=FACE_OUTER_BOUND('',#1757,.T.);
#1254=FACE_OUTER_BOUND('',#1758,.T.);
#1255=FACE_OUTER_BOUND('',#1765,.T.);
#1256=FACE_OUTER_BOUND('',#1766,.T.);
#1257=FACE_OUTER_BOUND('',#1767,.T.);
#1258=FACE_OUTER_BOUND('',#1768,.T.);
#1259=FACE_OUTER_BOUND('',#1769,.T.);
#1555=EDGE_LOOP('',(#5573,#5574,#5575,#5576));
#1556=EDGE_LOOP('',(#5577,#5578,#5579,#5580));
#1557=EDGE_LOOP('',(#5581,#5582,#5583,#5584));
#1558=EDGE_LOOP('',(#5585,#5586,#5587,#5588));
#1559=EDGE_LOOP('',(#5589,#5590,#5591,#5592));
#1560=EDGE_LOOP('',(#5593,#5594,#5595,#5596));
#1561=EDGE_LOOP('',(#5597,#5598,#5599,#5600));
#1562=EDGE_LOOP('',(#5601,#5602,#5603,#5604));
#1563=EDGE_LOOP('',(#5605,#5606,#5607,#5608));
#1564=EDGE_LOOP('',(#5609,#5610,#5611,#5612));
#1565=EDGE_LOOP('',(#5613,#5614,#5615,#5616));
#1566=EDGE_LOOP('',(#5617,#5618,#5619,#5620));
#1567=EDGE_LOOP('',(#5621,#5622,#5623,#5624));
#1568=EDGE_LOOP('',(#5625,#5626,#5627,#5628));
#1569=EDGE_LOOP('',(#5629,#5630,#5631,#5632));
#1570=EDGE_LOOP('',(#5633,#5634,#5635,#5636));
#1571=EDGE_LOOP('',(#5637,#5638,#5639,#5640));
#1572=EDGE_LOOP('',(#5641,#5642,#5643,#5644));
#1573=EDGE_LOOP('',(#5645,#5646,#5647,#5648));
#1574=EDGE_LOOP('',(#5649,#5650,#5651,#5652));
#1575=EDGE_LOOP('',(#5653,#5654,#5655,#5656));
#1576=EDGE_LOOP('',(#5657,#5658,#5659,#5660));
#1577=EDGE_LOOP('',(#5661,#5662,#5663,#5664));
#1578=EDGE_LOOP('',(#5665,#5666,#5667,#5668));
#1579=EDGE_LOOP('',(#5669,#5670,#5671,#5672));
#1580=EDGE_LOOP('',(#5673,#5674,#5675,#5676));
#1581=EDGE_LOOP('',(#5677,#5678,#5679,#5680));
#1582=EDGE_LOOP('',(#5681,#5682,#5683,#5684));
#1583=EDGE_LOOP('',(#5685,#5686,#5687,#5688));
#1584=EDGE_LOOP('',(#5689,#5690,#5691,#5692));
#1585=EDGE_LOOP('',(#5693,#5694,#5695,#5696));
#1586=EDGE_LOOP('',(#5697,#5698,#5699,#5700));
#1587=EDGE_LOOP('',(#5701,#5702,#5703,#5704));
#1588=EDGE_LOOP('',(#5705,#5706,#5707,#5708));
#1589=EDGE_LOOP('',(#5709,#5710,#5711,#5712));
#1590=EDGE_LOOP('',(#5713,#5714,#5715,#5716));
#1591=EDGE_LOOP('',(#5717,#5718,#5719,#5720));
#1592=EDGE_LOOP('',(#5721,#5722,#5723,#5724));
#1593=EDGE_LOOP('',(#5725,#5726,#5727,#5728));
#1594=EDGE_LOOP('',(#5729,#5730,#5731,#5732));
#1595=EDGE_LOOP('',(#5733,#5734,#5735,#5736));
#1596=EDGE_LOOP('',(#5737,#5738,#5739,#5740));
#1597=EDGE_LOOP('',(#5741,#5742,#5743,#5744));
#1598=EDGE_LOOP('',(#5745,#5746,#5747,#5748));
#1599=EDGE_LOOP('',(#5749,#5750,#5751,#5752));
#1600=EDGE_LOOP('',(#5753,#5754,#5755,#5756));
#1601=EDGE_LOOP('',(#5757,#5758,#5759,#5760));
#1602=EDGE_LOOP('',(#5761,#5762,#5763,#5764));
#1603=EDGE_LOOP('',(#5765,#5766,#5767,#5768));
#1604=EDGE_LOOP('',(#5769,#5770,#5771,#5772));
#1605=EDGE_LOOP('',(#5773,#5774,#5775,#5776));
#1606=EDGE_LOOP('',(#5777,#5778,#5779,#5780));
#1607=EDGE_LOOP('',(#5781,#5782,#5783,#5784));
#1608=EDGE_LOOP('',(#5785,#5786,#5787,#5788));
#1609=EDGE_LOOP('',(#5789,#5790,#5791,#5792));
#1610=EDGE_LOOP('',(#5793,#5794,#5795,#5796));
#1611=EDGE_LOOP('',(#5797,#5798,#5799,#5800));
#1612=EDGE_LOOP('',(#5801,#5802,#5803,#5804));
#1613=EDGE_LOOP('',(#5805,#5806,#5807,#5808));
#1614=EDGE_LOOP('',(#5809,#5810,#5811,#5812));
#1615=EDGE_LOOP('',(#5813,#5814,#5815,#5816));
#1616=EDGE_LOOP('',(#5817,#5818,#5819,#5820));
#1617=EDGE_LOOP('',(#5821,#5822,#5823,#5824));
#1618=EDGE_LOOP('',(#5825,#5826,#5827,#5828));
#1619=EDGE_LOOP('',(#5829,#5830,#5831,#5832));
#1620=EDGE_LOOP('',(#5833,#5834,#5835,#5836));
#1621=EDGE_LOOP('',(#5837,#5838,#5839,#5840));
#1622=EDGE_LOOP('',(#5841,#5842,#5843,#5844));
#1623=EDGE_LOOP('',(#5845,#5846,#5847,#5848));
#1624=EDGE_LOOP('',(#5849,#5850,#5851,#5852));
#1625=EDGE_LOOP('',(#5853,#5854,#5855,#5856));
#1626=EDGE_LOOP('',(#5857,#5858,#5859,#5860));
#1627=EDGE_LOOP('',(#5861,#5862,#5863,#5864));
#1628=EDGE_LOOP('',(#5865,#5866,#5867,#5868));
#1629=EDGE_LOOP('',(#5869,#5870,#5871,#5872));
#1630=EDGE_LOOP('',(#5873,#5874,#5875,#5876));
#1631=EDGE_LOOP('',(#5877,#5878,#5879,#5880));
#1632=EDGE_LOOP('',(#5881,#5882,#5883,#5884));
#1633=EDGE_LOOP('',(#5885,#5886,#5887,#5888));
#1634=EDGE_LOOP('',(#5889,#5890,#5891,#5892));
#1635=EDGE_LOOP('',(#5893,#5894,#5895,#5896));
#1636=EDGE_LOOP('',(#5897,#5898,#5899,#5900));
#1637=EDGE_LOOP('',(#5901,#5902,#5903,#5904));
#1638=EDGE_LOOP('',(#5905,#5906,#5907,#5908));
#1639=EDGE_LOOP('',(#5909,#5910,#5911,#5912));
#1640=EDGE_LOOP('',(#5913,#5914,#5915,#5916));
#1641=EDGE_LOOP('',(#5917,#5918,#5919,#5920));
#1642=EDGE_LOOP('',(#5921,#5922,#5923,#5924));
#1643=EDGE_LOOP('',(#5925,#5926,#5927,#5928));
#1644=EDGE_LOOP('',(#5929,#5930,#5931,#5932));
#1645=EDGE_LOOP('',(#5933,#5934,#5935,#5936));
#1646=EDGE_LOOP('',(#5937,#5938,#5939,#5940));
#1647=EDGE_LOOP('',(#5941,#5942,#5943,#5944));
#1648=EDGE_LOOP('',(#5945,#5946,#5947,#5948));
#1649=EDGE_LOOP('',(#5949,#5950,#5951,#5952));
#1650=EDGE_LOOP('',(#5953,#5954,#5955,#5956));
#1651=EDGE_LOOP('',(#5957,#5958,#5959,#5960));
#1652=EDGE_LOOP('',(#5961,#5962,#5963,#5964));
#1653=EDGE_LOOP('',(#5965,#5966,#5967,#5968));
#1654=EDGE_LOOP('',(#5969,#5970,#5971,#5972));
#1655=EDGE_LOOP('',(#5973,#5974,#5975,#5976));
#1656=EDGE_LOOP('',(#5977,#5978,#5979,#5980));
#1657=EDGE_LOOP('',(#5981,#5982,#5983,#5984));
#1658=EDGE_LOOP('',(#5985,#5986,#5987,#5988));
#1659=EDGE_LOOP('',(#5989,#5990,#5991,#5992));
#1660=EDGE_LOOP('',(#5993,#5994,#5995,#5996));
#1661=EDGE_LOOP('',(#5997,#5998,#5999,#6000));
#1662=EDGE_LOOP('',(#6001,#6002,#6003,#6004));
#1663=EDGE_LOOP('',(#6005,#6006,#6007,#6008));
#1664=EDGE_LOOP('',(#6009,#6010,#6011,#6012));
#1665=EDGE_LOOP('',(#6013,#6014,#6015,#6016));
#1666=EDGE_LOOP('',(#6017,#6018,#6019,#6020));
#1667=EDGE_LOOP('',(#6021,#6022,#6023,#6024));
#1668=EDGE_LOOP('',(#6025,#6026,#6027,#6028));
#1669=EDGE_LOOP('',(#6029,#6030,#6031,#6032));
#1670=EDGE_LOOP('',(#6033,#6034,#6035,#6036));
#1671=EDGE_LOOP('',(#6037,#6038,#6039,#6040));
#1672=EDGE_LOOP('',(#6041,#6042,#6043,#6044));
#1673=EDGE_LOOP('',(#6045,#6046,#6047,#6048));
#1674=EDGE_LOOP('',(#6049,#6050,#6051,#6052));
#1675=EDGE_LOOP('',(#6053,#6054,#6055,#6056));
#1676=EDGE_LOOP('',(#6057,#6058,#6059,#6060));
#1677=EDGE_LOOP('',(#6061,#6062,#6063,#6064));
#1678=EDGE_LOOP('',(#6065,#6066,#6067,#6068));
#1679=EDGE_LOOP('',(#6069,#6070,#6071,#6072));
#1680=EDGE_LOOP('',(#6073,#6074,#6075,#6076));
#1681=EDGE_LOOP('',(#6077,#6078,#6079,#6080));
#1682=EDGE_LOOP('',(#6081,#6082,#6083,#6084));
#1683=EDGE_LOOP('',(#6085,#6086,#6087,#6088));
#1684=EDGE_LOOP('',(#6089,#6090,#6091,#6092));
#1685=EDGE_LOOP('',(#6093,#6094,#6095,#6096));
#1686=EDGE_LOOP('',(#6097,#6098,#6099,#6100));
#1687=EDGE_LOOP('',(#6101,#6102,#6103,#6104));
#1688=EDGE_LOOP('',(#6105,#6106,#6107,#6108));
#1689=EDGE_LOOP('',(#6109,#6110,#6111,#6112));
#1690=EDGE_LOOP('',(#6113,#6114,#6115,#6116));
#1691=EDGE_LOOP('',(#6117,#6118,#6119,#6120));
#1692=EDGE_LOOP('',(#6121,#6122,#6123,#6124));
#1693=EDGE_LOOP('',(#6125,#6126,#6127,#6128));
#1694=EDGE_LOOP('',(#6129,#6130,#6131,#6132));
#1695=EDGE_LOOP('',(#6133,#6134,#6135,#6136));
#1696=EDGE_LOOP('',(#6137,#6138,#6139,#6140));
#1697=EDGE_LOOP('',(#6141,#6142,#6143,#6144));
#1698=EDGE_LOOP('',(#6145,#6146,#6147,#6148));
#1699=EDGE_LOOP('',(#6149,#6150,#6151,#6152));
#1700=EDGE_LOOP('',(#6153,#6154,#6155,#6156));
#1701=EDGE_LOOP('',(#6157,#6158,#6159,#6160));
#1702=EDGE_LOOP('',(#6161,#6162,#6163,#6164));
#1703=EDGE_LOOP('',(#6165,#6166,#6167,#6168));
#1704=EDGE_LOOP('',(#6169,#6170,#6171,#6172));
#1705=EDGE_LOOP('',(#6173,#6174,#6175,#6176));
#1706=EDGE_LOOP('',(#6177,#6178,#6179,#6180));
#1707=EDGE_LOOP('',(#6181,#6182,#6183,#6184));
#1708=EDGE_LOOP('',(#6185,#6186,#6187,#6188));
#1709=EDGE_LOOP('',(#6189,#6190,#6191,#6192));
#1710=EDGE_LOOP('',(#6193,#6194,#6195,#6196));
#1711=EDGE_LOOP('',(#6197,#6198,#6199,#6200));
#1712=EDGE_LOOP('',(#6201,#6202,#6203,#6204));
#1713=EDGE_LOOP('',(#6205,#6206,#6207,#6208));
#1714=EDGE_LOOP('',(#6209,#6210,#6211,#6212));
#1715=EDGE_LOOP('',(#6213,#6214,#6215,#6216));
#1716=EDGE_LOOP('',(#6217,#6218,#6219,#6220));
#1717=EDGE_LOOP('',(#6221,#6222,#6223,#6224));
#1718=EDGE_LOOP('',(#6225,#6226,#6227,#6228));
#1719=EDGE_LOOP('',(#6229,#6230,#6231,#6232));
#1720=EDGE_LOOP('',(#6233,#6234,#6235,#6236));
#1721=EDGE_LOOP('',(#6237,#6238,#6239,#6240));
#1722=EDGE_LOOP('',(#6241,#6242,#6243,#6244));
#1723=EDGE_LOOP('',(#6245,#6246,#6247,#6248));
#1724=EDGE_LOOP('',(#6249,#6250,#6251,#6252));
#1725=EDGE_LOOP('',(#6253,#6254,#6255,#6256));
#1726=EDGE_LOOP('',(#6257,#6258,#6259,#6260));
#1727=EDGE_LOOP('',(#6261,#6262,#6263,#6264));
#1728=EDGE_LOOP('',(#6265,#6266,#6267,#6268));
#1729=EDGE_LOOP('',(#6269,#6270,#6271,#6272));
#1730=EDGE_LOOP('',(#6273,#6274,#6275,#6276));
#1731=EDGE_LOOP('',(#6277,#6278,#6279,#6280));
#1732=EDGE_LOOP('',(#6281,#6282,#6283,#6284));
#1733=EDGE_LOOP('',(#6285,#6286,#6287,#6288));
#1734=EDGE_LOOP('',(#6289,#6290,#6291,#6292));
#1735=EDGE_LOOP('',(#6293,#6294,#6295,#6296));
#1736=EDGE_LOOP('',(#6297,#6298,#6299,#6300));
#1737=EDGE_LOOP('',(#6301,#6302,#6303,#6304));
#1738=EDGE_LOOP('',(#6305,#6306,#6307,#6308));
#1739=EDGE_LOOP('',(#6309,#6310,#6311,#6312));
#1740=EDGE_LOOP('',(#6313,#6314,#6315,#6316));
#1741=EDGE_LOOP('',(#6317,#6318,#6319,#6320));
#1742=EDGE_LOOP('',(#6321,#6322,#6323,#6324));
#1743=EDGE_LOOP('',(#6325,#6326,#6327,#6328));
#1744=EDGE_LOOP('',(#6329,#6330,#6331,#6332));
#1745=EDGE_LOOP('',(#6333,#6334,#6335,#6336));
#1746=EDGE_LOOP('',(#6337,#6338,#6339,#6340));
#1747=EDGE_LOOP('',(#6341,#6342,#6343,#6344));
#1748=EDGE_LOOP('',(#6345,#6346,#6347,#6348));
#1749=EDGE_LOOP('',(#6349));
#1750=EDGE_LOOP('',(#6350));
#1751=EDGE_LOOP('',(#6351));
#1752=EDGE_LOOP('',(#6352,#6353,#6354,#6355));
#1753=EDGE_LOOP('',(#6356));
#1754=EDGE_LOOP('',(#6357));
#1755=EDGE_LOOP('',(#6358));
#1756=EDGE_LOOP('',(#6359));
#1757=EDGE_LOOP('',(#6360,#6361,#6362,#6363));
#1758=EDGE_LOOP('',(#6364));
#1759=EDGE_LOOP('',(#6365));
#1760=EDGE_LOOP('',(#6366));
#1761=EDGE_LOOP('',(#6367));
#1762=EDGE_LOOP('',(#6368));
#1763=EDGE_LOOP('',(#6369));
#1764=EDGE_LOOP('',(#6370));
#1765=EDGE_LOOP('',(#6371,#6372,#6373,#6374,#6375,#6376,#6377,#6378,#6379,
#6380,#6381,#6382,#6383,#6384,#6385,#6386,#6387,#6388,#6389,#6390,#6391,
#6392,#6393,#6394,#6395,#6396,#6397,#6398,#6399,#6400,#6401,#6402,#6403,
#6404,#6405,#6406,#6407,#6408,#6409,#6410,#6411,#6412,#6413,#6414,#6415,
#6416,#6417,#6418,#6419,#6420,#6421,#6422,#6423,#6424,#6425,#6426,#6427,
#6428,#6429,#6430,#6431,#6432,#6433,#6434,#6435,#6436,#6437,#6438,#6439,
#6440,#6441,#6442,#6443,#6444,#6445,#6446,#6447,#6448,#6449,#6450,#6451,
#6452,#6453,#6454,#6455,#6456,#6457,#6458,#6459,#6460,#6461,#6462,#6463,
#6464,#6465,#6466,#6467,#6468,#6469,#6470,#6471,#6472,#6473,#6474,#6475,
#6476,#6477,#6478,#6479,#6480,#6481,#6482,#6483,#6484,#6485,#6486,#6487,
#6488,#6489,#6490,#6491,#6492,#6493,#6494,#6495,#6496,#6497,#6498,#6499,
#6500,#6501,#6502,#6503,#6504,#6505,#6506,#6507,#6508,#6509,#6510,#6511,
#6512,#6513,#6514,#6515,#6516,#6517,#6518,#6519,#6520,#6521,#6522,#6523,
#6524,#6525,#6526,#6527,#6528,#6529,#6530,#6531,#6532,#6533,#6534,#6535,
#6536,#6537,#6538,#6539,#6540,#6541,#6542,#6543,#6544,#6545,#6546,#6547,
#6548,#6549,#6550,#6551,#6552,#6553,#6554,#6555,#6556,#6557,#6558,#6559,
#6560,#6561,#6562));
#1766=EDGE_LOOP('',(#6563,#6564,#6565,#6566));
#1767=EDGE_LOOP('',(#6567,#6568,#6569,#6570,#6571,#6572,#6573,#6574,#6575,
#6576,#6577,#6578,#6579,#6580,#6581,#6582,#6583,#6584,#6585,#6586,#6587,
#6588,#6589,#6590,#6591,#6592,#6593,#6594,#6595,#6596,#6597,#6598,#6599,
#6600,#6601,#6602,#6603,#6604,#6605,#6606,#6607,#6608,#6609,#6610,#6611,
#6612,#6613,#6614,#6615,#6616,#6617,#6618,#6619,#6620,#6621,#6622,#6623,
#6624,#6625,#6626,#6627,#6628,#6629,#6630,#6631,#6632,#6633,#6634,#6635,
#6636,#6637,#6638,#6639,#6640,#6641,#6642,#6643,#6644,#6645,#6646,#6647,
#6648,#6649,#6650,#6651,#6652,#6653,#6654,#6655,#6656,#6657,#6658,#6659,
#6660,#6661,#6662,#6663,#6664,#6665,#6666,#6667,#6668,#6669,#6670,#6671,
#6672,#6673,#6674,#6675,#6676,#6677,#6678,#6679,#6680,#6681,#6682,#6683,
#6684,#6685,#6686,#6687,#6688,#6689,#6690,#6691,#6692,#6693,#6694,#6695,
#6696,#6697,#6698,#6699,#6700,#6701,#6702,#6703,#6704,#6705,#6706,#6707,
#6708,#6709,#6710,#6711,#6712,#6713,#6714,#6715,#6716,#6717,#6718,#6719,
#6720,#6721,#6722,#6723,#6724,#6725,#6726,#6727,#6728,#6729,#6730,#6731,
#6732,#6733,#6734,#6735,#6736,#6737,#6738,#6739,#6740,#6741,#6742,#6743,
#6744,#6745,#6746,#6747,#6748,#6749,#6750,#6751,#6752,#6753,#6754,#6755,
#6756,#6757,#6758));
#1768=EDGE_LOOP('',(#6759,#6760,#6761,#6762));
#1769=EDGE_LOOP('',(#6763,#6764,#6765,#6766));
#2094=LINE('',#11777,#2711);
#2095=LINE('',#11804,#2712);
#2096=LINE('',#11858,#2713);
#2097=LINE('',#11918,#2714);
#2098=LINE('',#11975,#2715);
#2099=LINE('',#12035,#2716);
#2100=LINE('',#12095,#2717);
#2101=LINE('',#12152,#2718);
#2102=LINE('',#12212,#2719);
#2103=LINE('',#12272,#2720);
#2104=LINE('',#12332,#2721);
#2105=LINE('',#12392,#2722);
#2106=LINE('',#12452,#2723);
#2107=LINE('',#12509,#2724);
#2108=LINE('',#12569,#2725);
#2109=LINE('',#12629,#2726);
#2110=LINE('',#12689,#2727);
#2111=LINE('',#12749,#2728);
#2112=LINE('',#12806,#2729);
#2113=LINE('',#12866,#2730);
#2114=LINE('',#12926,#2731);
#2115=LINE('',#12986,#2732);
#2116=LINE('',#13046,#2733);
#2117=LINE('',#13100,#2734);
#2118=LINE('',#13160,#2735);
#2119=LINE('',#13220,#2736);
#2120=LINE('',#13280,#2737);
#2121=LINE('',#13337,#2738);
#2122=LINE('',#13397,#2739);
#2123=LINE('',#13457,#2740);
#2124=LINE('',#13517,#2741);
#2125=LINE('',#13577,#2742);
#2126=LINE('',#13637,#2743);
#2127=LINE('',#13697,#2744);
#2128=LINE('',#13757,#2745);
#2129=LINE('',#13817,#2746);
#2130=LINE('',#13877,#2747);
#2131=LINE('',#13934,#2748);
#2132=LINE('',#13994,#2749);
#2133=LINE('',#14054,#2750);
#2134=LINE('',#14114,#2751);
#2135=LINE('',#14174,#2752);
#2136=LINE('',#14231,#2753);
#2137=LINE('',#14291,#2754);
#2138=LINE('',#14351,#2755);
#2139=LINE('',#14411,#2756);
#2140=LINE('',#14471,#2757);
#2141=LINE('',#14531,#2758);
#2142=LINE('',#14591,#2759);
#2143=LINE('',#14648,#2760);
#2144=LINE('',#14708,#2761);
#2145=LINE('',#14768,#2762);
#2146=LINE('',#14828,#2763);
#2147=LINE('',#14888,#2764);
#2148=LINE('',#14945,#2765);
#2149=LINE('',#15005,#2766);
#2150=LINE('',#15065,#2767);
#2151=LINE('',#15125,#2768);
#2152=LINE('',#15185,#2769);
#2153=LINE('',#15245,#2770);
#2154=LINE('',#15302,#2771);
#2155=LINE('',#15362,#2772);
#2156=LINE('',#15422,#2773);
#2157=LINE('',#15482,#2774);
#2158=LINE('',#15542,#2775);
#2159=LINE('',#15599,#2776);
#2160=LINE('',#15659,#2777);
#2161=LINE('',#15719,#2778);
#2162=LINE('',#15779,#2779);
#2163=LINE('',#15836,#2780);
#2164=LINE('',#15896,#2781);
#2165=LINE('',#15956,#2782);
#2166=LINE('',#16016,#2783);
#2167=LINE('',#16076,#2784);
#2168=LINE('',#16136,#2785);
#2169=LINE('',#16196,#2786);
#2170=LINE('',#16256,#2787);
#2171=LINE('',#16316,#2788);
#2172=LINE('',#16376,#2789);
#2173=LINE('',#16433,#2790);
#2174=LINE('',#16493,#2791);
#2175=LINE('',#16553,#2792);
#2176=LINE('',#16613,#2793);
#2177=LINE('',#16673,#2794);
#2178=LINE('',#16730,#2795);
#2179=LINE('',#16790,#2796);
#2180=LINE('',#16850,#2797);
#2181=LINE('',#16910,#2798);
#2182=LINE('',#16970,#2799);
#2183=LINE('',#17030,#2800);
#2184=LINE('',#17090,#2801);
#2185=LINE('',#17150,#2802);
#2186=LINE('',#17210,#2803);
#2187=LINE('',#17270,#2804);
#2188=LINE('',#17327,#2805);
#2189=LINE('',#17349,#2806);
#2190=LINE('',#17409,#2807);
#2191=LINE('',#17466,#2808);
#2192=LINE('',#17526,#2809);
#2193=LINE('',#17586,#2810);
#2194=LINE('',#17629,#2811);
#2195=LINE('',#17672,#2812);
#2196=LINE('',#17714,#2813);
#2197=LINE('',#17774,#2814);
#2198=LINE('',#17834,#2815);
#2199=LINE('',#17894,#2816);
#2200=LINE('',#17954,#2817);
#2201=LINE('',#17997,#2818);
#2202=LINE('',#18057,#2819);
#2203=LINE('',#18117,#2820);
#2204=LINE('',#18177,#2821);
#2205=LINE('',#18220,#2822);
#2206=LINE('',#18280,#2823);
#2207=LINE('',#18340,#2824);
#2208=LINE('',#18400,#2825);
#2209=LINE('',#18460,#2826);
#2210=LINE('',#18503,#2827);
#2211=LINE('',#18563,#2828);
#2212=LINE('',#18623,#2829);
#2213=LINE('',#18683,#2830);
#2214=LINE('',#18743,#2831);
#2215=LINE('',#18768,#2832);
#2216=LINE('',#18812,#2833);
#2217=LINE('',#18872,#2834);
#2218=LINE('',#18932,#2835);
#2219=LINE('',#18975,#2836);
#2220=LINE('',#19018,#2837);
#2221=LINE('',#19061,#2838);
#2222=LINE('',#19121,#2839);
#2223=LINE('',#19181,#2840);
#2224=LINE('',#19224,#2841);
#2225=LINE('',#19267,#2842);
#2226=LINE('',#19327,#2843);
#2227=LINE('',#19387,#2844);
#2228=LINE('',#19447,#2845);
#2229=LINE('',#19507,#2846);
#2230=LINE('',#19550,#2847);
#2231=LINE('',#19593,#2848);
#2232=LINE('',#19653,#2849);
#2233=LINE('',#19713,#2850);
#2234=LINE('',#19756,#2851);
#2235=LINE('',#19799,#2852);
#2236=LINE('',#19842,#2853);
#2237=LINE('',#19902,#2854);
#2238=LINE('',#19945,#2855);
#2239=LINE('',#20005,#2856);
#2240=LINE('',#20065,#2857);
#2241=LINE('',#20125,#2858);
#2242=LINE('',#20185,#2859);
#2243=LINE('',#20228,#2860);
#2244=LINE('',#20288,#2861);
#2245=LINE('',#20348,#2862);
#2246=LINE('',#20408,#2863);
#2247=LINE('',#20451,#2864);
#2248=LINE('',#20511,#2865);
#2249=LINE('',#20571,#2866);
#2250=LINE('',#20631,#2867);
#2251=LINE('',#20691,#2868);
#2252=LINE('',#20733,#2869);
#2253=LINE('',#20793,#2870);
#2254=LINE('',#20836,#2871);
#2255=LINE('',#20896,#2872);
#2256=LINE('',#20956,#2873);
#2257=LINE('',#20999,#2874);
#2258=LINE('',#21043,#2875);
#2259=LINE('',#21103,#2876);
#2260=LINE('',#21163,#2877);
#2261=LINE('',#21206,#2878);
#2262=LINE('',#21249,#2879);
#2263=LINE('',#21309,#2880);
#2264=LINE('',#21369,#2881);
#2265=LINE('',#21429,#2882);
#2266=LINE('',#21472,#2883);
#2267=LINE('',#21515,#2884);
#2268=LINE('',#21575,#2885);
#2269=LINE('',#21635,#2886);
#2270=LINE('',#21695,#2887);
#2271=LINE('',#21755,#2888);
#2272=LINE('',#21798,#2889);
#2273=LINE('',#21825,#2890);
#2274=LINE('',#21885,#2891);
#2275=LINE('',#21928,#2892);
#2276=LINE('',#21971,#2893);
#2277=LINE('',#22014,#2894);
#2278=LINE('',#22057,#2895);
#2279=LINE('',#22117,#2896);
#2280=LINE('',#22177,#2897);
#2281=LINE('',#22220,#2898);
#2282=LINE('',#22247,#2899);
#2283=LINE('',#22253,#2900);
#2284=LINE('',#22259,#2901);
#2285=LINE('',#22265,#2902);
#2286=LINE('',#22271,#2903);
#2287=LINE('',#22277,#2904);
#2288=LINE('',#22383,#2905);
#2711=VECTOR('',#9805,1.2);
#2712=VECTOR('',#9810,1.2);
#2713=VECTOR('',#9813,1.2);
#2714=VECTOR('',#9816,1.2);
#2715=VECTOR('',#9819,1.2);
#2716=VECTOR('',#9822,1.2);
#2717=VECTOR('',#9825,1.2);
#2718=VECTOR('',#9828,1.2);
#2719=VECTOR('',#9831,1.2);
#2720=VECTOR('',#9834,1.2);
#2721=VECTOR('',#9837,1.2);
#2722=VECTOR('',#9840,1.2);
#2723=VECTOR('',#9843,1.2);
#2724=VECTOR('',#9846,1.2);
#2725=VECTOR('',#9849,1.2);
#2726=VECTOR('',#9852,1.2);
#2727=VECTOR('',#9855,1.2);
#2728=VECTOR('',#9858,1.2);
#2729=VECTOR('',#9861,1.2);
#2730=VECTOR('',#9864,1.2);
#2731=VECTOR('',#9867,1.2);
#2732=VECTOR('',#9870,1.2);
#2733=VECTOR('',#9873,1.2);
#2734=VECTOR('',#9876,1.2);
#2735=VECTOR('',#9879,1.2);
#2736=VECTOR('',#9882,1.2);
#2737=VECTOR('',#9885,1.2);
#2738=VECTOR('',#9888,1.2);
#2739=VECTOR('',#9891,1.2);
#2740=VECTOR('',#9894,1.2);
#2741=VECTOR('',#9897,1.2);
#2742=VECTOR('',#9900,1.2);
#2743=VECTOR('',#9903,1.2);
#2744=VECTOR('',#9906,1.2);
#2745=VECTOR('',#9909,1.2);
#2746=VECTOR('',#9912,1.2);
#2747=VECTOR('',#9915,1.2);
#2748=VECTOR('',#9918,1.2);
#2749=VECTOR('',#9921,1.2);
#2750=VECTOR('',#9924,1.2);
#2751=VECTOR('',#9927,1.2);
#2752=VECTOR('',#9930,1.2);
#2753=VECTOR('',#9933,1.2);
#2754=VECTOR('',#9936,1.2);
#2755=VECTOR('',#9939,1.2);
#2756=VECTOR('',#9942,1.2);
#2757=VECTOR('',#9945,1.2);
#2758=VECTOR('',#9948,1.2);
#2759=VECTOR('',#9951,1.2);
#2760=VECTOR('',#9954,1.2);
#2761=VECTOR('',#9957,1.2);
#2762=VECTOR('',#9960,1.2);
#2763=VECTOR('',#9963,1.2);
#2764=VECTOR('',#9966,1.2);
#2765=VECTOR('',#9969,1.2);
#2766=VECTOR('',#9972,1.2);
#2767=VECTOR('',#9975,1.2);
#2768=VECTOR('',#9978,1.2);
#2769=VECTOR('',#9981,1.2);
#2770=VECTOR('',#9984,1.2);
#2771=VECTOR('',#9987,1.2);
#2772=VECTOR('',#9990,1.2);
#2773=VECTOR('',#9993,1.2);
#2774=VECTOR('',#9996,1.2);
#2775=VECTOR('',#9999,1.2);
#2776=VECTOR('',#10002,1.2);
#2777=VECTOR('',#10005,1.2);
#2778=VECTOR('',#10008,1.2);
#2779=VECTOR('',#10011,1.2);
#2780=VECTOR('',#10014,1.2);
#2781=VECTOR('',#10017,1.2);
#2782=VECTOR('',#10020,1.2);
#2783=VECTOR('',#10023,1.2);
#2784=VECTOR('',#10026,1.2);
#2785=VECTOR('',#10029,1.2);
#2786=VECTOR('',#10032,1.2);
#2787=VECTOR('',#10035,1.2);
#2788=VECTOR('',#10038,1.2);
#2789=VECTOR('',#10041,1.2);
#2790=VECTOR('',#10044,1.2);
#2791=VECTOR('',#10047,1.2);
#2792=VECTOR('',#10050,1.2);
#2793=VECTOR('',#10053,1.2);
#2794=VECTOR('',#10056,1.2);
#2795=VECTOR('',#10059,1.2);
#2796=VECTOR('',#10062,1.2);
#2797=VECTOR('',#10065,1.2);
#2798=VECTOR('',#10068,1.2);
#2799=VECTOR('',#10071,1.2);
#2800=VECTOR('',#10074,1.2);
#2801=VECTOR('',#10077,1.2);
#2802=VECTOR('',#10080,1.2);
#2803=VECTOR('',#10083,1.2);
#2804=VECTOR('',#10086,1.2);
#2805=VECTOR('',#10089,1.016475);
#2806=VECTOR('',#10094,1.016475);
#2807=VECTOR('',#10097,1.016475);
#2808=VECTOR('',#10100,1.016475);
#2809=VECTOR('',#10103,1.016475);
#2810=VECTOR('',#10106,1.016475);
#2811=VECTOR('',#10109,1.016475);
#2812=VECTOR('',#10112,1.016475);
#2813=VECTOR('',#10115,1.016475);
#2814=VECTOR('',#10118,1.016475);
#2815=VECTOR('',#10121,1.016475);
#2816=VECTOR('',#10124,1.016475);
#2817=VECTOR('',#10127,1.016475);
#2818=VECTOR('',#10130,1.016475);
#2819=VECTOR('',#10133,1.016475);
#2820=VECTOR('',#10136,1.016475);
#2821=VECTOR('',#10139,1.016475);
#2822=VECTOR('',#10142,1.016475);
#2823=VECTOR('',#10145,1.016475);
#2824=VECTOR('',#10148,1.016475);
#2825=VECTOR('',#10151,1.016475);
#2826=VECTOR('',#10154,1.016475);
#2827=VECTOR('',#10157,1.016475);
#2828=VECTOR('',#10160,1.016475);
#2829=VECTOR('',#10163,1.016475);
#2830=VECTOR('',#10166,1.016475);
#2831=VECTOR('',#10169,1.016475);
#2832=VECTOR('',#10172,1.016475);
#2833=VECTOR('',#10175,1.016475);
#2834=VECTOR('',#10178,1.016475);
#2835=VECTOR('',#10181,1.016475);
#2836=VECTOR('',#10184,1.016475);
#2837=VECTOR('',#10187,1.016475);
#2838=VECTOR('',#10190,1.016475);
#2839=VECTOR('',#10193,1.016475);
#2840=VECTOR('',#10196,1.016475);
#2841=VECTOR('',#10199,1.016475);
#2842=VECTOR('',#10202,1.016475);
#2843=VECTOR('',#10205,1.016475);
#2844=VECTOR('',#10208,1.016475);
#2845=VECTOR('',#10211,1.016475);
#2846=VECTOR('',#10214,1.016475);
#2847=VECTOR('',#10217,1.016475);
#2848=VECTOR('',#10220,1.016475);
#2849=VECTOR('',#10223,1.016475);
#2850=VECTOR('',#10226,1.016475);
#2851=VECTOR('',#10229,1.016475);
#2852=VECTOR('',#10232,1.016475);
#2853=VECTOR('',#10235,1.016475);
#2854=VECTOR('',#10238,1.016475);
#2855=VECTOR('',#10241,1.016475);
#2856=VECTOR('',#10244,1.016475);
#2857=VECTOR('',#10247,1.016475);
#2858=VECTOR('',#10250,1.016475);
#2859=VECTOR('',#10253,1.016475);
#2860=VECTOR('',#10256,1.016475);
#2861=VECTOR('',#10259,1.016475);
#2862=VECTOR('',#10262,1.016475);
#2863=VECTOR('',#10265,1.016475);
#2864=VECTOR('',#10268,1.016475);
#2865=VECTOR('',#10271,1.016475);
#2866=VECTOR('',#10274,1.016475);
#2867=VECTOR('',#10277,1.016475);
#2868=VECTOR('',#10280,1.016475);
#2869=VECTOR('',#10283,1.016475);
#2870=VECTOR('',#10286,1.016475);
#2871=VECTOR('',#10289,1.016475);
#2872=VECTOR('',#10292,1.016475);
#2873=VECTOR('',#10295,1.016475);
#2874=VECTOR('',#10298,1.016475);
#2875=VECTOR('',#10301,1.016475);
#2876=VECTOR('',#10304,1.016475);
#2877=VECTOR('',#10307,1.016475);
#2878=VECTOR('',#10310,1.016475);
#2879=VECTOR('',#10313,1.016475);
#2880=VECTOR('',#10316,1.016475);
#2881=VECTOR('',#10319,1.016475);
#2882=VECTOR('',#10322,1.016475);
#2883=VECTOR('',#10325,1.016475);
#2884=VECTOR('',#10328,1.016475);
#2885=VECTOR('',#10331,1.016475);
#2886=VECTOR('',#10334,1.016475);
#2887=VECTOR('',#10337,1.016475);
#2888=VECTOR('',#10340,1.016475);
#2889=VECTOR('',#10343,1.016475);
#2890=VECTOR('',#10346,1.016475);
#2891=VECTOR('',#10349,1.016475);
#2892=VECTOR('',#10352,1.016475);
#2893=VECTOR('',#10355,1.016475);
#2894=VECTOR('',#10358,1.016475);
#2895=VECTOR('',#10361,1.016475);
#2896=VECTOR('',#10364,1.016475);
#2897=VECTOR('',#10367,1.016475);
#2898=VECTOR('',#10370,1.016475);
#2899=VECTOR('',#10375,0.15);
#2900=VECTOR('',#10382,0.15);
#2901=VECTOR('',#10389,0.33);
#2902=VECTOR('',#10396,0.33);
#2903=VECTOR('',#10403,0.33);
#2904=VECTOR('',#10410,0.33);
#2905=VECTOR('',#10421,3.8);
#3322=CIRCLE('',#9074,1.188225);
#3323=CIRCLE('',#9169,1.016475);
#3324=CIRCLE('',#9264,0.15);
#3325=CIRCLE('',#9265,0.15);
#3326=CIRCLE('',#9267,0.15);
#3327=CIRCLE('',#9268,0.15);
#3328=CIRCLE('',#9270,0.33);
#3329=CIRCLE('',#9271,0.33);
#3330=CIRCLE('',#9273,0.33);
#3331=CIRCLE('',#9274,0.33);
#3332=CIRCLE('',#9276,0.33);
#3333=CIRCLE('',#9277,0.33);
#3334=CIRCLE('',#9279,0.33);
#3335=CIRCLE('',#9280,0.33);
#3336=CIRCLE('',#9282,3.8);
#3337=CIRCLE('',#9283,1.016475);
#3338=CIRCLE('',#9285,3.8);
#3339=CIRCLE('',#9289,1.188225);
#3464=VERTEX_POINT('',#11775);
#3465=VERTEX_POINT('',#11776);
#3466=VERTEX_POINT('',#11778);
#3467=VERTEX_POINT('',#11789);
#3468=VERTEX_POINT('',#11802);
#3469=VERTEX_POINT('',#11803);
#3470=VERTEX_POINT('',#11856);
#3471=VERTEX_POINT('',#11857);
#3472=VERTEX_POINT('',#11916);
#3473=VERTEX_POINT('',#11917);
#3474=VERTEX_POINT('',#11973);
#3475=VERTEX_POINT('',#11974);
#3476=VERTEX_POINT('',#12033);
#3477=VERTEX_POINT('',#12034);
#3478=VERTEX_POINT('',#12093);
#3479=VERTEX_POINT('',#12094);
#3480=VERTEX_POINT('',#12150);
#3481=VERTEX_POINT('',#12151);
#3482=VERTEX_POINT('',#12210);
#3483=VERTEX_POINT('',#12211);
#3484=VERTEX_POINT('',#12270);
#3485=VERTEX_POINT('',#12271);
#3486=VERTEX_POINT('',#12330);
#3487=VERTEX_POINT('',#12331);
#3488=VERTEX_POINT('',#12390);
#3489=VERTEX_POINT('',#12391);
#3490=VERTEX_POINT('',#12450);
#3491=VERTEX_POINT('',#12451);
#3492=VERTEX_POINT('',#12507);
#3493=VERTEX_POINT('',#12508);
#3494=VERTEX_POINT('',#12567);
#3495=VERTEX_POINT('',#12568);
#3496=VERTEX_POINT('',#12627);
#3497=VERTEX_POINT('',#12628);
#3498=VERTEX_POINT('',#12687);
#3499=VERTEX_POINT('',#12688);
#3500=VERTEX_POINT('',#12747);
#3501=VERTEX_POINT('',#12748);
#3502=VERTEX_POINT('',#12804);
#3503=VERTEX_POINT('',#12805);
#3504=VERTEX_POINT('',#12864);
#3505=VERTEX_POINT('',#12865);
#3506=VERTEX_POINT('',#12924);
#3507=VERTEX_POINT('',#12925);
#3508=VERTEX_POINT('',#12984);
#3509=VERTEX_POINT('',#12985);
#3510=VERTEX_POINT('',#13044);
#3511=VERTEX_POINT('',#13045);
#3512=VERTEX_POINT('',#13098);
#3513=VERTEX_POINT('',#13099);
#3514=VERTEX_POINT('',#13158);
#3515=VERTEX_POINT('',#13159);
#3516=VERTEX_POINT('',#13218);
#3517=VERTEX_POINT('',#13219);
#3518=VERTEX_POINT('',#13278);
#3519=VERTEX_POINT('',#13279);
#3520=VERTEX_POINT('',#13335);
#3521=VERTEX_POINT('',#13336);
#3522=VERTEX_POINT('',#13395);
#3523=VERTEX_POINT('',#13396);
#3524=VERTEX_POINT('',#13455);
#3525=VERTEX_POINT('',#13456);
#3526=VERTEX_POINT('',#13515);
#3527=VERTEX_POINT('',#13516);
#3528=VERTEX_POINT('',#13575);
#3529=VERTEX_POINT('',#13576);
#3530=VERTEX_POINT('',#13635);
#3531=VERTEX_POINT('',#13636);
#3532=VERTEX_POINT('',#13695);
#3533=VERTEX_POINT('',#13696);
#3534=VERTEX_POINT('',#13755);
#3535=VERTEX_POINT('',#13756);
#3536=VERTEX_POINT('',#13815);
#3537=VERTEX_POINT('',#13816);
#3538=VERTEX_POINT('',#13875);
#3539=VERTEX_POINT('',#13876);
#3540=VERTEX_POINT('',#13932);
#3541=VERTEX_POINT('',#13933);
#3542=VERTEX_POINT('',#13992);
#3543=VERTEX_POINT('',#13993);
#3544=VERTEX_POINT('',#14052);
#3545=VERTEX_POINT('',#14053);
#3546=VERTEX_POINT('',#14112);
#3547=VERTEX_POINT('',#14113);
#3548=VERTEX_POINT('',#14172);
#3549=VERTEX_POINT('',#14173);
#3550=VERTEX_POINT('',#14229);
#3551=VERTEX_POINT('',#14230);
#3552=VERTEX_POINT('',#14289);
#3553=VERTEX_POINT('',#14290);
#3554=VERTEX_POINT('',#14349);
#3555=VERTEX_POINT('',#14350);
#3556=VERTEX_POINT('',#14409);
#3557=VERTEX_POINT('',#14410);
#3558=VERTEX_POINT('',#14469);
#3559=VERTEX_POINT('',#14470);
#3560=VERTEX_POINT('',#14529);
#3561=VERTEX_POINT('',#14530);
#3562=VERTEX_POINT('',#14589);
#3563=VERTEX_POINT('',#14590);
#3564=VERTEX_POINT('',#14646);
#3565=VERTEX_POINT('',#14647);
#3566=VERTEX_POINT('',#14706);
#3567=VERTEX_POINT('',#14707);
#3568=VERTEX_POINT('',#14766);
#3569=VERTEX_POINT('',#14767);
#3570=VERTEX_POINT('',#14826);
#3571=VERTEX_POINT('',#14827);
#3572=VERTEX_POINT('',#14886);
#3573=VERTEX_POINT('',#14887);
#3574=VERTEX_POINT('',#14943);
#3575=VERTEX_POINT('',#14944);
#3576=VERTEX_POINT('',#15003);
#3577=VERTEX_POINT('',#15004);
#3578=VERTEX_POINT('',#15063);
#3579=VERTEX_POINT('',#15064);
#3580=VERTEX_POINT('',#15123);
#3581=VERTEX_POINT('',#15124);
#3582=VERTEX_POINT('',#15183);
#3583=VERTEX_POINT('',#15184);
#3584=VERTEX_POINT('',#15243);
#3585=VERTEX_POINT('',#15244);
#3586=VERTEX_POINT('',#15300);
#3587=VERTEX_POINT('',#15301);
#3588=VERTEX_POINT('',#15360);
#3589=VERTEX_POINT('',#15361);
#3590=VERTEX_POINT('',#15420);
#3591=VERTEX_POINT('',#15421);
#3592=VERTEX_POINT('',#15480);
#3593=VERTEX_POINT('',#15481);
#3594=VERTEX_POINT('',#15540);
#3595=VERTEX_POINT('',#15541);
#3596=VERTEX_POINT('',#15597);
#3597=VERTEX_POINT('',#15598);
#3598=VERTEX_POINT('',#15657);
#3599=VERTEX_POINT('',#15658);
#3600=VERTEX_POINT('',#15717);
#3601=VERTEX_POINT('',#15718);
#3602=VERTEX_POINT('',#15777);
#3603=VERTEX_POINT('',#15778);
#3604=VERTEX_POINT('',#15834);
#3605=VERTEX_POINT('',#15835);
#3606=VERTEX_POINT('',#15894);
#3607=VERTEX_POINT('',#15895);
#3608=VERTEX_POINT('',#15954);
#3609=VERTEX_POINT('',#15955);
#3610=VERTEX_POINT('',#16014);
#3611=VERTEX_POINT('',#16015);
#3612=VERTEX_POINT('',#16074);
#3613=VERTEX_POINT('',#16075);
#3614=VERTEX_POINT('',#16134);
#3615=VERTEX_POINT('',#16135);
#3616=VERTEX_POINT('',#16194);
#3617=VERTEX_POINT('',#16195);
#3618=VERTEX_POINT('',#16254);
#3619=VERTEX_POINT('',#16255);
#3620=VERTEX_POINT('',#16314);
#3621=VERTEX_POINT('',#16315);
#3622=VERTEX_POINT('',#16374);
#3623=VERTEX_POINT('',#16375);
#3624=VERTEX_POINT('',#16431);
#3625=VERTEX_POINT('',#16432);
#3626=VERTEX_POINT('',#16491);
#3627=VERTEX_POINT('',#16492);
#3628=VERTEX_POINT('',#16551);
#3629=VERTEX_POINT('',#16552);
#3630=VERTEX_POINT('',#16611);
#3631=VERTEX_POINT('',#16612);
#3632=VERTEX_POINT('',#16671);
#3633=VERTEX_POINT('',#16672);
#3634=VERTEX_POINT('',#16728);
#3635=VERTEX_POINT('',#16729);
#3636=VERTEX_POINT('',#16788);
#3637=VERTEX_POINT('',#16789);
#3638=VERTEX_POINT('',#16848);
#3639=VERTEX_POINT('',#16849);
#3640=VERTEX_POINT('',#16908);
#3641=VERTEX_POINT('',#16909);
#3642=VERTEX_POINT('',#16968);
#3643=VERTEX_POINT('',#16969);
#3644=VERTEX_POINT('',#17028);
#3645=VERTEX_POINT('',#17029);
#3646=VERTEX_POINT('',#17088);
#3647=VERTEX_POINT('',#17089);
#3648=VERTEX_POINT('',#17148);
#3649=VERTEX_POINT('',#17149);
#3650=VERTEX_POINT('',#17208);
#3651=VERTEX_POINT('',#17209);
#3652=VERTEX_POINT('',#17268);
#3653=VERTEX_POINT('',#17269);
#3654=VERTEX_POINT('',#17325);
#3655=VERTEX_POINT('',#17326);
#3656=VERTEX_POINT('',#17328);
#3657=VERTEX_POINT('',#17339);
#3658=VERTEX_POINT('',#17347);
#3659=VERTEX_POINT('',#17348);
#3660=VERTEX_POINT('',#17407);
#3661=VERTEX_POINT('',#17408);
#3662=VERTEX_POINT('',#17464);
#3663=VERTEX_POINT('',#17465);
#3664=VERTEX_POINT('',#17524);
#3665=VERTEX_POINT('',#17525);
#3666=VERTEX_POINT('',#17584);
#3667=VERTEX_POINT('',#17585);
#3668=VERTEX_POINT('',#17627);
#3669=VERTEX_POINT('',#17628);
#3670=VERTEX_POINT('',#17670);
#3671=VERTEX_POINT('',#17671);
#3672=VERTEX_POINT('',#17712);
#3673=VERTEX_POINT('',#17713);
#3674=VERTEX_POINT('',#17772);
#3675=VERTEX_POINT('',#17773);
#3676=VERTEX_POINT('',#17832);
#3677=VERTEX_POINT('',#17833);
#3678=VERTEX_POINT('',#17892);
#3679=VERTEX_POINT('',#17893);
#3680=VERTEX_POINT('',#17952);
#3681=VERTEX_POINT('',#17953);
#3682=VERTEX_POINT('',#17995);
#3683=VERTEX_POINT('',#17996);
#3684=VERTEX_POINT('',#18055);
#3685=VERTEX_POINT('',#18056);
#3686=VERTEX_POINT('',#18115);
#3687=VERTEX_POINT('',#18116);
#3688=VERTEX_POINT('',#18175);
#3689=VERTEX_POINT('',#18176);
#3690=VERTEX_POINT('',#18218);
#3691=VERTEX_POINT('',#18219);
#3692=VERTEX_POINT('',#18278);
#3693=VERTEX_POINT('',#18279);
#3694=VERTEX_POINT('',#18338);
#3695=VERTEX_POINT('',#18339);
#3696=VERTEX_POINT('',#18398);
#3697=VERTEX_POINT('',#18399);
#3698=VERTEX_POINT('',#18458);
#3699=VERTEX_POINT('',#18459);
#3700=VERTEX_POINT('',#18501);
#3701=VERTEX_POINT('',#18502);
#3702=VERTEX_POINT('',#18561);
#3703=VERTEX_POINT('',#18562);
#3704=VERTEX_POINT('',#18621);
#3705=VERTEX_POINT('',#18622);
#3706=VERTEX_POINT('',#18681);
#3707=VERTEX_POINT('',#18682);
#3708=VERTEX_POINT('',#18741);
#3709=VERTEX_POINT('',#18742);
#3710=VERTEX_POINT('',#18766);
#3711=VERTEX_POINT('',#18767);
#3712=VERTEX_POINT('',#18810);
#3713=VERTEX_POINT('',#18811);
#3714=VERTEX_POINT('',#18870);
#3715=VERTEX_POINT('',#18871);
#3716=VERTEX_POINT('',#18930);
#3717=VERTEX_POINT('',#18931);
#3718=VERTEX_POINT('',#18973);
#3719=VERTEX_POINT('',#18974);
#3720=VERTEX_POINT('',#19016);
#3721=VERTEX_POINT('',#19017);
#3722=VERTEX_POINT('',#19059);
#3723=VERTEX_POINT('',#19060);
#3724=VERTEX_POINT('',#19119);
#3725=VERTEX_POINT('',#19120);
#3726=VERTEX_POINT('',#19179);
#3727=VERTEX_POINT('',#19180);
#3728=VERTEX_POINT('',#19222);
#3729=VERTEX_POINT('',#19223);
#3730=VERTEX_POINT('',#19265);
#3731=VERTEX_POINT('',#19266);
#3732=VERTEX_POINT('',#19325);
#3733=VERTEX_POINT('',#19326);
#3734=VERTEX_POINT('',#19385);
#3735=VERTEX_POINT('',#19386);
#3736=VERTEX_POINT('',#19445);
#3737=VERTEX_POINT('',#19446);
#3738=VERTEX_POINT('',#19505);
#3739=VERTEX_POINT('',#19506);
#3740=VERTEX_POINT('',#19548);
#3741=VERTEX_POINT('',#19549);
#3742=VERTEX_POINT('',#19591);
#3743=VERTEX_POINT('',#19592);
#3744=VERTEX_POINT('',#19651);
#3745=VERTEX_POINT('',#19652);
#3746=VERTEX_POINT('',#19711);
#3747=VERTEX_POINT('',#19712);
#3748=VERTEX_POINT('',#19754);
#3749=VERTEX_POINT('',#19755);
#3750=VERTEX_POINT('',#19797);
#3751=VERTEX_POINT('',#19798);
#3752=VERTEX_POINT('',#19840);
#3753=VERTEX_POINT('',#19841);
#3754=VERTEX_POINT('',#19900);
#3755=VERTEX_POINT('',#19901);
#3756=VERTEX_POINT('',#19943);
#3757=VERTEX_POINT('',#19944);
#3758=VERTEX_POINT('',#20003);
#3759=VERTEX_POINT('',#20004);
#3760=VERTEX_POINT('',#20063);
#3761=VERTEX_POINT('',#20064);
#3762=VERTEX_POINT('',#20123);
#3763=VERTEX_POINT('',#20124);
#3764=VERTEX_POINT('',#20183);
#3765=VERTEX_POINT('',#20184);
#3766=VERTEX_POINT('',#20226);
#3767=VERTEX_POINT('',#20227);
#3768=VERTEX_POINT('',#20286);
#3769=VERTEX_POINT('',#20287);
#3770=VERTEX_POINT('',#20346);
#3771=VERTEX_POINT('',#20347);
#3772=VERTEX_POINT('',#20406);
#3773=VERTEX_POINT('',#20407);
#3774=VERTEX_POINT('',#20449);
#3775=VERTEX_POINT('',#20450);
#3776=VERTEX_POINT('',#20509);
#3777=VERTEX_POINT('',#20510);
#3778=VERTEX_POINT('',#20569);
#3779=VERTEX_POINT('',#20570);
#3780=VERTEX_POINT('',#20629);
#3781=VERTEX_POINT('',#20630);
#3782=VERTEX_POINT('',#20689);
#3783=VERTEX_POINT('',#20690);
#3784=VERTEX_POINT('',#20731);
#3785=VERTEX_POINT('',#20732);
#3786=VERTEX_POINT('',#20791);
#3787=VERTEX_POINT('',#20792);
#3788=VERTEX_POINT('',#20834);
#3789=VERTEX_POINT('',#20835);
#3790=VERTEX_POINT('',#20894);
#3791=VERTEX_POINT('',#20895);
#3792=VERTEX_POINT('',#20954);
#3793=VERTEX_POINT('',#20955);
#3794=VERTEX_POINT('',#20997);
#3795=VERTEX_POINT('',#20998);
#3796=VERTEX_POINT('',#21041);
#3797=VERTEX_POINT('',#21042);
#3798=VERTEX_POINT('',#21101);
#3799=VERTEX_POINT('',#21102);
#3800=VERTEX_POINT('',#21161);
#3801=VERTEX_POINT('',#21162);
#3802=VERTEX_POINT('',#21204);
#3803=VERTEX_POINT('',#21205);
#3804=VERTEX_POINT('',#21247);
#3805=VERTEX_POINT('',#21248);
#3806=VERTEX_POINT('',#21307);
#3807=VERTEX_POINT('',#21308);
#3808=VERTEX_POINT('',#21367);
#3809=VERTEX_POINT('',#21368);
#3810=VERTEX_POINT('',#21427);
#3811=VERTEX_POINT('',#21428);
#3812=VERTEX_POINT('',#21470);
#3813=VERTEX_POINT('',#21471);
#3814=VERTEX_POINT('',#21513);
#3815=VERTEX_POINT('',#21514);
#3816=VERTEX_POINT('',#21573);
#3817=VERTEX_POINT('',#21574);
#3818=VERTEX_POINT('',#21633);
#3819=VERTEX_POINT('',#21634);
#3820=VERTEX_POINT('',#21693);
#3821=VERTEX_POINT('',#21694);
#3822=VERTEX_POINT('',#21753);
#3823=VERTEX_POINT('',#21754);
#3824=VERTEX_POINT('',#21796);
#3825=VERTEX_POINT('',#21797);
#3826=VERTEX_POINT('',#21823);
#3827=VERTEX_POINT('',#21824);
#3828=VERTEX_POINT('',#21883);
#3829=VERTEX_POINT('',#21884);
#3830=VERTEX_POINT('',#21926);
#3831=VERTEX_POINT('',#21927);
#3832=VERTEX_POINT('',#21969);
#3833=VERTEX_POINT('',#21970);
#3834=VERTEX_POINT('',#22012);
#3835=VERTEX_POINT('',#22013);
#3836=VERTEX_POINT('',#22055);
#3837=VERTEX_POINT('',#22056);
#3838=VERTEX_POINT('',#22115);
#3839=VERTEX_POINT('',#22116);
#3840=VERTEX_POINT('',#22175);
#3841=VERTEX_POINT('',#22176);
#3842=VERTEX_POINT('',#22218);
#3843=VERTEX_POINT('',#22219);
#3844=VERTEX_POINT('',#22244);
#3845=VERTEX_POINT('',#22246);
#3846=VERTEX_POINT('',#22250);
#3847=VERTEX_POINT('',#22252);
#3848=VERTEX_POINT('',#22256);
#3849=VERTEX_POINT('',#22258);
#3850=VERTEX_POINT('',#22262);
#3851=VERTEX_POINT('',#22264);
#3852=VERTEX_POINT('',#22268);
#3853=VERTEX_POINT('',#22270);
#3854=VERTEX_POINT('',#22274);
#3855=VERTEX_POINT('',#22276);
#3856=VERTEX_POINT('',#22280);
#3857=VERTEX_POINT('',#22282);
#3858=VERTEX_POINT('',#22297);
#3859=VERTEX_POINT('',#22382);
#3860=VERTEX_POINT('',#25114);
#3861=VERTEX_POINT('',#27977);
#4300=EDGE_CURVE('',#3464,#3465,#2094,.T.);
#4301=EDGE_CURVE('',#3464,#3466,#217,.T.);
#4302=EDGE_CURVE('',#3466,#3467,#3322,.F.);
#4303=EDGE_CURVE('',#3467,#3465,#218,.T.);
#4304=EDGE_CURVE('',#3468,#3469,#2095,.T.);
#4305=EDGE_CURVE('',#3468,#3464,#219,.T.);
#4306=EDGE_CURVE('',#3465,#3469,#220,.T.);
#4307=EDGE_CURVE('',#3470,#3471,#2096,.T.);
#4308=EDGE_CURVE('',#3470,#3468,#221,.T.);
#4309=EDGE_CURVE('',#3469,#3471,#222,.T.);
#4310=EDGE_CURVE('',#3472,#3473,#2097,.T.);
#4311=EDGE_CURVE('',#3472,#3470,#223,.T.);
#4312=EDGE_CURVE('',#3471,#3473,#224,.T.);
#4313=EDGE_CURVE('',#3474,#3475,#2098,.T.);
#4314=EDGE_CURVE('',#3474,#3472,#225,.T.);
#4315=EDGE_CURVE('',#3473,#3475,#226,.T.);
#4316=EDGE_CURVE('',#3476,#3477,#2099,.T.);
#4317=EDGE_CURVE('',#3476,#3474,#227,.T.);
#4318=EDGE_CURVE('',#3475,#3477,#228,.T.);
#4319=EDGE_CURVE('',#3478,#3479,#2100,.T.);
#4320=EDGE_CURVE('',#3478,#3476,#229,.T.);
#4321=EDGE_CURVE('',#3477,#3479,#230,.T.);
#4322=EDGE_CURVE('',#3480,#3481,#2101,.T.);
#4323=EDGE_CURVE('',#3480,#3478,#231,.T.);
#4324=EDGE_CURVE('',#3479,#3481,#232,.T.);
#4325=EDGE_CURVE('',#3482,#3483,#2102,.T.);
#4326=EDGE_CURVE('',#3482,#3480,#233,.T.);
#4327=EDGE_CURVE('',#3481,#3483,#234,.T.);
#4328=EDGE_CURVE('',#3484,#3485,#2103,.T.);
#4329=EDGE_CURVE('',#3484,#3482,#235,.T.);
#4330=EDGE_CURVE('',#3483,#3485,#236,.T.);
#4331=EDGE_CURVE('',#3486,#3487,#2104,.T.);
#4332=EDGE_CURVE('',#3486,#3484,#237,.T.);
#4333=EDGE_CURVE('',#3485,#3487,#238,.T.);
#4334=EDGE_CURVE('',#3488,#3489,#2105,.T.);
#4335=EDGE_CURVE('',#3488,#3486,#239,.T.);
#4336=EDGE_CURVE('',#3487,#3489,#240,.T.);
#4337=EDGE_CURVE('',#3490,#3491,#2106,.T.);
#4338=EDGE_CURVE('',#3490,#3488,#241,.T.);
#4339=EDGE_CURVE('',#3489,#3491,#242,.T.);
#4340=EDGE_CURVE('',#3492,#3493,#2107,.T.);
#4341=EDGE_CURVE('',#3492,#3490,#243,.T.);
#4342=EDGE_CURVE('',#3491,#3493,#244,.T.);
#4343=EDGE_CURVE('',#3494,#3495,#2108,.T.);
#4344=EDGE_CURVE('',#3494,#3492,#245,.T.);
#4345=EDGE_CURVE('',#3493,#3495,#246,.T.);
#4346=EDGE_CURVE('',#3496,#3497,#2109,.T.);
#4347=EDGE_CURVE('',#3496,#3494,#247,.T.);
#4348=EDGE_CURVE('',#3495,#3497,#248,.T.);
#4349=EDGE_CURVE('',#3498,#3499,#2110,.T.);
#4350=EDGE_CURVE('',#3498,#3496,#249,.T.);
#4351=EDGE_CURVE('',#3497,#3499,#250,.T.);
#4352=EDGE_CURVE('',#3500,#3501,#2111,.T.);
#4353=EDGE_CURVE('',#3500,#3498,#251,.T.);
#4354=EDGE_CURVE('',#3499,#3501,#252,.T.);
#4355=EDGE_CURVE('',#3502,#3503,#2112,.T.);
#4356=EDGE_CURVE('',#3502,#3500,#253,.T.);
#4357=EDGE_CURVE('',#3501,#3503,#254,.T.);
#4358=EDGE_CURVE('',#3504,#3505,#2113,.T.);
#4359=EDGE_CURVE('',#3504,#3502,#255,.T.);
#4360=EDGE_CURVE('',#3503,#3505,#256,.T.);
#4361=EDGE_CURVE('',#3506,#3507,#2114,.T.);
#4362=EDGE_CURVE('',#3506,#3504,#257,.T.);
#4363=EDGE_CURVE('',#3505,#3507,#258,.T.);
#4364=EDGE_CURVE('',#3508,#3509,#2115,.T.);
#4365=EDGE_CURVE('',#3508,#3506,#259,.T.);
#4366=EDGE_CURVE('',#3507,#3509,#260,.T.);
#4367=EDGE_CURVE('',#3510,#3511,#2116,.T.);
#4368=EDGE_CURVE('',#3510,#3508,#261,.T.);
#4369=EDGE_CURVE('',#3509,#3511,#262,.T.);
#4370=EDGE_CURVE('',#3512,#3513,#2117,.T.);
#4371=EDGE_CURVE('',#3512,#3510,#263,.T.);
#4372=EDGE_CURVE('',#3511,#3513,#264,.T.);
#4373=EDGE_CURVE('',#3514,#3515,#2118,.T.);
#4374=EDGE_CURVE('',#3514,#3512,#265,.T.);
#4375=EDGE_CURVE('',#3513,#3515,#266,.T.);
#4376=EDGE_CURVE('',#3516,#3517,#2119,.T.);
#4377=EDGE_CURVE('',#3516,#3514,#267,.T.);
#4378=EDGE_CURVE('',#3515,#3517,#268,.T.);
#4379=EDGE_CURVE('',#3518,#3519,#2120,.T.);
#4380=EDGE_CURVE('',#3518,#3516,#269,.T.);
#4381=EDGE_CURVE('',#3517,#3519,#270,.T.);
#4382=EDGE_CURVE('',#3520,#3521,#2121,.T.);
#4383=EDGE_CURVE('',#3520,#3518,#271,.T.);
#4384=EDGE_CURVE('',#3519,#3521,#272,.T.);
#4385=EDGE_CURVE('',#3522,#3523,#2122,.T.);
#4386=EDGE_CURVE('',#3522,#3520,#273,.T.);
#4387=EDGE_CURVE('',#3521,#3523,#274,.T.);
#4388=EDGE_CURVE('',#3524,#3525,#2123,.T.);
#4389=EDGE_CURVE('',#3524,#3522,#275,.T.);
#4390=EDGE_CURVE('',#3523,#3525,#276,.T.);
#4391=EDGE_CURVE('',#3526,#3527,#2124,.T.);
#4392=EDGE_CURVE('',#3526,#3524,#277,.T.);
#4393=EDGE_CURVE('',#3525,#3527,#278,.T.);
#4394=EDGE_CURVE('',#3528,#3529,#2125,.T.);
#4395=EDGE_CURVE('',#3528,#3526,#279,.T.);
#4396=EDGE_CURVE('',#3527,#3529,#280,.T.);
#4397=EDGE_CURVE('',#3530,#3531,#2126,.T.);
#4398=EDGE_CURVE('',#3530,#3528,#281,.T.);
#4399=EDGE_CURVE('',#3529,#3531,#282,.T.);
#4400=EDGE_CURVE('',#3532,#3533,#2127,.T.);
#4401=EDGE_CURVE('',#3532,#3530,#283,.T.);
#4402=EDGE_CURVE('',#3531,#3533,#284,.T.);
#4403=EDGE_CURVE('',#3534,#3535,#2128,.T.);
#4404=EDGE_CURVE('',#3534,#3532,#285,.T.);
#4405=EDGE_CURVE('',#3533,#3535,#286,.T.);
#4406=EDGE_CURVE('',#3536,#3537,#2129,.T.);
#4407=EDGE_CURVE('',#3536,#3534,#287,.T.);
#4408=EDGE_CURVE('',#3535,#3537,#288,.T.);
#4409=EDGE_CURVE('',#3538,#3539,#2130,.T.);
#4410=EDGE_CURVE('',#3538,#3536,#289,.T.);
#4411=EDGE_CURVE('',#3537,#3539,#290,.T.);
#4412=EDGE_CURVE('',#3540,#3541,#2131,.T.);
#4413=EDGE_CURVE('',#3540,#3538,#291,.T.);
#4414=EDGE_CURVE('',#3539,#3541,#292,.T.);
#4415=EDGE_CURVE('',#3542,#3543,#2132,.T.);
#4416=EDGE_CURVE('',#3542,#3540,#293,.T.);
#4417=EDGE_CURVE('',#3541,#3543,#294,.T.);
#4418=EDGE_CURVE('',#3544,#3545,#2133,.T.);
#4419=EDGE_CURVE('',#3544,#3542,#295,.T.);
#4420=EDGE_CURVE('',#3543,#3545,#296,.T.);
#4421=EDGE_CURVE('',#3546,#3547,#2134,.T.);
#4422=EDGE_CURVE('',#3546,#3544,#297,.T.);
#4423=EDGE_CURVE('',#3545,#3547,#298,.T.);
#4424=EDGE_CURVE('',#3548,#3549,#2135,.T.);
#4425=EDGE_CURVE('',#3548,#3546,#299,.T.);
#4426=EDGE_CURVE('',#3547,#3549,#300,.T.);
#4427=EDGE_CURVE('',#3550,#3551,#2136,.T.);
#4428=EDGE_CURVE('',#3550,#3548,#301,.T.);
#4429=EDGE_CURVE('',#3549,#3551,#302,.T.);
#4430=EDGE_CURVE('',#3552,#3553,#2137,.T.);
#4431=EDGE_CURVE('',#3552,#3550,#303,.T.);
#4432=EDGE_CURVE('',#3551,#3553,#304,.T.);
#4433=EDGE_CURVE('',#3554,#3555,#2138,.T.);
#4434=EDGE_CURVE('',#3554,#3552,#305,.T.);
#4435=EDGE_CURVE('',#3553,#3555,#306,.T.);
#4436=EDGE_CURVE('',#3556,#3557,#2139,.T.);
#4437=EDGE_CURVE('',#3556,#3554,#307,.T.);
#4438=EDGE_CURVE('',#3555,#3557,#308,.T.);
#4439=EDGE_CURVE('',#3558,#3559,#2140,.T.);
#4440=EDGE_CURVE('',#3558,#3556,#309,.T.);
#4441=EDGE_CURVE('',#3557,#3559,#310,.T.);
#4442=EDGE_CURVE('',#3560,#3561,#2141,.T.);
#4443=EDGE_CURVE('',#3560,#3558,#311,.T.);
#4444=EDGE_CURVE('',#3559,#3561,#312,.T.);
#4445=EDGE_CURVE('',#3562,#3563,#2142,.T.);
#4446=EDGE_CURVE('',#3562,#3560,#313,.T.);
#4447=EDGE_CURVE('',#3561,#3563,#314,.T.);
#4448=EDGE_CURVE('',#3564,#3565,#2143,.T.);
#4449=EDGE_CURVE('',#3564,#3562,#315,.T.);
#4450=EDGE_CURVE('',#3563,#3565,#316,.T.);
#4451=EDGE_CURVE('',#3566,#3567,#2144,.T.);
#4452=EDGE_CURVE('',#3566,#3564,#317,.T.);
#4453=EDGE_CURVE('',#3565,#3567,#318,.T.);
#4454=EDGE_CURVE('',#3568,#3569,#2145,.T.);
#4455=EDGE_CURVE('',#3568,#3566,#319,.T.);
#4456=EDGE_CURVE('',#3567,#3569,#320,.T.);
#4457=EDGE_CURVE('',#3570,#3571,#2146,.T.);
#4458=EDGE_CURVE('',#3570,#3568,#321,.T.);
#4459=EDGE_CURVE('',#3569,#3571,#322,.T.);
#4460=EDGE_CURVE('',#3572,#3573,#2147,.T.);
#4461=EDGE_CURVE('',#3572,#3570,#323,.T.);
#4462=EDGE_CURVE('',#3571,#3573,#324,.T.);
#4463=EDGE_CURVE('',#3574,#3575,#2148,.T.);
#4464=EDGE_CURVE('',#3574,#3572,#325,.T.);
#4465=EDGE_CURVE('',#3573,#3575,#326,.T.);
#4466=EDGE_CURVE('',#3576,#3577,#2149,.T.);
#4467=EDGE_CURVE('',#3576,#3574,#327,.T.);
#4468=EDGE_CURVE('',#3575,#3577,#328,.T.);
#4469=EDGE_CURVE('',#3578,#3579,#2150,.T.);
#4470=EDGE_CURVE('',#3578,#3576,#329,.T.);
#4471=EDGE_CURVE('',#3577,#3579,#330,.T.);
#4472=EDGE_CURVE('',#3580,#3581,#2151,.T.);
#4473=EDGE_CURVE('',#3580,#3578,#331,.T.);
#4474=EDGE_CURVE('',#3579,#3581,#332,.T.);
#4475=EDGE_CURVE('',#3582,#3583,#2152,.T.);
#4476=EDGE_CURVE('',#3582,#3580,#333,.T.);
#4477=EDGE_CURVE('',#3581,#3583,#334,.T.);
#4478=EDGE_CURVE('',#3584,#3585,#2153,.T.);
#4479=EDGE_CURVE('',#3584,#3582,#335,.T.);
#4480=EDGE_CURVE('',#3583,#3585,#336,.T.);
#4481=EDGE_CURVE('',#3586,#3587,#2154,.T.);
#4482=EDGE_CURVE('',#3586,#3584,#337,.T.);
#4483=EDGE_CURVE('',#3585,#3587,#338,.T.);
#4484=EDGE_CURVE('',#3588,#3589,#2155,.T.);
#4485=EDGE_CURVE('',#3588,#3586,#339,.T.);
#4486=EDGE_CURVE('',#3587,#3589,#340,.T.);
#4487=EDGE_CURVE('',#3590,#3591,#2156,.T.);
#4488=EDGE_CURVE('',#3590,#3588,#341,.T.);
#4489=EDGE_CURVE('',#3589,#3591,#342,.T.);
#4490=EDGE_CURVE('',#3592,#3593,#2157,.T.);
#4491=EDGE_CURVE('',#3592,#3590,#343,.T.);
#4492=EDGE_CURVE('',#3591,#3593,#344,.T.);
#4493=EDGE_CURVE('',#3594,#3595,#2158,.T.);
#4494=EDGE_CURVE('',#3594,#3592,#345,.T.);
#4495=EDGE_CURVE('',#3593,#3595,#346,.T.);
#4496=EDGE_CURVE('',#3596,#3597,#2159,.T.);
#4497=EDGE_CURVE('',#3596,#3594,#347,.T.);
#4498=EDGE_CURVE('',#3595,#3597,#348,.T.);
#4499=EDGE_CURVE('',#3598,#3599,#2160,.T.);
#4500=EDGE_CURVE('',#3598,#3596,#349,.T.);
#4501=EDGE_CURVE('',#3597,#3599,#350,.T.);
#4502=EDGE_CURVE('',#3600,#3601,#2161,.T.);
#4503=EDGE_CURVE('',#3600,#3598,#351,.T.);
#4504=EDGE_CURVE('',#3599,#3601,#352,.T.);
#4505=EDGE_CURVE('',#3602,#3603,#2162,.T.);
#4506=EDGE_CURVE('',#3602,#3600,#353,.T.);
#4507=EDGE_CURVE('',#3601,#3603,#354,.T.);
#4508=EDGE_CURVE('',#3604,#3605,#2163,.T.);
#4509=EDGE_CURVE('',#3604,#3602,#355,.T.);
#4510=EDGE_CURVE('',#3603,#3605,#356,.T.);
#4511=EDGE_CURVE('',#3606,#3607,#2164,.T.);
#4512=EDGE_CURVE('',#3606,#3604,#357,.T.);
#4513=EDGE_CURVE('',#3605,#3607,#358,.T.);
#4514=EDGE_CURVE('',#3608,#3609,#2165,.T.);
#4515=EDGE_CURVE('',#3608,#3606,#359,.T.);
#4516=EDGE_CURVE('',#3607,#3609,#360,.T.);
#4517=EDGE_CURVE('',#3610,#3611,#2166,.T.);
#4518=EDGE_CURVE('',#3610,#3608,#361,.T.);
#4519=EDGE_CURVE('',#3609,#3611,#362,.T.);
#4520=EDGE_CURVE('',#3612,#3613,#2167,.T.);
#4521=EDGE_CURVE('',#3612,#3610,#363,.T.);
#4522=EDGE_CURVE('',#3611,#3613,#364,.T.);
#4523=EDGE_CURVE('',#3614,#3615,#2168,.T.);
#4524=EDGE_CURVE('',#3614,#3612,#365,.T.);
#4525=EDGE_CURVE('',#3613,#3615,#366,.T.);
#4526=EDGE_CURVE('',#3616,#3617,#2169,.T.);
#4527=EDGE_CURVE('',#3616,#3614,#367,.T.);
#4528=EDGE_CURVE('',#3615,#3617,#368,.T.);
#4529=EDGE_CURVE('',#3618,#3619,#2170,.T.);
#4530=EDGE_CURVE('',#3618,#3616,#369,.T.);
#4531=EDGE_CURVE('',#3617,#3619,#370,.T.);
#4532=EDGE_CURVE('',#3620,#3621,#2171,.T.);
#4533=EDGE_CURVE('',#3620,#3618,#371,.T.);
#4534=EDGE_CURVE('',#3619,#3621,#372,.T.);
#4535=EDGE_CURVE('',#3622,#3623,#2172,.T.);
#4536=EDGE_CURVE('',#3622,#3620,#373,.T.);
#4537=EDGE_CURVE('',#3621,#3623,#374,.T.);
#4538=EDGE_CURVE('',#3624,#3625,#2173,.T.);
#4539=EDGE_CURVE('',#3624,#3622,#375,.T.);
#4540=EDGE_CURVE('',#3623,#3625,#376,.T.);
#4541=EDGE_CURVE('',#3626,#3627,#2174,.T.);
#4542=EDGE_CURVE('',#3626,#3624,#377,.T.);
#4543=EDGE_CURVE('',#3625,#3627,#378,.T.);
#4544=EDGE_CURVE('',#3628,#3629,#2175,.T.);
#4545=EDGE_CURVE('',#3628,#3626,#379,.T.);
#4546=EDGE_CURVE('',#3627,#3629,#380,.T.);
#4547=EDGE_CURVE('',#3630,#3631,#2176,.T.);
#4548=EDGE_CURVE('',#3630,#3628,#381,.T.);
#4549=EDGE_CURVE('',#3629,#3631,#382,.T.);
#4550=EDGE_CURVE('',#3632,#3633,#2177,.T.);
#4551=EDGE_CURVE('',#3632,#3630,#383,.T.);
#4552=EDGE_CURVE('',#3631,#3633,#384,.T.);
#4553=EDGE_CURVE('',#3634,#3635,#2178,.T.);
#4554=EDGE_CURVE('',#3634,#3632,#385,.T.);
#4555=EDGE_CURVE('',#3633,#3635,#386,.T.);
#4556=EDGE_CURVE('',#3636,#3637,#2179,.T.);
#4557=EDGE_CURVE('',#3636,#3634,#387,.T.);
#4558=EDGE_CURVE('',#3635,#3637,#388,.T.);
#4559=EDGE_CURVE('',#3638,#3639,#2180,.T.);
#4560=EDGE_CURVE('',#3638,#3636,#389,.T.);
#4561=EDGE_CURVE('',#3637,#3639,#390,.T.);
#4562=EDGE_CURVE('',#3640,#3641,#2181,.T.);
#4563=EDGE_CURVE('',#3640,#3638,#391,.T.);
#4564=EDGE_CURVE('',#3639,#3641,#392,.T.);
#4565=EDGE_CURVE('',#3642,#3643,#2182,.T.);
#4566=EDGE_CURVE('',#3642,#3640,#393,.T.);
#4567=EDGE_CURVE('',#3641,#3643,#394,.T.);
#4568=EDGE_CURVE('',#3644,#3645,#2183,.T.);
#4569=EDGE_CURVE('',#3644,#3642,#395,.T.);
#4570=EDGE_CURVE('',#3643,#3645,#396,.T.);
#4571=EDGE_CURVE('',#3646,#3647,#2184,.T.);
#4572=EDGE_CURVE('',#3646,#3644,#397,.T.);
#4573=EDGE_CURVE('',#3645,#3647,#398,.T.);
#4574=EDGE_CURVE('',#3648,#3649,#2185,.T.);
#4575=EDGE_CURVE('',#3648,#3646,#399,.T.);
#4576=EDGE_CURVE('',#3647,#3649,#400,.T.);
#4577=EDGE_CURVE('',#3650,#3651,#2186,.T.);
#4578=EDGE_CURVE('',#3650,#3648,#401,.T.);
#4579=EDGE_CURVE('',#3649,#3651,#402,.T.);
#4580=EDGE_CURVE('',#3652,#3653,#2187,.T.);
#4581=EDGE_CURVE('',#3652,#3650,#403,.T.);
#4582=EDGE_CURVE('',#3651,#3653,#404,.T.);
#4583=EDGE_CURVE('',#3654,#3655,#2188,.T.);
#4584=EDGE_CURVE('',#3654,#3656,#405,.T.);
#4585=EDGE_CURVE('',#3657,#3656,#3323,.T.);
#4586=EDGE_CURVE('',#3655,#3657,#406,.T.);
#4587=EDGE_CURVE('',#3658,#3659,#2189,.T.);
#4588=EDGE_CURVE('',#3658,#3654,#407,.T.);
#4589=EDGE_CURVE('',#3659,#3655,#408,.T.);
#4590=EDGE_CURVE('',#3660,#3661,#2190,.T.);
#4591=EDGE_CURVE('',#3660,#3658,#409,.T.);
#4592=EDGE_CURVE('',#3661,#3659,#410,.T.);
#4593=EDGE_CURVE('',#3662,#3663,#2191,.T.);
#4594=EDGE_CURVE('',#3662,#3660,#411,.T.);
#4595=EDGE_CURVE('',#3663,#3661,#412,.T.);
#4596=EDGE_CURVE('',#3664,#3665,#2192,.T.);
#4597=EDGE_CURVE('',#3664,#3662,#413,.T.);
#4598=EDGE_CURVE('',#3665,#3663,#414,.T.);
#4599=EDGE_CURVE('',#3666,#3667,#2193,.T.);
#4600=EDGE_CURVE('',#3666,#3664,#415,.T.);
#4601=EDGE_CURVE('',#3667,#3665,#416,.T.);
#4602=EDGE_CURVE('',#3668,#3669,#2194,.T.);
#4603=EDGE_CURVE('',#3668,#3666,#417,.T.);
#4604=EDGE_CURVE('',#3669,#3667,#418,.T.);
#4605=EDGE_CURVE('',#3670,#3671,#2195,.T.);
#4606=EDGE_CURVE('',#3670,#3668,#419,.T.);
#4607=EDGE_CURVE('',#3671,#3669,#420,.T.);
#4608=EDGE_CURVE('',#3672,#3673,#2196,.T.);
#4609=EDGE_CURVE('',#3672,#3670,#421,.T.);
#4610=EDGE_CURVE('',#3673,#3671,#422,.T.);
#4611=EDGE_CURVE('',#3674,#3675,#2197,.T.);
#4612=EDGE_CURVE('',#3674,#3672,#423,.T.);
#4613=EDGE_CURVE('',#3675,#3673,#424,.T.);
#4614=EDGE_CURVE('',#3676,#3677,#2198,.T.);
#4615=EDGE_CURVE('',#3676,#3674,#425,.T.);
#4616=EDGE_CURVE('',#3677,#3675,#426,.T.);
#4617=EDGE_CURVE('',#3678,#3679,#2199,.T.);
#4618=EDGE_CURVE('',#3678,#3676,#427,.T.);
#4619=EDGE_CURVE('',#3679,#3677,#428,.T.);
#4620=EDGE_CURVE('',#3680,#3681,#2200,.T.);
#4621=EDGE_CURVE('',#3680,#3678,#429,.T.);
#4622=EDGE_CURVE('',#3681,#3679,#430,.T.);
#4623=EDGE_CURVE('',#3682,#3683,#2201,.T.);
#4624=EDGE_CURVE('',#3682,#3680,#431,.T.);
#4625=EDGE_CURVE('',#3683,#3681,#432,.T.);
#4626=EDGE_CURVE('',#3684,#3685,#2202,.T.);
#4627=EDGE_CURVE('',#3684,#3682,#433,.T.);
#4628=EDGE_CURVE('',#3685,#3683,#434,.T.);
#4629=EDGE_CURVE('',#3686,#3687,#2203,.T.);
#4630=EDGE_CURVE('',#3686,#3684,#435,.T.);
#4631=EDGE_CURVE('',#3687,#3685,#436,.T.);
#4632=EDGE_CURVE('',#3688,#3689,#2204,.T.);
#4633=EDGE_CURVE('',#3688,#3686,#437,.T.);
#4634=EDGE_CURVE('',#3689,#3687,#438,.T.);
#4635=EDGE_CURVE('',#3690,#3691,#2205,.T.);
#4636=EDGE_CURVE('',#3690,#3688,#439,.T.);
#4637=EDGE_CURVE('',#3691,#3689,#440,.T.);
#4638=EDGE_CURVE('',#3692,#3693,#2206,.T.);
#4639=EDGE_CURVE('',#3692,#3690,#441,.T.);
#4640=EDGE_CURVE('',#3693,#3691,#442,.T.);
#4641=EDGE_CURVE('',#3694,#3695,#2207,.T.);
#4642=EDGE_CURVE('',#3694,#3692,#443,.T.);
#4643=EDGE_CURVE('',#3695,#3693,#444,.T.);
#4644=EDGE_CURVE('',#3696,#3697,#2208,.T.);
#4645=EDGE_CURVE('',#3696,#3694,#445,.T.);
#4646=EDGE_CURVE('',#3697,#3695,#446,.T.);
#4647=EDGE_CURVE('',#3698,#3699,#2209,.T.);
#4648=EDGE_CURVE('',#3698,#3696,#447,.T.);
#4649=EDGE_CURVE('',#3699,#3697,#448,.T.);
#4650=EDGE_CURVE('',#3700,#3701,#2210,.T.);
#4651=EDGE_CURVE('',#3700,#3698,#449,.T.);
#4652=EDGE_CURVE('',#3701,#3699,#450,.T.);
#4653=EDGE_CURVE('',#3702,#3703,#2211,.T.);
#4654=EDGE_CURVE('',#3702,#3700,#451,.T.);
#4655=EDGE_CURVE('',#3703,#3701,#452,.T.);
#4656=EDGE_CURVE('',#3704,#3705,#2212,.T.);
#4657=EDGE_CURVE('',#3704,#3702,#453,.T.);
#4658=EDGE_CURVE('',#3705,#3703,#454,.T.);
#4659=EDGE_CURVE('',#3706,#3707,#2213,.T.);
#4660=EDGE_CURVE('',#3706,#3704,#455,.T.);
#4661=EDGE_CURVE('',#3707,#3705,#456,.T.);
#4662=EDGE_CURVE('',#3708,#3709,#2214,.T.);
#4663=EDGE_CURVE('',#3708,#3706,#457,.T.);
#4664=EDGE_CURVE('',#3709,#3707,#458,.T.);
#4665=EDGE_CURVE('',#3710,#3711,#2215,.T.);
#4666=EDGE_CURVE('',#3710,#3708,#459,.T.);
#4667=EDGE_CURVE('',#3711,#3709,#460,.T.);
#4668=EDGE_CURVE('',#3712,#3713,#2216,.T.);
#4669=EDGE_CURVE('',#3712,#3710,#461,.T.);
#4670=EDGE_CURVE('',#3713,#3711,#462,.T.);
#4671=EDGE_CURVE('',#3714,#3715,#2217,.T.);
#4672=EDGE_CURVE('',#3714,#3712,#463,.T.);
#4673=EDGE_CURVE('',#3715,#3713,#464,.T.);
#4674=EDGE_CURVE('',#3716,#3717,#2218,.T.);
#4675=EDGE_CURVE('',#3716,#3714,#465,.T.);
#4676=EDGE_CURVE('',#3717,#3715,#466,.T.);
#4677=EDGE_CURVE('',#3718,#3719,#2219,.T.);
#4678=EDGE_CURVE('',#3718,#3716,#467,.T.);
#4679=EDGE_CURVE('',#3719,#3717,#468,.T.);
#4680=EDGE_CURVE('',#3720,#3721,#2220,.T.);
#4681=EDGE_CURVE('',#3720,#3718,#469,.T.);
#4682=EDGE_CURVE('',#3721,#3719,#470,.T.);
#4683=EDGE_CURVE('',#3722,#3723,#2221,.T.);
#4684=EDGE_CURVE('',#3722,#3720,#471,.T.);
#4685=EDGE_CURVE('',#3723,#3721,#472,.T.);
#4686=EDGE_CURVE('',#3724,#3725,#2222,.T.);
#4687=EDGE_CURVE('',#3724,#3722,#473,.T.);
#4688=EDGE_CURVE('',#3725,#3723,#474,.T.);
#4689=EDGE_CURVE('',#3726,#3727,#2223,.T.);
#4690=EDGE_CURVE('',#3726,#3724,#475,.T.);
#4691=EDGE_CURVE('',#3727,#3725,#476,.T.);
#4692=EDGE_CURVE('',#3728,#3729,#2224,.T.);
#4693=EDGE_CURVE('',#3728,#3726,#477,.T.);
#4694=EDGE_CURVE('',#3729,#3727,#478,.T.);
#4695=EDGE_CURVE('',#3730,#3731,#2225,.T.);
#4696=EDGE_CURVE('',#3730,#3728,#479,.T.);
#4697=EDGE_CURVE('',#3731,#3729,#480,.T.);
#4698=EDGE_CURVE('',#3732,#3733,#2226,.T.);
#4699=EDGE_CURVE('',#3732,#3730,#481,.T.);
#4700=EDGE_CURVE('',#3733,#3731,#482,.T.);
#4701=EDGE_CURVE('',#3734,#3735,#2227,.T.);
#4702=EDGE_CURVE('',#3734,#3732,#483,.T.);
#4703=EDGE_CURVE('',#3735,#3733,#484,.T.);
#4704=EDGE_CURVE('',#3736,#3737,#2228,.T.);
#4705=EDGE_CURVE('',#3736,#3734,#485,.T.);
#4706=EDGE_CURVE('',#3737,#3735,#486,.T.);
#4707=EDGE_CURVE('',#3738,#3739,#2229,.T.);
#4708=EDGE_CURVE('',#3738,#3736,#487,.T.);
#4709=EDGE_CURVE('',#3739,#3737,#488,.T.);
#4710=EDGE_CURVE('',#3740,#3741,#2230,.T.);
#4711=EDGE_CURVE('',#3740,#3738,#489,.T.);
#4712=EDGE_CURVE('',#3741,#3739,#490,.T.);
#4713=EDGE_CURVE('',#3742,#3743,#2231,.T.);
#4714=EDGE_CURVE('',#3742,#3740,#491,.T.);
#4715=EDGE_CURVE('',#3743,#3741,#492,.T.);
#4716=EDGE_CURVE('',#3744,#3745,#2232,.T.);
#4717=EDGE_CURVE('',#3744,#3742,#493,.T.);
#4718=EDGE_CURVE('',#3745,#3743,#494,.T.);
#4719=EDGE_CURVE('',#3746,#3747,#2233,.T.);
#4720=EDGE_CURVE('',#3746,#3744,#495,.T.);
#4721=EDGE_CURVE('',#3747,#3745,#496,.T.);
#4722=EDGE_CURVE('',#3748,#3749,#2234,.T.);
#4723=EDGE_CURVE('',#3748,#3746,#497,.T.);
#4724=EDGE_CURVE('',#3749,#3747,#498,.T.);
#4725=EDGE_CURVE('',#3750,#3751,#2235,.T.);
#4726=EDGE_CURVE('',#3750,#3748,#499,.T.);
#4727=EDGE_CURVE('',#3751,#3749,#500,.T.);
#4728=EDGE_CURVE('',#3752,#3753,#2236,.T.);
#4729=EDGE_CURVE('',#3752,#3750,#501,.T.);
#4730=EDGE_CURVE('',#3753,#3751,#502,.T.);
#4731=EDGE_CURVE('',#3754,#3755,#2237,.T.);
#4732=EDGE_CURVE('',#3754,#3752,#503,.T.);
#4733=EDGE_CURVE('',#3755,#3753,#504,.T.);
#4734=EDGE_CURVE('',#3756,#3757,#2238,.T.);
#4735=EDGE_CURVE('',#3756,#3754,#505,.T.);
#4736=EDGE_CURVE('',#3757,#3755,#506,.T.);
#4737=EDGE_CURVE('',#3758,#3759,#2239,.T.);
#4738=EDGE_CURVE('',#3758,#3756,#507,.T.);
#4739=EDGE_CURVE('',#3759,#3757,#508,.T.);
#4740=EDGE_CURVE('',#3760,#3761,#2240,.T.);
#4741=EDGE_CURVE('',#3760,#3758,#509,.T.);
#4742=EDGE_CURVE('',#3761,#3759,#510,.T.);
#4743=EDGE_CURVE('',#3762,#3763,#2241,.T.);
#4744=EDGE_CURVE('',#3762,#3760,#511,.T.);
#4745=EDGE_CURVE('',#3763,#3761,#512,.T.);
#4746=EDGE_CURVE('',#3764,#3765,#2242,.T.);
#4747=EDGE_CURVE('',#3764,#3762,#513,.T.);
#4748=EDGE_CURVE('',#3765,#3763,#514,.T.);
#4749=EDGE_CURVE('',#3766,#3767,#2243,.T.);
#4750=EDGE_CURVE('',#3766,#3764,#515,.T.);
#4751=EDGE_CURVE('',#3767,#3765,#516,.T.);
#4752=EDGE_CURVE('',#3768,#3769,#2244,.T.);
#4753=EDGE_CURVE('',#3768,#3766,#517,.T.);
#4754=EDGE_CURVE('',#3769,#3767,#518,.T.);
#4755=EDGE_CURVE('',#3770,#3771,#2245,.T.);
#4756=EDGE_CURVE('',#3770,#3768,#519,.T.);
#4757=EDGE_CURVE('',#3771,#3769,#520,.T.);
#4758=EDGE_CURVE('',#3772,#3773,#2246,.T.);
#4759=EDGE_CURVE('',#3772,#3770,#521,.T.);
#4760=EDGE_CURVE('',#3773,#3771,#522,.T.);
#4761=EDGE_CURVE('',#3774,#3775,#2247,.T.);
#4762=EDGE_CURVE('',#3774,#3772,#523,.T.);
#4763=EDGE_CURVE('',#3775,#3773,#524,.T.);
#4764=EDGE_CURVE('',#3776,#3777,#2248,.T.);
#4765=EDGE_CURVE('',#3776,#3774,#525,.T.);
#4766=EDGE_CURVE('',#3777,#3775,#526,.T.);
#4767=EDGE_CURVE('',#3778,#3779,#2249,.T.);
#4768=EDGE_CURVE('',#3778,#3776,#527,.T.);
#4769=EDGE_CURVE('',#3779,#3777,#528,.T.);
#4770=EDGE_CURVE('',#3780,#3781,#2250,.T.);
#4771=EDGE_CURVE('',#3780,#3778,#529,.T.);
#4772=EDGE_CURVE('',#3781,#3779,#530,.T.);
#4773=EDGE_CURVE('',#3782,#3783,#2251,.T.);
#4774=EDGE_CURVE('',#3782,#3780,#531,.T.);
#4775=EDGE_CURVE('',#3783,#3781,#532,.T.);
#4776=EDGE_CURVE('',#3784,#3785,#2252,.T.);
#4777=EDGE_CURVE('',#3784,#3782,#533,.T.);
#4778=EDGE_CURVE('',#3785,#3783,#534,.T.);
#4779=EDGE_CURVE('',#3786,#3787,#2253,.T.);
#4780=EDGE_CURVE('',#3786,#3784,#535,.T.);
#4781=EDGE_CURVE('',#3787,#3785,#536,.T.);
#4782=EDGE_CURVE('',#3788,#3789,#2254,.T.);
#4783=EDGE_CURVE('',#3788,#3786,#537,.T.);
#4784=EDGE_CURVE('',#3789,#3787,#538,.T.);
#4785=EDGE_CURVE('',#3790,#3791,#2255,.T.);
#4786=EDGE_CURVE('',#3790,#3788,#539,.T.);
#4787=EDGE_CURVE('',#3791,#3789,#540,.T.);
#4788=EDGE_CURVE('',#3792,#3793,#2256,.T.);
#4789=EDGE_CURVE('',#3792,#3790,#541,.T.);
#4790=EDGE_CURVE('',#3793,#3791,#542,.T.);
#4791=EDGE_CURVE('',#3794,#3795,#2257,.T.);
#4792=EDGE_CURVE('',#3794,#3792,#543,.T.);
#4793=EDGE_CURVE('',#3795,#3793,#544,.T.);
#4794=EDGE_CURVE('',#3796,#3797,#2258,.T.);
#4795=EDGE_CURVE('',#3796,#3794,#545,.T.);
#4796=EDGE_CURVE('',#3797,#3795,#546,.T.);
#4797=EDGE_CURVE('',#3798,#3799,#2259,.T.);
#4798=EDGE_CURVE('',#3798,#3796,#547,.T.);
#4799=EDGE_CURVE('',#3799,#3797,#548,.T.);
#4800=EDGE_CURVE('',#3800,#3801,#2260,.T.);
#4801=EDGE_CURVE('',#3800,#3798,#549,.T.);
#4802=EDGE_CURVE('',#3801,#3799,#550,.T.);
#4803=EDGE_CURVE('',#3802,#3803,#2261,.T.);
#4804=EDGE_CURVE('',#3802,#3800,#551,.T.);
#4805=EDGE_CURVE('',#3803,#3801,#552,.T.);
#4806=EDGE_CURVE('',#3804,#3805,#2262,.T.);
#4807=EDGE_CURVE('',#3804,#3802,#553,.T.);
#4808=EDGE_CURVE('',#3805,#3803,#554,.T.);
#4809=EDGE_CURVE('',#3806,#3807,#2263,.T.);
#4810=EDGE_CURVE('',#3806,#3804,#555,.T.);
#4811=EDGE_CURVE('',#3807,#3805,#556,.T.);
#4812=EDGE_CURVE('',#3808,#3809,#2264,.T.);
#4813=EDGE_CURVE('',#3808,#3806,#557,.T.);
#4814=EDGE_CURVE('',#3809,#3807,#558,.T.);
#4815=EDGE_CURVE('',#3810,#3811,#2265,.T.);
#4816=EDGE_CURVE('',#3810,#3808,#559,.T.);
#4817=EDGE_CURVE('',#3811,#3809,#560,.T.);
#4818=EDGE_CURVE('',#3812,#3813,#2266,.T.);
#4819=EDGE_CURVE('',#3812,#3810,#561,.T.);
#4820=EDGE_CURVE('',#3813,#3811,#562,.T.);
#4821=EDGE_CURVE('',#3814,#3815,#2267,.T.);
#4822=EDGE_CURVE('',#3814,#3812,#563,.T.);
#4823=EDGE_CURVE('',#3815,#3813,#564,.T.);
#4824=EDGE_CURVE('',#3816,#3817,#2268,.T.);
#4825=EDGE_CURVE('',#3816,#3814,#565,.T.);
#4826=EDGE_CURVE('',#3817,#3815,#566,.T.);
#4827=EDGE_CURVE('',#3818,#3819,#2269,.T.);
#4828=EDGE_CURVE('',#3818,#3816,#567,.T.);
#4829=EDGE_CURVE('',#3819,#3817,#568,.T.);
#4830=EDGE_CURVE('',#3820,#3821,#2270,.T.);
#4831=EDGE_CURVE('',#3820,#3818,#569,.T.);
#4832=EDGE_CURVE('',#3821,#3819,#570,.T.);
#4833=EDGE_CURVE('',#3822,#3823,#2271,.T.);
#4834=EDGE_CURVE('',#3822,#3820,#571,.T.);
#4835=EDGE_CURVE('',#3823,#3821,#572,.T.);
#4836=EDGE_CURVE('',#3824,#3825,#2272,.T.);
#4837=EDGE_CURVE('',#3824,#3822,#573,.T.);
#4838=EDGE_CURVE('',#3825,#3823,#574,.T.);
#4839=EDGE_CURVE('',#3826,#3827,#2273,.T.);
#4840=EDGE_CURVE('',#3826,#3824,#575,.T.);
#4841=EDGE_CURVE('',#3827,#3825,#576,.T.);
#4842=EDGE_CURVE('',#3828,#3829,#2274,.T.);
#4843=EDGE_CURVE('',#3828,#3826,#577,.T.);
#4844=EDGE_CURVE('',#3829,#3827,#578,.T.);
#4845=EDGE_CURVE('',#3830,#3831,#2275,.T.);
#4846=EDGE_CURVE('',#3830,#3828,#579,.T.);
#4847=EDGE_CURVE('',#3831,#3829,#580,.T.);
#4848=EDGE_CURVE('',#3832,#3833,#2276,.T.);
#4849=EDGE_CURVE('',#3832,#3830,#581,.T.);
#4850=EDGE_CURVE('',#3833,#3831,#582,.T.);
#4851=EDGE_CURVE('',#3834,#3835,#2277,.T.);
#4852=EDGE_CURVE('',#3834,#3832,#583,.T.);
#4853=EDGE_CURVE('',#3835,#3833,#584,.T.);
#4854=EDGE_CURVE('',#3836,#3837,#2278,.T.);
#4855=EDGE_CURVE('',#3836,#3834,#585,.T.);
#4856=EDGE_CURVE('',#3837,#3835,#586,.T.);
#4857=EDGE_CURVE('',#3838,#3839,#2279,.T.);
#4858=EDGE_CURVE('',#3838,#3836,#587,.T.);
#4859=EDGE_CURVE('',#3839,#3837,#588,.T.);
#4860=EDGE_CURVE('',#3840,#3841,#2280,.T.);
#4861=EDGE_CURVE('',#3840,#3838,#589,.T.);
#4862=EDGE_CURVE('',#3841,#3839,#590,.T.);
#4863=EDGE_CURVE('',#3842,#3843,#2281,.T.);
#4864=EDGE_CURVE('',#3842,#3840,#591,.T.);
#4865=EDGE_CURVE('',#3843,#3841,#592,.T.);
#4866=EDGE_CURVE('',#3844,#3844,#3324,.T.);
#4867=EDGE_CURVE('',#3844,#3845,#2282,.T.);
#4868=EDGE_CURVE('',#3845,#3845,#3325,.T.);
#4869=EDGE_CURVE('',#3846,#3846,#3326,.T.);
#4870=EDGE_CURVE('',#3846,#3847,#2283,.T.);
#4871=EDGE_CURVE('',#3847,#3847,#3327,.T.);
#4872=EDGE_CURVE('',#3848,#3848,#3328,.T.);
#4873=EDGE_CURVE('',#3848,#3849,#2284,.T.);
#4874=EDGE_CURVE('',#3849,#3849,#3329,.T.);
#4875=EDGE_CURVE('',#3850,#3850,#3330,.T.);
#4876=EDGE_CURVE('',#3850,#3851,#2285,.T.);
#4877=EDGE_CURVE('',#3851,#3851,#3331,.T.);
#4878=EDGE_CURVE('',#3852,#3852,#3332,.T.);
#4879=EDGE_CURVE('',#3852,#3853,#2286,.T.);
#4880=EDGE_CURVE('',#3853,#3853,#3333,.T.);
#4881=EDGE_CURVE('',#3854,#3854,#3334,.T.);
#4882=EDGE_CURVE('',#3854,#3855,#2287,.T.);
#4883=EDGE_CURVE('',#3855,#3855,#3335,.T.);
#4884=EDGE_CURVE('',#3856,#3856,#3336,.T.);
#4885=EDGE_CURVE('',#3857,#3467,#593,.T.);
#4886=EDGE_CURVE('',#3466,#3858,#594,.T.);
#4887=EDGE_CURVE('',#3858,#3857,#3337,.T.);
#4888=EDGE_CURVE('',#3856,#3859,#2288,.T.);
#4889=EDGE_CURVE('',#3859,#3859,#3338,.T.);
#4890=EDGE_CURVE('',#3860,#3657,#595,.T.);
#4891=EDGE_CURVE('',#3653,#3860,#596,.T.);
#4892=EDGE_CURVE('',#3857,#3843,#597,.T.);
#4893=EDGE_CURVE('',#3858,#3842,#598,.T.);
#4894=EDGE_CURVE('',#3656,#3861,#599,.T.);
#4895=EDGE_CURVE('',#3861,#3652,#600,.T.);
#4896=EDGE_CURVE('',#3861,#3860,#3339,.F.);
#5573=ORIENTED_EDGE('',*,*,#4300,.F.);
#5574=ORIENTED_EDGE('',*,*,#4301,.T.);
#5575=ORIENTED_EDGE('',*,*,#4302,.T.);
#5576=ORIENTED_EDGE('',*,*,#4303,.T.);
#5577=ORIENTED_EDGE('',*,*,#4304,.F.);
#5578=ORIENTED_EDGE('',*,*,#4305,.T.);
#5579=ORIENTED_EDGE('',*,*,#4300,.T.);
#5580=ORIENTED_EDGE('',*,*,#4306,.T.);
#5581=ORIENTED_EDGE('',*,*,#4307,.F.);
#5582=ORIENTED_EDGE('',*,*,#4308,.T.);
#5583=ORIENTED_EDGE('',*,*,#4304,.T.);
#5584=ORIENTED_EDGE('',*,*,#4309,.T.);
#5585=ORIENTED_EDGE('',*,*,#4310,.F.);
#5586=ORIENTED_EDGE('',*,*,#4311,.T.);
#5587=ORIENTED_EDGE('',*,*,#4307,.T.);
#5588=ORIENTED_EDGE('',*,*,#4312,.T.);
#5589=ORIENTED_EDGE('',*,*,#4313,.F.);
#5590=ORIENTED_EDGE('',*,*,#4314,.T.);
#5591=ORIENTED_EDGE('',*,*,#4310,.T.);
#5592=ORIENTED_EDGE('',*,*,#4315,.T.);
#5593=ORIENTED_EDGE('',*,*,#4316,.F.);
#5594=ORIENTED_EDGE('',*,*,#4317,.T.);
#5595=ORIENTED_EDGE('',*,*,#4313,.T.);
#5596=ORIENTED_EDGE('',*,*,#4318,.T.);
#5597=ORIENTED_EDGE('',*,*,#4319,.F.);
#5598=ORIENTED_EDGE('',*,*,#4320,.T.);
#5599=ORIENTED_EDGE('',*,*,#4316,.T.);
#5600=ORIENTED_EDGE('',*,*,#4321,.T.);
#5601=ORIENTED_EDGE('',*,*,#4322,.F.);
#5602=ORIENTED_EDGE('',*,*,#4323,.T.);
#5603=ORIENTED_EDGE('',*,*,#4319,.T.);
#5604=ORIENTED_EDGE('',*,*,#4324,.T.);
#5605=ORIENTED_EDGE('',*,*,#4325,.F.);
#5606=ORIENTED_EDGE('',*,*,#4326,.T.);
#5607=ORIENTED_EDGE('',*,*,#4322,.T.);
#5608=ORIENTED_EDGE('',*,*,#4327,.T.);
#5609=ORIENTED_EDGE('',*,*,#4328,.F.);
#5610=ORIENTED_EDGE('',*,*,#4329,.T.);
#5611=ORIENTED_EDGE('',*,*,#4325,.T.);
#5612=ORIENTED_EDGE('',*,*,#4330,.T.);
#5613=ORIENTED_EDGE('',*,*,#4331,.F.);
#5614=ORIENTED_EDGE('',*,*,#4332,.T.);
#5615=ORIENTED_EDGE('',*,*,#4328,.T.);
#5616=ORIENTED_EDGE('',*,*,#4333,.T.);
#5617=ORIENTED_EDGE('',*,*,#4334,.F.);
#5618=ORIENTED_EDGE('',*,*,#4335,.T.);
#5619=ORIENTED_EDGE('',*,*,#4331,.T.);
#5620=ORIENTED_EDGE('',*,*,#4336,.T.);
#5621=ORIENTED_EDGE('',*,*,#4337,.F.);
#5622=ORIENTED_EDGE('',*,*,#4338,.T.);
#5623=ORIENTED_EDGE('',*,*,#4334,.T.);
#5624=ORIENTED_EDGE('',*,*,#4339,.T.);
#5625=ORIENTED_EDGE('',*,*,#4340,.F.);
#5626=ORIENTED_EDGE('',*,*,#4341,.T.);
#5627=ORIENTED_EDGE('',*,*,#4337,.T.);
#5628=ORIENTED_EDGE('',*,*,#4342,.T.);
#5629=ORIENTED_EDGE('',*,*,#4343,.F.);
#5630=ORIENTED_EDGE('',*,*,#4344,.T.);
#5631=ORIENTED_EDGE('',*,*,#4340,.T.);
#5632=ORIENTED_EDGE('',*,*,#4345,.T.);
#5633=ORIENTED_EDGE('',*,*,#4346,.F.);
#5634=ORIENTED_EDGE('',*,*,#4347,.T.);
#5635=ORIENTED_EDGE('',*,*,#4343,.T.);
#5636=ORIENTED_EDGE('',*,*,#4348,.T.);
#5637=ORIENTED_EDGE('',*,*,#4349,.F.);
#5638=ORIENTED_EDGE('',*,*,#4350,.T.);
#5639=ORIENTED_EDGE('',*,*,#4346,.T.);
#5640=ORIENTED_EDGE('',*,*,#4351,.T.);
#5641=ORIENTED_EDGE('',*,*,#4352,.F.);
#5642=ORIENTED_EDGE('',*,*,#4353,.T.);
#5643=ORIENTED_EDGE('',*,*,#4349,.T.);
#5644=ORIENTED_EDGE('',*,*,#4354,.T.);
#5645=ORIENTED_EDGE('',*,*,#4355,.F.);
#5646=ORIENTED_EDGE('',*,*,#4356,.T.);
#5647=ORIENTED_EDGE('',*,*,#4352,.T.);
#5648=ORIENTED_EDGE('',*,*,#4357,.T.);
#5649=ORIENTED_EDGE('',*,*,#4358,.F.);
#5650=ORIENTED_EDGE('',*,*,#4359,.T.);
#5651=ORIENTED_EDGE('',*,*,#4355,.T.);
#5652=ORIENTED_EDGE('',*,*,#4360,.T.);
#5653=ORIENTED_EDGE('',*,*,#4361,.F.);
#5654=ORIENTED_EDGE('',*,*,#4362,.T.);
#5655=ORIENTED_EDGE('',*,*,#4358,.T.);
#5656=ORIENTED_EDGE('',*,*,#4363,.T.);
#5657=ORIENTED_EDGE('',*,*,#4364,.F.);
#5658=ORIENTED_EDGE('',*,*,#4365,.T.);
#5659=ORIENTED_EDGE('',*,*,#4361,.T.);
#5660=ORIENTED_EDGE('',*,*,#4366,.T.);
#5661=ORIENTED_EDGE('',*,*,#4367,.F.);
#5662=ORIENTED_EDGE('',*,*,#4368,.T.);
#5663=ORIENTED_EDGE('',*,*,#4364,.T.);
#5664=ORIENTED_EDGE('',*,*,#4369,.T.);
#5665=ORIENTED_EDGE('',*,*,#4370,.F.);
#5666=ORIENTED_EDGE('',*,*,#4371,.T.);
#5667=ORIENTED_EDGE('',*,*,#4367,.T.);
#5668=ORIENTED_EDGE('',*,*,#4372,.T.);
#5669=ORIENTED_EDGE('',*,*,#4373,.F.);
#5670=ORIENTED_EDGE('',*,*,#4374,.T.);
#5671=ORIENTED_EDGE('',*,*,#4370,.T.);
#5672=ORIENTED_EDGE('',*,*,#4375,.T.);
#5673=ORIENTED_EDGE('',*,*,#4376,.F.);
#5674=ORIENTED_EDGE('',*,*,#4377,.T.);
#5675=ORIENTED_EDGE('',*,*,#4373,.T.);
#5676=ORIENTED_EDGE('',*,*,#4378,.T.);
#5677=ORIENTED_EDGE('',*,*,#4379,.F.);
#5678=ORIENTED_EDGE('',*,*,#4380,.T.);
#5679=ORIENTED_EDGE('',*,*,#4376,.T.);
#5680=ORIENTED_EDGE('',*,*,#4381,.T.);
#5681=ORIENTED_EDGE('',*,*,#4382,.F.);
#5682=ORIENTED_EDGE('',*,*,#4383,.T.);
#5683=ORIENTED_EDGE('',*,*,#4379,.T.);
#5684=ORIENTED_EDGE('',*,*,#4384,.T.);
#5685=ORIENTED_EDGE('',*,*,#4385,.F.);
#5686=ORIENTED_EDGE('',*,*,#4386,.T.);
#5687=ORIENTED_EDGE('',*,*,#4382,.T.);
#5688=ORIENTED_EDGE('',*,*,#4387,.T.);
#5689=ORIENTED_EDGE('',*,*,#4388,.F.);
#5690=ORIENTED_EDGE('',*,*,#4389,.T.);
#5691=ORIENTED_EDGE('',*,*,#4385,.T.);
#5692=ORIENTED_EDGE('',*,*,#4390,.T.);
#5693=ORIENTED_EDGE('',*,*,#4391,.F.);
#5694=ORIENTED_EDGE('',*,*,#4392,.T.);
#5695=ORIENTED_EDGE('',*,*,#4388,.T.);
#5696=ORIENTED_EDGE('',*,*,#4393,.T.);
#5697=ORIENTED_EDGE('',*,*,#4394,.F.);
#5698=ORIENTED_EDGE('',*,*,#4395,.T.);
#5699=ORIENTED_EDGE('',*,*,#4391,.T.);
#5700=ORIENTED_EDGE('',*,*,#4396,.T.);
#5701=ORIENTED_EDGE('',*,*,#4397,.F.);
#5702=ORIENTED_EDGE('',*,*,#4398,.T.);
#5703=ORIENTED_EDGE('',*,*,#4394,.T.);
#5704=ORIENTED_EDGE('',*,*,#4399,.T.);
#5705=ORIENTED_EDGE('',*,*,#4400,.F.);
#5706=ORIENTED_EDGE('',*,*,#4401,.T.);
#5707=ORIENTED_EDGE('',*,*,#4397,.T.);
#5708=ORIENTED_EDGE('',*,*,#4402,.T.);
#5709=ORIENTED_EDGE('',*,*,#4403,.F.);
#5710=ORIENTED_EDGE('',*,*,#4404,.T.);
#5711=ORIENTED_EDGE('',*,*,#4400,.T.);
#5712=ORIENTED_EDGE('',*,*,#4405,.T.);
#5713=ORIENTED_EDGE('',*,*,#4406,.F.);
#5714=ORIENTED_EDGE('',*,*,#4407,.T.);
#5715=ORIENTED_EDGE('',*,*,#4403,.T.);
#5716=ORIENTED_EDGE('',*,*,#4408,.T.);
#5717=ORIENTED_EDGE('',*,*,#4409,.F.);
#5718=ORIENTED_EDGE('',*,*,#4410,.T.);
#5719=ORIENTED_EDGE('',*,*,#4406,.T.);
#5720=ORIENTED_EDGE('',*,*,#4411,.T.);
#5721=ORIENTED_EDGE('',*,*,#4412,.F.);
#5722=ORIENTED_EDGE('',*,*,#4413,.T.);
#5723=ORIENTED_EDGE('',*,*,#4409,.T.);
#5724=ORIENTED_EDGE('',*,*,#4414,.T.);
#5725=ORIENTED_EDGE('',*,*,#4415,.F.);
#5726=ORIENTED_EDGE('',*,*,#4416,.T.);
#5727=ORIENTED_EDGE('',*,*,#4412,.T.);
#5728=ORIENTED_EDGE('',*,*,#4417,.T.);
#5729=ORIENTED_EDGE('',*,*,#4418,.F.);
#5730=ORIENTED_EDGE('',*,*,#4419,.T.);
#5731=ORIENTED_EDGE('',*,*,#4415,.T.);
#5732=ORIENTED_EDGE('',*,*,#4420,.T.);
#5733=ORIENTED_EDGE('',*,*,#4421,.F.);
#5734=ORIENTED_EDGE('',*,*,#4422,.T.);
#5735=ORIENTED_EDGE('',*,*,#4418,.T.);
#5736=ORIENTED_EDGE('',*,*,#4423,.T.);
#5737=ORIENTED_EDGE('',*,*,#4424,.F.);
#5738=ORIENTED_EDGE('',*,*,#4425,.T.);
#5739=ORIENTED_EDGE('',*,*,#4421,.T.);
#5740=ORIENTED_EDGE('',*,*,#4426,.T.);
#5741=ORIENTED_EDGE('',*,*,#4427,.F.);
#5742=ORIENTED_EDGE('',*,*,#4428,.T.);
#5743=ORIENTED_EDGE('',*,*,#4424,.T.);
#5744=ORIENTED_EDGE('',*,*,#4429,.T.);
#5745=ORIENTED_EDGE('',*,*,#4430,.F.);
#5746=ORIENTED_EDGE('',*,*,#4431,.T.);
#5747=ORIENTED_EDGE('',*,*,#4427,.T.);
#5748=ORIENTED_EDGE('',*,*,#4432,.T.);
#5749=ORIENTED_EDGE('',*,*,#4433,.F.);
#5750=ORIENTED_EDGE('',*,*,#4434,.T.);
#5751=ORIENTED_EDGE('',*,*,#4430,.T.);
#5752=ORIENTED_EDGE('',*,*,#4435,.T.);
#5753=ORIENTED_EDGE('',*,*,#4436,.F.);
#5754=ORIENTED_EDGE('',*,*,#4437,.T.);
#5755=ORIENTED_EDGE('',*,*,#4433,.T.);
#5756=ORIENTED_EDGE('',*,*,#4438,.T.);
#5757=ORIENTED_EDGE('',*,*,#4439,.F.);
#5758=ORIENTED_EDGE('',*,*,#4440,.T.);
#5759=ORIENTED_EDGE('',*,*,#4436,.T.);
#5760=ORIENTED_EDGE('',*,*,#4441,.T.);
#5761=ORIENTED_EDGE('',*,*,#4442,.F.);
#5762=ORIENTED_EDGE('',*,*,#4443,.T.);
#5763=ORIENTED_EDGE('',*,*,#4439,.T.);
#5764=ORIENTED_EDGE('',*,*,#4444,.T.);
#5765=ORIENTED_EDGE('',*,*,#4445,.F.);
#5766=ORIENTED_EDGE('',*,*,#4446,.T.);
#5767=ORIENTED_EDGE('',*,*,#4442,.T.);
#5768=ORIENTED_EDGE('',*,*,#4447,.T.);
#5769=ORIENTED_EDGE('',*,*,#4448,.F.);
#5770=ORIENTED_EDGE('',*,*,#4449,.T.);
#5771=ORIENTED_EDGE('',*,*,#4445,.T.);
#5772=ORIENTED_EDGE('',*,*,#4450,.T.);
#5773=ORIENTED_EDGE('',*,*,#4451,.F.);
#5774=ORIENTED_EDGE('',*,*,#4452,.T.);
#5775=ORIENTED_EDGE('',*,*,#4448,.T.);
#5776=ORIENTED_EDGE('',*,*,#4453,.T.);
#5777=ORIENTED_EDGE('',*,*,#4454,.F.);
#5778=ORIENTED_EDGE('',*,*,#4455,.T.);
#5779=ORIENTED_EDGE('',*,*,#4451,.T.);
#5780=ORIENTED_EDGE('',*,*,#4456,.T.);
#5781=ORIENTED_EDGE('',*,*,#4457,.F.);
#5782=ORIENTED_EDGE('',*,*,#4458,.T.);
#5783=ORIENTED_EDGE('',*,*,#4454,.T.);
#5784=ORIENTED_EDGE('',*,*,#4459,.T.);
#5785=ORIENTED_EDGE('',*,*,#4460,.F.);
#5786=ORIENTED_EDGE('',*,*,#4461,.T.);
#5787=ORIENTED_EDGE('',*,*,#4457,.T.);
#5788=ORIENTED_EDGE('',*,*,#4462,.T.);
#5789=ORIENTED_EDGE('',*,*,#4463,.F.);
#5790=ORIENTED_EDGE('',*,*,#4464,.T.);
#5791=ORIENTED_EDGE('',*,*,#4460,.T.);
#5792=ORIENTED_EDGE('',*,*,#4465,.T.);
#5793=ORIENTED_EDGE('',*,*,#4466,.F.);
#5794=ORIENTED_EDGE('',*,*,#4467,.T.);
#5795=ORIENTED_EDGE('',*,*,#4463,.T.);
#5796=ORIENTED_EDGE('',*,*,#4468,.T.);
#5797=ORIENTED_EDGE('',*,*,#4469,.F.);
#5798=ORIENTED_EDGE('',*,*,#4470,.T.);
#5799=ORIENTED_EDGE('',*,*,#4466,.T.);
#5800=ORIENTED_EDGE('',*,*,#4471,.T.);
#5801=ORIENTED_EDGE('',*,*,#4472,.F.);
#5802=ORIENTED_EDGE('',*,*,#4473,.T.);
#5803=ORIENTED_EDGE('',*,*,#4469,.T.);
#5804=ORIENTED_EDGE('',*,*,#4474,.T.);
#5805=ORIENTED_EDGE('',*,*,#4475,.F.);
#5806=ORIENTED_EDGE('',*,*,#4476,.T.);
#5807=ORIENTED_EDGE('',*,*,#4472,.T.);
#5808=ORIENTED_EDGE('',*,*,#4477,.T.);
#5809=ORIENTED_EDGE('',*,*,#4478,.F.);
#5810=ORIENTED_EDGE('',*,*,#4479,.T.);
#5811=ORIENTED_EDGE('',*,*,#4475,.T.);
#5812=ORIENTED_EDGE('',*,*,#4480,.T.);
#5813=ORIENTED_EDGE('',*,*,#4481,.F.);
#5814=ORIENTED_EDGE('',*,*,#4482,.T.);
#5815=ORIENTED_EDGE('',*,*,#4478,.T.);
#5816=ORIENTED_EDGE('',*,*,#4483,.T.);
#5817=ORIENTED_EDGE('',*,*,#4484,.F.);
#5818=ORIENTED_EDGE('',*,*,#4485,.T.);
#5819=ORIENTED_EDGE('',*,*,#4481,.T.);
#5820=ORIENTED_EDGE('',*,*,#4486,.T.);
#5821=ORIENTED_EDGE('',*,*,#4487,.F.);
#5822=ORIENTED_EDGE('',*,*,#4488,.T.);
#5823=ORIENTED_EDGE('',*,*,#4484,.T.);
#5824=ORIENTED_EDGE('',*,*,#4489,.T.);
#5825=ORIENTED_EDGE('',*,*,#4490,.F.);
#5826=ORIENTED_EDGE('',*,*,#4491,.T.);
#5827=ORIENTED_EDGE('',*,*,#4487,.T.);
#5828=ORIENTED_EDGE('',*,*,#4492,.T.);
#5829=ORIENTED_EDGE('',*,*,#4493,.F.);
#5830=ORIENTED_EDGE('',*,*,#4494,.T.);
#5831=ORIENTED_EDGE('',*,*,#4490,.T.);
#5832=ORIENTED_EDGE('',*,*,#4495,.T.);
#5833=ORIENTED_EDGE('',*,*,#4496,.F.);
#5834=ORIENTED_EDGE('',*,*,#4497,.T.);
#5835=ORIENTED_EDGE('',*,*,#4493,.T.);
#5836=ORIENTED_EDGE('',*,*,#4498,.T.);
#5837=ORIENTED_EDGE('',*,*,#4499,.F.);
#5838=ORIENTED_EDGE('',*,*,#4500,.T.);
#5839=ORIENTED_EDGE('',*,*,#4496,.T.);
#5840=ORIENTED_EDGE('',*,*,#4501,.T.);
#5841=ORIENTED_EDGE('',*,*,#4502,.F.);
#5842=ORIENTED_EDGE('',*,*,#4503,.T.);
#5843=ORIENTED_EDGE('',*,*,#4499,.T.);
#5844=ORIENTED_EDGE('',*,*,#4504,.T.);
#5845=ORIENTED_EDGE('',*,*,#4505,.F.);
#5846=ORIENTED_EDGE('',*,*,#4506,.T.);
#5847=ORIENTED_EDGE('',*,*,#4502,.T.);
#5848=ORIENTED_EDGE('',*,*,#4507,.T.);
#5849=ORIENTED_EDGE('',*,*,#4508,.F.);
#5850=ORIENTED_EDGE('',*,*,#4509,.T.);
#5851=ORIENTED_EDGE('',*,*,#4505,.T.);
#5852=ORIENTED_EDGE('',*,*,#4510,.T.);
#5853=ORIENTED_EDGE('',*,*,#4511,.F.);
#5854=ORIENTED_EDGE('',*,*,#4512,.T.);
#5855=ORIENTED_EDGE('',*,*,#4508,.T.);
#5856=ORIENTED_EDGE('',*,*,#4513,.T.);
#5857=ORIENTED_EDGE('',*,*,#4514,.F.);
#5858=ORIENTED_EDGE('',*,*,#4515,.T.);
#5859=ORIENTED_EDGE('',*,*,#4511,.T.);
#5860=ORIENTED_EDGE('',*,*,#4516,.T.);
#5861=ORIENTED_EDGE('',*,*,#4517,.F.);
#5862=ORIENTED_EDGE('',*,*,#4518,.T.);
#5863=ORIENTED_EDGE('',*,*,#4514,.T.);
#5864=ORIENTED_EDGE('',*,*,#4519,.T.);
#5865=ORIENTED_EDGE('',*,*,#4520,.F.);
#5866=ORIENTED_EDGE('',*,*,#4521,.T.);
#5867=ORIENTED_EDGE('',*,*,#4517,.T.);
#5868=ORIENTED_EDGE('',*,*,#4522,.T.);
#5869=ORIENTED_EDGE('',*,*,#4523,.F.);
#5870=ORIENTED_EDGE('',*,*,#4524,.T.);
#5871=ORIENTED_EDGE('',*,*,#4520,.T.);
#5872=ORIENTED_EDGE('',*,*,#4525,.T.);
#5873=ORIENTED_EDGE('',*,*,#4526,.F.);
#5874=ORIENTED_EDGE('',*,*,#4527,.T.);
#5875=ORIENTED_EDGE('',*,*,#4523,.T.);
#5876=ORIENTED_EDGE('',*,*,#4528,.T.);
#5877=ORIENTED_EDGE('',*,*,#4529,.F.);
#5878=ORIENTED_EDGE('',*,*,#4530,.T.);
#5879=ORIENTED_EDGE('',*,*,#4526,.T.);
#5880=ORIENTED_EDGE('',*,*,#4531,.T.);
#5881=ORIENTED_EDGE('',*,*,#4532,.F.);
#5882=ORIENTED_EDGE('',*,*,#4533,.T.);
#5883=ORIENTED_EDGE('',*,*,#4529,.T.);
#5884=ORIENTED_EDGE('',*,*,#4534,.T.);
#5885=ORIENTED_EDGE('',*,*,#4535,.F.);
#5886=ORIENTED_EDGE('',*,*,#4536,.T.);
#5887=ORIENTED_EDGE('',*,*,#4532,.T.);
#5888=ORIENTED_EDGE('',*,*,#4537,.T.);
#5889=ORIENTED_EDGE('',*,*,#4538,.F.);
#5890=ORIENTED_EDGE('',*,*,#4539,.T.);
#5891=ORIENTED_EDGE('',*,*,#4535,.T.);
#5892=ORIENTED_EDGE('',*,*,#4540,.T.);
#5893=ORIENTED_EDGE('',*,*,#4541,.F.);
#5894=ORIENTED_EDGE('',*,*,#4542,.T.);
#5895=ORIENTED_EDGE('',*,*,#4538,.T.);
#5896=ORIENTED_EDGE('',*,*,#4543,.T.);
#5897=ORIENTED_EDGE('',*,*,#4544,.F.);
#5898=ORIENTED_EDGE('',*,*,#4545,.T.);
#5899=ORIENTED_EDGE('',*,*,#4541,.T.);
#5900=ORIENTED_EDGE('',*,*,#4546,.T.);
#5901=ORIENTED_EDGE('',*,*,#4547,.F.);
#5902=ORIENTED_EDGE('',*,*,#4548,.T.);
#5903=ORIENTED_EDGE('',*,*,#4544,.T.);
#5904=ORIENTED_EDGE('',*,*,#4549,.T.);
#5905=ORIENTED_EDGE('',*,*,#4550,.F.);
#5906=ORIENTED_EDGE('',*,*,#4551,.T.);
#5907=ORIENTED_EDGE('',*,*,#4547,.T.);
#5908=ORIENTED_EDGE('',*,*,#4552,.T.);
#5909=ORIENTED_EDGE('',*,*,#4553,.F.);
#5910=ORIENTED_EDGE('',*,*,#4554,.T.);
#5911=ORIENTED_EDGE('',*,*,#4550,.T.);
#5912=ORIENTED_EDGE('',*,*,#4555,.T.);
#5913=ORIENTED_EDGE('',*,*,#4556,.F.);
#5914=ORIENTED_EDGE('',*,*,#4557,.T.);
#5915=ORIENTED_EDGE('',*,*,#4553,.T.);
#5916=ORIENTED_EDGE('',*,*,#4558,.T.);
#5917=ORIENTED_EDGE('',*,*,#4559,.F.);
#5918=ORIENTED_EDGE('',*,*,#4560,.T.);
#5919=ORIENTED_EDGE('',*,*,#4556,.T.);
#5920=ORIENTED_EDGE('',*,*,#4561,.T.);
#5921=ORIENTED_EDGE('',*,*,#4562,.F.);
#5922=ORIENTED_EDGE('',*,*,#4563,.T.);
#5923=ORIENTED_EDGE('',*,*,#4559,.T.);
#5924=ORIENTED_EDGE('',*,*,#4564,.T.);
#5925=ORIENTED_EDGE('',*,*,#4565,.F.);
#5926=ORIENTED_EDGE('',*,*,#4566,.T.);
#5927=ORIENTED_EDGE('',*,*,#4562,.T.);
#5928=ORIENTED_EDGE('',*,*,#4567,.T.);
#5929=ORIENTED_EDGE('',*,*,#4568,.F.);
#5930=ORIENTED_EDGE('',*,*,#4569,.T.);
#5931=ORIENTED_EDGE('',*,*,#4565,.T.);
#5932=ORIENTED_EDGE('',*,*,#4570,.T.);
#5933=ORIENTED_EDGE('',*,*,#4571,.F.);
#5934=ORIENTED_EDGE('',*,*,#4572,.T.);
#5935=ORIENTED_EDGE('',*,*,#4568,.T.);
#5936=ORIENTED_EDGE('',*,*,#4573,.T.);
#5937=ORIENTED_EDGE('',*,*,#4574,.F.);
#5938=ORIENTED_EDGE('',*,*,#4575,.T.);
#5939=ORIENTED_EDGE('',*,*,#4571,.T.);
#5940=ORIENTED_EDGE('',*,*,#4576,.T.);
#5941=ORIENTED_EDGE('',*,*,#4577,.F.);
#5942=ORIENTED_EDGE('',*,*,#4578,.T.);
#5943=ORIENTED_EDGE('',*,*,#4574,.T.);
#5944=ORIENTED_EDGE('',*,*,#4579,.T.);
#5945=ORIENTED_EDGE('',*,*,#4580,.F.);
#5946=ORIENTED_EDGE('',*,*,#4581,.T.);
#5947=ORIENTED_EDGE('',*,*,#4577,.T.);
#5948=ORIENTED_EDGE('',*,*,#4582,.T.);
#5949=ORIENTED_EDGE('',*,*,#4583,.F.);
#5950=ORIENTED_EDGE('',*,*,#4584,.T.);
#5951=ORIENTED_EDGE('',*,*,#4585,.F.);
#5952=ORIENTED_EDGE('',*,*,#4586,.F.);
#5953=ORIENTED_EDGE('',*,*,#4587,.F.);
#5954=ORIENTED_EDGE('',*,*,#4588,.T.);
#5955=ORIENTED_EDGE('',*,*,#4583,.T.);
#5956=ORIENTED_EDGE('',*,*,#4589,.F.);
#5957=ORIENTED_EDGE('',*,*,#4590,.F.);
#5958=ORIENTED_EDGE('',*,*,#4591,.T.);
#5959=ORIENTED_EDGE('',*,*,#4587,.T.);
#5960=ORIENTED_EDGE('',*,*,#4592,.F.);
#5961=ORIENTED_EDGE('',*,*,#4593,.F.);
#5962=ORIENTED_EDGE('',*,*,#4594,.T.);
#5963=ORIENTED_EDGE('',*,*,#4590,.T.);
#5964=ORIENTED_EDGE('',*,*,#4595,.F.);
#5965=ORIENTED_EDGE('',*,*,#4596,.F.);
#5966=ORIENTED_EDGE('',*,*,#4597,.T.);
#5967=ORIENTED_EDGE('',*,*,#4593,.T.);
#5968=ORIENTED_EDGE('',*,*,#4598,.F.);
#5969=ORIENTED_EDGE('',*,*,#4599,.F.);
#5970=ORIENTED_EDGE('',*,*,#4600,.T.);
#5971=ORIENTED_EDGE('',*,*,#4596,.T.);
#5972=ORIENTED_EDGE('',*,*,#4601,.F.);
#5973=ORIENTED_EDGE('',*,*,#4602,.F.);
#5974=ORIENTED_EDGE('',*,*,#4603,.T.);
#5975=ORIENTED_EDGE('',*,*,#4599,.T.);
#5976=ORIENTED_EDGE('',*,*,#4604,.F.);
#5977=ORIENTED_EDGE('',*,*,#4605,.F.);
#5978=ORIENTED_EDGE('',*,*,#4606,.T.);
#5979=ORIENTED_EDGE('',*,*,#4602,.T.);
#5980=ORIENTED_EDGE('',*,*,#4607,.F.);
#5981=ORIENTED_EDGE('',*,*,#4608,.F.);
#5982=ORIENTED_EDGE('',*,*,#4609,.T.);
#5983=ORIENTED_EDGE('',*,*,#4605,.T.);
#5984=ORIENTED_EDGE('',*,*,#4610,.F.);
#5985=ORIENTED_EDGE('',*,*,#4611,.F.);
#5986=ORIENTED_EDGE('',*,*,#4612,.T.);
#5987=ORIENTED_EDGE('',*,*,#4608,.T.);
#5988=ORIENTED_EDGE('',*,*,#4613,.F.);
#5989=ORIENTED_EDGE('',*,*,#4614,.F.);
#5990=ORIENTED_EDGE('',*,*,#4615,.T.);
#5991=ORIENTED_EDGE('',*,*,#4611,.T.);
#5992=ORIENTED_EDGE('',*,*,#4616,.F.);
#5993=ORIENTED_EDGE('',*,*,#4617,.F.);
#5994=ORIENTED_EDGE('',*,*,#4618,.T.);
#5995=ORIENTED_EDGE('',*,*,#4614,.T.);
#5996=ORIENTED_EDGE('',*,*,#4619,.F.);
#5997=ORIENTED_EDGE('',*,*,#4620,.F.);
#5998=ORIENTED_EDGE('',*,*,#4621,.T.);
#5999=ORIENTED_EDGE('',*,*,#4617,.T.);
#6000=ORIENTED_EDGE('',*,*,#4622,.F.);
#6001=ORIENTED_EDGE('',*,*,#4623,.F.);
#6002=ORIENTED_EDGE('',*,*,#4624,.T.);
#6003=ORIENTED_EDGE('',*,*,#4620,.T.);
#6004=ORIENTED_EDGE('',*,*,#4625,.F.);
#6005=ORIENTED_EDGE('',*,*,#4626,.F.);
#6006=ORIENTED_EDGE('',*,*,#4627,.T.);
#6007=ORIENTED_EDGE('',*,*,#4623,.T.);
#6008=ORIENTED_EDGE('',*,*,#4628,.F.);
#6009=ORIENTED_EDGE('',*,*,#4629,.F.);
#6010=ORIENTED_EDGE('',*,*,#4630,.T.);
#6011=ORIENTED_EDGE('',*,*,#4626,.T.);
#6012=ORIENTED_EDGE('',*,*,#4631,.F.);
#6013=ORIENTED_EDGE('',*,*,#4632,.F.);
#6014=ORIENTED_EDGE('',*,*,#4633,.T.);
#6015=ORIENTED_EDGE('',*,*,#4629,.T.);
#6016=ORIENTED_EDGE('',*,*,#4634,.F.);
#6017=ORIENTED_EDGE('',*,*,#4635,.F.);
#6018=ORIENTED_EDGE('',*,*,#4636,.T.);
#6019=ORIENTED_EDGE('',*,*,#4632,.T.);
#6020=ORIENTED_EDGE('',*,*,#4637,.F.);
#6021=ORIENTED_EDGE('',*,*,#4638,.F.);
#6022=ORIENTED_EDGE('',*,*,#4639,.T.);
#6023=ORIENTED_EDGE('',*,*,#4635,.T.);
#6024=ORIENTED_EDGE('',*,*,#4640,.F.);
#6025=ORIENTED_EDGE('',*,*,#4641,.F.);
#6026=ORIENTED_EDGE('',*,*,#4642,.T.);
#6027=ORIENTED_EDGE('',*,*,#4638,.T.);
#6028=ORIENTED_EDGE('',*,*,#4643,.F.);
#6029=ORIENTED_EDGE('',*,*,#4644,.F.);
#6030=ORIENTED_EDGE('',*,*,#4645,.T.);
#6031=ORIENTED_EDGE('',*,*,#4641,.T.);
#6032=ORIENTED_EDGE('',*,*,#4646,.F.);
#6033=ORIENTED_EDGE('',*,*,#4647,.F.);
#6034=ORIENTED_EDGE('',*,*,#4648,.T.);
#6035=ORIENTED_EDGE('',*,*,#4644,.T.);
#6036=ORIENTED_EDGE('',*,*,#4649,.F.);
#6037=ORIENTED_EDGE('',*,*,#4650,.F.);
#6038=ORIENTED_EDGE('',*,*,#4651,.T.);
#6039=ORIENTED_EDGE('',*,*,#4647,.T.);
#6040=ORIENTED_EDGE('',*,*,#4652,.F.);
#6041=ORIENTED_EDGE('',*,*,#4653,.F.);
#6042=ORIENTED_EDGE('',*,*,#4654,.T.);
#6043=ORIENTED_EDGE('',*,*,#4650,.T.);
#6044=ORIENTED_EDGE('',*,*,#4655,.F.);
#6045=ORIENTED_EDGE('',*,*,#4656,.F.);
#6046=ORIENTED_EDGE('',*,*,#4657,.T.);
#6047=ORIENTED_EDGE('',*,*,#4653,.T.);
#6048=ORIENTED_EDGE('',*,*,#4658,.F.);
#6049=ORIENTED_EDGE('',*,*,#4659,.F.);
#6050=ORIENTED_EDGE('',*,*,#4660,.T.);
#6051=ORIENTED_EDGE('',*,*,#4656,.T.);
#6052=ORIENTED_EDGE('',*,*,#4661,.F.);
#6053=ORIENTED_EDGE('',*,*,#4662,.F.);
#6054=ORIENTED_EDGE('',*,*,#4663,.T.);
#6055=ORIENTED_EDGE('',*,*,#4659,.T.);
#6056=ORIENTED_EDGE('',*,*,#4664,.F.);
#6057=ORIENTED_EDGE('',*,*,#4665,.F.);
#6058=ORIENTED_EDGE('',*,*,#4666,.T.);
#6059=ORIENTED_EDGE('',*,*,#4662,.T.);
#6060=ORIENTED_EDGE('',*,*,#4667,.F.);
#6061=ORIENTED_EDGE('',*,*,#4668,.F.);
#6062=ORIENTED_EDGE('',*,*,#4669,.T.);
#6063=ORIENTED_EDGE('',*,*,#4665,.T.);
#6064=ORIENTED_EDGE('',*,*,#4670,.F.);
#6065=ORIENTED_EDGE('',*,*,#4671,.F.);
#6066=ORIENTED_EDGE('',*,*,#4672,.T.);
#6067=ORIENTED_EDGE('',*,*,#4668,.T.);
#6068=ORIENTED_EDGE('',*,*,#4673,.F.);
#6069=ORIENTED_EDGE('',*,*,#4674,.F.);
#6070=ORIENTED_EDGE('',*,*,#4675,.T.);
#6071=ORIENTED_EDGE('',*,*,#4671,.T.);
#6072=ORIENTED_EDGE('',*,*,#4676,.F.);
#6073=ORIENTED_EDGE('',*,*,#4677,.F.);
#6074=ORIENTED_EDGE('',*,*,#4678,.T.);
#6075=ORIENTED_EDGE('',*,*,#4674,.T.);
#6076=ORIENTED_EDGE('',*,*,#4679,.F.);
#6077=ORIENTED_EDGE('',*,*,#4680,.F.);
#6078=ORIENTED_EDGE('',*,*,#4681,.T.);
#6079=ORIENTED_EDGE('',*,*,#4677,.T.);
#6080=ORIENTED_EDGE('',*,*,#4682,.F.);
#6081=ORIENTED_EDGE('',*,*,#4683,.F.);
#6082=ORIENTED_EDGE('',*,*,#4684,.T.);
#6083=ORIENTED_EDGE('',*,*,#4680,.T.);
#6084=ORIENTED_EDGE('',*,*,#4685,.F.);
#6085=ORIENTED_EDGE('',*,*,#4686,.F.);
#6086=ORIENTED_EDGE('',*,*,#4687,.T.);
#6087=ORIENTED_EDGE('',*,*,#4683,.T.);
#6088=ORIENTED_EDGE('',*,*,#4688,.F.);
#6089=ORIENTED_EDGE('',*,*,#4689,.F.);
#6090=ORIENTED_EDGE('',*,*,#4690,.T.);
#6091=ORIENTED_EDGE('',*,*,#4686,.T.);
#6092=ORIENTED_EDGE('',*,*,#4691,.F.);
#6093=ORIENTED_EDGE('',*,*,#4692,.F.);
#6094=ORIENTED_EDGE('',*,*,#4693,.T.);
#6095=ORIENTED_EDGE('',*,*,#4689,.T.);
#6096=ORIENTED_EDGE('',*,*,#4694,.F.);
#6097=ORIENTED_EDGE('',*,*,#4695,.F.);
#6098=ORIENTED_EDGE('',*,*,#4696,.T.);
#6099=ORIENTED_EDGE('',*,*,#4692,.T.);
#6100=ORIENTED_EDGE('',*,*,#4697,.F.);
#6101=ORIENTED_EDGE('',*,*,#4698,.F.);
#6102=ORIENTED_EDGE('',*,*,#4699,.T.);
#6103=ORIENTED_EDGE('',*,*,#4695,.T.);
#6104=ORIENTED_EDGE('',*,*,#4700,.F.);
#6105=ORIENTED_EDGE('',*,*,#4701,.F.);
#6106=ORIENTED_EDGE('',*,*,#4702,.T.);
#6107=ORIENTED_EDGE('',*,*,#4698,.T.);
#6108=ORIENTED_EDGE('',*,*,#4703,.F.);
#6109=ORIENTED_EDGE('',*,*,#4704,.F.);
#6110=ORIENTED_EDGE('',*,*,#4705,.T.);
#6111=ORIENTED_EDGE('',*,*,#4701,.T.);
#6112=ORIENTED_EDGE('',*,*,#4706,.F.);
#6113=ORIENTED_EDGE('',*,*,#4707,.F.);
#6114=ORIENTED_EDGE('',*,*,#4708,.T.);
#6115=ORIENTED_EDGE('',*,*,#4704,.T.);
#6116=ORIENTED_EDGE('',*,*,#4709,.F.);
#6117=ORIENTED_EDGE('',*,*,#4710,.F.);
#6118=ORIENTED_EDGE('',*,*,#4711,.T.);
#6119=ORIENTED_EDGE('',*,*,#4707,.T.);
#6120=ORIENTED_EDGE('',*,*,#4712,.F.);
#6121=ORIENTED_EDGE('',*,*,#4713,.F.);
#6122=ORIENTED_EDGE('',*,*,#4714,.T.);
#6123=ORIENTED_EDGE('',*,*,#4710,.T.);
#6124=ORIENTED_EDGE('',*,*,#4715,.F.);
#6125=ORIENTED_EDGE('',*,*,#4716,.F.);
#6126=ORIENTED_EDGE('',*,*,#4717,.T.);
#6127=ORIENTED_EDGE('',*,*,#4713,.T.);
#6128=ORIENTED_EDGE('',*,*,#4718,.F.);
#6129=ORIENTED_EDGE('',*,*,#4719,.F.);
#6130=ORIENTED_EDGE('',*,*,#4720,.T.);
#6131=ORIENTED_EDGE('',*,*,#4716,.T.);
#6132=ORIENTED_EDGE('',*,*,#4721,.F.);
#6133=ORIENTED_EDGE('',*,*,#4722,.F.);
#6134=ORIENTED_EDGE('',*,*,#4723,.T.);
#6135=ORIENTED_EDGE('',*,*,#4719,.T.);
#6136=ORIENTED_EDGE('',*,*,#4724,.F.);
#6137=ORIENTED_EDGE('',*,*,#4725,.F.);
#6138=ORIENTED_EDGE('',*,*,#4726,.T.);
#6139=ORIENTED_EDGE('',*,*,#4722,.T.);
#6140=ORIENTED_EDGE('',*,*,#4727,.F.);
#6141=ORIENTED_EDGE('',*,*,#4728,.F.);
#6142=ORIENTED_EDGE('',*,*,#4729,.T.);
#6143=ORIENTED_EDGE('',*,*,#4725,.T.);
#6144=ORIENTED_EDGE('',*,*,#4730,.F.);
#6145=ORIENTED_EDGE('',*,*,#4731,.F.);
#6146=ORIENTED_EDGE('',*,*,#4732,.T.);
#6147=ORIENTED_EDGE('',*,*,#4728,.T.);
#6148=ORIENTED_EDGE('',*,*,#4733,.F.);
#6149=ORIENTED_EDGE('',*,*,#4734,.F.);
#6150=ORIENTED_EDGE('',*,*,#4735,.T.);
#6151=ORIENTED_EDGE('',*,*,#4731,.T.);
#6152=ORIENTED_EDGE('',*,*,#4736,.F.);
#6153=ORIENTED_EDGE('',*,*,#4737,.F.);
#6154=ORIENTED_EDGE('',*,*,#4738,.T.);
#6155=ORIENTED_EDGE('',*,*,#4734,.T.);
#6156=ORIENTED_EDGE('',*,*,#4739,.F.);
#6157=ORIENTED_EDGE('',*,*,#4740,.F.);
#6158=ORIENTED_EDGE('',*,*,#4741,.T.);
#6159=ORIENTED_EDGE('',*,*,#4737,.T.);
#6160=ORIENTED_EDGE('',*,*,#4742,.F.);
#6161=ORIENTED_EDGE('',*,*,#4743,.F.);
#6162=ORIENTED_EDGE('',*,*,#4744,.T.);
#6163=ORIENTED_EDGE('',*,*,#4740,.T.);
#6164=ORIENTED_EDGE('',*,*,#4745,.F.);
#6165=ORIENTED_EDGE('',*,*,#4746,.F.);
#6166=ORIENTED_EDGE('',*,*,#4747,.T.);
#6167=ORIENTED_EDGE('',*,*,#4743,.T.);
#6168=ORIENTED_EDGE('',*,*,#4748,.F.);
#6169=ORIENTED_EDGE('',*,*,#4749,.F.);
#6170=ORIENTED_EDGE('',*,*,#4750,.T.);
#6171=ORIENTED_EDGE('',*,*,#4746,.T.);
#6172=ORIENTED_EDGE('',*,*,#4751,.F.);
#6173=ORIENTED_EDGE('',*,*,#4752,.F.);
#6174=ORIENTED_EDGE('',*,*,#4753,.T.);
#6175=ORIENTED_EDGE('',*,*,#4749,.T.);
#6176=ORIENTED_EDGE('',*,*,#4754,.F.);
#6177=ORIENTED_EDGE('',*,*,#4755,.F.);
#6178=ORIENTED_EDGE('',*,*,#4756,.T.);
#6179=ORIENTED_EDGE('',*,*,#4752,.T.);
#6180=ORIENTED_EDGE('',*,*,#4757,.F.);
#6181=ORIENTED_EDGE('',*,*,#4758,.F.);
#6182=ORIENTED_EDGE('',*,*,#4759,.T.);
#6183=ORIENTED_EDGE('',*,*,#4755,.T.);
#6184=ORIENTED_EDGE('',*,*,#4760,.F.);
#6185=ORIENTED_EDGE('',*,*,#4761,.F.);
#6186=ORIENTED_EDGE('',*,*,#4762,.T.);
#6187=ORIENTED_EDGE('',*,*,#4758,.T.);
#6188=ORIENTED_EDGE('',*,*,#4763,.F.);
#6189=ORIENTED_EDGE('',*,*,#4764,.F.);
#6190=ORIENTED_EDGE('',*,*,#4765,.T.);
#6191=ORIENTED_EDGE('',*,*,#4761,.T.);
#6192=ORIENTED_EDGE('',*,*,#4766,.F.);
#6193=ORIENTED_EDGE('',*,*,#4767,.F.);
#6194=ORIENTED_EDGE('',*,*,#4768,.T.);
#6195=ORIENTED_EDGE('',*,*,#4764,.T.);
#6196=ORIENTED_EDGE('',*,*,#4769,.F.);
#6197=ORIENTED_EDGE('',*,*,#4770,.F.);
#6198=ORIENTED_EDGE('',*,*,#4771,.T.);
#6199=ORIENTED_EDGE('',*,*,#4767,.T.);
#6200=ORIENTED_EDGE('',*,*,#4772,.F.);
#6201=ORIENTED_EDGE('',*,*,#4773,.F.);
#6202=ORIENTED_EDGE('',*,*,#4774,.T.);
#6203=ORIENTED_EDGE('',*,*,#4770,.T.);
#6204=ORIENTED_EDGE('',*,*,#4775,.F.);
#6205=ORIENTED_EDGE('',*,*,#4776,.F.);
#6206=ORIENTED_EDGE('',*,*,#4777,.T.);
#6207=ORIENTED_EDGE('',*,*,#4773,.T.);
#6208=ORIENTED_EDGE('',*,*,#4778,.F.);
#6209=ORIENTED_EDGE('',*,*,#4779,.F.);
#6210=ORIENTED_EDGE('',*,*,#4780,.T.);
#6211=ORIENTED_EDGE('',*,*,#4776,.T.);
#6212=ORIENTED_EDGE('',*,*,#4781,.F.);
#6213=ORIENTED_EDGE('',*,*,#4782,.F.);
#6214=ORIENTED_EDGE('',*,*,#4783,.T.);
#6215=ORIENTED_EDGE('',*,*,#4779,.T.);
#6216=ORIENTED_EDGE('',*,*,#4784,.F.);
#6217=ORIENTED_EDGE('',*,*,#4785,.F.);
#6218=ORIENTED_EDGE('',*,*,#4786,.T.);
#6219=ORIENTED_EDGE('',*,*,#4782,.T.);
#6220=ORIENTED_EDGE('',*,*,#4787,.F.);
#6221=ORIENTED_EDGE('',*,*,#4788,.F.);
#6222=ORIENTED_EDGE('',*,*,#4789,.T.);
#6223=ORIENTED_EDGE('',*,*,#4785,.T.);
#6224=ORIENTED_EDGE('',*,*,#4790,.F.);
#6225=ORIENTED_EDGE('',*,*,#4791,.F.);
#6226=ORIENTED_EDGE('',*,*,#4792,.T.);
#6227=ORIENTED_EDGE('',*,*,#4788,.T.);
#6228=ORIENTED_EDGE('',*,*,#4793,.F.);
#6229=ORIENTED_EDGE('',*,*,#4794,.F.);
#6230=ORIENTED_EDGE('',*,*,#4795,.T.);
#6231=ORIENTED_EDGE('',*,*,#4791,.T.);
#6232=ORIENTED_EDGE('',*,*,#4796,.F.);
#6233=ORIENTED_EDGE('',*,*,#4797,.F.);
#6234=ORIENTED_EDGE('',*,*,#4798,.T.);
#6235=ORIENTED_EDGE('',*,*,#4794,.T.);
#6236=ORIENTED_EDGE('',*,*,#4799,.F.);
#6237=ORIENTED_EDGE('',*,*,#4800,.F.);
#6238=ORIENTED_EDGE('',*,*,#4801,.T.);
#6239=ORIENTED_EDGE('',*,*,#4797,.T.);
#6240=ORIENTED_EDGE('',*,*,#4802,.F.);
#6241=ORIENTED_EDGE('',*,*,#4803,.F.);
#6242=ORIENTED_EDGE('',*,*,#4804,.T.);
#6243=ORIENTED_EDGE('',*,*,#4800,.T.);
#6244=ORIENTED_EDGE('',*,*,#4805,.F.);
#6245=ORIENTED_EDGE('',*,*,#4806,.F.);
#6246=ORIENTED_EDGE('',*,*,#4807,.T.);
#6247=ORIENTED_EDGE('',*,*,#4803,.T.);
#6248=ORIENTED_EDGE('',*,*,#4808,.F.);
#6249=ORIENTED_EDGE('',*,*,#4809,.F.);
#6250=ORIENTED_EDGE('',*,*,#4810,.T.);
#6251=ORIENTED_EDGE('',*,*,#4806,.T.);
#6252=ORIENTED_EDGE('',*,*,#4811,.F.);
#6253=ORIENTED_EDGE('',*,*,#4812,.F.);
#6254=ORIENTED_EDGE('',*,*,#4813,.T.);
#6255=ORIENTED_EDGE('',*,*,#4809,.T.);
#6256=ORIENTED_EDGE('',*,*,#4814,.F.);
#6257=ORIENTED_EDGE('',*,*,#4815,.F.);
#6258=ORIENTED_EDGE('',*,*,#4816,.T.);
#6259=ORIENTED_EDGE('',*,*,#4812,.T.);
#6260=ORIENTED_EDGE('',*,*,#4817,.F.);
#6261=ORIENTED_EDGE('',*,*,#4818,.F.);
#6262=ORIENTED_EDGE('',*,*,#4819,.T.);
#6263=ORIENTED_EDGE('',*,*,#4815,.T.);
#6264=ORIENTED_EDGE('',*,*,#4820,.F.);
#6265=ORIENTED_EDGE('',*,*,#4821,.F.);
#6266=ORIENTED_EDGE('',*,*,#4822,.T.);
#6267=ORIENTED_EDGE('',*,*,#4818,.T.);
#6268=ORIENTED_EDGE('',*,*,#4823,.F.);
#6269=ORIENTED_EDGE('',*,*,#4824,.F.);
#6270=ORIENTED_EDGE('',*,*,#4825,.T.);
#6271=ORIENTED_EDGE('',*,*,#4821,.T.);
#6272=ORIENTED_EDGE('',*,*,#4826,.F.);
#6273=ORIENTED_EDGE('',*,*,#4827,.F.);
#6274=ORIENTED_EDGE('',*,*,#4828,.T.);
#6275=ORIENTED_EDGE('',*,*,#4824,.T.);
#6276=ORIENTED_EDGE('',*,*,#4829,.F.);
#6277=ORIENTED_EDGE('',*,*,#4830,.F.);
#6278=ORIENTED_EDGE('',*,*,#4831,.T.);
#6279=ORIENTED_EDGE('',*,*,#4827,.T.);
#6280=ORIENTED_EDGE('',*,*,#4832,.F.);
#6281=ORIENTED_EDGE('',*,*,#4833,.F.);
#6282=ORIENTED_EDGE('',*,*,#4834,.T.);
#6283=ORIENTED_EDGE('',*,*,#4830,.T.);
#6284=ORIENTED_EDGE('',*,*,#4835,.F.);
#6285=ORIENTED_EDGE('',*,*,#4836,.F.);
#6286=ORIENTED_EDGE('',*,*,#4837,.T.);
#6287=ORIENTED_EDGE('',*,*,#4833,.T.);
#6288=ORIENTED_EDGE('',*,*,#4838,.F.);
#6289=ORIENTED_EDGE('',*,*,#4839,.F.);
#6290=ORIENTED_EDGE('',*,*,#4840,.T.);
#6291=ORIENTED_EDGE('',*,*,#4836,.T.);
#6292=ORIENTED_EDGE('',*,*,#4841,.F.);
#6293=ORIENTED_EDGE('',*,*,#4842,.F.);
#6294=ORIENTED_EDGE('',*,*,#4843,.T.);
#6295=ORIENTED_EDGE('',*,*,#4839,.T.);
#6296=ORIENTED_EDGE('',*,*,#4844,.F.);
#6297=ORIENTED_EDGE('',*,*,#4845,.F.);
#6298=ORIENTED_EDGE('',*,*,#4846,.T.);
#6299=ORIENTED_EDGE('',*,*,#4842,.T.);
#6300=ORIENTED_EDGE('',*,*,#4847,.F.);
#6301=ORIENTED_EDGE('',*,*,#4848,.F.);
#6302=ORIENTED_EDGE('',*,*,#4849,.T.);
#6303=ORIENTED_EDGE('',*,*,#4845,.T.);
#6304=ORIENTED_EDGE('',*,*,#4850,.F.);
#6305=ORIENTED_EDGE('',*,*,#4851,.F.);
#6306=ORIENTED_EDGE('',*,*,#4852,.T.);
#6307=ORIENTED_EDGE('',*,*,#4848,.T.);
#6308=ORIENTED_EDGE('',*,*,#4853,.F.);
#6309=ORIENTED_EDGE('',*,*,#4854,.F.);
#6310=ORIENTED_EDGE('',*,*,#4855,.T.);
#6311=ORIENTED_EDGE('',*,*,#4851,.T.);
#6312=ORIENTED_EDGE('',*,*,#4856,.F.);
#6313=ORIENTED_EDGE('',*,*,#4857,.F.);
#6314=ORIENTED_EDGE('',*,*,#4858,.T.);
#6315=ORIENTED_EDGE('',*,*,#4854,.T.);
#6316=ORIENTED_EDGE('',*,*,#4859,.F.);
#6317=ORIENTED_EDGE('',*,*,#4860,.F.);
#6318=ORIENTED_EDGE('',*,*,#4861,.T.);
#6319=ORIENTED_EDGE('',*,*,#4857,.T.);
#6320=ORIENTED_EDGE('',*,*,#4862,.F.);
#6321=ORIENTED_EDGE('',*,*,#4863,.F.);
#6322=ORIENTED_EDGE('',*,*,#4864,.T.);
#6323=ORIENTED_EDGE('',*,*,#4860,.T.);
#6324=ORIENTED_EDGE('',*,*,#4865,.F.);
#6325=ORIENTED_EDGE('',*,*,#4866,.F.);
#6326=ORIENTED_EDGE('',*,*,#4867,.T.);
#6327=ORIENTED_EDGE('',*,*,#4868,.F.);
#6328=ORIENTED_EDGE('',*,*,#4867,.F.);
#6329=ORIENTED_EDGE('',*,*,#4869,.F.);
#6330=ORIENTED_EDGE('',*,*,#4870,.T.);
#6331=ORIENTED_EDGE('',*,*,#4871,.F.);
#6332=ORIENTED_EDGE('',*,*,#4870,.F.);
#6333=ORIENTED_EDGE('',*,*,#4872,.F.);
#6334=ORIENTED_EDGE('',*,*,#4873,.T.);
#6335=ORIENTED_EDGE('',*,*,#4874,.F.);
#6336=ORIENTED_EDGE('',*,*,#4873,.F.);
#6337=ORIENTED_EDGE('',*,*,#4875,.F.);
#6338=ORIENTED_EDGE('',*,*,#4876,.T.);
#6339=ORIENTED_EDGE('',*,*,#4877,.F.);
#6340=ORIENTED_EDGE('',*,*,#4876,.F.);
#6341=ORIENTED_EDGE('',*,*,#4878,.F.);
#6342=ORIENTED_EDGE('',*,*,#4879,.T.);
#6343=ORIENTED_EDGE('',*,*,#4880,.F.);
#6344=ORIENTED_EDGE('',*,*,#4879,.F.);
#6345=ORIENTED_EDGE('',*,*,#4881,.F.);
#6346=ORIENTED_EDGE('',*,*,#4882,.T.);
#6347=ORIENTED_EDGE('',*,*,#4883,.F.);
#6348=ORIENTED_EDGE('',*,*,#4882,.F.);
#6349=ORIENTED_EDGE('',*,*,#4884,.T.);
#6350=ORIENTED_EDGE('',*,*,#4868,.T.);
#6351=ORIENTED_EDGE('',*,*,#4871,.T.);
#6352=ORIENTED_EDGE('',*,*,#4885,.T.);
#6353=ORIENTED_EDGE('',*,*,#4302,.F.);
#6354=ORIENTED_EDGE('',*,*,#4886,.T.);
#6355=ORIENTED_EDGE('',*,*,#4887,.T.);
#6356=ORIENTED_EDGE('',*,*,#4883,.T.);
#6357=ORIENTED_EDGE('',*,*,#4880,.T.);
#6358=ORIENTED_EDGE('',*,*,#4877,.T.);
#6359=ORIENTED_EDGE('',*,*,#4874,.T.);
#6360=ORIENTED_EDGE('',*,*,#4884,.F.);
#6361=ORIENTED_EDGE('',*,*,#4888,.T.);
#6362=ORIENTED_EDGE('',*,*,#4889,.T.);
#6363=ORIENTED_EDGE('',*,*,#4888,.F.);
#6364=ORIENTED_EDGE('',*,*,#4889,.F.);
#6365=ORIENTED_EDGE('',*,*,#4866,.T.);
#6366=ORIENTED_EDGE('',*,*,#4869,.T.);
#6367=ORIENTED_EDGE('',*,*,#4872,.T.);
#6368=ORIENTED_EDGE('',*,*,#4875,.T.);
#6369=ORIENTED_EDGE('',*,*,#4878,.T.);
#6370=ORIENTED_EDGE('',*,*,#4881,.T.);
#6371=ORIENTED_EDGE('',*,*,#4890,.F.);
#6372=ORIENTED_EDGE('',*,*,#4891,.F.);
#6373=ORIENTED_EDGE('',*,*,#4582,.F.);
#6374=ORIENTED_EDGE('',*,*,#4579,.F.);
#6375=ORIENTED_EDGE('',*,*,#4576,.F.);
#6376=ORIENTED_EDGE('',*,*,#4573,.F.);
#6377=ORIENTED_EDGE('',*,*,#4570,.F.);
#6378=ORIENTED_EDGE('',*,*,#4567,.F.);
#6379=ORIENTED_EDGE('',*,*,#4564,.F.);
#6380=ORIENTED_EDGE('',*,*,#4561,.F.);
#6381=ORIENTED_EDGE('',*,*,#4558,.F.);
#6382=ORIENTED_EDGE('',*,*,#4555,.F.);
#6383=ORIENTED_EDGE('',*,*,#4552,.F.);
#6384=ORIENTED_EDGE('',*,*,#4549,.F.);
#6385=ORIENTED_EDGE('',*,*,#4546,.F.);
#6386=ORIENTED_EDGE('',*,*,#4543,.F.);
#6387=ORIENTED_EDGE('',*,*,#4540,.F.);
#6388=ORIENTED_EDGE('',*,*,#4537,.F.);
#6389=ORIENTED_EDGE('',*,*,#4534,.F.);
#6390=ORIENTED_EDGE('',*,*,#4531,.F.);
#6391=ORIENTED_EDGE('',*,*,#4528,.F.);
#6392=ORIENTED_EDGE('',*,*,#4525,.F.);
#6393=ORIENTED_EDGE('',*,*,#4522,.F.);
#6394=ORIENTED_EDGE('',*,*,#4519,.F.);
#6395=ORIENTED_EDGE('',*,*,#4516,.F.);
#6396=ORIENTED_EDGE('',*,*,#4513,.F.);
#6397=ORIENTED_EDGE('',*,*,#4510,.F.);
#6398=ORIENTED_EDGE('',*,*,#4507,.F.);
#6399=ORIENTED_EDGE('',*,*,#4504,.F.);
#6400=ORIENTED_EDGE('',*,*,#4501,.F.);
#6401=ORIENTED_EDGE('',*,*,#4498,.F.);
#6402=ORIENTED_EDGE('',*,*,#4495,.F.);
#6403=ORIENTED_EDGE('',*,*,#4492,.F.);
#6404=ORIENTED_EDGE('',*,*,#4489,.F.);
#6405=ORIENTED_EDGE('',*,*,#4486,.F.);
#6406=ORIENTED_EDGE('',*,*,#4483,.F.);
#6407=ORIENTED_EDGE('',*,*,#4480,.F.);
#6408=ORIENTED_EDGE('',*,*,#4477,.F.);
#6409=ORIENTED_EDGE('',*,*,#4474,.F.);
#6410=ORIENTED_EDGE('',*,*,#4471,.F.);
#6411=ORIENTED_EDGE('',*,*,#4468,.F.);
#6412=ORIENTED_EDGE('',*,*,#4465,.F.);
#6413=ORIENTED_EDGE('',*,*,#4462,.F.);
#6414=ORIENTED_EDGE('',*,*,#4459,.F.);
#6415=ORIENTED_EDGE('',*,*,#4456,.F.);
#6416=ORIENTED_EDGE('',*,*,#4453,.F.);
#6417=ORIENTED_EDGE('',*,*,#4450,.F.);
#6418=ORIENTED_EDGE('',*,*,#4447,.F.);
#6419=ORIENTED_EDGE('',*,*,#4444,.F.);
#6420=ORIENTED_EDGE('',*,*,#4441,.F.);
#6421=ORIENTED_EDGE('',*,*,#4438,.F.);
#6422=ORIENTED_EDGE('',*,*,#4435,.F.);
#6423=ORIENTED_EDGE('',*,*,#4432,.F.);
#6424=ORIENTED_EDGE('',*,*,#4429,.F.);
#6425=ORIENTED_EDGE('',*,*,#4426,.F.);
#6426=ORIENTED_EDGE('',*,*,#4423,.F.);
#6427=ORIENTED_EDGE('',*,*,#4420,.F.);
#6428=ORIENTED_EDGE('',*,*,#4417,.F.);
#6429=ORIENTED_EDGE('',*,*,#4414,.F.);
#6430=ORIENTED_EDGE('',*,*,#4411,.F.);
#6431=ORIENTED_EDGE('',*,*,#4408,.F.);
#6432=ORIENTED_EDGE('',*,*,#4405,.F.);
#6433=ORIENTED_EDGE('',*,*,#4402,.F.);
#6434=ORIENTED_EDGE('',*,*,#4399,.F.);
#6435=ORIENTED_EDGE('',*,*,#4396,.F.);
#6436=ORIENTED_EDGE('',*,*,#4393,.F.);
#6437=ORIENTED_EDGE('',*,*,#4390,.F.);
#6438=ORIENTED_EDGE('',*,*,#4387,.F.);
#6439=ORIENTED_EDGE('',*,*,#4384,.F.);
#6440=ORIENTED_EDGE('',*,*,#4381,.F.);
#6441=ORIENTED_EDGE('',*,*,#4378,.F.);
#6442=ORIENTED_EDGE('',*,*,#4375,.F.);
#6443=ORIENTED_EDGE('',*,*,#4372,.F.);
#6444=ORIENTED_EDGE('',*,*,#4369,.F.);
#6445=ORIENTED_EDGE('',*,*,#4366,.F.);
#6446=ORIENTED_EDGE('',*,*,#4363,.F.);
#6447=ORIENTED_EDGE('',*,*,#4360,.F.);
#6448=ORIENTED_EDGE('',*,*,#4357,.F.);
#6449=ORIENTED_EDGE('',*,*,#4354,.F.);
#6450=ORIENTED_EDGE('',*,*,#4351,.F.);
#6451=ORIENTED_EDGE('',*,*,#4348,.F.);
#6452=ORIENTED_EDGE('',*,*,#4345,.F.);
#6453=ORIENTED_EDGE('',*,*,#4342,.F.);
#6454=ORIENTED_EDGE('',*,*,#4339,.F.);
#6455=ORIENTED_EDGE('',*,*,#4336,.F.);
#6456=ORIENTED_EDGE('',*,*,#4333,.F.);
#6457=ORIENTED_EDGE('',*,*,#4330,.F.);
#6458=ORIENTED_EDGE('',*,*,#4327,.F.);
#6459=ORIENTED_EDGE('',*,*,#4324,.F.);
#6460=ORIENTED_EDGE('',*,*,#4321,.F.);
#6461=ORIENTED_EDGE('',*,*,#4318,.F.);
#6462=ORIENTED_EDGE('',*,*,#4315,.F.);
#6463=ORIENTED_EDGE('',*,*,#4312,.F.);
#6464=ORIENTED_EDGE('',*,*,#4309,.F.);
#6465=ORIENTED_EDGE('',*,*,#4306,.F.);
#6466=ORIENTED_EDGE('',*,*,#4303,.F.);
#6467=ORIENTED_EDGE('',*,*,#4885,.F.);
#6468=ORIENTED_EDGE('',*,*,#4892,.T.);
#6469=ORIENTED_EDGE('',*,*,#4865,.T.);
#6470=ORIENTED_EDGE('',*,*,#4862,.T.);
#6471=ORIENTED_EDGE('',*,*,#4859,.T.);
#6472=ORIENTED_EDGE('',*,*,#4856,.T.);
#6473=ORIENTED_EDGE('',*,*,#4853,.T.);
#6474=ORIENTED_EDGE('',*,*,#4850,.T.);
#6475=ORIENTED_EDGE('',*,*,#4847,.T.);
#6476=ORIENTED_EDGE('',*,*,#4844,.T.);
#6477=ORIENTED_EDGE('',*,*,#4841,.T.);
#6478=ORIENTED_EDGE('',*,*,#4838,.T.);
#6479=ORIENTED_EDGE('',*,*,#4835,.T.);
#6480=ORIENTED_EDGE('',*,*,#4832,.T.);
#6481=ORIENTED_EDGE('',*,*,#4829,.T.);
#6482=ORIENTED_EDGE('',*,*,#4826,.T.);
#6483=ORIENTED_EDGE('',*,*,#4823,.T.);
#6484=ORIENTED_EDGE('',*,*,#4820,.T.);
#6485=ORIENTED_EDGE('',*,*,#4817,.T.);
#6486=ORIENTED_EDGE('',*,*,#4814,.T.);
#6487=ORIENTED_EDGE('',*,*,#4811,.T.);
#6488=ORIENTED_EDGE('',*,*,#4808,.T.);
#6489=ORIENTED_EDGE('',*,*,#4805,.T.);
#6490=ORIENTED_EDGE('',*,*,#4802,.T.);
#6491=ORIENTED_EDGE('',*,*,#4799,.T.);
#6492=ORIENTED_EDGE('',*,*,#4796,.T.);
#6493=ORIENTED_EDGE('',*,*,#4793,.T.);
#6494=ORIENTED_EDGE('',*,*,#4790,.T.);
#6495=ORIENTED_EDGE('',*,*,#4787,.T.);
#6496=ORIENTED_EDGE('',*,*,#4784,.T.);
#6497=ORIENTED_EDGE('',*,*,#4781,.T.);
#6498=ORIENTED_EDGE('',*,*,#4778,.T.);
#6499=ORIENTED_EDGE('',*,*,#4775,.T.);
#6500=ORIENTED_EDGE('',*,*,#4772,.T.);
#6501=ORIENTED_EDGE('',*,*,#4769,.T.);
#6502=ORIENTED_EDGE('',*,*,#4766,.T.);
#6503=ORIENTED_EDGE('',*,*,#4763,.T.);
#6504=ORIENTED_EDGE('',*,*,#4760,.T.);
#6505=ORIENTED_EDGE('',*,*,#4757,.T.);
#6506=ORIENTED_EDGE('',*,*,#4754,.T.);
#6507=ORIENTED_EDGE('',*,*,#4751,.T.);
#6508=ORIENTED_EDGE('',*,*,#4748,.T.);
#6509=ORIENTED_EDGE('',*,*,#4745,.T.);
#6510=ORIENTED_EDGE('',*,*,#4742,.T.);
#6511=ORIENTED_EDGE('',*,*,#4739,.T.);
#6512=ORIENTED_EDGE('',*,*,#4736,.T.);
#6513=ORIENTED_EDGE('',*,*,#4733,.T.);
#6514=ORIENTED_EDGE('',*,*,#4730,.T.);
#6515=ORIENTED_EDGE('',*,*,#4727,.T.);
#6516=ORIENTED_EDGE('',*,*,#4724,.T.);
#6517=ORIENTED_EDGE('',*,*,#4721,.T.);
#6518=ORIENTED_EDGE('',*,*,#4718,.T.);
#6519=ORIENTED_EDGE('',*,*,#4715,.T.);
#6520=ORIENTED_EDGE('',*,*,#4712,.T.);
#6521=ORIENTED_EDGE('',*,*,#4709,.T.);
#6522=ORIENTED_EDGE('',*,*,#4706,.T.);
#6523=ORIENTED_EDGE('',*,*,#4703,.T.);
#6524=ORIENTED_EDGE('',*,*,#4700,.T.);
#6525=ORIENTED_EDGE('',*,*,#4697,.T.);
#6526=ORIENTED_EDGE('',*,*,#4694,.T.);
#6527=ORIENTED_EDGE('',*,*,#4691,.T.);
#6528=ORIENTED_EDGE('',*,*,#4688,.T.);
#6529=ORIENTED_EDGE('',*,*,#4685,.T.);
#6530=ORIENTED_EDGE('',*,*,#4682,.T.);
#6531=ORIENTED_EDGE('',*,*,#4679,.T.);
#6532=ORIENTED_EDGE('',*,*,#4676,.T.);
#6533=ORIENTED_EDGE('',*,*,#4673,.T.);
#6534=ORIENTED_EDGE('',*,*,#4670,.T.);
#6535=ORIENTED_EDGE('',*,*,#4667,.T.);
#6536=ORIENTED_EDGE('',*,*,#4664,.T.);
#6537=ORIENTED_EDGE('',*,*,#4661,.T.);
#6538=ORIENTED_EDGE('',*,*,#4658,.T.);
#6539=ORIENTED_EDGE('',*,*,#4655,.T.);
#6540=ORIENTED_EDGE('',*,*,#4652,.T.);
#6541=ORIENTED_EDGE('',*,*,#4649,.T.);
#6542=ORIENTED_EDGE('',*,*,#4646,.T.);
#6543=ORIENTED_EDGE('',*,*,#4643,.T.);
#6544=ORIENTED_EDGE('',*,*,#4640,.T.);
#6545=ORIENTED_EDGE('',*,*,#4637,.T.);
#6546=ORIENTED_EDGE('',*,*,#4634,.T.);
#6547=ORIENTED_EDGE('',*,*,#4631,.T.);
#6548=ORIENTED_EDGE('',*,*,#4628,.T.);
#6549=ORIENTED_EDGE('',*,*,#4625,.T.);
#6550=ORIENTED_EDGE('',*,*,#4622,.T.);
#6551=ORIENTED_EDGE('',*,*,#4619,.T.);
#6552=ORIENTED_EDGE('',*,*,#4616,.T.);
#6553=ORIENTED_EDGE('',*,*,#4613,.T.);
#6554=ORIENTED_EDGE('',*,*,#4610,.T.);
#6555=ORIENTED_EDGE('',*,*,#4607,.T.);
#6556=ORIENTED_EDGE('',*,*,#4604,.T.);
#6557=ORIENTED_EDGE('',*,*,#4601,.T.);
#6558=ORIENTED_EDGE('',*,*,#4598,.T.);
#6559=ORIENTED_EDGE('',*,*,#4595,.T.);
#6560=ORIENTED_EDGE('',*,*,#4592,.T.);
#6561=ORIENTED_EDGE('',*,*,#4589,.T.);
#6562=ORIENTED_EDGE('',*,*,#4586,.T.);
#6563=ORIENTED_EDGE('',*,*,#4863,.T.);
#6564=ORIENTED_EDGE('',*,*,#4892,.F.);
#6565=ORIENTED_EDGE('',*,*,#4887,.F.);
#6566=ORIENTED_EDGE('',*,*,#4893,.T.);
#6567=ORIENTED_EDGE('',*,*,#4894,.F.);
#6568=ORIENTED_EDGE('',*,*,#4584,.F.);
#6569=ORIENTED_EDGE('',*,*,#4588,.F.);
#6570=ORIENTED_EDGE('',*,*,#4591,.F.);
#6571=ORIENTED_EDGE('',*,*,#4594,.F.);
#6572=ORIENTED_EDGE('',*,*,#4597,.F.);
#6573=ORIENTED_EDGE('',*,*,#4600,.F.);
#6574=ORIENTED_EDGE('',*,*,#4603,.F.);
#6575=ORIENTED_EDGE('',*,*,#4606,.F.);
#6576=ORIENTED_EDGE('',*,*,#4609,.F.);
#6577=ORIENTED_EDGE('',*,*,#4612,.F.);
#6578=ORIENTED_EDGE('',*,*,#4615,.F.);
#6579=ORIENTED_EDGE('',*,*,#4618,.F.);
#6580=ORIENTED_EDGE('',*,*,#4621,.F.);
#6581=ORIENTED_EDGE('',*,*,#4624,.F.);
#6582=ORIENTED_EDGE('',*,*,#4627,.F.);
#6583=ORIENTED_EDGE('',*,*,#4630,.F.);
#6584=ORIENTED_EDGE('',*,*,#4633,.F.);
#6585=ORIENTED_EDGE('',*,*,#4636,.F.);
#6586=ORIENTED_EDGE('',*,*,#4639,.F.);
#6587=ORIENTED_EDGE('',*,*,#4642,.F.);
#6588=ORIENTED_EDGE('',*,*,#4645,.F.);
#6589=ORIENTED_EDGE('',*,*,#4648,.F.);
#6590=ORIENTED_EDGE('',*,*,#4651,.F.);
#6591=ORIENTED_EDGE('',*,*,#4654,.F.);
#6592=ORIENTED_EDGE('',*,*,#4657,.F.);
#6593=ORIENTED_EDGE('',*,*,#4660,.F.);
#6594=ORIENTED_EDGE('',*,*,#4663,.F.);
#6595=ORIENTED_EDGE('',*,*,#4666,.F.);
#6596=ORIENTED_EDGE('',*,*,#4669,.F.);
#6597=ORIENTED_EDGE('',*,*,#4672,.F.);
#6598=ORIENTED_EDGE('',*,*,#4675,.F.);
#6599=ORIENTED_EDGE('',*,*,#4678,.F.);
#6600=ORIENTED_EDGE('',*,*,#4681,.F.);
#6601=ORIENTED_EDGE('',*,*,#4684,.F.);
#6602=ORIENTED_EDGE('',*,*,#4687,.F.);
#6603=ORIENTED_EDGE('',*,*,#4690,.F.);
#6604=ORIENTED_EDGE('',*,*,#4693,.F.);
#6605=ORIENTED_EDGE('',*,*,#4696,.F.);
#6606=ORIENTED_EDGE('',*,*,#4699,.F.);
#6607=ORIENTED_EDGE('',*,*,#4702,.F.);
#6608=ORIENTED_EDGE('',*,*,#4705,.F.);
#6609=ORIENTED_EDGE('',*,*,#4708,.F.);
#6610=ORIENTED_EDGE('',*,*,#4711,.F.);
#6611=ORIENTED_EDGE('',*,*,#4714,.F.);
#6612=ORIENTED_EDGE('',*,*,#4717,.F.);
#6613=ORIENTED_EDGE('',*,*,#4720,.F.);
#6614=ORIENTED_EDGE('',*,*,#4723,.F.);
#6615=ORIENTED_EDGE('',*,*,#4726,.F.);
#6616=ORIENTED_EDGE('',*,*,#4729,.F.);
#6617=ORIENTED_EDGE('',*,*,#4732,.F.);
#6618=ORIENTED_EDGE('',*,*,#4735,.F.);
#6619=ORIENTED_EDGE('',*,*,#4738,.F.);
#6620=ORIENTED_EDGE('',*,*,#4741,.F.);
#6621=ORIENTED_EDGE('',*,*,#4744,.F.);
#6622=ORIENTED_EDGE('',*,*,#4747,.F.);
#6623=ORIENTED_EDGE('',*,*,#4750,.F.);
#6624=ORIENTED_EDGE('',*,*,#4753,.F.);
#6625=ORIENTED_EDGE('',*,*,#4756,.F.);
#6626=ORIENTED_EDGE('',*,*,#4759,.F.);
#6627=ORIENTED_EDGE('',*,*,#4762,.F.);
#6628=ORIENTED_EDGE('',*,*,#4765,.F.);
#6629=ORIENTED_EDGE('',*,*,#4768,.F.);
#6630=ORIENTED_EDGE('',*,*,#4771,.F.);
#6631=ORIENTED_EDGE('',*,*,#4774,.F.);
#6632=ORIENTED_EDGE('',*,*,#4777,.F.);
#6633=ORIENTED_EDGE('',*,*,#4780,.F.);
#6634=ORIENTED_EDGE('',*,*,#4783,.F.);
#6635=ORIENTED_EDGE('',*,*,#4786,.F.);
#6636=ORIENTED_EDGE('',*,*,#4789,.F.);
#6637=ORIENTED_EDGE('',*,*,#4792,.F.);
#6638=ORIENTED_EDGE('',*,*,#4795,.F.);
#6639=ORIENTED_EDGE('',*,*,#4798,.F.);
#6640=ORIENTED_EDGE('',*,*,#4801,.F.);
#6641=ORIENTED_EDGE('',*,*,#4804,.F.);
#6642=ORIENTED_EDGE('',*,*,#4807,.F.);
#6643=ORIENTED_EDGE('',*,*,#4810,.F.);
#6644=ORIENTED_EDGE('',*,*,#4813,.F.);
#6645=ORIENTED_EDGE('',*,*,#4816,.F.);
#6646=ORIENTED_EDGE('',*,*,#4819,.F.);
#6647=ORIENTED_EDGE('',*,*,#4822,.F.);
#6648=ORIENTED_EDGE('',*,*,#4825,.F.);
#6649=ORIENTED_EDGE('',*,*,#4828,.F.);
#6650=ORIENTED_EDGE('',*,*,#4831,.F.);
#6651=ORIENTED_EDGE('',*,*,#4834,.F.);
#6652=ORIENTED_EDGE('',*,*,#4837,.F.);
#6653=ORIENTED_EDGE('',*,*,#4840,.F.);
#6654=ORIENTED_EDGE('',*,*,#4843,.F.);
#6655=ORIENTED_EDGE('',*,*,#4846,.F.);
#6656=ORIENTED_EDGE('',*,*,#4849,.F.);
#6657=ORIENTED_EDGE('',*,*,#4852,.F.);
#6658=ORIENTED_EDGE('',*,*,#4855,.F.);
#6659=ORIENTED_EDGE('',*,*,#4858,.F.);
#6660=ORIENTED_EDGE('',*,*,#4861,.F.);
#6661=ORIENTED_EDGE('',*,*,#4864,.F.);
#6662=ORIENTED_EDGE('',*,*,#4893,.F.);
#6663=ORIENTED_EDGE('',*,*,#4886,.F.);
#6664=ORIENTED_EDGE('',*,*,#4301,.F.);
#6665=ORIENTED_EDGE('',*,*,#4305,.F.);
#6666=ORIENTED_EDGE('',*,*,#4308,.F.);
#6667=ORIENTED_EDGE('',*,*,#4311,.F.);
#6668=ORIENTED_EDGE('',*,*,#4314,.F.);
#6669=ORIENTED_EDGE('',*,*,#4317,.F.);
#6670=ORIENTED_EDGE('',*,*,#4320,.F.);
#6671=ORIENTED_EDGE('',*,*,#4323,.F.);
#6672=ORIENTED_EDGE('',*,*,#4326,.F.);
#6673=ORIENTED_EDGE('',*,*,#4329,.F.);
#6674=ORIENTED_EDGE('',*,*,#4332,.F.);
#6675=ORIENTED_EDGE('',*,*,#4335,.F.);
#6676=ORIENTED_EDGE('',*,*,#4338,.F.);
#6677=ORIENTED_EDGE('',*,*,#4341,.F.);
#6678=ORIENTED_EDGE('',*,*,#4344,.F.);
#6679=ORIENTED_EDGE('',*,*,#4347,.F.);
#6680=ORIENTED_EDGE('',*,*,#4350,.F.);
#6681=ORIENTED_EDGE('',*,*,#4353,.F.);
#6682=ORIENTED_EDGE('',*,*,#4356,.F.);
#6683=ORIENTED_EDGE('',*,*,#4359,.F.);
#6684=ORIENTED_EDGE('',*,*,#4362,.F.);
#6685=ORIENTED_EDGE('',*,*,#4365,.F.);
#6686=ORIENTED_EDGE('',*,*,#4368,.F.);
#6687=ORIENTED_EDGE('',*,*,#4371,.F.);
#6688=ORIENTED_EDGE('',*,*,#4374,.F.);
#6689=ORIENTED_EDGE('',*,*,#4377,.F.);
#6690=ORIENTED_EDGE('',*,*,#4380,.F.);
#6691=ORIENTED_EDGE('',*,*,#4383,.F.);
#6692=ORIENTED_EDGE('',*,*,#4386,.F.);
#6693=ORIENTED_EDGE('',*,*,#4389,.F.);
#6694=ORIENTED_EDGE('',*,*,#4392,.F.);
#6695=ORIENTED_EDGE('',*,*,#4395,.F.);
#6696=ORIENTED_EDGE('',*,*,#4398,.F.);
#6697=ORIENTED_EDGE('',*,*,#4401,.F.);
#6698=ORIENTED_EDGE('',*,*,#4404,.F.);
#6699=ORIENTED_EDGE('',*,*,#4407,.F.);
#6700=ORIENTED_EDGE('',*,*,#4410,.F.);
#6701=ORIENTED_EDGE('',*,*,#4413,.F.);
#6702=ORIENTED_EDGE('',*,*,#4416,.F.);
#6703=ORIENTED_EDGE('',*,*,#4419,.F.);
#6704=ORIENTED_EDGE('',*,*,#4422,.F.);
#6705=ORIENTED_EDGE('',*,*,#4425,.F.);
#6706=ORIENTED_EDGE('',*,*,#4428,.F.);
#6707=ORIENTED_EDGE('',*,*,#4431,.F.);
#6708=ORIENTED_EDGE('',*,*,#4434,.F.);
#6709=ORIENTED_EDGE('',*,*,#4437,.F.);
#6710=ORIENTED_EDGE('',*,*,#4440,.F.);
#6711=ORIENTED_EDGE('',*,*,#4443,.F.);
#6712=ORIENTED_EDGE('',*,*,#4446,.F.);
#6713=ORIENTED_EDGE('',*,*,#4449,.F.);
#6714=ORIENTED_EDGE('',*,*,#4452,.F.);
#6715=ORIENTED_EDGE('',*,*,#4455,.F.);
#6716=ORIENTED_EDGE('',*,*,#4458,.F.);
#6717=ORIENTED_EDGE('',*,*,#4461,.F.);
#6718=ORIENTED_EDGE('',*,*,#4464,.F.);
#6719=ORIENTED_EDGE('',*,*,#4467,.F.);
#6720=ORIENTED_EDGE('',*,*,#4470,.F.);
#6721=ORIENTED_EDGE('',*,*,#4473,.F.);
#6722=ORIENTED_EDGE('',*,*,#4476,.F.);
#6723=ORIENTED_EDGE('',*,*,#4479,.F.);
#6724=ORIENTED_EDGE('',*,*,#4482,.F.);
#6725=ORIENTED_EDGE('',*,*,#4485,.F.);
#6726=ORIENTED_EDGE('',*,*,#4488,.F.);
#6727=ORIENTED_EDGE('',*,*,#4491,.F.);
#6728=ORIENTED_EDGE('',*,*,#4494,.F.);
#6729=ORIENTED_EDGE('',*,*,#4497,.F.);
#6730=ORIENTED_EDGE('',*,*,#4500,.F.);
#6731=ORIENTED_EDGE('',*,*,#4503,.F.);
#6732=ORIENTED_EDGE('',*,*,#4506,.F.);
#6733=ORIENTED_EDGE('',*,*,#4509,.F.);
#6734=ORIENTED_EDGE('',*,*,#4512,.F.);
#6735=ORIENTED_EDGE('',*,*,#4515,.F.);
#6736=ORIENTED_EDGE('',*,*,#4518,.F.);
#6737=ORIENTED_EDGE('',*,*,#4521,.F.);
#6738=ORIENTED_EDGE('',*,*,#4524,.F.);
#6739=ORIENTED_EDGE('',*,*,#4527,.F.);
#6740=ORIENTED_EDGE('',*,*,#4530,.F.);
#6741=ORIENTED_EDGE('',*,*,#4533,.F.);
#6742=ORIENTED_EDGE('',*,*,#4536,.F.);
#6743=ORIENTED_EDGE('',*,*,#4539,.F.);
#6744=ORIENTED_EDGE('',*,*,#4542,.F.);
#6745=ORIENTED_EDGE('',*,*,#4545,.F.);
#6746=ORIENTED_EDGE('',*,*,#4548,.F.);
#6747=ORIENTED_EDGE('',*,*,#4551,.F.);
#6748=ORIENTED_EDGE('',*,*,#4554,.F.);
#6749=ORIENTED_EDGE('',*,*,#4557,.F.);
#6750=ORIENTED_EDGE('',*,*,#4560,.F.);
#6751=ORIENTED_EDGE('',*,*,#4563,.F.);
#6752=ORIENTED_EDGE('',*,*,#4566,.F.);
#6753=ORIENTED_EDGE('',*,*,#4569,.F.);
#6754=ORIENTED_EDGE('',*,*,#4572,.F.);
#6755=ORIENTED_EDGE('',*,*,#4575,.F.);
#6756=ORIENTED_EDGE('',*,*,#4578,.F.);
#6757=ORIENTED_EDGE('',*,*,#4581,.F.);
#6758=ORIENTED_EDGE('',*,*,#4895,.F.);
#6759=ORIENTED_EDGE('',*,*,#4890,.T.);
#6760=ORIENTED_EDGE('',*,*,#4585,.T.);
#6761=ORIENTED_EDGE('',*,*,#4894,.T.);
#6762=ORIENTED_EDGE('',*,*,#4896,.T.);
#6763=ORIENTED_EDGE('',*,*,#4580,.T.);
#6764=ORIENTED_EDGE('',*,*,#4891,.T.);
#6765=ORIENTED_EDGE('',*,*,#4896,.F.);
#6766=ORIENTED_EDGE('',*,*,#4895,.T.);
#8005=CYLINDRICAL_SURFACE('',#9073,1.188225);
#8006=CYLINDRICAL_SURFACE('',#9075,1.188225);
#8007=CYLINDRICAL_SURFACE('',#9076,1.188225);
#8008=CYLINDRICAL_SURFACE('',#9077,1.188225);
#8009=CYLINDRICAL_SURFACE('',#9078,1.188225);
#8010=CYLINDRICAL_SURFACE('',#9079,1.188225);
#8011=CYLINDRICAL_SURFACE('',#9080,1.188225);
#8012=CYLINDRICAL_SURFACE('',#9081,1.188225);
#8013=CYLINDRICAL_SURFACE('',#9082,1.188225);
#8014=CYLINDRICAL_SURFACE('',#9083,1.188225);
#8015=CYLINDRICAL_SURFACE('',#9084,1.188225);
#8016=CYLINDRICAL_SURFACE('',#9085,1.188225);
#8017=CYLINDRICAL_SURFACE('',#9086,1.188225);
#8018=CYLINDRICAL_SURFACE('',#9087,1.188225);
#8019=CYLINDRICAL_SURFACE('',#9088,1.188225);
#8020=CYLINDRICAL_SURFACE('',#9089,1.188225);
#8021=CYLINDRICAL_SURFACE('',#9090,1.188225);
#8022=CYLINDRICAL_SURFACE('',#9091,1.188225);
#8023=CYLINDRICAL_SURFACE('',#9092,1.188225);
#8024=CYLINDRICAL_SURFACE('',#9093,1.188225);
#8025=CYLINDRICAL_SURFACE('',#9094,1.188225);
#8026=CYLINDRICAL_SURFACE('',#9095,1.188225);
#8027=CYLINDRICAL_SURFACE('',#9096,1.188225);
#8028=CYLINDRICAL_SURFACE('',#9097,1.188225);
#8029=CYLINDRICAL_SURFACE('',#9098,1.188225);
#8030=CYLINDRICAL_SURFACE('',#9099,1.188225);
#8031=CYLINDRICAL_SURFACE('',#9100,1.188225);
#8032=CYLINDRICAL_SURFACE('',#9101,1.188225);
#8033=CYLINDRICAL_SURFACE('',#9102,1.188225);
#8034=CYLINDRICAL_SURFACE('',#9103,1.188225);
#8035=CYLINDRICAL_SURFACE('',#9104,1.188225);
#8036=CYLINDRICAL_SURFACE('',#9105,1.188225);
#8037=CYLINDRICAL_SURFACE('',#9106,1.188225);
#8038=CYLINDRICAL_SURFACE('',#9107,1.188225);
#8039=CYLINDRICAL_SURFACE('',#9108,1.188225);
#8040=CYLINDRICAL_SURFACE('',#9109,1.188225);
#8041=CYLINDRICAL_SURFACE('',#9110,1.188225);
#8042=CYLINDRICAL_SURFACE('',#9111,1.188225);
#8043=CYLINDRICAL_SURFACE('',#9112,1.188225);
#8044=CYLINDRICAL_SURFACE('',#9113,1.188225);
#8045=CYLINDRICAL_SURFACE('',#9114,1.188225);
#8046=CYLINDRICAL_SURFACE('',#9115,1.188225);
#8047=CYLINDRICAL_SURFACE('',#9116,1.188225);
#8048=CYLINDRICAL_SURFACE('',#9117,1.188225);
#8049=CYLINDRICAL_SURFACE('',#9118,1.188225);
#8050=CYLINDRICAL_SURFACE('',#9119,1.188225);
#8051=CYLINDRICAL_SURFACE('',#9120,1.188225);
#8052=CYLINDRICAL_SURFACE('',#9121,1.188225);
#8053=CYLINDRICAL_SURFACE('',#9122,1.188225);
#8054=CYLINDRICAL_SURFACE('',#9123,1.188225);
#8055=CYLINDRICAL_SURFACE('',#9124,1.188225);
#8056=CYLINDRICAL_SURFACE('',#9125,1.188225);
#8057=CYLINDRICAL_SURFACE('',#9126,1.188225);
#8058=CYLINDRICAL_SURFACE('',#9127,1.188225);
#8059=CYLINDRICAL_SURFACE('',#9128,1.188225);
#8060=CYLINDRICAL_SURFACE('',#9129,1.188225);
#8061=CYLINDRICAL_SURFACE('',#9130,1.188225);
#8062=CYLINDRICAL_SURFACE('',#9131,1.188225);
#8063=CYLINDRICAL_SURFACE('',#9132,1.188225);
#8064=CYLINDRICAL_SURFACE('',#9133,1.188225);
#8065=CYLINDRICAL_SURFACE('',#9134,1.188225);
#8066=CYLINDRICAL_SURFACE('',#9135,1.188225);
#8067=CYLINDRICAL_SURFACE('',#9136,1.188225);
#8068=CYLINDRICAL_SURFACE('',#9137,1.188225);
#8069=CYLINDRICAL_SURFACE('',#9138,1.188225);
#8070=CYLINDRICAL_SURFACE('',#9139,1.188225);
#8071=CYLINDRICAL_SURFACE('',#9140,1.188225);
#8072=CYLINDRICAL_SURFACE('',#9141,1.188225);
#8073=CYLINDRICAL_SURFACE('',#9142,1.188225);
#8074=CYLINDRICAL_SURFACE('',#9143,1.188225);
#8075=CYLINDRICAL_SURFACE('',#9144,1.188225);
#8076=CYLINDRICAL_SURFACE('',#9145,1.188225);
#8077=CYLINDRICAL_SURFACE('',#9146,1.188225);
#8078=CYLINDRICAL_SURFACE('',#9147,1.188225);
#8079=CYLINDRICAL_SURFACE('',#9148,1.188225);
#8080=CYLINDRICAL_SURFACE('',#9149,1.188225);
#8081=CYLINDRICAL_SURFACE('',#9150,1.188225);
#8082=CYLINDRICAL_SURFACE('',#9151,1.188225);
#8083=CYLINDRICAL_SURFACE('',#9152,1.188225);
#8084=CYLINDRICAL_SURFACE('',#9153,1.188225);
#8085=CYLINDRICAL_SURFACE('',#9154,1.188225);
#8086=CYLINDRICAL_SURFACE('',#9155,1.188225);
#8087=CYLINDRICAL_SURFACE('',#9156,1.188225);
#8088=CYLINDRICAL_SURFACE('',#9157,1.188225);
#8089=CYLINDRICAL_SURFACE('',#9158,1.188225);
#8090=CYLINDRICAL_SURFACE('',#9159,1.188225);
#8091=CYLINDRICAL_SURFACE('',#9160,1.188225);
#8092=CYLINDRICAL_SURFACE('',#9161,1.188225);
#8093=CYLINDRICAL_SURFACE('',#9162,1.188225);
#8094=CYLINDRICAL_SURFACE('',#9163,1.188225);
#8095=CYLINDRICAL_SURFACE('',#9164,1.188225);
#8096=CYLINDRICAL_SURFACE('',#9165,1.188225);
#8097=CYLINDRICAL_SURFACE('',#9166,1.188225);
#8098=CYLINDRICAL_SURFACE('',#9167,1.188225);
#8099=CYLINDRICAL_SURFACE('',#9168,1.016475);
#8100=CYLINDRICAL_SURFACE('',#9170,1.016475);
#8101=CYLINDRICAL_SURFACE('',#9171,1.016475);
#8102=CYLINDRICAL_SURFACE('',#9172,1.016475);
#8103=CYLINDRICAL_SURFACE('',#9173,1.016475);
#8104=CYLINDRICAL_SURFACE('',#9174,1.016475);
#8105=CYLINDRICAL_SURFACE('',#9175,1.016475);
#8106=CYLINDRICAL_SURFACE('',#9176,1.016475);
#8107=CYLINDRICAL_SURFACE('',#9177,1.016475);
#8108=CYLINDRICAL_SURFACE('',#9178,1.016475);
#8109=CYLINDRICAL_SURFACE('',#9179,1.016475);
#8110=CYLINDRICAL_SURFACE('',#9180,1.016475);
#8111=CYLINDRICAL_SURFACE('',#9181,1.016475);
#8112=CYLINDRICAL_SURFACE('',#9182,1.016475);
#8113=CYLINDRICAL_SURFACE('',#9183,1.016475);
#8114=CYLINDRICAL_SURFACE('',#9184,1.016475);
#8115=CYLINDRICAL_SURFACE('',#9185,1.016475);
#8116=CYLINDRICAL_SURFACE('',#9186,1.016475);
#8117=CYLINDRICAL_SURFACE('',#9187,1.016475);
#8118=CYLINDRICAL_SURFACE('',#9188,1.016475);
#8119=CYLINDRICAL_SURFACE('',#9189,1.016475);
#8120=CYLINDRICAL_SURFACE('',#9190,1.016475);
#8121=CYLINDRICAL_SURFACE('',#9191,1.016475);
#8122=CYLINDRICAL_SURFACE('',#9192,1.016475);
#8123=CYLINDRICAL_SURFACE('',#9193,1.016475);
#8124=CYLINDRICAL_SURFACE('',#9194,1.016475);
#8125=CYLINDRICAL_SURFACE('',#9195,1.016475);
#8126=CYLINDRICAL_SURFACE('',#9196,1.016475);
#8127=CYLINDRICAL_SURFACE('',#9197,1.016475);
#8128=CYLINDRICAL_SURFACE('',#9198,1.016475);
#8129=CYLINDRICAL_SURFACE('',#9199,1.016475);
#8130=CYLINDRICAL_SURFACE('',#9200,1.016475);
#8131=CYLINDRICAL_SURFACE('',#9201,1.016475);
#8132=CYLINDRICAL_SURFACE('',#9202,1.016475);
#8133=CYLINDRICAL_SURFACE('',#9203,1.016475);
#8134=CYLINDRICAL_SURFACE('',#9204,1.016475);
#8135=CYLINDRICAL_SURFACE('',#9205,1.016475);
#8136=CYLINDRICAL_SURFACE('',#9206,1.016475);
#8137=CYLINDRICAL_SURFACE('',#9207,1.016475);
#8138=CYLINDRICAL_SURFACE('',#9208,1.016475);
#8139=CYLINDRICAL_SURFACE('',#9209,1.016475);
#8140=CYLINDRICAL_SURFACE('',#9210,1.016475);
#8141=CYLINDRICAL_SURFACE('',#9211,1.016475);
#8142=CYLINDRICAL_SURFACE('',#9212,1.016475);
#8143=CYLINDRICAL_SURFACE('',#9213,1.016475);
#8144=CYLINDRICAL_SURFACE('',#9214,1.016475);
#8145=CYLINDRICAL_SURFACE('',#9215,1.016475);
#8146=CYLINDRICAL_SURFACE('',#9216,1.016475);
#8147=CYLINDRICAL_SURFACE('',#9217,1.016475);
#8148=CYLINDRICAL_SURFACE('',#9218,1.016475);
#8149=CYLINDRICAL_SURFACE('',#9219,1.016475);
#8150=CYLINDRICAL_SURFACE('',#9220,1.016475);
#8151=CYLINDRICAL_SURFACE('',#9221,1.016475);
#8152=CYLINDRICAL_SURFACE('',#9222,1.016475);
#8153=CYLINDRICAL_SURFACE('',#9223,1.016475);
#8154=CYLINDRICAL_SURFACE('',#9224,1.016475);
#8155=CYLINDRICAL_SURFACE('',#9225,1.016475);
#8156=CYLINDRICAL_SURFACE('',#9226,1.016475);
#8157=CYLINDRICAL_SURFACE('',#9227,1.016475);
#8158=CYLINDRICAL_SURFACE('',#9228,1.016475);
#8159=CYLINDRICAL_SURFACE('',#9229,1.016475);
#8160=CYLINDRICAL_SURFACE('',#9230,1.016475);
#8161=CYLINDRICAL_SURFACE('',#9231,1.016475);
#8162=CYLINDRICAL_SURFACE('',#9232,1.016475);
#8163=CYLINDRICAL_SURFACE('',#9233,1.016475);
#8164=CYLINDRICAL_SURFACE('',#9234,1.016475);
#8165=CYLINDRICAL_SURFACE('',#9235,1.016475);
#8166=CYLINDRICAL_SURFACE('',#9236,1.016475);
#8167=CYLINDRICAL_SURFACE('',#9237,1.016475);
#8168=CYLINDRICAL_SURFACE('',#9238,1.016475);
#8169=CYLINDRICAL_SURFACE('',#9239,1.016475);
#8170=CYLINDRICAL_SURFACE('',#9240,1.016475);
#8171=CYLINDRICAL_SURFACE('',#9241,1.016475);
#8172=CYLINDRICAL_SURFACE('',#9242,1.016475);
#8173=CYLINDRICAL_SURFACE('',#9243,1.016475);
#8174=CYLINDRICAL_SURFACE('',#9244,1.016475);
#8175=CYLINDRICAL_SURFACE('',#9245,1.016475);
#8176=CYLINDRICAL_SURFACE('',#9246,1.016475);
#8177=CYLINDRICAL_SURFACE('',#9247,1.016475);
#8178=CYLINDRICAL_SURFACE('',#9248,1.016475);
#8179=CYLINDRICAL_SURFACE('',#9249,1.016475);
#8180=CYLINDRICAL_SURFACE('',#9250,1.016475);
#8181=CYLINDRICAL_SURFACE('',#9251,1.016475);
#8182=CYLINDRICAL_SURFACE('',#9252,1.016475);
#8183=CYLINDRICAL_SURFACE('',#9253,1.016475);
#8184=CYLINDRICAL_SURFACE('',#9254,1.016475);
#8185=CYLINDRICAL_SURFACE('',#9255,1.016475);
#8186=CYLINDRICAL_SURFACE('',#9256,1.016475);
#8187=CYLINDRICAL_SURFACE('',#9257,1.016475);
#8188=CYLINDRICAL_SURFACE('',#9258,1.016475);
#8189=CYLINDRICAL_SURFACE('',#9259,1.016475);
#8190=CYLINDRICAL_SURFACE('',#9260,1.016475);
#8191=CYLINDRICAL_SURFACE('',#9261,1.016475);
#8192=CYLINDRICAL_SURFACE('',#9262,1.016475);
#8193=CYLINDRICAL_SURFACE('',#9263,0.15);
#8194=CYLINDRICAL_SURFACE('',#9266,0.15);
#8195=CYLINDRICAL_SURFACE('',#9269,0.33);
#8196=CYLINDRICAL_SURFACE('',#9272,0.33);
#8197=CYLINDRICAL_SURFACE('',#9275,0.33);
#8198=CYLINDRICAL_SURFACE('',#9278,0.33);
#8199=CYLINDRICAL_SURFACE('',#9284,3.8);
#8200=CYLINDRICAL_SURFACE('',#9287,1.016475);
#8201=CYLINDRICAL_SURFACE('',#9290,1.188225);
#8295=ADVANCED_FACE('',(#1058),#8005,.T.);
#8296=ADVANCED_FACE('',(#1059),#8006,.T.);
#8297=ADVANCED_FACE('',(#1060),#8007,.T.);
#8298=ADVANCED_FACE('',(#1061),#8008,.T.);
#8299=ADVANCED_FACE('',(#1062),#8009,.T.);
#8300=ADVANCED_FACE('',(#1063),#8010,.T.);
#8301=ADVANCED_FACE('',(#1064),#8011,.T.);
#8302=ADVANCED_FACE('',(#1065),#8012,.T.);
#8303=ADVANCED_FACE('',(#1066),#8013,.T.);
#8304=ADVANCED_FACE('',(#1067),#8014,.T.);
#8305=ADVANCED_FACE('',(#1068),#8015,.T.);
#8306=ADVANCED_FACE('',(#1069),#8016,.T.);
#8307=ADVANCED_FACE('',(#1070),#8017,.T.);
#8308=ADVANCED_FACE('',(#1071),#8018,.T.);
#8309=ADVANCED_FACE('',(#1072),#8019,.T.);
#8310=ADVANCED_FACE('',(#1073),#8020,.T.);
#8311=ADVANCED_FACE('',(#1074),#8021,.T.);
#8312=ADVANCED_FACE('',(#1075),#8022,.T.);
#8313=ADVANCED_FACE('',(#1076),#8023,.T.);
#8314=ADVANCED_FACE('',(#1077),#8024,.T.);
#8315=ADVANCED_FACE('',(#1078),#8025,.T.);
#8316=ADVANCED_FACE('',(#1079),#8026,.T.);
#8317=ADVANCED_FACE('',(#1080),#8027,.T.);
#8318=ADVANCED_FACE('',(#1081),#8028,.T.);
#8319=ADVANCED_FACE('',(#1082),#8029,.T.);
#8320=ADVANCED_FACE('',(#1083),#8030,.T.);
#8321=ADVANCED_FACE('',(#1084),#8031,.T.);
#8322=ADVANCED_FACE('',(#1085),#8032,.T.);
#8323=ADVANCED_FACE('',(#1086),#8033,.T.);
#8324=ADVANCED_FACE('',(#1087),#8034,.T.);
#8325=ADVANCED_FACE('',(#1088),#8035,.T.);
#8326=ADVANCED_FACE('',(#1089),#8036,.T.);
#8327=ADVANCED_FACE('',(#1090),#8037,.T.);
#8328=ADVANCED_FACE('',(#1091),#8038,.T.);
#8329=ADVANCED_FACE('',(#1092),#8039,.T.);
#8330=ADVANCED_FACE('',(#1093),#8040,.T.);
#8331=ADVANCED_FACE('',(#1094),#8041,.T.);
#8332=ADVANCED_FACE('',(#1095),#8042,.T.);
#8333=ADVANCED_FACE('',(#1096),#8043,.T.);
#8334=ADVANCED_FACE('',(#1097),#8044,.T.);
#8335=ADVANCED_FACE('',(#1098),#8045,.T.);
#8336=ADVANCED_FACE('',(#1099),#8046,.T.);
#8337=ADVANCED_FACE('',(#1100),#8047,.T.);
#8338=ADVANCED_FACE('',(#1101),#8048,.T.);
#8339=ADVANCED_FACE('',(#1102),#8049,.T.);
#8340=ADVANCED_FACE('',(#1103),#8050,.T.);
#8341=ADVANCED_FACE('',(#1104),#8051,.T.);
#8342=ADVANCED_FACE('',(#1105),#8052,.T.);
#8343=ADVANCED_FACE('',(#1106),#8053,.T.);
#8344=ADVANCED_FACE('',(#1107),#8054,.T.);
#8345=ADVANCED_FACE('',(#1108),#8055,.T.);
#8346=ADVANCED_FACE('',(#1109),#8056,.T.);
#8347=ADVANCED_FACE('',(#1110),#8057,.T.);
#8348=ADVANCED_FACE('',(#1111),#8058,.T.);
#8349=ADVANCED_FACE('',(#1112),#8059,.T.);
#8350=ADVANCED_FACE('',(#1113),#8060,.T.);
#8351=ADVANCED_FACE('',(#1114),#8061,.T.);
#8352=ADVANCED_FACE('',(#1115),#8062,.T.);
#8353=ADVANCED_FACE('',(#1116),#8063,.T.);
#8354=ADVANCED_FACE('',(#1117),#8064,.T.);
#8355=ADVANCED_FACE('',(#1118),#8065,.T.);
#8356=ADVANCED_FACE('',(#1119),#8066,.T.);
#8357=ADVANCED_FACE('',(#1120),#8067,.T.);
#8358=ADVANCED_FACE('',(#1121),#8068,.T.);
#8359=ADVANCED_FACE('',(#1122),#8069,.T.);
#8360=ADVANCED_FACE('',(#1123),#8070,.T.);
#8361=ADVANCED_FACE('',(#1124),#8071,.T.);
#8362=ADVANCED_FACE('',(#1125),#8072,.T.);
#8363=ADVANCED_FACE('',(#1126),#8073,.T.);
#8364=ADVANCED_FACE('',(#1127),#8074,.T.);
#8365=ADVANCED_FACE('',(#1128),#8075,.T.);
#8366=ADVANCED_FACE('',(#1129),#8076,.T.);
#8367=ADVANCED_FACE('',(#1130),#8077,.T.);
#8368=ADVANCED_FACE('',(#1131),#8078,.T.);
#8369=ADVANCED_FACE('',(#1132),#8079,.T.);
#8370=ADVANCED_FACE('',(#1133),#8080,.T.);
#8371=ADVANCED_FACE('',(#1134),#8081,.T.);
#8372=ADVANCED_FACE('',(#1135),#8082,.T.);
#8373=ADVANCED_FACE('',(#1136),#8083,.T.);
#8374=ADVANCED_FACE('',(#1137),#8084,.T.);
#8375=ADVANCED_FACE('',(#1138),#8085,.T.);
#8376=ADVANCED_FACE('',(#1139),#8086,.T.);
#8377=ADVANCED_FACE('',(#1140),#8087,.T.);
#8378=ADVANCED_FACE('',(#1141),#8088,.T.);
#8379=ADVANCED_FACE('',(#1142),#8089,.T.);
#8380=ADVANCED_FACE('',(#1143),#8090,.T.);
#8381=ADVANCED_FACE('',(#1144),#8091,.T.);
#8382=ADVANCED_FACE('',(#1145),#8092,.T.);
#8383=ADVANCED_FACE('',(#1146),#8093,.T.);
#8384=ADVANCED_FACE('',(#1147),#8094,.T.);
#8385=ADVANCED_FACE('',(#1148),#8095,.T.);
#8386=ADVANCED_FACE('',(#1149),#8096,.T.);
#8387=ADVANCED_FACE('',(#1150),#8097,.T.);
#8388=ADVANCED_FACE('',(#1151),#8098,.T.);
#8389=ADVANCED_FACE('',(#1152),#8099,.T.);
#8390=ADVANCED_FACE('',(#1153),#8100,.T.);
#8391=ADVANCED_FACE('',(#1154),#8101,.T.);
#8392=ADVANCED_FACE('',(#1155),#8102,.T.);
#8393=ADVANCED_FACE('',(#1156),#8103,.T.);
#8394=ADVANCED_FACE('',(#1157),#8104,.T.);
#8395=ADVANCED_FACE('',(#1158),#8105,.T.);
#8396=ADVANCED_FACE('',(#1159),#8106,.T.);
#8397=ADVANCED_FACE('',(#1160),#8107,.T.);
#8398=ADVANCED_FACE('',(#1161),#8108,.T.);
#8399=ADVANCED_FACE('',(#1162),#8109,.T.);
#8400=ADVANCED_FACE('',(#1163),#8110,.T.);
#8401=ADVANCED_FACE('',(#1164),#8111,.T.);
#8402=ADVANCED_FACE('',(#1165),#8112,.T.);
#8403=ADVANCED_FACE('',(#1166),#8113,.T.);
#8404=ADVANCED_FACE('',(#1167),#8114,.T.);
#8405=ADVANCED_FACE('',(#1168),#8115,.T.);
#8406=ADVANCED_FACE('',(#1169),#8116,.T.);
#8407=ADVANCED_FACE('',(#1170),#8117,.T.);
#8408=ADVANCED_FACE('',(#1171),#8118,.T.);
#8409=ADVANCED_FACE('',(#1172),#8119,.T.);
#8410=ADVANCED_FACE('',(#1173),#8120,.T.);
#8411=ADVANCED_FACE('',(#1174),#8121,.T.);
#8412=ADVANCED_FACE('',(#1175),#8122,.T.);
#8413=ADVANCED_FACE('',(#1176),#8123,.T.);
#8414=ADVANCED_FACE('',(#1177),#8124,.T.);
#8415=ADVANCED_FACE('',(#1178),#8125,.T.);
#8416=ADVANCED_FACE('',(#1179),#8126,.T.);
#8417=ADVANCED_FACE('',(#1180),#8127,.T.);
#8418=ADVANCED_FACE('',(#1181),#8128,.T.);
#8419=ADVANCED_FACE('',(#1182),#8129,.T.);
#8420=ADVANCED_FACE('',(#1183),#8130,.T.);
#8421=ADVANCED_FACE('',(#1184),#8131,.T.);
#8422=ADVANCED_FACE('',(#1185),#8132,.T.);
#8423=ADVANCED_FACE('',(#1186),#8133,.T.);
#8424=ADVANCED_FACE('',(#1187),#8134,.T.);
#8425=ADVANCED_FACE('',(#1188),#8135,.T.);
#8426=ADVANCED_FACE('',(#1189),#8136,.T.);
#8427=ADVANCED_FACE('',(#1190),#8137,.T.);
#8428=ADVANCED_FACE('',(#1191),#8138,.T.);
#8429=ADVANCED_FACE('',(#1192),#8139,.T.);
#8430=ADVANCED_FACE('',(#1193),#8140,.T.);
#8431=ADVANCED_FACE('',(#1194),#8141,.T.);
#8432=ADVANCED_FACE('',(#1195),#8142,.T.);
#8433=ADVANCED_FACE('',(#1196),#8143,.T.);
#8434=ADVANCED_FACE('',(#1197),#8144,.T.);
#8435=ADVANCED_FACE('',(#1198),#8145,.T.);
#8436=ADVANCED_FACE('',(#1199),#8146,.T.);
#8437=ADVANCED_FACE('',(#1200),#8147,.T.);
#8438=ADVANCED_FACE('',(#1201),#8148,.T.);
#8439=ADVANCED_FACE('',(#1202),#8149,.T.);
#8440=ADVANCED_FACE('',(#1203),#8150,.T.);
#8441=ADVANCED_FACE('',(#1204),#8151,.T.);
#8442=ADVANCED_FACE('',(#1205),#8152,.T.);
#8443=ADVANCED_FACE('',(#1206),#8153,.T.);
#8444=ADVANCED_FACE('',(#1207),#8154,.T.);
#8445=ADVANCED_FACE('',(#1208),#8155,.T.);
#8446=ADVANCED_FACE('',(#1209),#8156,.T.);
#8447=ADVANCED_FACE('',(#1210),#8157,.T.);
#8448=ADVANCED_FACE('',(#1211),#8158,.T.);
#8449=ADVANCED_FACE('',(#1212),#8159,.T.);
#8450=ADVANCED_FACE('',(#1213),#8160,.T.);
#8451=ADVANCED_FACE('',(#1214),#8161,.T.);
#8452=ADVANCED_FACE('',(#1215),#8162,.T.);
#8453=ADVANCED_FACE('',(#1216),#8163,.T.);
#8454=ADVANCED_FACE('',(#1217),#8164,.T.);
#8455=ADVANCED_FACE('',(#1218),#8165,.T.);
#8456=ADVANCED_FACE('',(#1219),#8166,.T.);
#8457=ADVANCED_FACE('',(#1220),#8167,.T.);
#8458=ADVANCED_FACE('',(#1221),#8168,.T.);
#8459=ADVANCED_FACE('',(#1222),#8169,.T.);
#8460=ADVANCED_FACE('',(#1223),#8170,.T.);
#8461=ADVANCED_FACE('',(#1224),#8171,.T.);
#8462=ADVANCED_FACE('',(#1225),#8172,.T.);
#8463=ADVANCED_FACE('',(#1226),#8173,.T.);
#8464=ADVANCED_FACE('',(#1227),#8174,.T.);
#8465=ADVANCED_FACE('',(#1228),#8175,.T.);
#8466=ADVANCED_FACE('',(#1229),#8176,.T.);
#8467=ADVANCED_FACE('',(#1230),#8177,.T.);
#8468=ADVANCED_FACE('',(#1231),#8178,.T.);
#8469=ADVANCED_FACE('',(#1232),#8179,.T.);
#8470=ADVANCED_FACE('',(#1233),#8180,.T.);
#8471=ADVANCED_FACE('',(#1234),#8181,.T.);
#8472=ADVANCED_FACE('',(#1235),#8182,.T.);
#8473=ADVANCED_FACE('',(#1236),#8183,.T.);
#8474=ADVANCED_FACE('',(#1237),#8184,.T.);
#8475=ADVANCED_FACE('',(#1238),#8185,.T.);
#8476=ADVANCED_FACE('',(#1239),#8186,.T.);
#8477=ADVANCED_FACE('',(#1240),#8187,.T.);
#8478=ADVANCED_FACE('',(#1241),#8188,.T.);
#8479=ADVANCED_FACE('',(#1242),#8189,.T.);
#8480=ADVANCED_FACE('',(#1243),#8190,.T.);
#8481=ADVANCED_FACE('',(#1244),#8191,.T.);
#8482=ADVANCED_FACE('',(#1245),#8192,.T.);
#8483=ADVANCED_FACE('',(#1246),#8193,.F.);
#8484=ADVANCED_FACE('',(#1247),#8194,.F.);
#8485=ADVANCED_FACE('',(#1248),#8195,.F.);
#8486=ADVANCED_FACE('',(#1249),#8196,.F.);
#8487=ADVANCED_FACE('',(#1250),#8197,.F.);
#8488=ADVANCED_FACE('',(#1251),#8198,.F.);
#8489=ADVANCED_FACE('',(#1252,#809,#810,#811,#812,#813,#814,#815),#865,
 .T.);
#8490=ADVANCED_FACE('',(#1253),#8199,.T.);
#8491=ADVANCED_FACE('',(#1254,#816,#817,#818,#819,#820,#821),#866,.F.);
#8492=ADVANCED_FACE('',(#1255),#207,.F.);
#8493=ADVANCED_FACE('',(#1256),#8200,.T.);
#8494=ADVANCED_FACE('',(#1257),#208,.F.);
#8495=ADVANCED_FACE('',(#1258),#867,.T.);
#8496=ADVANCED_FACE('',(#1259),#8201,.T.);
#8769=CLOSED_SHELL('',(#8295,#8296,#8297,#8298,#8299,#8300,#8301,#8302,
#8303,#8304,#8305,#8306,#8307,#8308,#8309,#8310,#8311,#8312,#8313,#8314,
#8315,#8316,#8317,#8318,#8319,#8320,#8321,#8322,#8323,#8324,#8325,#8326,
#8327,#8328,#8329,#8330,#8331,#8332,#8333,#8334,#8335,#8336,#8337,#8338,
#8339,#8340,#8341,#8342,#8343,#8344,#8345,#8346,#8347,#8348,#8349,#8350,
#8351,#8352,#8353,#8354,#8355,#8356,#8357,#8358,#8359,#8360,#8361,#8362,
#8363,#8364,#8365,#8366,#8367,#8368,#8369,#8370,#8371,#8372,#8373,#8374,
#8375,#8376,#8377,#8378,#8379,#8380,#8381,#8382,#8383,#8384,#8385,#8386,
#8387,#8388,#8389,#8390,#8391,#8392,#8393,#8394,#8395,#8396,#8397,#8398,
#8399,#8400,#8401,#8402,#8403,#8404,#8405,#8406,#8407,#8408,#8409,#8410,
#8411,#8412,#8413,#8414,#8415,#8416,#8417,#8418,#8419,#8420,#8421,#8422,
#8423,#8424,#8425,#8426,#8427,#8428,#8429,#8430,#8431,#8432,#8433,#8434,
#8435,#8436,#8437,#8438,#8439,#8440,#8441,#8442,#8443,#8444,#8445,#8446,
#8447,#8448,#8449,#8450,#8451,#8452,#8453,#8454,#8455,#8456,#8457,#8458,
#8459,#8460,#8461,#8462,#8463,#8464,#8465,#8466,#8467,#8468,#8469,#8470,
#8471,#8472,#8473,#8474,#8475,#8476,#8477,#8478,#8479,#8480,#8481,#8482,
#8483,#8484,#8485,#8486,#8487,#8488,#8489,#8490,#8491,#8492,#8493,#8494,
#8495,#8496));
#9072=AXIS2_PLACEMENT_3D('',#11773,#9801,#9802);
#9073=AXIS2_PLACEMENT_3D('',#11774,#9803,#9804);
#9074=AXIS2_PLACEMENT_3D('',#11790,#9806,#9807);
#9075=AXIS2_PLACEMENT_3D('',#11801,#9808,#9809);
#9076=AXIS2_PLACEMENT_3D('',#11855,#9811,#9812);
#9077=AXIS2_PLACEMENT_3D('',#11915,#9814,#9815);
#9078=AXIS2_PLACEMENT_3D('',#11972,#9817,#9818);
#9079=AXIS2_PLACEMENT_3D('',#12032,#9820,#9821);
#9080=AXIS2_PLACEMENT_3D('',#12092,#9823,#9824);
#9081=AXIS2_PLACEMENT_3D('',#12149,#9826,#9827);
#9082=AXIS2_PLACEMENT_3D('',#12209,#9829,#9830);
#9083=AXIS2_PLACEMENT_3D('',#12269,#9832,#9833);
#9084=AXIS2_PLACEMENT_3D('',#12329,#9835,#9836);
#9085=AXIS2_PLACEMENT_3D('',#12389,#9838,#9839);
#9086=AXIS2_PLACEMENT_3D('',#12449,#9841,#9842);
#9087=AXIS2_PLACEMENT_3D('',#12506,#9844,#9845);
#9088=AXIS2_PLACEMENT_3D('',#12566,#9847,#9848);
#9089=AXIS2_PLACEMENT_3D('',#12626,#9850,#9851);
#9090=AXIS2_PLACEMENT_3D('',#12686,#9853,#9854);
#9091=AXIS2_PLACEMENT_3D('',#12746,#9856,#9857);
#9092=AXIS2_PLACEMENT_3D('',#12803,#9859,#9860);
#9093=AXIS2_PLACEMENT_3D('',#12863,#9862,#9863);
#9094=AXIS2_PLACEMENT_3D('',#12923,#9865,#9866);
#9095=AXIS2_PLACEMENT_3D('',#12983,#9868,#9869);
#9096=AXIS2_PLACEMENT_3D('',#13043,#9871,#9872);
#9097=AXIS2_PLACEMENT_3D('',#13097,#9874,#9875);
#9098=AXIS2_PLACEMENT_3D('',#13157,#9877,#9878);
#9099=AXIS2_PLACEMENT_3D('',#13217,#9880,#9881);
#9100=AXIS2_PLACEMENT_3D('',#13277,#9883,#9884);
#9101=AXIS2_PLACEMENT_3D('',#13334,#9886,#9887);
#9102=AXIS2_PLACEMENT_3D('',#13394,#9889,#9890);
#9103=AXIS2_PLACEMENT_3D('',#13454,#9892,#9893);
#9104=AXIS2_PLACEMENT_3D('',#13514,#9895,#9896);
#9105=AXIS2_PLACEMENT_3D('',#13574,#9898,#9899);
#9106=AXIS2_PLACEMENT_3D('',#13634,#9901,#9902);
#9107=AXIS2_PLACEMENT_3D('',#13694,#9904,#9905);
#9108=AXIS2_PLACEMENT_3D('',#13754,#9907,#9908);
#9109=AXIS2_PLACEMENT_3D('',#13814,#9910,#9911);
#9110=AXIS2_PLACEMENT_3D('',#13874,#9913,#9914);
#9111=AXIS2_PLACEMENT_3D('',#13931,#9916,#9917);
#9112=AXIS2_PLACEMENT_3D('',#13991,#9919,#9920);
#9113=AXIS2_PLACEMENT_3D('',#14051,#9922,#9923);
#9114=AXIS2_PLACEMENT_3D('',#14111,#9925,#9926);
#9115=AXIS2_PLACEMENT_3D('',#14171,#9928,#9929);
#9116=AXIS2_PLACEMENT_3D('',#14228,#9931,#9932);
#9117=AXIS2_PLACEMENT_3D('',#14288,#9934,#9935);
#9118=AXIS2_PLACEMENT_3D('',#14348,#9937,#9938);
#9119=AXIS2_PLACEMENT_3D('',#14408,#9940,#9941);
#9120=AXIS2_PLACEMENT_3D('',#14468,#9943,#9944);
#9121=AXIS2_PLACEMENT_3D('',#14528,#9946,#9947);
#9122=AXIS2_PLACEMENT_3D('',#14588,#9949,#9950);
#9123=AXIS2_PLACEMENT_3D('',#14645,#9952,#9953);
#9124=AXIS2_PLACEMENT_3D('',#14705,#9955,#9956);
#9125=AXIS2_PLACEMENT_3D('',#14765,#9958,#9959);
#9126=AXIS2_PLACEMENT_3D('',#14825,#9961,#9962);
#9127=AXIS2_PLACEMENT_3D('',#14885,#9964,#9965);
#9128=AXIS2_PLACEMENT_3D('',#14942,#9967,#9968);
#9129=AXIS2_PLACEMENT_3D('',#15002,#9970,#9971);
#9130=AXIS2_PLACEMENT_3D('',#15062,#9973,#9974);
#9131=AXIS2_PLACEMENT_3D('',#15122,#9976,#9977);
#9132=AXIS2_PLACEMENT_3D('',#15182,#9979,#9980);
#9133=AXIS2_PLACEMENT_3D('',#15242,#9982,#9983);
#9134=AXIS2_PLACEMENT_3D('',#15299,#9985,#9986);
#9135=AXIS2_PLACEMENT_3D('',#15359,#9988,#9989);
#9136=AXIS2_PLACEMENT_3D('',#15419,#9991,#9992);
#9137=AXIS2_PLACEMENT_3D('',#15479,#9994,#9995);
#9138=AXIS2_PLACEMENT_3D('',#15539,#9997,#9998);
#9139=AXIS2_PLACEMENT_3D('',#15596,#10000,#10001);
#9140=AXIS2_PLACEMENT_3D('',#15656,#10003,#10004);
#9141=AXIS2_PLACEMENT_3D('',#15716,#10006,#10007);
#9142=AXIS2_PLACEMENT_3D('',#15776,#10009,#10010);
#9143=AXIS2_PLACEMENT_3D('',#15833,#10012,#10013);
#9144=AXIS2_PLACEMENT_3D('',#15893,#10015,#10016);
#9145=AXIS2_PLACEMENT_3D('',#15953,#10018,#10019);
#9146=AXIS2_PLACEMENT_3D('',#16013,#10021,#10022);
#9147=AXIS2_PLACEMENT_3D('',#16073,#10024,#10025);
#9148=AXIS2_PLACEMENT_3D('',#16133,#10027,#10028);
#9149=AXIS2_PLACEMENT_3D('',#16193,#10030,#10031);
#9150=AXIS2_PLACEMENT_3D('',#16253,#10033,#10034);
#9151=AXIS2_PLACEMENT_3D('',#16313,#10036,#10037);
#9152=AXIS2_PLACEMENT_3D('',#16373,#10039,#10040);
#9153=AXIS2_PLACEMENT_3D('',#16430,#10042,#10043);
#9154=AXIS2_PLACEMENT_3D('',#16490,#10045,#10046);
#9155=AXIS2_PLACEMENT_3D('',#16550,#10048,#10049);
#9156=AXIS2_PLACEMENT_3D('',#16610,#10051,#10052);
#9157=AXIS2_PLACEMENT_3D('',#16670,#10054,#10055);
#9158=AXIS2_PLACEMENT_3D('',#16727,#10057,#10058);
#9159=AXIS2_PLACEMENT_3D('',#16787,#10060,#10061);
#9160=AXIS2_PLACEMENT_3D('',#16847,#10063,#10064);
#9161=AXIS2_PLACEMENT_3D('',#16907,#10066,#10067);
#9162=AXIS2_PLACEMENT_3D('',#16967,#10069,#10070);
#9163=AXIS2_PLACEMENT_3D('',#17027,#10072,#10073);
#9164=AXIS2_PLACEMENT_3D('',#17087,#10075,#10076);
#9165=AXIS2_PLACEMENT_3D('',#17147,#10078,#10079);
#9166=AXIS2_PLACEMENT_3D('',#17207,#10081,#10082);
#9167=AXIS2_PLACEMENT_3D('',#17267,#10084,#10085);
#9168=AXIS2_PLACEMENT_3D('',#17324,#10087,#10088);
#9169=AXIS2_PLACEMENT_3D('',#17340,#10090,#10091);
#9170=AXIS2_PLACEMENT_3D('',#17346,#10092,#10093);
#9171=AXIS2_PLACEMENT_3D('',#17406,#10095,#10096);
#9172=AXIS2_PLACEMENT_3D('',#17463,#10098,#10099);
#9173=AXIS2_PLACEMENT_3D('',#17523,#10101,#10102);
#9174=AXIS2_PLACEMENT_3D('',#17583,#10104,#10105);
#9175=AXIS2_PLACEMENT_3D('',#17626,#10107,#10108);
#9176=AXIS2_PLACEMENT_3D('',#17669,#10110,#10111);
#9177=AXIS2_PLACEMENT_3D('',#17711,#10113,#10114);
#9178=AXIS2_PLACEMENT_3D('',#17771,#10116,#10117);
#9179=AXIS2_PLACEMENT_3D('',#17831,#10119,#10120);
#9180=AXIS2_PLACEMENT_3D('',#17891,#10122,#10123);
#9181=AXIS2_PLACEMENT_3D('',#17951,#10125,#10126);
#9182=AXIS2_PLACEMENT_3D('',#17994,#10128,#10129);
#9183=AXIS2_PLACEMENT_3D('',#18054,#10131,#10132);
#9184=AXIS2_PLACEMENT_3D('',#18114,#10134,#10135);
#9185=AXIS2_PLACEMENT_3D('',#18174,#10137,#10138);
#9186=AXIS2_PLACEMENT_3D('',#18217,#10140,#10141);
#9187=AXIS2_PLACEMENT_3D('',#18277,#10143,#10144);
#9188=AXIS2_PLACEMENT_3D('',#18337,#10146,#10147);
#9189=AXIS2_PLACEMENT_3D('',#18397,#10149,#10150);
#9190=AXIS2_PLACEMENT_3D('',#18457,#10152,#10153);
#9191=AXIS2_PLACEMENT_3D('',#18500,#10155,#10156);
#9192=AXIS2_PLACEMENT_3D('',#18560,#10158,#10159);
#9193=AXIS2_PLACEMENT_3D('',#18620,#10161,#10162);
#9194=AXIS2_PLACEMENT_3D('',#18680,#10164,#10165);
#9195=AXIS2_PLACEMENT_3D('',#18740,#10167,#10168);
#9196=AXIS2_PLACEMENT_3D('',#18765,#10170,#10171);
#9197=AXIS2_PLACEMENT_3D('',#18809,#10173,#10174);
#9198=AXIS2_PLACEMENT_3D('',#18869,#10176,#10177);
#9199=AXIS2_PLACEMENT_3D('',#18929,#10179,#10180);
#9200=AXIS2_PLACEMENT_3D('',#18972,#10182,#10183);
#9201=AXIS2_PLACEMENT_3D('',#19015,#10185,#10186);
#9202=AXIS2_PLACEMENT_3D('',#19058,#10188,#10189);
#9203=AXIS2_PLACEMENT_3D('',#19118,#10191,#10192);
#9204=AXIS2_PLACEMENT_3D('',#19178,#10194,#10195);
#9205=AXIS2_PLACEMENT_3D('',#19221,#10197,#10198);
#9206=AXIS2_PLACEMENT_3D('',#19264,#10200,#10201);
#9207=AXIS2_PLACEMENT_3D('',#19324,#10203,#10204);
#9208=AXIS2_PLACEMENT_3D('',#19384,#10206,#10207);
#9209=AXIS2_PLACEMENT_3D('',#19444,#10209,#10210);
#9210=AXIS2_PLACEMENT_3D('',#19504,#10212,#10213);
#9211=AXIS2_PLACEMENT_3D('',#19547,#10215,#10216);
#9212=AXIS2_PLACEMENT_3D('',#19590,#10218,#10219);
#9213=AXIS2_PLACEMENT_3D('',#19650,#10221,#10222);
#9214=AXIS2_PLACEMENT_3D('',#19710,#10224,#10225);
#9215=AXIS2_PLACEMENT_3D('',#19753,#10227,#10228);
#9216=AXIS2_PLACEMENT_3D('',#19796,#10230,#10231);
#9217=AXIS2_PLACEMENT_3D('',#19839,#10233,#10234);
#9218=AXIS2_PLACEMENT_3D('',#19899,#10236,#10237);
#9219=AXIS2_PLACEMENT_3D('',#19942,#10239,#10240);
#9220=AXIS2_PLACEMENT_3D('',#20002,#10242,#10243);
#9221=AXIS2_PLACEMENT_3D('',#20062,#10245,#10246);
#9222=AXIS2_PLACEMENT_3D('',#20122,#10248,#10249);
#9223=AXIS2_PLACEMENT_3D('',#20182,#10251,#10252);
#9224=AXIS2_PLACEMENT_3D('',#20225,#10254,#10255);
#9225=AXIS2_PLACEMENT_3D('',#20285,#10257,#10258);
#9226=AXIS2_PLACEMENT_3D('',#20345,#10260,#10261);
#9227=AXIS2_PLACEMENT_3D('',#20405,#10263,#10264);
#9228=AXIS2_PLACEMENT_3D('',#20448,#10266,#10267);
#9229=AXIS2_PLACEMENT_3D('',#20508,#10269,#10270);
#9230=AXIS2_PLACEMENT_3D('',#20568,#10272,#10273);
#9231=AXIS2_PLACEMENT_3D('',#20628,#10275,#10276);
#9232=AXIS2_PLACEMENT_3D('',#20688,#10278,#10279);
#9233=AXIS2_PLACEMENT_3D('',#20730,#10281,#10282);
#9234=AXIS2_PLACEMENT_3D('',#20790,#10284,#10285);
#9235=AXIS2_PLACEMENT_3D('',#20833,#10287,#10288);
#9236=AXIS2_PLACEMENT_3D('',#20893,#10290,#10291);
#9237=AXIS2_PLACEMENT_3D('',#20953,#10293,#10294);
#9238=AXIS2_PLACEMENT_3D('',#20996,#10296,#10297);
#9239=AXIS2_PLACEMENT_3D('',#21040,#10299,#10300);
#9240=AXIS2_PLACEMENT_3D('',#21100,#10302,#10303);
#9241=AXIS2_PLACEMENT_3D('',#21160,#10305,#10306);
#9242=AXIS2_PLACEMENT_3D('',#21203,#10308,#10309);
#9243=AXIS2_PLACEMENT_3D('',#21246,#10311,#10312);
#9244=AXIS2_PLACEMENT_3D('',#21306,#10314,#10315);
#9245=AXIS2_PLACEMENT_3D('',#21366,#10317,#10318);
#9246=AXIS2_PLACEMENT_3D('',#21426,#10320,#10321);
#9247=AXIS2_PLACEMENT_3D('',#21469,#10323,#10324);
#9248=AXIS2_PLACEMENT_3D('',#21512,#10326,#10327);
#9249=AXIS2_PLACEMENT_3D('',#21572,#10329,#10330);
#9250=AXIS2_PLACEMENT_3D('',#21632,#10332,#10333);
#9251=AXIS2_PLACEMENT_3D('',#21692,#10335,#10336);
#9252=AXIS2_PLACEMENT_3D('',#21752,#10338,#10339);
#9253=AXIS2_PLACEMENT_3D('',#21795,#10341,#10342);
#9254=AXIS2_PLACEMENT_3D('',#21822,#10344,#10345);
#9255=AXIS2_PLACEMENT_3D('',#21882,#10347,#10348);
#9256=AXIS2_PLACEMENT_3D('',#21925,#10350,#10351);
#9257=AXIS2_PLACEMENT_3D('',#21968,#10353,#10354);
#9258=AXIS2_PLACEMENT_3D('',#22011,#10356,#10357);
#9259=AXIS2_PLACEMENT_3D('',#22054,#10359,#10360);
#9260=AXIS2_PLACEMENT_3D('',#22114,#10362,#10363);
#9261=AXIS2_PLACEMENT_3D('',#22174,#10365,#10366);
#9262=AXIS2_PLACEMENT_3D('',#22217,#10368,#10369);
#9263=AXIS2_PLACEMENT_3D('',#22243,#10371,#10372);
#9264=AXIS2_PLACEMENT_3D('',#22245,#10373,#10374);
#9265=AXIS2_PLACEMENT_3D('',#22248,#10376,#10377);
#9266=AXIS2_PLACEMENT_3D('',#22249,#10378,#10379);
#9267=AXIS2_PLACEMENT_3D('',#22251,#10380,#10381);
#9268=AXIS2_PLACEMENT_3D('',#22254,#10383,#10384);
#9269=AXIS2_PLACEMENT_3D('',#22255,#10385,#10386);
#9270=AXIS2_PLACEMENT_3D('',#22257,#10387,#10388);
#9271=AXIS2_PLACEMENT_3D('',#22260,#10390,#10391);
#9272=AXIS2_PLACEMENT_3D('',#22261,#10392,#10393);
#9273=AXIS2_PLACEMENT_3D('',#22263,#10394,#10395);
#9274=AXIS2_PLACEMENT_3D('',#22266,#10397,#10398);
#9275=AXIS2_PLACEMENT_3D('',#22267,#10399,#10400);
#9276=AXIS2_PLACEMENT_3D('',#22269,#10401,#10402);
#9277=AXIS2_PLACEMENT_3D('',#22272,#10404,#10405);
#9278=AXIS2_PLACEMENT_3D('',#22273,#10406,#10407);
#9279=AXIS2_PLACEMENT_3D('',#22275,#10408,#10409);
#9280=AXIS2_PLACEMENT_3D('',#22278,#10411,#10412);
#9281=AXIS2_PLACEMENT_3D('',#22279,#10413,#10414);
#9282=AXIS2_PLACEMENT_3D('',#22281,#10415,#10416);
#9283=AXIS2_PLACEMENT_3D('',#22380,#10417,#10418);
#9284=AXIS2_PLACEMENT_3D('',#22381,#10419,#10420);
#9285=AXIS2_PLACEMENT_3D('',#22384,#10422,#10423);
#9286=AXIS2_PLACEMENT_3D('',#22385,#10424,#10425);
#9287=AXIS2_PLACEMENT_3D('',#25229,#10426,#10427);
#9288=AXIS2_PLACEMENT_3D('',#28011,#10428,#10429);
#9289=AXIS2_PLACEMENT_3D('',#28012,#10430,#10431);
#9290=AXIS2_PLACEMENT_3D('',#28013,#10432,#10433);
#9801=DIRECTION('axis',(0.,0.,1.));
#9802=DIRECTION('refdir',(1.,0.,0.));
#9803=DIRECTION('center_axis',(0.,0.,1.));
#9804=DIRECTION('ref_axis',(1.,0.,0.));
#9805=DIRECTION('',(0.,0.,-1.));
#9806=DIRECTION('center_axis',(0.,0.,-1.));
#9807=DIRECTION('ref_axis',(1.,0.,0.));
#9808=DIRECTION('center_axis',(0.,0.,1.));
#9809=DIRECTION('ref_axis',(1.,0.,0.));
#9810=DIRECTION('',(0.,0.,-1.));
#9811=DIRECTION('center_axis',(0.,0.,1.));
#9812=DIRECTION('ref_axis',(1.,0.,0.));
#9813=DIRECTION('',(0.,0.,-1.));
#9814=DIRECTION('center_axis',(0.,0.,1.));
#9815=DIRECTION('ref_axis',(1.,0.,0.));
#9816=DIRECTION('',(0.,0.,-1.));
#9817=DIRECTION('center_axis',(0.,0.,1.));
#9818=DIRECTION('ref_axis',(1.,0.,0.));
#9819=DIRECTION('',(0.,0.,-1.));
#9820=DIRECTION('center_axis',(0.,0.,1.));
#9821=DIRECTION('ref_axis',(1.,0.,0.));
#9822=DIRECTION('',(0.,0.,-1.));
#9823=DIRECTION('center_axis',(0.,0.,1.));
#9824=DIRECTION('ref_axis',(1.,0.,0.));
#9825=DIRECTION('',(0.,0.,-1.));
#9826=DIRECTION('center_axis',(0.,0.,1.));
#9827=DIRECTION('ref_axis',(1.,0.,0.));
#9828=DIRECTION('',(0.,0.,-1.));
#9829=DIRECTION('center_axis',(0.,0.,1.));
#9830=DIRECTION('ref_axis',(1.,0.,0.));
#9831=DIRECTION('',(0.,0.,-1.));
#9832=DIRECTION('center_axis',(0.,0.,1.));
#9833=DIRECTION('ref_axis',(1.,0.,0.));
#9834=DIRECTION('',(0.,0.,-1.));
#9835=DIRECTION('center_axis',(0.,0.,1.));
#9836=DIRECTION('ref_axis',(1.,0.,0.));
#9837=DIRECTION('',(0.,0.,-1.));
#9838=DIRECTION('center_axis',(0.,0.,1.));
#9839=DIRECTION('ref_axis',(1.,0.,0.));
#9840=DIRECTION('',(0.,0.,-1.));
#9841=DIRECTION('center_axis',(0.,0.,1.));
#9842=DIRECTION('ref_axis',(1.,0.,0.));
#9843=DIRECTION('',(0.,0.,-1.));
#9844=DIRECTION('center_axis',(0.,0.,1.));
#9845=DIRECTION('ref_axis',(1.,0.,0.));
#9846=DIRECTION('',(0.,0.,-1.));
#9847=DIRECTION('center_axis',(0.,0.,1.));
#9848=DIRECTION('ref_axis',(1.,0.,0.));
#9849=DIRECTION('',(0.,0.,-1.));
#9850=DIRECTION('center_axis',(0.,0.,1.));
#9851=DIRECTION('ref_axis',(1.,0.,0.));
#9852=DIRECTION('',(0.,0.,-1.));
#9853=DIRECTION('center_axis',(0.,0.,1.));
#9854=DIRECTION('ref_axis',(1.,0.,0.));
#9855=DIRECTION('',(0.,0.,-1.));
#9856=DIRECTION('center_axis',(0.,0.,1.));
#9857=DIRECTION('ref_axis',(1.,0.,0.));
#9858=DIRECTION('',(0.,0.,-1.));
#9859=DIRECTION('center_axis',(0.,0.,1.));
#9860=DIRECTION('ref_axis',(1.,0.,0.));
#9861=DIRECTION('',(0.,0.,-1.));
#9862=DIRECTION('center_axis',(0.,0.,1.));
#9863=DIRECTION('ref_axis',(1.,0.,0.));
#9864=DIRECTION('',(0.,0.,-1.));
#9865=DIRECTION('center_axis',(0.,0.,1.));
#9866=DIRECTION('ref_axis',(1.,0.,0.));
#9867=DIRECTION('',(0.,0.,-1.));
#9868=DIRECTION('center_axis',(0.,0.,1.));
#9869=DIRECTION('ref_axis',(1.,0.,0.));
#9870=DIRECTION('',(0.,0.,-1.));
#9871=DIRECTION('center_axis',(0.,0.,1.));
#9872=DIRECTION('ref_axis',(1.,0.,0.));
#9873=DIRECTION('',(0.,0.,-1.));
#9874=DIRECTION('center_axis',(0.,0.,1.));
#9875=DIRECTION('ref_axis',(1.,0.,0.));
#9876=DIRECTION('',(0.,0.,-1.));
#9877=DIRECTION('center_axis',(0.,0.,1.));
#9878=DIRECTION('ref_axis',(1.,0.,0.));
#9879=DIRECTION('',(0.,0.,-1.));
#9880=DIRECTION('center_axis',(0.,0.,1.));
#9881=DIRECTION('ref_axis',(1.,0.,0.));
#9882=DIRECTION('',(0.,0.,-1.));
#9883=DIRECTION('center_axis',(0.,0.,1.));
#9884=DIRECTION('ref_axis',(1.,0.,0.));
#9885=DIRECTION('',(0.,0.,-1.));
#9886=DIRECTION('center_axis',(0.,0.,1.));
#9887=DIRECTION('ref_axis',(1.,0.,0.));
#9888=DIRECTION('',(0.,0.,-1.));
#9889=DIRECTION('center_axis',(0.,0.,1.));
#9890=DIRECTION('ref_axis',(1.,0.,0.));
#9891=DIRECTION('',(0.,0.,-1.));
#9892=DIRECTION('center_axis',(0.,0.,1.));
#9893=DIRECTION('ref_axis',(1.,0.,0.));
#9894=DIRECTION('',(0.,0.,-1.));
#9895=DIRECTION('center_axis',(0.,0.,1.));
#9896=DIRECTION('ref_axis',(1.,0.,0.));
#9897=DIRECTION('',(0.,0.,-1.));
#9898=DIRECTION('center_axis',(0.,0.,1.));
#9899=DIRECTION('ref_axis',(1.,0.,0.));
#9900=DIRECTION('',(0.,0.,-1.));
#9901=DIRECTION('center_axis',(0.,0.,1.));
#9902=DIRECTION('ref_axis',(1.,0.,0.));
#9903=DIRECTION('',(0.,0.,-1.));
#9904=DIRECTION('center_axis',(0.,0.,1.));
#9905=DIRECTION('ref_axis',(1.,0.,0.));
#9906=DIRECTION('',(0.,0.,-1.));
#9907=DIRECTION('center_axis',(0.,0.,1.));
#9908=DIRECTION('ref_axis',(1.,0.,0.));
#9909=DIRECTION('',(0.,0.,-1.));
#9910=DIRECTION('center_axis',(0.,0.,1.));
#9911=DIRECTION('ref_axis',(1.,0.,0.));
#9912=DIRECTION('',(0.,0.,-1.));
#9913=DIRECTION('center_axis',(0.,0.,1.));
#9914=DIRECTION('ref_axis',(1.,0.,0.));
#9915=DIRECTION('',(0.,0.,-1.));
#9916=DIRECTION('center_axis',(0.,0.,1.));
#9917=DIRECTION('ref_axis',(1.,0.,0.));
#9918=DIRECTION('',(0.,0.,-1.));
#9919=DIRECTION('center_axis',(0.,0.,1.));
#9920=DIRECTION('ref_axis',(1.,0.,0.));
#9921=DIRECTION('',(0.,0.,-1.));
#9922=DIRECTION('center_axis',(0.,0.,1.));
#9923=DIRECTION('ref_axis',(1.,0.,0.));
#9924=DIRECTION('',(0.,0.,-1.));
#9925=DIRECTION('center_axis',(0.,0.,1.));
#9926=DIRECTION('ref_axis',(1.,0.,0.));
#9927=DIRECTION('',(0.,0.,-1.));
#9928=DIRECTION('center_axis',(0.,0.,1.));
#9929=DIRECTION('ref_axis',(1.,0.,0.));
#9930=DIRECTION('',(0.,0.,-1.));
#9931=DIRECTION('center_axis',(0.,0.,1.));
#9932=DIRECTION('ref_axis',(1.,0.,0.));
#9933=DIRECTION('',(0.,0.,-1.));
#9934=DIRECTION('center_axis',(0.,0.,1.));
#9935=DIRECTION('ref_axis',(1.,0.,0.));
#9936=DIRECTION('',(0.,0.,-1.));
#9937=DIRECTION('center_axis',(0.,0.,1.));
#9938=DIRECTION('ref_axis',(1.,0.,0.));
#9939=DIRECTION('',(0.,0.,-1.));
#9940=DIRECTION('center_axis',(0.,0.,1.));
#9941=DIRECTION('ref_axis',(1.,0.,0.));
#9942=DIRECTION('',(0.,0.,-1.));
#9943=DIRECTION('center_axis',(0.,0.,1.));
#9944=DIRECTION('ref_axis',(1.,0.,0.));
#9945=DIRECTION('',(0.,0.,-1.));
#9946=DIRECTION('center_axis',(0.,0.,1.));
#9947=DIRECTION('ref_axis',(1.,0.,0.));
#9948=DIRECTION('',(0.,0.,-1.));
#9949=DIRECTION('center_axis',(0.,0.,1.));
#9950=DIRECTION('ref_axis',(1.,0.,0.));
#9951=DIRECTION('',(0.,0.,-1.));
#9952=DIRECTION('center_axis',(0.,0.,1.));
#9953=DIRECTION('ref_axis',(1.,0.,0.));
#9954=DIRECTION('',(0.,0.,-1.));
#9955=DIRECTION('center_axis',(0.,0.,1.));
#9956=DIRECTION('ref_axis',(1.,0.,0.));
#9957=DIRECTION('',(0.,0.,-1.));
#9958=DIRECTION('center_axis',(0.,0.,1.));
#9959=DIRECTION('ref_axis',(1.,0.,0.));
#9960=DIRECTION('',(0.,0.,-1.));
#9961=DIRECTION('center_axis',(0.,0.,1.));
#9962=DIRECTION('ref_axis',(1.,0.,0.));
#9963=DIRECTION('',(0.,0.,-1.));
#9964=DIRECTION('center_axis',(0.,0.,1.));
#9965=DIRECTION('ref_axis',(1.,0.,0.));
#9966=DIRECTION('',(0.,0.,-1.));
#9967=DIRECTION('center_axis',(0.,0.,1.));
#9968=DIRECTION('ref_axis',(1.,0.,0.));
#9969=DIRECTION('',(0.,0.,-1.));
#9970=DIRECTION('center_axis',(0.,0.,1.));
#9971=DIRECTION('ref_axis',(1.,0.,0.));
#9972=DIRECTION('',(0.,0.,-1.));
#9973=DIRECTION('center_axis',(0.,0.,1.));
#9974=DIRECTION('ref_axis',(1.,0.,0.));
#9975=DIRECTION('',(0.,0.,-1.));
#9976=DIRECTION('center_axis',(0.,0.,1.));
#9977=DIRECTION('ref_axis',(1.,0.,0.));
#9978=DIRECTION('',(0.,0.,-1.));
#9979=DIRECTION('center_axis',(0.,0.,1.));
#9980=DIRECTION('ref_axis',(1.,0.,0.));
#9981=DIRECTION('',(0.,0.,-1.));
#9982=DIRECTION('center_axis',(0.,0.,1.));
#9983=DIRECTION('ref_axis',(1.,0.,0.));
#9984=DIRECTION('',(0.,0.,-1.));
#9985=DIRECTION('center_axis',(0.,0.,1.));
#9986=DIRECTION('ref_axis',(1.,0.,0.));
#9987=DIRECTION('',(0.,0.,-1.));
#9988=DIRECTION('center_axis',(0.,0.,1.));
#9989=DIRECTION('ref_axis',(1.,0.,0.));
#9990=DIRECTION('',(0.,0.,-1.));
#9991=DIRECTION('center_axis',(0.,0.,1.));
#9992=DIRECTION('ref_axis',(1.,0.,0.));
#9993=DIRECTION('',(0.,0.,-1.));
#9994=DIRECTION('center_axis',(0.,0.,1.));
#9995=DIRECTION('ref_axis',(1.,0.,0.));
#9996=DIRECTION('',(0.,0.,-1.));
#9997=DIRECTION('center_axis',(0.,0.,1.));
#9998=DIRECTION('ref_axis',(1.,0.,0.));
#9999=DIRECTION('',(0.,0.,-1.));
#10000=DIRECTION('center_axis',(0.,0.,1.));
#10001=DIRECTION('ref_axis',(1.,0.,0.));
#10002=DIRECTION('',(0.,0.,-1.));
#10003=DIRECTION('center_axis',(0.,0.,1.));
#10004=DIRECTION('ref_axis',(1.,0.,0.));
#10005=DIRECTION('',(0.,0.,-1.));
#10006=DIRECTION('center_axis',(0.,0.,1.));
#10007=DIRECTION('ref_axis',(1.,0.,0.));
#10008=DIRECTION('',(0.,0.,-1.));
#10009=DIRECTION('center_axis',(0.,0.,1.));
#10010=DIRECTION('ref_axis',(1.,0.,0.));
#10011=DIRECTION('',(0.,0.,-1.));
#10012=DIRECTION('center_axis',(0.,0.,1.));
#10013=DIRECTION('ref_axis',(1.,0.,0.));
#10014=DIRECTION('',(0.,0.,-1.));
#10015=DIRECTION('center_axis',(0.,0.,1.));
#10016=DIRECTION('ref_axis',(1.,0.,0.));
#10017=DIRECTION('',(0.,0.,-1.));
#10018=DIRECTION('center_axis',(0.,0.,1.));
#10019=DIRECTION('ref_axis',(1.,0.,0.));
#10020=DIRECTION('',(0.,0.,-1.));
#10021=DIRECTION('center_axis',(0.,0.,1.));
#10022=DIRECTION('ref_axis',(1.,0.,0.));
#10023=DIRECTION('',(0.,0.,-1.));
#10024=DIRECTION('center_axis',(0.,0.,1.));
#10025=DIRECTION('ref_axis',(1.,0.,0.));
#10026=DIRECTION('',(0.,0.,-1.));
#10027=DIRECTION('center_axis',(0.,0.,1.));
#10028=DIRECTION('ref_axis',(1.,0.,0.));
#10029=DIRECTION('',(0.,0.,-1.));
#10030=DIRECTION('center_axis',(0.,0.,1.));
#10031=DIRECTION('ref_axis',(1.,0.,0.));
#10032=DIRECTION('',(0.,0.,-1.));
#10033=DIRECTION('center_axis',(0.,0.,1.));
#10034=DIRECTION('ref_axis',(1.,0.,0.));
#10035=DIRECTION('',(0.,0.,-1.));
#10036=DIRECTION('center_axis',(0.,0.,1.));
#10037=DIRECTION('ref_axis',(1.,0.,0.));
#10038=DIRECTION('',(0.,0.,-1.));
#10039=DIRECTION('center_axis',(0.,0.,1.));
#10040=DIRECTION('ref_axis',(1.,0.,0.));
#10041=DIRECTION('',(0.,0.,-1.));
#10042=DIRECTION('center_axis',(0.,0.,1.));
#10043=DIRECTION('ref_axis',(1.,0.,0.));
#10044=DIRECTION('',(0.,0.,-1.));
#10045=DIRECTION('center_axis',(0.,0.,1.));
#10046=DIRECTION('ref_axis',(1.,0.,0.));
#10047=DIRECTION('',(0.,0.,-1.));
#10048=DIRECTION('center_axis',(0.,0.,1.));
#10049=DIRECTION('ref_axis',(1.,0.,0.));
#10050=DIRECTION('',(0.,0.,-1.));
#10051=DIRECTION('center_axis',(0.,0.,1.));
#10052=DIRECTION('ref_axis',(1.,0.,0.));
#10053=DIRECTION('',(0.,0.,-1.));
#10054=DIRECTION('center_axis',(0.,0.,1.));
#10055=DIRECTION('ref_axis',(1.,0.,0.));
#10056=DIRECTION('',(0.,0.,-1.));
#10057=DIRECTION('center_axis',(0.,0.,1.));
#10058=DIRECTION('ref_axis',(1.,0.,0.));
#10059=DIRECTION('',(0.,0.,-1.));
#10060=DIRECTION('center_axis',(0.,0.,1.));
#10061=DIRECTION('ref_axis',(1.,0.,0.));
#10062=DIRECTION('',(0.,0.,-1.));
#10063=DIRECTION('center_axis',(0.,0.,1.));
#10064=DIRECTION('ref_axis',(1.,0.,0.));
#10065=DIRECTION('',(0.,0.,-1.));
#10066=DIRECTION('center_axis',(0.,0.,1.));
#10067=DIRECTION('ref_axis',(1.,0.,0.));
#10068=DIRECTION('',(0.,0.,-1.));
#10069=DIRECTION('center_axis',(0.,0.,1.));
#10070=DIRECTION('ref_axis',(1.,0.,0.));
#10071=DIRECTION('',(0.,0.,-1.));
#10072=DIRECTION('center_axis',(0.,0.,1.));
#10073=DIRECTION('ref_axis',(1.,0.,0.));
#10074=DIRECTION('',(0.,0.,-1.));
#10075=DIRECTION('center_axis',(0.,0.,1.));
#10076=DIRECTION('ref_axis',(1.,0.,0.));
#10077=DIRECTION('',(0.,0.,-1.));
#10078=DIRECTION('center_axis',(0.,0.,1.));
#10079=DIRECTION('ref_axis',(1.,0.,0.));
#10080=DIRECTION('',(0.,0.,-1.));
#10081=DIRECTION('center_axis',(0.,0.,1.));
#10082=DIRECTION('ref_axis',(1.,0.,0.));
#10083=DIRECTION('',(0.,0.,-1.));
#10084=DIRECTION('center_axis',(0.,0.,1.));
#10085=DIRECTION('ref_axis',(1.,0.,0.));
#10086=DIRECTION('',(0.,0.,-1.));
#10087=DIRECTION('center_axis',(0.,0.,1.));
#10088=DIRECTION('ref_axis',(-0.457993717575288,-0.888955428951063,0.));
#10089=DIRECTION('',(0.,0.,1.));
#10090=DIRECTION('center_axis',(0.,0.,1.));
#10091=DIRECTION('ref_axis',(1.,-1.75643374117547E-12,0.));
#10092=DIRECTION('center_axis',(0.,0.,1.));
#10093=DIRECTION('ref_axis',(1.,-1.75643374117547E-12,0.));
#10094=DIRECTION('',(0.,0.,1.));
#10095=DIRECTION('center_axis',(0.,0.,1.));
#10096=DIRECTION('ref_axis',(1.,-1.75643374117547E-12,0.));
#10097=DIRECTION('',(0.,0.,1.));
#10098=DIRECTION('center_axis',(0.,0.,1.));
#10099=DIRECTION('ref_axis',(1.,-1.75643374117547E-12,0.));
#10100=DIRECTION('',(0.,0.,1.));
#10101=DIRECTION('center_axis',(0.,0.,1.));
#10102=DIRECTION('ref_axis',(1.,-1.75643374117547E-12,0.));
#10103=DIRECTION('',(0.,0.,1.));
#10104=DIRECTION('center_axis',(0.,0.,1.));
#10105=DIRECTION('ref_axis',(1.,-1.75643374117547E-12,0.));
#10106=DIRECTION('',(0.,0.,1.));
#10107=DIRECTION('center_axis',(0.,0.,1.));
#10108=DIRECTION('ref_axis',(1.,-1.75643374117547E-12,0.));
#10109=DIRECTION('',(0.,0.,1.));
#10110=DIRECTION('center_axis',(0.,0.,1.));
#10111=DIRECTION('ref_axis',(1.,-1.75643374117547E-12,0.));
#10112=DIRECTION('',(0.,0.,1.));
#10113=DIRECTION('center_axis',(0.,0.,1.));
#10114=DIRECTION('ref_axis',(1.,-1.75643374117547E-12,0.));
#10115=DIRECTION('',(0.,0.,1.));
#10116=DIRECTION('center_axis',(0.,0.,1.));
#10117=DIRECTION('ref_axis',(1.,-1.75643374117547E-12,0.));
#10118=DIRECTION('',(0.,0.,1.));
#10119=DIRECTION('center_axis',(0.,0.,1.));
#10120=DIRECTION('ref_axis',(1.,-1.75643374117547E-12,0.));
#10121=DIRECTION('',(0.,0.,1.));
#10122=DIRECTION('center_axis',(0.,0.,1.));
#10123=DIRECTION('ref_axis',(1.,-1.75643374117547E-12,0.));
#10124=DIRECTION('',(0.,0.,1.));
#10125=DIRECTION('center_axis',(0.,0.,1.));
#10126=DIRECTION('ref_axis',(1.,-1.75643374117547E-12,0.));
#10127=DIRECTION('',(0.,0.,1.));
#10128=DIRECTION('center_axis',(0.,0.,1.));
#10129=DIRECTION('ref_axis',(1.,-1.75643374117547E-12,0.));
#10130=DIRECTION('',(0.,0.,1.));
#10131=DIRECTION('center_axis',(0.,0.,1.));
#10132=DIRECTION('ref_axis',(1.,-1.75643374117547E-12,0.));
#10133=DIRECTION('',(0.,0.,1.));
#10134=DIRECTION('center_axis',(0.,0.,1.));
#10135=DIRECTION('ref_axis',(1.,-1.75643374117547E-12,0.));
#10136=DIRECTION('',(0.,0.,1.));
#10137=DIRECTION('center_axis',(0.,0.,1.));
#10138=DIRECTION('ref_axis',(1.,-1.75643374117547E-12,0.));
#10139=DIRECTION('',(0.,0.,1.));
#10140=DIRECTION('center_axis',(0.,0.,1.));
#10141=DIRECTION('ref_axis',(1.,-1.75643374117547E-12,0.));
#10142=DIRECTION('',(0.,0.,1.));
#10143=DIRECTION('center_axis',(0.,0.,1.));
#10144=DIRECTION('ref_axis',(1.,-1.75643374117547E-12,0.));
#10145=DIRECTION('',(0.,0.,1.));
#10146=DIRECTION('center_axis',(0.,0.,1.));
#10147=DIRECTION('ref_axis',(1.,-1.75643374117547E-12,0.));
#10148=DIRECTION('',(0.,0.,1.));
#10149=DIRECTION('center_axis',(0.,0.,1.));
#10150=DIRECTION('ref_axis',(1.,-1.75643374117547E-12,0.));
#10151=DIRECTION('',(0.,0.,1.));
#10152=DIRECTION('center_axis',(0.,0.,1.));
#10153=DIRECTION('ref_axis',(1.,-1.75643374117547E-12,0.));
#10154=DIRECTION('',(0.,0.,1.));
#10155=DIRECTION('center_axis',(0.,0.,1.));
#10156=DIRECTION('ref_axis',(1.,-1.75643374117547E-12,0.));
#10157=DIRECTION('',(0.,0.,1.));
#10158=DIRECTION('center_axis',(0.,0.,1.));
#10159=DIRECTION('ref_axis',(1.,-1.75643374117547E-12,0.));
#10160=DIRECTION('',(0.,0.,1.));
#10161=DIRECTION('center_axis',(0.,0.,1.));
#10162=DIRECTION('ref_axis',(1.,-1.75643374117547E-12,0.));
#10163=DIRECTION('',(0.,0.,1.));
#10164=DIRECTION('center_axis',(0.,0.,1.));
#10165=DIRECTION('ref_axis',(1.,-1.75643374117547E-12,0.));
#10166=DIRECTION('',(0.,0.,1.));
#10167=DIRECTION('center_axis',(0.,0.,1.));
#10168=DIRECTION('ref_axis',(1.,-1.75643374117547E-12,0.));
#10169=DIRECTION('',(0.,0.,1.));
#10170=DIRECTION('center_axis',(0.,0.,1.));
#10171=DIRECTION('ref_axis',(1.,-1.75643374117547E-12,0.));
#10172=DIRECTION('',(0.,0.,1.));
#10173=DIRECTION('center_axis',(0.,0.,1.));
#10174=DIRECTION('ref_axis',(1.,-1.75643374117547E-12,0.));
#10175=DIRECTION('',(0.,0.,1.));
#10176=DIRECTION('center_axis',(0.,0.,1.));
#10177=DIRECTION('ref_axis',(1.,-1.75643374117547E-12,0.));
#10178=DIRECTION('',(0.,0.,1.));
#10179=DIRECTION('center_axis',(0.,0.,1.));
#10180=DIRECTION('ref_axis',(1.,-1.75643374117547E-12,0.));
#10181=DIRECTION('',(0.,0.,1.));
#10182=DIRECTION('center_axis',(0.,0.,1.));
#10183=DIRECTION('ref_axis',(1.,-1.75643374117547E-12,0.));
#10184=DIRECTION('',(0.,0.,1.));
#10185=DIRECTION('center_axis',(0.,0.,1.));
#10186=DIRECTION('ref_axis',(1.,-1.75643374117547E-12,0.));
#10187=DIRECTION('',(0.,0.,1.));
#10188=DIRECTION('center_axis',(0.,0.,1.));
#10189=DIRECTION('ref_axis',(1.,-1.75643374117547E-12,0.));
#10190=DIRECTION('',(0.,0.,1.));
#10191=DIRECTION('center_axis',(0.,0.,1.));
#10192=DIRECTION('ref_axis',(1.,-1.75643374117547E-12,0.));
#10193=DIRECTION('',(0.,0.,1.));
#10194=DIRECTION('center_axis',(0.,0.,1.));
#10195=DIRECTION('ref_axis',(1.,-1.75643374117547E-12,0.));
#10196=DIRECTION('',(0.,0.,1.));
#10197=DIRECTION('center_axis',(0.,0.,1.));
#10198=DIRECTION('ref_axis',(1.,-1.75643374117547E-12,0.));
#10199=DIRECTION('',(0.,0.,1.));
#10200=DIRECTION('center_axis',(0.,0.,1.));
#10201=DIRECTION('ref_axis',(1.,-1.75643374117547E-12,0.));
#10202=DIRECTION('',(0.,0.,1.));
#10203=DIRECTION('center_axis',(0.,0.,1.));
#10204=DIRECTION('ref_axis',(1.,-1.75643374117547E-12,0.));
#10205=DIRECTION('',(0.,0.,1.));
#10206=DIRECTION('center_axis',(0.,0.,1.));
#10207=DIRECTION('ref_axis',(1.,-1.75643374117547E-12,0.));
#10208=DIRECTION('',(0.,0.,1.));
#10209=DIRECTION('center_axis',(0.,0.,1.));
#10210=DIRECTION('ref_axis',(1.,-1.75643374117547E-12,0.));
#10211=DIRECTION('',(0.,0.,1.));
#10212=DIRECTION('center_axis',(0.,0.,1.));
#10213=DIRECTION('ref_axis',(1.,-1.75643374117547E-12,0.));
#10214=DIRECTION('',(0.,0.,1.));
#10215=DIRECTION('center_axis',(0.,0.,1.));
#10216=DIRECTION('ref_axis',(1.,-1.75643374117547E-12,0.));
#10217=DIRECTION('',(0.,0.,1.));
#10218=DIRECTION('center_axis',(0.,0.,1.));
#10219=DIRECTION('ref_axis',(1.,-1.75643374117547E-12,0.));
#10220=DIRECTION('',(0.,0.,1.));
#10221=DIRECTION('center_axis',(0.,0.,1.));
#10222=DIRECTION('ref_axis',(1.,-1.75643374117547E-12,0.));
#10223=DIRECTION('',(0.,0.,1.));
#10224=DIRECTION('center_axis',(0.,0.,1.));
#10225=DIRECTION('ref_axis',(1.,-1.75643374117547E-12,0.));
#10226=DIRECTION('',(0.,0.,1.));
#10227=DIRECTION('center_axis',(0.,0.,1.));
#10228=DIRECTION('ref_axis',(1.,-1.75643374117547E-12,0.));
#10229=DIRECTION('',(0.,0.,1.));
#10230=DIRECTION('center_axis',(0.,0.,1.));
#10231=DIRECTION('ref_axis',(1.,-1.75643374117547E-12,0.));
#10232=DIRECTION('',(0.,0.,1.));
#10233=DIRECTION('center_axis',(0.,0.,1.));
#10234=DIRECTION('ref_axis',(1.,-1.75643374117547E-12,0.));
#10235=DIRECTION('',(0.,0.,1.));
#10236=DIRECTION('center_axis',(0.,0.,1.));
#10237=DIRECTION('ref_axis',(1.,-1.75643374117547E-12,0.));
#10238=DIRECTION('',(0.,0.,1.));
#10239=DIRECTION('center_axis',(0.,0.,1.));
#10240=DIRECTION('ref_axis',(1.,-1.75643374117547E-12,0.));
#10241=DIRECTION('',(0.,0.,1.));
#10242=DIRECTION('center_axis',(0.,0.,1.));
#10243=DIRECTION('ref_axis',(1.,-1.75643374117547E-12,0.));
#10244=DIRECTION('',(0.,0.,1.));
#10245=DIRECTION('center_axis',(0.,0.,1.));
#10246=DIRECTION('ref_axis',(1.,-1.75643374117547E-12,0.));
#10247=DIRECTION('',(0.,0.,1.));
#10248=DIRECTION('center_axis',(0.,0.,1.));
#10249=DIRECTION('ref_axis',(1.,-1.75643374117547E-12,0.));
#10250=DIRECTION('',(0.,0.,1.));
#10251=DIRECTION('center_axis',(0.,0.,1.));
#10252=DIRECTION('ref_axis',(1.,-1.75643374117547E-12,0.));
#10253=DIRECTION('',(0.,0.,1.));
#10254=DIRECTION('center_axis',(0.,0.,1.));
#10255=DIRECTION('ref_axis',(1.,-1.75643374117547E-12,0.));
#10256=DIRECTION('',(0.,0.,1.));
#10257=DIRECTION('center_axis',(0.,0.,1.));
#10258=DIRECTION('ref_axis',(1.,-1.75643374117547E-12,0.));
#10259=DIRECTION('',(0.,0.,1.));
#10260=DIRECTION('center_axis',(0.,0.,1.));
#10261=DIRECTION('ref_axis',(1.,-1.75643374117547E-12,0.));
#10262=DIRECTION('',(0.,0.,1.));
#10263=DIRECTION('center_axis',(0.,0.,1.));
#10264=DIRECTION('ref_axis',(1.,-1.75643374117547E-12,0.));
#10265=DIRECTION('',(0.,0.,1.));
#10266=DIRECTION('center_axis',(0.,0.,1.));
#10267=DIRECTION('ref_axis',(1.,-1.75643374117547E-12,0.));
#10268=DIRECTION('',(0.,0.,1.));
#10269=DIRECTION('center_axis',(0.,0.,1.));
#10270=DIRECTION('ref_axis',(1.,-1.75643374117547E-12,0.));
#10271=DIRECTION('',(0.,0.,1.));
#10272=DIRECTION('center_axis',(0.,0.,1.));
#10273=DIRECTION('ref_axis',(1.,-1.75643374117547E-12,0.));
#10274=DIRECTION('',(0.,0.,1.));
#10275=DIRECTION('center_axis',(0.,0.,1.));
#10276=DIRECTION('ref_axis',(1.,-1.75643374117547E-12,0.));
#10277=DIRECTION('',(0.,0.,1.));
#10278=DIRECTION('center_axis',(0.,0.,1.));
#10279=DIRECTION('ref_axis',(1.,-1.75643374117547E-12,0.));
#10280=DIRECTION('',(0.,0.,1.));
#10281=DIRECTION('center_axis',(0.,0.,1.));
#10282=DIRECTION('ref_axis',(1.,-1.75643374117547E-12,0.));
#10283=DIRECTION('',(0.,0.,1.));
#10284=DIRECTION('center_axis',(0.,0.,1.));
#10285=DIRECTION('ref_axis',(1.,-1.75643374117547E-12,0.));
#10286=DIRECTION('',(0.,0.,1.));
#10287=DIRECTION('center_axis',(0.,0.,1.));
#10288=DIRECTION('ref_axis',(1.,-1.75643374117547E-12,0.));
#10289=DIRECTION('',(0.,0.,1.));
#10290=DIRECTION('center_axis',(0.,0.,1.));
#10291=DIRECTION('ref_axis',(1.,-1.75643374117547E-12,0.));
#10292=DIRECTION('',(0.,0.,1.));
#10293=DIRECTION('center_axis',(0.,0.,1.));
#10294=DIRECTION('ref_axis',(1.,-1.75643374117547E-12,0.));
#10295=DIRECTION('',(0.,0.,1.));
#10296=DIRECTION('center_axis',(0.,0.,1.));
#10297=DIRECTION('ref_axis',(1.,-1.75643374117547E-12,0.));
#10298=DIRECTION('',(0.,0.,1.));
#10299=DIRECTION('center_axis',(0.,0.,1.));
#10300=DIRECTION('ref_axis',(1.,-1.75643374117547E-12,0.));
#10301=DIRECTION('',(0.,0.,1.));
#10302=DIRECTION('center_axis',(0.,0.,1.));
#10303=DIRECTION('ref_axis',(1.,-1.75643374117547E-12,0.));
#10304=DIRECTION('',(0.,0.,1.));
#10305=DIRECTION('center_axis',(0.,0.,1.));
#10306=DIRECTION('ref_axis',(1.,-1.75643374117547E-12,0.));
#10307=DIRECTION('',(0.,0.,1.));
#10308=DIRECTION('center_axis',(0.,0.,1.));
#10309=DIRECTION('ref_axis',(1.,-1.75643374117547E-12,0.));
#10310=DIRECTION('',(0.,0.,1.));
#10311=DIRECTION('center_axis',(0.,0.,1.));
#10312=DIRECTION('ref_axis',(1.,-1.75643374117547E-12,0.));
#10313=DIRECTION('',(0.,0.,1.));
#10314=DIRECTION('center_axis',(0.,0.,1.));
#10315=DIRECTION('ref_axis',(1.,-1.75643374117547E-12,0.));
#10316=DIRECTION('',(0.,0.,1.));
#10317=DIRECTION('center_axis',(0.,0.,1.));
#10318=DIRECTION('ref_axis',(1.,-1.75643374117547E-12,0.));
#10319=DIRECTION('',(0.,0.,1.));
#10320=DIRECTION('center_axis',(0.,0.,1.));
#10321=DIRECTION('ref_axis',(1.,-1.75643374117547E-12,0.));
#10322=DIRECTION('',(0.,0.,1.));
#10323=DIRECTION('center_axis',(0.,0.,1.));
#10324=DIRECTION('ref_axis',(1.,-1.75643374117547E-12,0.));
#10325=DIRECTION('',(0.,0.,1.));
#10326=DIRECTION('center_axis',(0.,0.,1.));
#10327=DIRECTION('ref_axis',(1.,-1.75643374117547E-12,0.));
#10328=DIRECTION('',(0.,0.,1.));
#10329=DIRECTION('center_axis',(0.,0.,1.));
#10330=DIRECTION('ref_axis',(1.,-1.75643374117547E-12,0.));
#10331=DIRECTION('',(0.,0.,1.));
#10332=DIRECTION('center_axis',(0.,0.,1.));
#10333=DIRECTION('ref_axis',(1.,-1.75643374117547E-12,0.));
#10334=DIRECTION('',(0.,0.,1.));
#10335=DIRECTION('center_axis',(0.,0.,1.));
#10336=DIRECTION('ref_axis',(1.,-1.75643374117547E-12,0.));
#10337=DIRECTION('',(0.,0.,1.));
#10338=DIRECTION('center_axis',(0.,0.,1.));
#10339=DIRECTION('ref_axis',(1.,-1.75643374117547E-12,0.));
#10340=DIRECTION('',(0.,0.,1.));
#10341=DIRECTION('center_axis',(0.,0.,1.));
#10342=DIRECTION('ref_axis',(1.,-1.75643374117547E-12,0.));
#10343=DIRECTION('',(0.,0.,1.));
#10344=DIRECTION('center_axis',(0.,0.,1.));
#10345=DIRECTION('ref_axis',(1.,-1.75643374117547E-12,0.));
#10346=DIRECTION('',(0.,0.,1.));
#10347=DIRECTION('center_axis',(0.,0.,1.));
#10348=DIRECTION('ref_axis',(1.,-1.75643374117547E-12,0.));
#10349=DIRECTION('',(0.,0.,1.));
#10350=DIRECTION('center_axis',(0.,0.,1.));
#10351=DIRECTION('ref_axis',(1.,-1.75643374117547E-12,0.));
#10352=DIRECTION('',(0.,0.,1.));
#10353=DIRECTION('center_axis',(0.,0.,1.));
#10354=DIRECTION('ref_axis',(1.,-1.75643374117547E-12,0.));
#10355=DIRECTION('',(0.,0.,1.));
#10356=DIRECTION('center_axis',(0.,0.,1.));
#10357=DIRECTION('ref_axis',(1.,-1.75643374117547E-12,0.));
#10358=DIRECTION('',(0.,0.,1.));
#10359=DIRECTION('center_axis',(0.,0.,1.));
#10360=DIRECTION('ref_axis',(1.,-1.75643374117547E-12,0.));
#10361=DIRECTION('',(0.,0.,1.));
#10362=DIRECTION('center_axis',(0.,0.,1.));
#10363=DIRECTION('ref_axis',(1.,-1.75643374117547E-12,0.));
#10364=DIRECTION('',(0.,0.,1.));
#10365=DIRECTION('center_axis',(0.,0.,1.));
#10366=DIRECTION('ref_axis',(1.,-1.75643374117547E-12,0.));
#10367=DIRECTION('',(0.,0.,1.));
#10368=DIRECTION('center_axis',(0.,0.,1.));
#10369=DIRECTION('ref_axis',(1.,-1.75643374117547E-12,0.));
#10370=DIRECTION('',(0.,0.,1.));
#10371=DIRECTION('center_axis',(0.,0.,1.));
#10372=DIRECTION('ref_axis',(1.,0.,0.));
#10373=DIRECTION('center_axis',(0.,0.,1.));
#10374=DIRECTION('ref_axis',(1.,0.,0.));
#10375=DIRECTION('',(0.,0.,1.));
#10376=DIRECTION('center_axis',(0.,0.,-1.));
#10377=DIRECTION('ref_axis',(1.,0.,0.));
#10378=DIRECTION('center_axis',(0.,0.,1.));
#10379=DIRECTION('ref_axis',(1.,0.,0.));
#10380=DIRECTION('center_axis',(0.,0.,1.));
#10381=DIRECTION('ref_axis',(1.,0.,0.));
#10382=DIRECTION('',(0.,0.,1.));
#10383=DIRECTION('center_axis',(0.,0.,-1.));
#10384=DIRECTION('ref_axis',(1.,0.,0.));
#10385=DIRECTION('center_axis',(0.,0.,1.));
#10386=DIRECTION('ref_axis',(1.,0.,0.));
#10387=DIRECTION('center_axis',(0.,0.,1.));
#10388=DIRECTION('ref_axis',(1.,0.,0.));
#10389=DIRECTION('',(0.,0.,1.));
#10390=DIRECTION('center_axis',(0.,0.,-1.));
#10391=DIRECTION('ref_axis',(1.,0.,0.));
#10392=DIRECTION('center_axis',(0.,0.,1.));
#10393=DIRECTION('ref_axis',(1.,0.,0.));
#10394=DIRECTION('center_axis',(0.,0.,1.));
#10395=DIRECTION('ref_axis',(1.,0.,0.));
#10396=DIRECTION('',(0.,0.,1.));
#10397=DIRECTION('center_axis',(0.,0.,-1.));
#10398=DIRECTION('ref_axis',(1.,0.,0.));
#10399=DIRECTION('center_axis',(0.,0.,1.));
#10400=DIRECTION('ref_axis',(1.,0.,0.));
#10401=DIRECTION('center_axis',(0.,0.,1.));
#10402=DIRECTION('ref_axis',(1.,0.,0.));
#10403=DIRECTION('',(0.,0.,1.));
#10404=DIRECTION('center_axis',(0.,0.,-1.));
#10405=DIRECTION('ref_axis',(1.,0.,0.));
#10406=DIRECTION('center_axis',(0.,0.,1.));
#10407=DIRECTION('ref_axis',(1.,0.,0.));
#10408=DIRECTION('center_axis',(0.,0.,1.));
#10409=DIRECTION('ref_axis',(1.,0.,0.));
#10410=DIRECTION('',(0.,0.,1.));
#10411=DIRECTION('center_axis',(0.,0.,-1.));
#10412=DIRECTION('ref_axis',(1.,0.,0.));
#10413=DIRECTION('center_axis',(0.,0.,1.));
#10414=DIRECTION('ref_axis',(1.,0.,0.));
#10415=DIRECTION('center_axis',(0.,0.,1.));
#10416=DIRECTION('ref_axis',(1.,0.,0.));
#10417=DIRECTION('center_axis',(0.,0.,-1.));
#10418=DIRECTION('ref_axis',(1.,-1.75643374117547E-12,0.));
#10419=DIRECTION('center_axis',(0.,0.,1.));
#10420=DIRECTION('ref_axis',(1.,0.,0.));
#10421=DIRECTION('',(0.,0.,-1.));
#10422=DIRECTION('center_axis',(0.,0.,1.));
#10423=DIRECTION('ref_axis',(1.,0.,0.));
#10424=DIRECTION('center_axis',(0.,0.,1.));
#10425=DIRECTION('ref_axis',(1.,0.,0.));
#10426=DIRECTION('center_axis',(0.,0.,1.));
#10427=DIRECTION('ref_axis',(1.,-1.75643374117547E-12,0.));
#10428=DIRECTION('center_axis',(0.,0.,1.));
#10429=DIRECTION('ref_axis',(1.,0.,0.));
#10430=DIRECTION('center_axis',(0.,0.,-1.));
#10431=DIRECTION('ref_axis',(1.,0.,0.));
#10432=DIRECTION('center_axis',(0.,0.,1.));
#10433=DIRECTION('ref_axis',(1.,0.,0.));
#11773=CARTESIAN_POINT('',(0.,0.,0.));
#11774=CARTESIAN_POINT('Origin',(-8.5,0.,1.8));
#11775=CARTESIAN_POINT('',(-9.68946857590504,0.000315360110501401,1.89626312369518));
#11776=CARTESIAN_POINT('',(-9.68870505254289,0.000360304848219705,1.85373687630491));
#11777=CARTESIAN_POINT('',(-9.688225,-1.45515594291686E-16,1.8));
#11778=CARTESIAN_POINT('',(-7.98816118883252,1.07233375495116,1.8));
#11779=CARTESIAN_POINT('Ctrl Pts',(-9.688225,1.66533453693773E-15,1.89626312369518));
#11780=CARTESIAN_POINT('Ctrl Pts',(-9.688225,0.298712821306094,1.88425993690586));
#11781=CARTESIAN_POINT('Ctrl Pts',(-9.57054245632586,0.595858078271529,
1.87225675011654));
#11782=CARTESIAN_POINT('Ctrl Pts',(-9.36601586214935,0.813569405232719,
1.86025356332722));
#11783=CARTESIAN_POINT('Ctrl Pts',(-9.16148926797284,1.03128073219391,1.8482503765379));
#11784=CARTESIAN_POINT('Ctrl Pts',(-8.87226522412846,1.16727314847136,1.83624718974859));
#11785=CARTESIAN_POINT('Ctrl Pts',(-8.57413435701451,1.1859100926019,1.82424400295927));
#11786=CARTESIAN_POINT('Ctrl Pts',(-8.37341306103911,1.1984577084027,1.81616266863951));
#11787=CARTESIAN_POINT('Ctrl Pts',(-8.16965911380568,1.15896506886691,1.80808133431976));
#11788=CARTESIAN_POINT('Ctrl Pts',(-7.98816118883253,1.07233375495117,1.8));
#11789=CARTESIAN_POINT('',(-9.0118388111672,1.0723337549513,1.8));
#11790=CARTESIAN_POINT('Origin',(-8.5,0.,1.8));
#11791=CARTESIAN_POINT('Ctrl Pts',(-9.0118388111672,1.0723337549513,1.79999999999999));
#11792=CARTESIAN_POINT('Ctrl Pts',(-9.19046954816081,0.987070987050382,
1.8079536705758));
#11793=CARTESIAN_POINT('Ctrl Pts',(-9.34601190633409,0.856319638879147,
1.81590734115161));
#11794=CARTESIAN_POINT('Ctrl Pts',(-9.46235005017619,0.695941065062742,
1.82386101172742));
#11795=CARTESIAN_POINT('Ctrl Pts',(-9.57868819401829,0.535562491246337,
1.83181468230323));
#11796=CARTESIAN_POINT('Ctrl Pts',(-9.6558221235292,0.345556691784764,1.83976835287904));
#11797=CARTESIAN_POINT('Ctrl Pts',(-9.68019148863806,0.149449620287358,
1.84772202345485));
#11798=CARTESIAN_POINT('Ctrl Pts',(-9.68633448654835,0.10001520437127,1.84972697440487));
#11799=CARTESIAN_POINT('Ctrl Pts',(-9.68912463030123,0.0501930912280235,
1.85173192535489));
#11800=CARTESIAN_POINT('Ctrl Pts',(-9.68870505254289,0.000360304848219705,
1.85373687630491));
#11801=CARTESIAN_POINT('Origin',(-8.5,0.,1.8));
#11802=CARTESIAN_POINT('',(-9.68793925643297,0.00019677074638643,2.19626312369517));
#11803=CARTESIAN_POINT('',(-9.68748917149883,0.000243143348928272,2.15373687630491));
#11804=CARTESIAN_POINT('',(-9.688225,-1.45515594291686E-16,1.8));
#11805=CARTESIAN_POINT('Ctrl Pts',(-9.6874734085738,0.00051756617809895,
2.19626312369517));
#11806=CARTESIAN_POINT('Ctrl Pts',(-9.68805588513481,0.151871918451282,
2.19019552440188));
#11807=CARTESIAN_POINT('Ctrl Pts',(-9.66063518694746,0.302992792078646,
2.18412792510859));
#11808=CARTESIAN_POINT('Ctrl Pts',(-9.60441870150575,0.442514540719334,
2.1780603258153));
#11809=CARTESIAN_POINT('Ctrl Pts',(-9.45703671910369,0.808296779528733,
2.16215298466368));
#11810=CARTESIAN_POINT('Ctrl Pts',(-9.1117344267537,1.09435546738227,2.14624564351206));
#11811=CARTESIAN_POINT('Ctrl Pts',(-8.7250756969201,1.1688514604035,2.13033830236044));
#11812=CARTESIAN_POINT('Ctrl Pts',(-8.33841696708651,1.24334745342473,2.11443096120882));
#11813=CARTESIAN_POINT('Ctrl Pts',(-7.91040179976933,1.10628075161366,2.0985236200572));
#11814=CARTESIAN_POINT('Ctrl Pts',(-7.6383599938754,0.821043330033441,2.08261627890558));
#11815=CARTESIAN_POINT('Ctrl Pts',(-7.36631818798147,0.535805908453222,
2.06670893775396));
#11816=CARTESIAN_POINT('Ctrl Pts',(-7.25024974351079,0.102397767103854,
2.05080159660234));
#11817=CARTESIAN_POINT('Ctrl Pts',(-7.34335808136087,-0.28060568798053,
2.03489425545072));
#11818=CARTESIAN_POINT('Ctrl Pts',(-7.43646641921094,-0.663609143064914,
2.0189869142991));
#11819=CARTESIAN_POINT('Ctrl Pts',(-7.73875153938177,-0.996207911884313,
2.00307957314748));
#11820=CARTESIAN_POINT('Ctrl Pts',(-8.11087993218691,-1.12491486892692,
1.98717223199585));
#11821=CARTESIAN_POINT('Ctrl Pts',(-8.48300832499204,-1.25362182596952,
1.97126489084423));
#11822=CARTESIAN_POINT('Ctrl Pts',(-8.92497999043149,-1.17843697123532,
1.95535754969261));
#11823=CARTESIAN_POINT('Ctrl Pts',(-9.23549131184823,-0.935203778959572,
1.93945020854099));
#11824=CARTESIAN_POINT('Ctrl Pts',(-9.3907469725566,-0.813587182821698,
1.93149653796518));
#11825=CARTESIAN_POINT('Ctrl Pts',(-9.5131375472593,-0.649958502298435,
1.92354286738937));
#11826=CARTESIAN_POINT('Ctrl Pts',(-9.59128485561407,-0.46747485804336,
1.91558919681356));
#11827=CARTESIAN_POINT('Ctrl Pts',(-9.65457976584342,-0.319673403014159,
1.90914717244076));
#11828=CARTESIAN_POINT('Ctrl Pts',(-9.68885071316148,-0.159502929754193,
1.90270514806797));
#11829=CARTESIAN_POINT('Ctrl Pts',(-9.68946857590504,0.000315360110501401,
1.89626312369518));
#11830=CARTESIAN_POINT('Ctrl Pts',(-9.68870505254289,0.000360304848219705,
1.85373687630491));
#11831=CARTESIAN_POINT('Ctrl Pts',(-9.68579568774457,-0.345181735009932,
1.86763926650651));
#11832=CARTESIAN_POINT('Ctrl Pts',(-9.52856043097317,-0.691236952334183,
1.88154165670811));
#11833=CARTESIAN_POINT('Ctrl Pts',(-9.26471878006929,-0.912107988881616,
1.89544404690971));
#11834=CARTESIAN_POINT('Ctrl Pts',(-8.96282686867327,-1.16483222391764,
1.91135138806133));
#11835=CARTESIAN_POINT('Ctrl Pts',(-8.5213625732717,-1.25366146285155,1.92725872921295));
#11836=CARTESIAN_POINT('Ctrl Pts',(-8.1453201794112,-1.13646221921786,1.94316607036457));
#11837=CARTESIAN_POINT('Ctrl Pts',(-7.7692777855507,-1.01926297558418,1.95907341151619));
#11838=CARTESIAN_POINT('Ctrl Pts',(-7.45865729323126,-0.69603524938291,
1.97498075266782));
#11839=CARTESIAN_POINT('Ctrl Pts',(-7.35313075502305,-0.316068910845257,
1.99088809381944));
#11840=CARTESIAN_POINT('Ctrl Pts',(-7.30036748591894,-0.126085741576431,
1.99884176439525));
#11841=CARTESIAN_POINT('Ctrl Pts',(-7.29887770534264,0.0780820807764889,
2.00679543497106));
#11842=CARTESIAN_POINT('Ctrl Pts',(-7.34422871925985,0.271345030563532,
2.01474910554687));
#11843=CARTESIAN_POINT('Ctrl Pts',(-7.38957973317705,0.464607980350577,
2.02270277612268));
#11844=CARTESIAN_POINT('Ctrl Pts',(-7.48177154158776,0.646966057571745,
2.03065644669849));
#11845=CARTESIAN_POINT('Ctrl Pts',(-7.6136099013672,0.793641084515056,2.0386101172743));
#11846=CARTESIAN_POINT('Ctrl Pts',(-7.87728662092608,1.08699113840168,2.05451745842592));
#11847=CARTESIAN_POINT('Ctrl Pts',(-8.29954954595991,1.23760899117687,2.07042479957754));
#11848=CARTESIAN_POINT('Ctrl Pts',(-8.68834880695705,1.1753180915929,2.08633214072916));
#11849=CARTESIAN_POINT('Ctrl Pts',(-9.07714806795419,1.11302719200893,2.10223948188078));
#11850=CARTESIAN_POINT('Ctrl Pts',(-9.43248366491464,0.837827540065792,
2.1181468230324));
#11851=CARTESIAN_POINT('Ctrl Pts',(-9.59053795470158,0.476746315597217,
2.13405416418402));
#11852=CARTESIAN_POINT('Ctrl Pts',(-9.65572666339682,0.327820153650373,
2.14061506822432));
#11853=CARTESIAN_POINT('Ctrl Pts',(-9.6873556683552,0.164284598792956,2.14717597226461));
#11854=CARTESIAN_POINT('Ctrl Pts',(-9.68668762773837,0.000508001308789992,
2.1537368763049));
#11855=CARTESIAN_POINT('Origin',(-8.5,0.,1.8));
#11856=CARTESIAN_POINT('',(-9.688225,-8.88178419700125E-16,2.49626312369518));
#11857=CARTESIAN_POINT('',(-9.68781667187452,-0.000480474173583903,2.45373687630491));
#11858=CARTESIAN_POINT('',(-9.688225,-1.45515594291686E-16,1.8));
#11859=CARTESIAN_POINT('Ctrl Pts',(-9.688225,-8.88178419700125E-16,2.49626312369518));
#11860=CARTESIAN_POINT('Ctrl Pts',(-9.688225,0.298712821306089,2.48425993690586));
#11861=CARTESIAN_POINT('Ctrl Pts',(-9.57054245632587,0.595858078271521,
2.47225675011654));
#11862=CARTESIAN_POINT('Ctrl Pts',(-9.36601586214936,0.813569405232711,
2.46025356332722));
#11863=CARTESIAN_POINT('Ctrl Pts',(-9.16148926797285,1.0312807321939,2.4482503765379));
#11864=CARTESIAN_POINT('Ctrl Pts',(-8.87226522412848,1.16727314847135,2.43624718974859));
#11865=CARTESIAN_POINT('Ctrl Pts',(-8.57413435701453,1.1859100926019,2.42424400295927));
#11866=CARTESIAN_POINT('Ctrl Pts',(-8.27600348990057,1.20454703673245,2.41224081616995));
#11867=CARTESIAN_POINT('Ctrl Pts',(-7.97209482032098,1.10563290540111,2.40023762938063));
#11868=CARTESIAN_POINT('Ctrl Pts',(-7.74204705372066,0.915087963996611,
2.38823444259132));
#11869=CARTESIAN_POINT('Ctrl Pts',(-7.51199928712033,0.724543022592107,
2.376231255802));
#11870=CARTESIAN_POINT('Ctrl Pts',(-7.35822688079637,0.444367128061535,
2.36422806901268));
#11871=CARTESIAN_POINT('Ctrl Pts',(-7.32102560975818,0.147979855990369,
2.35222488222336));
#11872=CARTESIAN_POINT('Ctrl Pts',(-7.28382433871999,-0.148407416080797,
2.34022169543405));
#11873=CARTESIAN_POINT('Ctrl Pts',(-7.36358464744633,-0.457895344721877,
2.32821850864473));
#11874=CARTESIAN_POINT('Ctrl Pts',(-7.53940549437877,-0.699383189957625,
2.31621532185541));
#11875=CARTESIAN_POINT('Ctrl Pts',(-7.71522634131121,-0.940871035193373,
2.30421213506609));
#11876=CARTESIAN_POINT('Ctrl Pts',(-7.98526240565775,-1.11182427083078,
2.29220894827677));
#11877=CARTESIAN_POINT('Ctrl Pts',(-8.27875123560107,-1.16744491727745,
2.28020576148746));
#11878=CARTESIAN_POINT('Ctrl Pts',(-8.57224006554438,-1.22306556372412,
2.26820257469814));
#11879=CARTESIAN_POINT('Ctrl Pts',(-8.8861013605993,-1.16276985667028,2.25619938790882));
#11880=CARTESIAN_POINT('Ctrl Pts',(-9.13808834820084,-1.00235817476355,
2.2441962011195));
#11881=CARTESIAN_POINT('Ctrl Pts',(-9.39007533580238,-0.841946492856832,
2.23219301433019));
#11882=CARTESIAN_POINT('Ctrl Pts',(-9.5775432964213,-0.583102430603028,
2.22018982754087));
#11883=CARTESIAN_POINT('Ctrl Pts',(-9.65136659729188,-0.293655596346343,
2.20818664075155));
#11884=CARTESIAN_POINT('Ctrl Pts',(-9.67581103310541,-0.197813707972594,
2.20421213506609));
#11885=CARTESIAN_POINT('Ctrl Pts',(-9.688225,-0.0989100500924339,2.20023762938063));
#11886=CARTESIAN_POINT('Ctrl Pts',(-9.688225,2.99760216648792E-15,2.19626312369518));
#11887=CARTESIAN_POINT('Ctrl Pts',(-9.688225,-1.74171788103195E-12,2.15373687630491));
#11888=CARTESIAN_POINT('Ctrl Pts',(-9.68822499999956,-0.298712821307831,
2.16574006309422));
#11889=CARTESIAN_POINT('Ctrl Pts',(-9.57054245632499,-0.595858078273089,
2.17774324988354));
#11890=CARTESIAN_POINT('Ctrl Pts',(-9.36601586214817,-0.813569405233979,
2.18974643667286));
#11891=CARTESIAN_POINT('Ctrl Pts',(-9.16148926797134,-1.03128073219487,
2.20174962346218));
#11892=CARTESIAN_POINT('Ctrl Pts',(-8.87226522412677,-1.16727314847189,
2.2137528102515));
#11893=CARTESIAN_POINT('Ctrl Pts',(-8.57413435701279,-1.18591009260201,
2.22575599704081));
#11894=CARTESIAN_POINT('Ctrl Pts',(-8.27600348989881,-1.20454703673212,
2.23775918383013));
#11895=CARTESIAN_POINT('Ctrl Pts',(-7.97209482031937,-1.10563290540034,
2.24976237061945));
#11896=CARTESIAN_POINT('Ctrl Pts',(-7.74204705371932,-0.915087963995503,
2.26176555740877));
#11897=CARTESIAN_POINT('Ctrl Pts',(-7.51199928711927,-0.724543022590664,
2.27376874419808));
#11898=CARTESIAN_POINT('Ctrl Pts',(-7.35822688079572,-0.444367128059868,
2.2857719309874));
#11899=CARTESIAN_POINT('Ctrl Pts',(-7.32102560975796,-0.147979855988648,
2.29777511777672));
#11900=CARTESIAN_POINT('Ctrl Pts',(-7.28382433872021,0.148407416082571,
2.30977830456604));
#11901=CARTESIAN_POINT('Ctrl Pts',(-7.363584647447,0.457895344723534,2.32178149135536));
#11902=CARTESIAN_POINT('Ctrl Pts',(-7.53940549437979,0.699383189959025,
2.33378467814467));
#11903=CARTESIAN_POINT('Ctrl Pts',(-7.71522634131258,0.940871035194516,
2.34578786493399));
#11904=CARTESIAN_POINT('Ctrl Pts',(-7.98526240565937,1.11182427083153,2.35779105172331));
#11905=CARTESIAN_POINT('Ctrl Pts',(-8.27875123560277,1.16744491727777,2.36979423851263));
#11906=CARTESIAN_POINT('Ctrl Pts',(-8.57224006554616,1.22306556372401,2.38179742530194));
#11907=CARTESIAN_POINT('Ctrl Pts',(-8.88610136060099,1.16276985666972,2.39380061209126));
#11908=CARTESIAN_POINT('Ctrl Pts',(-9.1380883482023,1.00235817476263,2.40580379888058));
#11909=CARTESIAN_POINT('Ctrl Pts',(-9.39007533580361,0.841946492855538,
2.4178069856699));
#11910=CARTESIAN_POINT('Ctrl Pts',(-9.57754329642215,0.583102430601462,
2.42981017245921));
#11911=CARTESIAN_POINT('Ctrl Pts',(-9.6513665972923,0.293655596344671,2.44181335924853));
#11912=CARTESIAN_POINT('Ctrl Pts',(-9.6758110331057,0.197813707970885,2.44578786493399));
#11913=CARTESIAN_POINT('Ctrl Pts',(-9.68822500000014,0.0989100500907039,
2.44976237061945));
#11914=CARTESIAN_POINT('Ctrl Pts',(-9.688225,-1.73505654288419E-12,2.45373687630491));
#11915=CARTESIAN_POINT('Origin',(-8.5,0.,1.8));
#11916=CARTESIAN_POINT('',(-9.688225,-5.55111512312578E-16,2.79626312369518));
#11917=CARTESIAN_POINT('',(-9.68934581032131,-0.000146828966271381,2.75373687630491));
#11918=CARTESIAN_POINT('',(-9.688225,-1.45515594291686E-16,1.8));
#11919=CARTESIAN_POINT('Ctrl Pts',(-9.688225,3.66373598126302E-15,2.79626312369518));
#11920=CARTESIAN_POINT('Ctrl Pts',(-9.688225,0.298712821306094,2.78425993690586));
#11921=CARTESIAN_POINT('Ctrl Pts',(-9.57054245632586,0.595858078271526,
2.77225675011654));
#11922=CARTESIAN_POINT('Ctrl Pts',(-9.36601586214935,0.813569405232716,
2.76025356332722));
#11923=CARTESIAN_POINT('Ctrl Pts',(-9.16148926797284,1.03128073219391,2.7482503765379));
#11924=CARTESIAN_POINT('Ctrl Pts',(-8.87226522412847,1.16727314847135,2.73624718974859));
#11925=CARTESIAN_POINT('Ctrl Pts',(-8.57413435701452,1.1859100926019,2.72424400295927));
#11926=CARTESIAN_POINT('Ctrl Pts',(-8.27600348990056,1.20454703673245,2.71224081616995));
#11927=CARTESIAN_POINT('Ctrl Pts',(-7.97209482032097,1.10563290540111,2.70023762938063));
#11928=CARTESIAN_POINT('Ctrl Pts',(-7.74204705372065,0.915087963996604,
2.68823444259132));
#11929=CARTESIAN_POINT('Ctrl Pts',(-7.51199928712032,0.724543022592098,
2.676231255802));
#11930=CARTESIAN_POINT('Ctrl Pts',(-7.35822688079636,0.444367128061523,
2.66422806901268));
#11931=CARTESIAN_POINT('Ctrl Pts',(-7.32102560975818,0.147979855990356,
2.65222488222336));
#11932=CARTESIAN_POINT('Ctrl Pts',(-7.28382433871999,-0.148407416080811,
2.64022169543404));
#11933=CARTESIAN_POINT('Ctrl Pts',(-7.36358464744634,-0.457895344721891,
2.62821850864473));
#11934=CARTESIAN_POINT('Ctrl Pts',(-7.53940549437878,-0.699383189957637,
2.61621532185541));
#11935=CARTESIAN_POINT('Ctrl Pts',(-7.71522634131122,-0.940871035193383,
2.60421213506609));
#11936=CARTESIAN_POINT('Ctrl Pts',(-7.98526240565776,-1.11182427083079,
2.59220894827677));
#11937=CARTESIAN_POINT('Ctrl Pts',(-8.27875123560108,-1.16744491727745,
2.58020576148746));
#11938=CARTESIAN_POINT('Ctrl Pts',(-8.5722400655444,-1.22306556372411,2.56820257469814));
#11939=CARTESIAN_POINT('Ctrl Pts',(-8.88610136059931,-1.16276985667027,
2.55619938790882));
#11940=CARTESIAN_POINT('Ctrl Pts',(-9.13808834820086,-1.00235817476354,
2.5441962011195));
#11941=CARTESIAN_POINT('Ctrl Pts',(-9.3900753358024,-0.841946492856817,
2.53219301433018));
#11942=CARTESIAN_POINT('Ctrl Pts',(-9.57754329642131,-0.583102430603009,
2.52018982754087));
#11943=CARTESIAN_POINT('Ctrl Pts',(-9.65136659729188,-0.293655596346323,
2.50818664075155));
#11944=CARTESIAN_POINT('Ctrl Pts',(-9.67581103310541,-0.197813707972581,
2.50421213506609));
#11945=CARTESIAN_POINT('Ctrl Pts',(-9.688225,-0.0989100500924293,2.50023762938063));
#11946=CARTESIAN_POINT('Ctrl Pts',(-9.688225,-8.88178419700125E-16,2.49626312369518));
#11947=CARTESIAN_POINT('Ctrl Pts',(-9.68737088905248,-0.00100502077275876,
2.45373687630491));
#11948=CARTESIAN_POINT('Ctrl Pts',(-9.68829445628317,-0.120370390803603,
2.45852736032596));
#11949=CARTESIAN_POINT('Ctrl Pts',(-9.67170875826749,-0.239475692471852,
2.46331784434701));
#11950=CARTESIAN_POINT('Ctrl Pts',(-9.63652762380349,-0.352808501661884,
2.46810832836806));
#11951=CARTESIAN_POINT('Ctrl Pts',(-9.51970470871583,-0.729142845234637,
2.48401566951968));
#11952=CARTESIAN_POINT('Ctrl Pts',(-9.19783981952358,-1.04182698858073,
2.4999230106713));
#11953=CARTESIAN_POINT('Ctrl Pts',(-8.8180025015363,-1.14702407757865,2.51583035182292));
#11954=CARTESIAN_POINT('Ctrl Pts',(-8.43816518354902,-1.25222116657657,
2.53173769297454));
#11955=CARTESIAN_POINT('Ctrl Pts',(-8.00035543676671,-1.14993120122632,
2.54764503412616));
#11956=CARTESIAN_POINT('Ctrl Pts',(-7.70675772214978,-0.887471152741141,
2.56355237527778));
#11957=CARTESIAN_POINT('Ctrl Pts',(-7.41316000753286,-0.625011104255964,
2.5794597164294));
#11958=CARTESIAN_POINT('Ctrl Pts',(-7.26377432508131,-0.202380972635861,
2.59536705758103));
#11959=CARTESIAN_POINT('Ctrl Pts',(-7.32507248791809,0.187188402540279,
2.61127439873265));
#11960=CARTESIAN_POINT('Ctrl Pts',(-7.35572156933647,0.381973090128349,
2.61922806930846));
#11961=CARTESIAN_POINT('Ctrl Pts',(-7.43904161207694,0.568492588605429,
2.62718173988427));
#11962=CARTESIAN_POINT('Ctrl Pts',(-7.56040023003843,0.725635480344461,
2.63513541046008));
#11963=CARTESIAN_POINT('Ctrl Pts',(-7.68175884799992,0.882778372083494,
2.64308908103589));
#11964=CARTESIAN_POINT('Ctrl Pts',(-7.84115604118242,1.01054465708448,2.6510427516117));
#11965=CARTESIAN_POINT('Ctrl Pts',(-8.02186533941589,1.08944057941184,2.65899642218751));
#11966=CARTESIAN_POINT('Ctrl Pts',(-8.38328393588282,1.24723242406657,2.67490376333913));
#11967=CARTESIAN_POINT('Ctrl Pts',(-8.8299509525536,1.2095428180268,2.69081110449075));
#11968=CARTESIAN_POINT('Ctrl Pts',(-9.15810856599484,0.991832674325304,
2.70671844564237));
#11969=CARTESIAN_POINT('Ctrl Pts',(-9.48142796607357,0.777332354450122,
2.72239125586322));
#11970=CARTESIAN_POINT('Ctrl Pts',(-9.68970670457596,0.38808065463741,2.73806406608406));
#11971=CARTESIAN_POINT('Ctrl Pts',(-9.69027298352254,-0.000268290982180393,
2.7537368763049));
#11972=CARTESIAN_POINT('Origin',(-8.5,0.,1.8));
#11973=CARTESIAN_POINT('',(-9.688225,-3.33066907387547E-16,3.09626312369518));
#11974=CARTESIAN_POINT('',(-9.688225,-1.73872027886546E-12,3.05373687630491));
#11975=CARTESIAN_POINT('',(-9.688225,-1.45515594291686E-16,1.8));
#11976=CARTESIAN_POINT('Ctrl Pts',(-9.688225,-4.55191440096314E-15,3.09626312369518));
#11977=CARTESIAN_POINT('Ctrl Pts',(-9.688225,0.298712821306082,3.08425993690586));
#11978=CARTESIAN_POINT('Ctrl Pts',(-9.57054245632587,0.595858078271511,
3.07225675011654));
#11979=CARTESIAN_POINT('Ctrl Pts',(-9.36601586214937,0.813569405232701,
3.06025356332722));
#11980=CARTESIAN_POINT('Ctrl Pts',(-9.16148926797286,1.03128073219389,3.04825037653791));
#11981=CARTESIAN_POINT('Ctrl Pts',(-8.8722652241285,1.16727314847134,3.03624718974859));
#11982=CARTESIAN_POINT('Ctrl Pts',(-8.57413435701455,1.1859100926019,3.02424400295927));
#11983=CARTESIAN_POINT('Ctrl Pts',(-8.2760034899006,1.20454703673245,3.01224081616995));
#11984=CARTESIAN_POINT('Ctrl Pts',(-7.97209482032101,1.10563290540113,3.00023762938064));
#11985=CARTESIAN_POINT('Ctrl Pts',(-7.74204705372068,0.915087963996633,
2.98823444259132));
#11986=CARTESIAN_POINT('Ctrl Pts',(-7.51199928712035,0.724543022592139,
2.976231255802));
#11987=CARTESIAN_POINT('Ctrl Pts',(-7.35822688079639,0.444367128061575,
2.96422806901268));
#11988=CARTESIAN_POINT('Ctrl Pts',(-7.32102560975819,0.147979855990414,
2.95222488222336));
#11989=CARTESIAN_POINT('Ctrl Pts',(-7.28382433871999,-0.148407416080746,
2.94022169543405));
#11990=CARTESIAN_POINT('Ctrl Pts',(-7.36358464744631,-0.457895344721826,
2.92821850864473));
#11991=CARTESIAN_POINT('Ctrl Pts',(-7.53940549437874,-0.69938318995758,
2.91621532185541));
#11992=CARTESIAN_POINT('Ctrl Pts',(-7.71522634131116,-0.940871035193333,
2.90421213506609));
#11993=CARTESIAN_POINT('Ctrl Pts',(-7.98526240565769,-1.11182427083075,
2.89220894827678));
#11994=CARTESIAN_POINT('Ctrl Pts',(-8.278751235601,-1.16744491727744,2.88020576148746));
#11995=CARTESIAN_POINT('Ctrl Pts',(-8.57224006554431,-1.22306556372412,
2.86820257469814));
#11996=CARTESIAN_POINT('Ctrl Pts',(-8.88610136059922,-1.1627698566703,2.85619938790882));
#11997=CARTESIAN_POINT('Ctrl Pts',(-9.13808834820077,-1.0023581747636,2.84419620111951));
#11998=CARTESIAN_POINT('Ctrl Pts',(-9.39007533580233,-0.841946492856892,
2.83219301433019));
#11999=CARTESIAN_POINT('Ctrl Pts',(-9.57754329642126,-0.583102430603105,
2.82018982754087));
#12000=CARTESIAN_POINT('Ctrl Pts',(-9.65136659729185,-0.293655596346429,
2.80818664075155));
#12001=CARTESIAN_POINT('Ctrl Pts',(-9.67581103310541,-0.197813707972653,
2.80421213506609));
#12002=CARTESIAN_POINT('Ctrl Pts',(-9.688225,-0.0989100500924628,2.80023762938063));
#12003=CARTESIAN_POINT('Ctrl Pts',(-9.688225,3.66373598126302E-15,2.79626312369518));
#12004=CARTESIAN_POINT('Ctrl Pts',(-9.688225,-1.73899783462161E-12,2.75373687630491));
#12005=CARTESIAN_POINT('Ctrl Pts',(-9.68822499999956,-0.298712821307831,
2.76574006309423));
#12006=CARTESIAN_POINT('Ctrl Pts',(-9.57054245632499,-0.595858078273093,
2.77774324988354));
#12007=CARTESIAN_POINT('Ctrl Pts',(-9.36601586214816,-0.813569405233984,
2.78974643667286));
#12008=CARTESIAN_POINT('Ctrl Pts',(-9.16148926797133,-1.03128073219487,
2.80174962346218));
#12009=CARTESIAN_POINT('Ctrl Pts',(-8.87226522412676,-1.1672731484719,2.8137528102515));
#12010=CARTESIAN_POINT('Ctrl Pts',(-8.57413435701278,-1.18591009260201,
2.82575599704081));
#12011=CARTESIAN_POINT('Ctrl Pts',(-8.27600348989879,-1.20454703673212,
2.83775918383013));
#12012=CARTESIAN_POINT('Ctrl Pts',(-7.97209482031935,-1.10563290540033,
2.84976237061945));
#12013=CARTESIAN_POINT('Ctrl Pts',(-7.7420470537193,-0.915087963995489,
2.86176555740877));
#12014=CARTESIAN_POINT('Ctrl Pts',(-7.51199928711925,-0.724543022590643,
2.87376874419809));
#12015=CARTESIAN_POINT('Ctrl Pts',(-7.35822688079571,-0.444367128059841,
2.8857719309874));
#12016=CARTESIAN_POINT('Ctrl Pts',(-7.32102560975796,-0.147979855988618,
2.89777511777672));
#12017=CARTESIAN_POINT('Ctrl Pts',(-7.28382433872021,0.148407416082605,
2.90977830456604));
#12018=CARTESIAN_POINT('Ctrl Pts',(-7.36358464744701,0.45789534472357,2.92178149135536));
#12019=CARTESIAN_POINT('Ctrl Pts',(-7.53940549437981,0.699383189959057,
2.93378467814467));
#12020=CARTESIAN_POINT('Ctrl Pts',(-7.71522634131261,0.940871035194545,
2.94578786493399));
#12021=CARTESIAN_POINT('Ctrl Pts',(-7.98526240565941,1.11182427083155,2.95779105172331));
#12022=CARTESIAN_POINT('Ctrl Pts',(-8.27875123560281,1.16744491727778,2.96979423851263));
#12023=CARTESIAN_POINT('Ctrl Pts',(-8.57224006554622,1.22306556372401,2.98179742530195));
#12024=CARTESIAN_POINT('Ctrl Pts',(-8.88610136060104,1.1627698566697,2.99380061209126));
#12025=CARTESIAN_POINT('Ctrl Pts',(-9.13808834820234,1.0023581747626,3.00580379888058));
#12026=CARTESIAN_POINT('Ctrl Pts',(-9.39007533580365,0.841946492855494,
3.0178069856699));
#12027=CARTESIAN_POINT('Ctrl Pts',(-9.57754329642218,0.583102430601406,
3.02981017245922));
#12028=CARTESIAN_POINT('Ctrl Pts',(-9.65136659729232,0.293655596344608,
3.04181335924854));
#12029=CARTESIAN_POINT('Ctrl Pts',(-9.67581103310571,0.197813707970839,
3.04578786493399));
#12030=CARTESIAN_POINT('Ctrl Pts',(-9.68822500000014,0.098910050090677,
3.04976237061945));
#12031=CARTESIAN_POINT('Ctrl Pts',(-9.688225,-1.74293912635903E-12,3.05373687630491));
#12032=CARTESIAN_POINT('Origin',(-8.5,0.,1.8));
#12033=CARTESIAN_POINT('',(-9.68741751198286,-6.04159293495165E-5,3.39626312369518));
#12034=CARTESIAN_POINT('',(-9.688225,-1.7384427231093E-12,3.35373687630491));
#12035=CARTESIAN_POINT('',(-9.688225,-1.45515594291686E-16,1.8));
#12036=CARTESIAN_POINT('Ctrl Pts',(-9.688225,-4.32986979603811E-15,3.39626312369518));
#12037=CARTESIAN_POINT('Ctrl Pts',(-9.688225,0.298712821306089,3.38425993690586));
#12038=CARTESIAN_POINT('Ctrl Pts',(-9.57054245632586,0.595858078271525,
3.37225675011654));
#12039=CARTESIAN_POINT('Ctrl Pts',(-9.36601586214935,0.813569405232716,
3.36025356332722));
#12040=CARTESIAN_POINT('Ctrl Pts',(-9.16148926797284,1.03128073219391,3.3482503765379));
#12041=CARTESIAN_POINT('Ctrl Pts',(-8.87226522412847,1.16727314847135,3.33624718974859));
#12042=CARTESIAN_POINT('Ctrl Pts',(-8.57413435701451,1.1859100926019,3.32424400295927));
#12043=CARTESIAN_POINT('Ctrl Pts',(-8.27600348990055,1.20454703673244,3.31224081616995));
#12044=CARTESIAN_POINT('Ctrl Pts',(-7.97209482032096,1.1056329054011,3.30023762938063));
#12045=CARTESIAN_POINT('Ctrl Pts',(-7.74204705372063,0.915087963996593,
3.28823444259131));
#12046=CARTESIAN_POINT('Ctrl Pts',(-7.51199928712031,0.724543022592082,
3.276231255802));
#12047=CARTESIAN_POINT('Ctrl Pts',(-7.35822688079636,0.444367128061501,
3.26422806901268));
#12048=CARTESIAN_POINT('Ctrl Pts',(-7.32102560975818,0.14797985599033,3.25222488222336));
#12049=CARTESIAN_POINT('Ctrl Pts',(-7.28382433872,-0.14840741608084,3.24022169543404));
#12050=CARTESIAN_POINT('Ctrl Pts',(-7.36358464744635,-0.457895344721922,
3.22821850864473));
#12051=CARTESIAN_POINT('Ctrl Pts',(-7.5394054943788,-0.699383189957665,
3.21621532185541));
#12052=CARTESIAN_POINT('Ctrl Pts',(-7.71522634131125,-0.940871035193408,
3.20421213506609));
#12053=CARTESIAN_POINT('Ctrl Pts',(-7.9852624056578,-1.1118242708308,3.19220894827677));
#12054=CARTESIAN_POINT('Ctrl Pts',(-8.27875123560113,-1.16744491727746,
3.18020576148745));
#12055=CARTESIAN_POINT('Ctrl Pts',(-8.57224006554445,-1.22306556372411,
3.16820257469814));
#12056=CARTESIAN_POINT('Ctrl Pts',(-8.88610136059936,-1.16276985667026,
3.15619938790882));
#12057=CARTESIAN_POINT('Ctrl Pts',(-9.1380883482009,-1.00235817476352,3.1441962011195));
#12058=CARTESIAN_POINT('Ctrl Pts',(-9.39007533580244,-0.841946492856777,
3.13219301433018));
#12059=CARTESIAN_POINT('Ctrl Pts',(-9.57754329642134,-0.583102430602958,
3.12018982754086));
#12060=CARTESIAN_POINT('Ctrl Pts',(-9.6513665972919,-0.293655596346265,
3.10818664075155));
#12061=CARTESIAN_POINT('Ctrl Pts',(-9.67581103310542,-0.197813707972543,
3.10421213506609));
#12062=CARTESIAN_POINT('Ctrl Pts',(-9.688225,-0.0989100500924119,3.10023762938063));
#12063=CARTESIAN_POINT('Ctrl Pts',(-9.688225,-4.55191440096314E-15,3.09626312369518));
#12064=CARTESIAN_POINT('Ctrl Pts',(-9.688225,-1.74293912635903E-12,3.05373687630491));
#12065=CARTESIAN_POINT('Ctrl Pts',(-9.68822499999956,-0.298712821307838,
3.06574006309423));
#12066=CARTESIAN_POINT('Ctrl Pts',(-9.57054245632499,-0.595858078273102,
3.07774324988354));
#12067=CARTESIAN_POINT('Ctrl Pts',(-9.36601586214815,-0.813569405233993,
3.08974643667286));
#12068=CARTESIAN_POINT('Ctrl Pts',(-9.16148926797132,-1.03128073219488,
3.10174962346218));
#12069=CARTESIAN_POINT('Ctrl Pts',(-8.87226522412674,-1.1672731484719,3.1137528102515));
#12070=CARTESIAN_POINT('Ctrl Pts',(-8.57413435701276,-1.18591009260201,
3.12575599704082));
#12071=CARTESIAN_POINT('Ctrl Pts',(-8.27600348989877,-1.20454703673211,
3.13775918383013));
#12072=CARTESIAN_POINT('Ctrl Pts',(-7.97209482031932,-1.10563290540032,
3.14976237061945));
#12073=CARTESIAN_POINT('Ctrl Pts',(-7.74204705371928,-0.91508796399547,
3.16176555740877));
#12074=CARTESIAN_POINT('Ctrl Pts',(-7.51199928711924,-0.724543022590617,
3.17376874419809));
#12075=CARTESIAN_POINT('Ctrl Pts',(-7.3582268807957,-0.444367128059807,
3.1857719309874));
#12076=CARTESIAN_POINT('Ctrl Pts',(-7.32102560975796,-0.14797985598858,
3.19777511777672));
#12077=CARTESIAN_POINT('Ctrl Pts',(-7.28382433872022,0.148407416082647,
3.20977830456604));
#12078=CARTESIAN_POINT('Ctrl Pts',(-7.36358464744703,0.457895344723612,
3.22178149135536));
#12079=CARTESIAN_POINT('Ctrl Pts',(-7.53940549437984,0.699383189959094,
3.23378467814468));
#12080=CARTESIAN_POINT('Ctrl Pts',(-7.71522634131265,0.940871035194577,
3.24578786493399));
#12081=CARTESIAN_POINT('Ctrl Pts',(-7.98526240565946,1.11182427083157,3.25779105172331));
#12082=CARTESIAN_POINT('Ctrl Pts',(-8.27875123560287,1.16744491727779,3.26979423851263));
#12083=CARTESIAN_POINT('Ctrl Pts',(-8.57224006554628,1.223065563724,3.28179742530195));
#12084=CARTESIAN_POINT('Ctrl Pts',(-8.8861013606011,1.16276985666968,3.29380061209127));
#12085=CARTESIAN_POINT('Ctrl Pts',(-9.1380883482024,1.00235817476256,3.30580379888058));
#12086=CARTESIAN_POINT('Ctrl Pts',(-9.3900753358037,0.841946492855445,3.3178069856699));
#12087=CARTESIAN_POINT('Ctrl Pts',(-9.57754329642222,0.583102430601342,
3.32981017245922));
#12088=CARTESIAN_POINT('Ctrl Pts',(-9.65136659729234,0.293655596344535,
3.34181335924854));
#12089=CARTESIAN_POINT('Ctrl Pts',(-9.67581103310571,0.19781370797079,3.34578786493399));
#12090=CARTESIAN_POINT('Ctrl Pts',(-9.68822500000014,0.0989100500906548,
3.34976237061945));
#12091=CARTESIAN_POINT('Ctrl Pts',(-9.688225,-1.7384427231093E-12,3.35373687630491));
#12092=CARTESIAN_POINT('Origin',(-8.5,0.,1.8));
#12093=CARTESIAN_POINT('',(-9.68847469849902,-0.000576838186012704,3.69626312369518));
#12094=CARTESIAN_POINT('',(-9.688225,-1.74654735118907E-12,3.65373687630491));
#12095=CARTESIAN_POINT('',(-9.688225,-1.45515594291686E-16,1.8));
#12096=CARTESIAN_POINT('Ctrl Pts',(-9.68866306042472,-0.00101198037532446,
3.69626312369518));
#12097=CARTESIAN_POINT('Ctrl Pts',(-9.68582589943624,0.320508041344992,
3.68332310010213));
#12098=CARTESIAN_POINT('Ctrl Pts',(-9.55110894064229,0.644172586075907,
3.67038307650908));
#12099=CARTESIAN_POINT('Ctrl Pts',(-9.31819110540849,0.864496431520476,
3.65744305291603));
#12100=CARTESIAN_POINT('Ctrl Pts',(-9.03186214791326,1.13534343176913,3.64153571176441));
#12101=CARTESIAN_POINT('Ctrl Pts',(-8.59713096356923,1.2500208492789,3.62562837061279));
#12102=CARTESIAN_POINT('Ctrl Pts',(-8.21479992629871,1.1556382784724,3.60972102946117));
#12103=CARTESIAN_POINT('Ctrl Pts',(-7.8324688890282,1.06125570766591,3.59381368830955));
#12104=CARTESIAN_POINT('Ctrl Pts',(-7.50253799883119,0.757813148543147,
3.57790634715793));
#12105=CARTESIAN_POINT('Ctrl Pts',(-7.37423722665768,0.384904745016853,
3.56199900600631));
#12106=CARTESIAN_POINT('Ctrl Pts',(-7.31008684057093,0.198450543253708,
3.5540453354305));
#12107=CARTESIAN_POINT('Ctrl Pts',(-7.29634398399005,-0.0053701196103213,
3.54609166485469));
#12108=CARTESIAN_POINT('Ctrl Pts',(-7.32996872509888,-0.201051408397636,
3.53813799427888));
#12109=CARTESIAN_POINT('Ctrl Pts',(-7.36359346620772,-0.396732697184954,
3.53018432370307));
#12110=CARTESIAN_POINT('Ctrl Pts',(-7.44458580500627,-0.584274611895558,
3.52223065312726));
#12111=CARTESIAN_POINT('Ctrl Pts',(-7.56729714878503,-0.738619574554616,
3.51427698255145));
#12112=CARTESIAN_POINT('Ctrl Pts',(-7.81271983634256,-1.04730949987273,
3.49836964139982));
#12113=CARTESIAN_POINT('Ctrl Pts',(-8.22501854382095,-1.22321161698467,
3.48246230024821));
#12114=CARTESIAN_POINT('Ctrl Pts',(-8.61692498285394,-1.18455369700755,
3.46655495909659));
#12115=CARTESIAN_POINT('Ctrl Pts',(-9.00883142188693,-1.14589577703044,
3.45064761794497));
#12116=CARTESIAN_POINT('Ctrl Pts',(-9.38034559247452,-0.892677819964278,
3.43474027679334));
#12117=CARTESIAN_POINT('Ctrl Pts',(-9.55983865925423,-0.541786656749807,
3.41883293564172));
#12118=CARTESIAN_POINT('Ctrl Pts',(-9.64472870518362,-0.375835026996589,
3.41130966499287));
#12119=CARTESIAN_POINT('Ctrl Pts',(-9.6866683579978,-0.188036305867981,
3.40378639434402));
#12120=CARTESIAN_POINT('Ctrl Pts',(-9.68633860011409,-0.000141139682333869,
3.39626312369518));
#12121=CARTESIAN_POINT('Ctrl Pts',(-9.688225,-1.7384427231093E-12,3.35373687630491));
#12122=CARTESIAN_POINT('Ctrl Pts',(-9.68822499999956,-0.298712821307826,
3.36574006309423));
#12123=CARTESIAN_POINT('Ctrl Pts',(-9.57054245632499,-0.595858078273084,
3.37774324988354));
#12124=CARTESIAN_POINT('Ctrl Pts',(-9.36601586214817,-0.813569405233974,
3.38974643667286));
#12125=CARTESIAN_POINT('Ctrl Pts',(-9.16148926797135,-1.03128073219486,
3.40174962346218));
#12126=CARTESIAN_POINT('Ctrl Pts',(-8.87226522412678,-1.16727314847189,
3.4137528102515));
#12127=CARTESIAN_POINT('Ctrl Pts',(-8.5741343570128,-1.18591009260201,3.42575599704081));
#12128=CARTESIAN_POINT('Ctrl Pts',(-8.27600348989882,-1.20454703673212,
3.43775918383013));
#12129=CARTESIAN_POINT('Ctrl Pts',(-7.97209482031938,-1.10563290540035,
3.44976237061945));
#12130=CARTESIAN_POINT('Ctrl Pts',(-7.74204705371933,-0.915087963995513,
3.46176555740877));
#12131=CARTESIAN_POINT('Ctrl Pts',(-7.51199928711928,-0.724543022590678,
3.47376874419808));
#12132=CARTESIAN_POINT('Ctrl Pts',(-7.35822688079573,-0.444367128059886,
3.4857719309874));
#12133=CARTESIAN_POINT('Ctrl Pts',(-7.32102560975797,-0.147979855988668,
3.49777511777672));
#12134=CARTESIAN_POINT('Ctrl Pts',(-7.28382433872021,0.148407416082549,
3.50977830456604));
#12135=CARTESIAN_POINT('Ctrl Pts',(-7.36358464744699,0.457895344723512,
3.52178149135535));
#12136=CARTESIAN_POINT('Ctrl Pts',(-7.53940549437977,0.699383189959006,
3.53378467814467));
#12137=CARTESIAN_POINT('Ctrl Pts',(-7.71522634131256,0.940871035194499,
3.54578786493399));
#12138=CARTESIAN_POINT('Ctrl Pts',(-7.98526240565934,1.11182427083152,3.55779105172331));
#12139=CARTESIAN_POINT('Ctrl Pts',(-8.27875123560274,1.16744491727776,3.56979423851263));
#12140=CARTESIAN_POINT('Ctrl Pts',(-8.57224006554613,1.22306556372401,3.58179742530194));
#12141=CARTESIAN_POINT('Ctrl Pts',(-8.88610136060096,1.16276985666972,3.59380061209126));
#12142=CARTESIAN_POINT('Ctrl Pts',(-9.13808834820227,1.00235817476264,3.60580379888058));
#12143=CARTESIAN_POINT('Ctrl Pts',(-9.39007533580358,0.841946492855563,
3.6178069856699));
#12144=CARTESIAN_POINT('Ctrl Pts',(-9.57754329642213,0.583102430601495,
3.62981017245921));
#12145=CARTESIAN_POINT('Ctrl Pts',(-9.65136659729229,0.293655596344707,
3.64181335924853));
#12146=CARTESIAN_POINT('Ctrl Pts',(-9.6758110331057,0.197813707970906,3.64578786493399));
#12147=CARTESIAN_POINT('Ctrl Pts',(-9.68822500000014,0.0989100500907086,
3.64976237061945));
#12148=CARTESIAN_POINT('Ctrl Pts',(-9.688225,-1.74654735118907E-12,3.65373687630491));
#12149=CARTESIAN_POINT('Origin',(-8.5,0.,1.8));
#12150=CARTESIAN_POINT('',(-9.688225,-2.04281036531029E-14,3.99626312369518));
#12151=CARTESIAN_POINT('',(-9.688225,-1.75470749042006E-12,3.95373687630491));
#12152=CARTESIAN_POINT('',(-9.688225,-1.45515594291686E-16,1.8));
#12153=CARTESIAN_POINT('Ctrl Pts',(-9.688225,-3.66373598126302E-15,3.99626312369518));
#12154=CARTESIAN_POINT('Ctrl Pts',(-9.688225,0.29871282130609,3.98425993690586));
#12155=CARTESIAN_POINT('Ctrl Pts',(-9.57054245632586,0.595858078271525,
3.97225675011654));
#12156=CARTESIAN_POINT('Ctrl Pts',(-9.36601586214935,0.813569405232717,
3.96025356332722));
#12157=CARTESIAN_POINT('Ctrl Pts',(-9.16148926797284,1.03128073219391,3.94825037653791));
#12158=CARTESIAN_POINT('Ctrl Pts',(-8.87226522412847,1.16727314847135,3.93624718974859));
#12159=CARTESIAN_POINT('Ctrl Pts',(-8.57413435701451,1.1859100926019,3.92424400295927));
#12160=CARTESIAN_POINT('Ctrl Pts',(-8.27600348990055,1.20454703673244,3.91224081616995));
#12161=CARTESIAN_POINT('Ctrl Pts',(-7.97209482032096,1.1056329054011,3.90023762938063));
#12162=CARTESIAN_POINT('Ctrl Pts',(-7.74204705372063,0.915087963996592,
3.88823444259132));
#12163=CARTESIAN_POINT('Ctrl Pts',(-7.51199928712031,0.724543022592081,
3.876231255802));
#12164=CARTESIAN_POINT('Ctrl Pts',(-7.35822688079636,0.4443671280615,3.86422806901268));
#12165=CARTESIAN_POINT('Ctrl Pts',(-7.32102560975818,0.14797985599033,3.85222488222336));
#12166=CARTESIAN_POINT('Ctrl Pts',(-7.28382433872,-0.148407416080841,3.84022169543404));
#12167=CARTESIAN_POINT('Ctrl Pts',(-7.36358464744635,-0.457895344721922,
3.82821850864473));
#12168=CARTESIAN_POINT('Ctrl Pts',(-7.5394054943788,-0.699383189957666,
3.81621532185541));
#12169=CARTESIAN_POINT('Ctrl Pts',(-7.71522634131125,-0.940871035193409,
3.80421213506609));
#12170=CARTESIAN_POINT('Ctrl Pts',(-7.9852624056578,-1.11182427083081,3.79220894827677));
#12171=CARTESIAN_POINT('Ctrl Pts',(-8.27875123560113,-1.16744491727746,
3.78020576148745));
#12172=CARTESIAN_POINT('Ctrl Pts',(-8.57224006554445,-1.22306556372411,
3.76820257469814));
#12173=CARTESIAN_POINT('Ctrl Pts',(-8.88610136059936,-1.16276985667026,
3.75619938790882));
#12174=CARTESIAN_POINT('Ctrl Pts',(-9.1380883482009,-1.00235817476352,3.7441962011195));
#12175=CARTESIAN_POINT('Ctrl Pts',(-9.39007533580244,-0.841946492856777,
3.73219301433018));
#12176=CARTESIAN_POINT('Ctrl Pts',(-9.57754329642134,-0.583102430602957,
3.72018982754087));
#12177=CARTESIAN_POINT('Ctrl Pts',(-9.6513665972919,-0.293655596346264,
3.70818664075155));
#12178=CARTESIAN_POINT('Ctrl Pts',(-9.67581103310542,-0.197813707972545,
3.70421213506609));
#12179=CARTESIAN_POINT('Ctrl Pts',(-9.688225,-0.0989100500924169,3.70023762938063));
#12180=CARTESIAN_POINT('Ctrl Pts',(-9.688225,-1.24344978758018E-14,3.69626312369518));
#12181=CARTESIAN_POINT('Ctrl Pts',(-9.688225,-1.74654735118907E-12,3.65373687630491));
#12182=CARTESIAN_POINT('Ctrl Pts',(-9.68822499999956,-0.298712821307834,
3.66574006309423));
#12183=CARTESIAN_POINT('Ctrl Pts',(-9.57054245632499,-0.595858078273091,
3.67774324988354));
#12184=CARTESIAN_POINT('Ctrl Pts',(-9.36601586214816,-0.81356940523398,
3.68974643667286));
#12185=CARTESIAN_POINT('Ctrl Pts',(-9.16148926797134,-1.03128073219487,
3.70174962346218));
#12186=CARTESIAN_POINT('Ctrl Pts',(-8.87226522412678,-1.16727314847189,
3.7137528102515));
#12187=CARTESIAN_POINT('Ctrl Pts',(-8.5741343570128,-1.18591009260201,3.72575599704081));
#12188=CARTESIAN_POINT('Ctrl Pts',(-8.27600348989881,-1.20454703673212,
3.73775918383013));
#12189=CARTESIAN_POINT('Ctrl Pts',(-7.97209482031937,-1.10563290540034,
3.74976237061945));
#12190=CARTESIAN_POINT('Ctrl Pts',(-7.74204705371933,-0.915087963995508,
3.76176555740877));
#12191=CARTESIAN_POINT('Ctrl Pts',(-7.51199928711928,-0.724543022590671,
3.77376874419808));
#12192=CARTESIAN_POINT('Ctrl Pts',(-7.35822688079573,-0.444367128059878,
3.7857719309874));
#12193=CARTESIAN_POINT('Ctrl Pts',(-7.32102560975797,-0.14797985598866,
3.79777511777672));
#12194=CARTESIAN_POINT('Ctrl Pts',(-7.28382433872021,0.148407416082557,
3.80977830456604));
#12195=CARTESIAN_POINT('Ctrl Pts',(-7.363584647447,0.45789534472352,3.82178149135535));
#12196=CARTESIAN_POINT('Ctrl Pts',(-7.53940549437978,0.699383189959012,
3.83378467814467));
#12197=CARTESIAN_POINT('Ctrl Pts',(-7.71522634131256,0.940871035194504,
3.84578786493399));
#12198=CARTESIAN_POINT('Ctrl Pts',(-7.98526240565935,1.11182427083152,3.85779105172331));
#12199=CARTESIAN_POINT('Ctrl Pts',(-8.27875123560275,1.16744491727777,3.86979423851263));
#12200=CARTESIAN_POINT('Ctrl Pts',(-8.57224006554614,1.22306556372401,3.88179742530194));
#12201=CARTESIAN_POINT('Ctrl Pts',(-8.88610136060096,1.16276985666972,3.89380061209126));
#12202=CARTESIAN_POINT('Ctrl Pts',(-9.13808834820228,1.00235817476264,3.90580379888058));
#12203=CARTESIAN_POINT('Ctrl Pts',(-9.39007533580359,0.841946492855557,
3.9178069856699));
#12204=CARTESIAN_POINT('Ctrl Pts',(-9.57754329642214,0.583102430601487,
3.92981017245921));
#12205=CARTESIAN_POINT('Ctrl Pts',(-9.6513665972923,0.293655596344699,3.94181335924853));
#12206=CARTESIAN_POINT('Ctrl Pts',(-9.6758110331057,0.1978137079709,3.94578786493399));
#12207=CARTESIAN_POINT('Ctrl Pts',(-9.68822500000014,0.0989100500907061,
3.94976237061945));
#12208=CARTESIAN_POINT('Ctrl Pts',(-9.688225,-1.74621428428168E-12,3.95373687630491));
#12209=CARTESIAN_POINT('Origin',(-8.5,0.,1.8));
#12210=CARTESIAN_POINT('',(-9.688225,-2.87547763377916E-14,4.29626312369518));
#12211=CARTESIAN_POINT('',(-9.688225,-1.76286762965105E-12,4.25373687630491));
#12212=CARTESIAN_POINT('',(-9.688225,-1.45515594291686E-16,1.8));
#12213=CARTESIAN_POINT('Ctrl Pts',(-9.688225,-2.03170813506404E-14,4.29626312369518));
#12214=CARTESIAN_POINT('Ctrl Pts',(-9.68822500000001,0.298712821306068,
4.28425993690586));
#12215=CARTESIAN_POINT('Ctrl Pts',(-9.57054245632588,0.595858078271499,
4.27225675011654));
#12216=CARTESIAN_POINT('Ctrl Pts',(-9.36601586214937,0.813569405232692,
4.26025356332722));
#12217=CARTESIAN_POINT('Ctrl Pts',(-9.16148926797287,1.03128073219389,4.24825037653791));
#12218=CARTESIAN_POINT('Ctrl Pts',(-8.87226522412851,1.16727314847134,4.23624718974859));
#12219=CARTESIAN_POINT('Ctrl Pts',(-8.57413435701456,1.1859100926019,4.22424400295927));
#12220=CARTESIAN_POINT('Ctrl Pts',(-8.2760034899006,1.20454703673245,4.21224081616995));
#12221=CARTESIAN_POINT('Ctrl Pts',(-7.97209482032102,1.10563290540113,4.20023762938064));
#12222=CARTESIAN_POINT('Ctrl Pts',(-7.74204705372069,0.915087963996635,
4.18823444259132));
#12223=CARTESIAN_POINT('Ctrl Pts',(-7.51199928712035,0.724543022592141,
4.176231255802));
#12224=CARTESIAN_POINT('Ctrl Pts',(-7.35822688079639,0.444367128061576,
4.16422806901268));
#12225=CARTESIAN_POINT('Ctrl Pts',(-7.32102560975819,0.147979855990413,
4.15222488222336));
#12226=CARTESIAN_POINT('Ctrl Pts',(-7.28382433871999,-0.148407416080749,
4.14022169543405));
#12227=CARTESIAN_POINT('Ctrl Pts',(-7.36358464744631,-0.45789534472183,
4.12821850864473));
#12228=CARTESIAN_POINT('Ctrl Pts',(-7.53940549437874,-0.699383189957584,
4.11621532185541));
#12229=CARTESIAN_POINT('Ctrl Pts',(-7.71522634131116,-0.940871035193337,
4.10421213506609));
#12230=CARTESIAN_POINT('Ctrl Pts',(-7.9852624056577,-1.11182427083076,4.09220894827678));
#12231=CARTESIAN_POINT('Ctrl Pts',(-8.27875123560101,-1.16744491727744,
4.08020576148746));
#12232=CARTESIAN_POINT('Ctrl Pts',(-8.57224006554433,-1.22306556372412,
4.06820257469814));
#12233=CARTESIAN_POINT('Ctrl Pts',(-8.88610136059923,-1.1627698566703,4.05619938790882));
#12234=CARTESIAN_POINT('Ctrl Pts',(-9.13808834820079,-1.00235817476359,
4.04419620111951));
#12235=CARTESIAN_POINT('Ctrl Pts',(-9.39007533580234,-0.841946492856881,
4.03219301433019));
#12236=CARTESIAN_POINT('Ctrl Pts',(-9.57754329642127,-0.58310243060309,
4.02018982754087));
#12237=CARTESIAN_POINT('Ctrl Pts',(-9.65136659729186,-0.293655596346411,
4.00818664075155));
#12238=CARTESIAN_POINT('Ctrl Pts',(-9.67581103310541,-0.197813707972643,
4.00421213506609));
#12239=CARTESIAN_POINT('Ctrl Pts',(-9.688225,-0.0989100500924617,4.00023762938063));
#12240=CARTESIAN_POINT('Ctrl Pts',(-9.688225,-3.66373598126302E-15,3.99626312369518));
#12241=CARTESIAN_POINT('Ctrl Pts',(-9.688225,-1.74621428428168E-12,3.95373687630491));
#12242=CARTESIAN_POINT('Ctrl Pts',(-9.68822499999956,-0.298712821307834,
3.96574006309423));
#12243=CARTESIAN_POINT('Ctrl Pts',(-9.57054245632499,-0.595858078273091,
3.97774324988354));
#12244=CARTESIAN_POINT('Ctrl Pts',(-9.36601586214816,-0.81356940523398,
3.98974643667286));
#12245=CARTESIAN_POINT('Ctrl Pts',(-9.16148926797134,-1.03128073219487,
4.00174962346218));
#12246=CARTESIAN_POINT('Ctrl Pts',(-8.87226522412678,-1.16727314847189,
4.0137528102515));
#12247=CARTESIAN_POINT('Ctrl Pts',(-8.5741343570128,-1.18591009260201,4.02575599704081));
#12248=CARTESIAN_POINT('Ctrl Pts',(-8.27600348989881,-1.20454703673212,
4.03775918383013));
#12249=CARTESIAN_POINT('Ctrl Pts',(-7.97209482031937,-1.10563290540034,
4.04976237061945));
#12250=CARTESIAN_POINT('Ctrl Pts',(-7.74204705371933,-0.915087963995508,
4.06176555740877));
#12251=CARTESIAN_POINT('Ctrl Pts',(-7.51199928711928,-0.724543022590671,
4.07376874419808));
#12252=CARTESIAN_POINT('Ctrl Pts',(-7.35822688079573,-0.444367128059878,
4.0857719309874));
#12253=CARTESIAN_POINT('Ctrl Pts',(-7.32102560975797,-0.14797985598866,
4.09777511777672));
#12254=CARTESIAN_POINT('Ctrl Pts',(-7.28382433872021,0.148407416082557,
4.10977830456604));
#12255=CARTESIAN_POINT('Ctrl Pts',(-7.363584647447,0.45789534472352,4.12178149135535));
#12256=CARTESIAN_POINT('Ctrl Pts',(-7.53940549437978,0.699383189959012,
4.13378467814467));
#12257=CARTESIAN_POINT('Ctrl Pts',(-7.71522634131256,0.940871035194504,
4.14578786493399));
#12258=CARTESIAN_POINT('Ctrl Pts',(-7.98526240565935,1.11182427083152,4.15779105172331));
#12259=CARTESIAN_POINT('Ctrl Pts',(-8.27875123560275,1.16744491727777,4.16979423851263));
#12260=CARTESIAN_POINT('Ctrl Pts',(-8.57224006554614,1.22306556372401,4.18179742530194));
#12261=CARTESIAN_POINT('Ctrl Pts',(-8.88610136060096,1.16276985666972,4.19380061209126));
#12262=CARTESIAN_POINT('Ctrl Pts',(-9.13808834820228,1.00235817476264,4.20580379888058));
#12263=CARTESIAN_POINT('Ctrl Pts',(-9.39007533580359,0.841946492855557,
4.2178069856699));
#12264=CARTESIAN_POINT('Ctrl Pts',(-9.57754329642213,0.583102430601487,
4.22981017245921));
#12265=CARTESIAN_POINT('Ctrl Pts',(-9.6513665972923,0.293655596344699,4.24181335924853));
#12266=CARTESIAN_POINT('Ctrl Pts',(-9.6758110331057,0.197813707970898,4.24578786493399));
#12267=CARTESIAN_POINT('Ctrl Pts',(-9.68822500000014,0.0989100500907007,
4.24976237061945));
#12268=CARTESIAN_POINT('Ctrl Pts',(-9.688225,-1.7544299346639E-12,4.25373687630491));
#12269=CARTESIAN_POINT('Origin',(-8.5,0.,1.8));
#12270=CARTESIAN_POINT('',(-9.688225,-3.68594044175552E-14,4.59626312369518));
#12271=CARTESIAN_POINT('',(-9.688225,-1.77097225773082E-12,4.55373687630491));
#12272=CARTESIAN_POINT('',(-9.688225,-1.45515594291686E-16,1.8));
#12273=CARTESIAN_POINT('Ctrl Pts',(-9.688225,-1.15463194561016E-14,4.59626312369518));
#12274=CARTESIAN_POINT('Ctrl Pts',(-9.688225,0.298712821306079,4.58425993690586));
#12275=CARTESIAN_POINT('Ctrl Pts',(-9.57054245632587,0.595858078271513,
4.57225675011654));
#12276=CARTESIAN_POINT('Ctrl Pts',(-9.36601586214936,0.813569405232705,
4.56025356332722));
#12277=CARTESIAN_POINT('Ctrl Pts',(-9.16148926797286,1.0312807321939,4.54825037653791));
#12278=CARTESIAN_POINT('Ctrl Pts',(-8.87226522412849,1.16727314847135,4.53624718974859));
#12279=CARTESIAN_POINT('Ctrl Pts',(-8.57413435701453,1.1859100926019,4.52424400295927));
#12280=CARTESIAN_POINT('Ctrl Pts',(-8.27600348990058,1.20454703673245,4.51224081616995));
#12281=CARTESIAN_POINT('Ctrl Pts',(-7.97209482032099,1.10563290540112,4.50023762938063));
#12282=CARTESIAN_POINT('Ctrl Pts',(-7.74204705372066,0.915087963996614,
4.48823444259132));
#12283=CARTESIAN_POINT('Ctrl Pts',(-7.51199928712033,0.724543022592111,
4.476231255802));
#12284=CARTESIAN_POINT('Ctrl Pts',(-7.35822688079637,0.444367128061538,
4.46422806901268));
#12285=CARTESIAN_POINT('Ctrl Pts',(-7.32102560975818,0.147979855990371,
4.45222488222336));
#12286=CARTESIAN_POINT('Ctrl Pts',(-7.28382433871999,-0.148407416080795,
4.44022169543405));
#12287=CARTESIAN_POINT('Ctrl Pts',(-7.36358464744633,-0.457895344721877,
4.42821850864473));
#12288=CARTESIAN_POINT('Ctrl Pts',(-7.53940549437877,-0.699383189957625,
4.41621532185541));
#12289=CARTESIAN_POINT('Ctrl Pts',(-7.71522634131121,-0.940871035193374,
4.40421213506609));
#12290=CARTESIAN_POINT('Ctrl Pts',(-7.98526240565775,-1.11182427083078,
4.39220894827677));
#12291=CARTESIAN_POINT('Ctrl Pts',(-8.27875123560107,-1.16744491727745,
4.38020576148746));
#12292=CARTESIAN_POINT('Ctrl Pts',(-8.57224006554439,-1.22306556372412,
4.36820257469814));
#12293=CARTESIAN_POINT('Ctrl Pts',(-8.8861013605993,-1.16276985667028,4.35619938790882));
#12294=CARTESIAN_POINT('Ctrl Pts',(-9.13808834820084,-1.00235817476355,
4.3441962011195));
#12295=CARTESIAN_POINT('Ctrl Pts',(-9.39007533580239,-0.841946492856829,
4.33219301433019));
#12296=CARTESIAN_POINT('Ctrl Pts',(-9.5775432964213,-0.583102430603023,
4.32018982754087));
#12297=CARTESIAN_POINT('Ctrl Pts',(-9.65136659729188,-0.293655596346337,
4.30818664075155));
#12298=CARTESIAN_POINT('Ctrl Pts',(-9.67581103310541,-0.197813707972598,
4.30421213506609));
#12299=CARTESIAN_POINT('Ctrl Pts',(-9.688225,-0.0989100500924473,4.30023762938063));
#12300=CARTESIAN_POINT('Ctrl Pts',(-9.688225,-2.03170813506404E-14,4.29626312369518));
#12301=CARTESIAN_POINT('Ctrl Pts',(-9.688225,-1.7544299346639E-12,4.25373687630491));
#12302=CARTESIAN_POINT('Ctrl Pts',(-9.68822499999956,-0.298712821307842,
4.26574006309423));
#12303=CARTESIAN_POINT('Ctrl Pts',(-9.57054245632498,-0.595858078273098,
4.27774324988354));
#12304=CARTESIAN_POINT('Ctrl Pts',(-9.36601586214816,-0.813569405233986,
4.28974643667286));
#12305=CARTESIAN_POINT('Ctrl Pts',(-9.16148926797133,-1.03128073219487,
4.30174962346218));
#12306=CARTESIAN_POINT('Ctrl Pts',(-8.87226522412677,-1.1672731484719,4.3137528102515));
#12307=CARTESIAN_POINT('Ctrl Pts',(-8.57413435701279,-1.18591009260201,
4.32575599704081));
#12308=CARTESIAN_POINT('Ctrl Pts',(-8.27600348989881,-1.20454703673212,
4.33775918383013));
#12309=CARTESIAN_POINT('Ctrl Pts',(-7.97209482031937,-1.10563290540034,
4.34976237061945));
#12310=CARTESIAN_POINT('Ctrl Pts',(-7.74204705371932,-0.915087963995503,
4.36176555740877));
#12311=CARTESIAN_POINT('Ctrl Pts',(-7.51199928711927,-0.724543022590665,
4.37376874419808));
#12312=CARTESIAN_POINT('Ctrl Pts',(-7.35822688079572,-0.44436712805987,
4.3857719309874));
#12313=CARTESIAN_POINT('Ctrl Pts',(-7.32102560975797,-0.147979855988652,
4.39777511777672));
#12314=CARTESIAN_POINT('Ctrl Pts',(-7.28382433872021,0.148407416082565,
4.40977830456604));
#12315=CARTESIAN_POINT('Ctrl Pts',(-7.363584647447,0.457895344723527,4.42178149135536));
#12316=CARTESIAN_POINT('Ctrl Pts',(-7.53940549437978,0.699383189959018,
4.43378467814467));
#12317=CARTESIAN_POINT('Ctrl Pts',(-7.71522634131257,0.94087103519451,4.44578786493399));
#12318=CARTESIAN_POINT('Ctrl Pts',(-7.98526240565936,1.11182427083152,4.45779105172331));
#12319=CARTESIAN_POINT('Ctrl Pts',(-8.27875123560275,1.16744491727777,4.46979423851263));
#12320=CARTESIAN_POINT('Ctrl Pts',(-8.57224006554615,1.22306556372401,4.48179742530194));
#12321=CARTESIAN_POINT('Ctrl Pts',(-8.88610136060097,1.16276985666972,4.49380061209126));
#12322=CARTESIAN_POINT('Ctrl Pts',(-9.13808834820228,1.00235817476264,4.50580379888058));
#12323=CARTESIAN_POINT('Ctrl Pts',(-9.39007533580359,0.841946492855551,
4.5178069856699));
#12324=CARTESIAN_POINT('Ctrl Pts',(-9.57754329642214,0.58310243060148,4.52981017245921));
#12325=CARTESIAN_POINT('Ctrl Pts',(-9.6513665972923,0.293655596344692,4.54181335924853));
#12326=CARTESIAN_POINT('Ctrl Pts',(-9.6758110331057,0.197813707970884,4.54578786493399));
#12327=CARTESIAN_POINT('Ctrl Pts',(-9.68822500000015,0.0989100500906813,
4.54976237061945));
#12328=CARTESIAN_POINT('Ctrl Pts',(-9.688225,-1.7794654638692E-12,4.55373687630491));
#12329=CARTESIAN_POINT('Origin',(-8.5,0.,1.8));
#12330=CARTESIAN_POINT('',(-9.688225,-4.50750547997814E-14,4.89626312369518));
#12331=CARTESIAN_POINT('',(-9.68890234474114,2.93777303478513E-5,4.85373687630491));
#12332=CARTESIAN_POINT('',(-9.688225,-1.45515594291686E-16,1.8));
#12333=CARTESIAN_POINT('Ctrl Pts',(-9.688225,-2.80886425230165E-14,4.89626312369518));
#12334=CARTESIAN_POINT('Ctrl Pts',(-9.68822500000001,0.29871282130606,4.88425993690586));
#12335=CARTESIAN_POINT('Ctrl Pts',(-9.57054245632588,0.595858078271492,
4.87225675011654));
#12336=CARTESIAN_POINT('Ctrl Pts',(-9.36601586214938,0.813569405232687,
4.86025356332722));
#12337=CARTESIAN_POINT('Ctrl Pts',(-9.16148926797288,1.03128073219388,4.84825037653791));
#12338=CARTESIAN_POINT('Ctrl Pts',(-8.87226522412852,1.16727314847134,4.83624718974859));
#12339=CARTESIAN_POINT('Ctrl Pts',(-8.57413435701457,1.1859100926019,4.82424400295927));
#12340=CARTESIAN_POINT('Ctrl Pts',(-8.27600348990061,1.20454703673246,4.81224081616995));
#12341=CARTESIAN_POINT('Ctrl Pts',(-7.97209482032102,1.10563290540113,4.80023762938064));
#12342=CARTESIAN_POINT('Ctrl Pts',(-7.74204705372069,0.91508796399664,4.78823444259132));
#12343=CARTESIAN_POINT('Ctrl Pts',(-7.51199928712036,0.724543022592147,
4.776231255802));
#12344=CARTESIAN_POINT('Ctrl Pts',(-7.35822688079639,0.444367128061583,
4.76422806901268));
#12345=CARTESIAN_POINT('Ctrl Pts',(-7.32102560975819,0.147979855990421,
4.75222488222337));
#12346=CARTESIAN_POINT('Ctrl Pts',(-7.28382433871998,-0.148407416080741,
4.74022169543405));
#12347=CARTESIAN_POINT('Ctrl Pts',(-7.36358464744631,-0.457895344721823,
4.72821850864473));
#12348=CARTESIAN_POINT('Ctrl Pts',(-7.53940549437873,-0.699383189957578,
4.71621532185541));
#12349=CARTESIAN_POINT('Ctrl Pts',(-7.71522634131116,-0.940871035193332,
4.7042121350661));
#12350=CARTESIAN_POINT('Ctrl Pts',(-7.98526240565769,-1.11182427083075,
4.69220894827678));
#12351=CARTESIAN_POINT('Ctrl Pts',(-8.278751235601,-1.16744491727744,4.68020576148746));
#12352=CARTESIAN_POINT('Ctrl Pts',(-8.57224006554432,-1.22306556372412,
4.66820257469814));
#12353=CARTESIAN_POINT('Ctrl Pts',(-8.88610136059923,-1.1627698566703,4.65619938790882));
#12354=CARTESIAN_POINT('Ctrl Pts',(-9.13808834820078,-1.00235817476359,
4.64419620111951));
#12355=CARTESIAN_POINT('Ctrl Pts',(-9.39007533580233,-0.841946492856887,
4.63219301433019));
#12356=CARTESIAN_POINT('Ctrl Pts',(-9.57754329642126,-0.583102430603097,
4.62018982754087));
#12357=CARTESIAN_POINT('Ctrl Pts',(-9.65136659729186,-0.293655596346419,
4.60818664075155));
#12358=CARTESIAN_POINT('Ctrl Pts',(-9.67581103310541,-0.197813707972651,
4.60421213506609));
#12359=CARTESIAN_POINT('Ctrl Pts',(-9.688225,-0.0989100500924695,4.60023762938064));
#12360=CARTESIAN_POINT('Ctrl Pts',(-9.688225,-1.15463194561016E-14,4.59626312369518));
#12361=CARTESIAN_POINT('Ctrl Pts',(-9.688225,-1.7794654638692E-12,4.55373687630491));
#12362=CARTESIAN_POINT('Ctrl Pts',(-9.68822499999955,-0.298712821307867,
4.56574006309423));
#12363=CARTESIAN_POINT('Ctrl Pts',(-9.57054245632497,-0.595858078273121,
4.57774324988354));
#12364=CARTESIAN_POINT('Ctrl Pts',(-9.36601586214814,-0.813569405234004,
4.58974643667286));
#12365=CARTESIAN_POINT('Ctrl Pts',(-9.16148926797131,-1.03128073219489,
4.60174962346218));
#12366=CARTESIAN_POINT('Ctrl Pts',(-8.87226522412674,-1.1672731484719,4.6137528102515));
#12367=CARTESIAN_POINT('Ctrl Pts',(-8.57413435701276,-1.18591009260201,
4.62575599704082));
#12368=CARTESIAN_POINT('Ctrl Pts',(-8.27600348989878,-1.20454703673211,
4.63775918383013));
#12369=CARTESIAN_POINT('Ctrl Pts',(-7.97209482031934,-1.10563290540033,
4.64976237061945));
#12370=CARTESIAN_POINT('Ctrl Pts',(-7.7420470537193,-0.915087963995487,
4.66176555740877));
#12371=CARTESIAN_POINT('Ctrl Pts',(-7.51199928711926,-0.724543022590644,
4.67376874419809));
#12372=CARTESIAN_POINT('Ctrl Pts',(-7.35822688079571,-0.444367128059846,
4.6857719309874));
#12373=CARTESIAN_POINT('Ctrl Pts',(-7.32102560975796,-0.147979855988628,
4.69777511777672));
#12374=CARTESIAN_POINT('Ctrl Pts',(-7.28382433872021,0.148407416082591,
4.70977830456604));
#12375=CARTESIAN_POINT('Ctrl Pts',(-7.36358464744701,0.457895344723551,
4.72178149135536));
#12376=CARTESIAN_POINT('Ctrl Pts',(-7.5394054943798,0.699383189959039,4.73378467814467));
#12377=CARTESIAN_POINT('Ctrl Pts',(-7.71522634131259,0.940871035194526,
4.74578786493399));
#12378=CARTESIAN_POINT('Ctrl Pts',(-7.98526240565938,1.11182427083153,4.75779105172331));
#12379=CARTESIAN_POINT('Ctrl Pts',(-8.27875123560278,1.16744491727777,4.76979423851263));
#12380=CARTESIAN_POINT('Ctrl Pts',(-8.57224006554618,1.22306556372401,4.78179742530194));
#12381=CARTESIAN_POINT('Ctrl Pts',(-8.886101360601,1.16276985666971,4.79380061209126));
#12382=CARTESIAN_POINT('Ctrl Pts',(-9.1380883482023,1.00235817476262,4.80580379888058));
#12383=CARTESIAN_POINT('Ctrl Pts',(-9.39007533580361,0.841946492855533,
4.8178069856699));
#12384=CARTESIAN_POINT('Ctrl Pts',(-9.57754329642215,0.583102430601457,
4.82981017245922));
#12385=CARTESIAN_POINT('Ctrl Pts',(-9.6513665972923,0.293655596344667,4.84181335924853));
#12386=CARTESIAN_POINT('Ctrl Pts',(-9.67581103310571,0.19781370797087,4.84578786493399));
#12387=CARTESIAN_POINT('Ctrl Pts',(-9.68822500000015,0.0989100500906788,
4.84976237061945));
#12388=CARTESIAN_POINT('Ctrl Pts',(-9.688225,-1.77075021312589E-12,4.85373687630491));
#12389=CARTESIAN_POINT('Origin',(-8.5,0.,1.8));
#12390=CARTESIAN_POINT('',(-9.688225,-5.3179682879545E-14,5.19626312369518));
#12391=CARTESIAN_POINT('',(-9.68763172722904,0.00105126113166729,5.15373687630492));
#12392=CARTESIAN_POINT('',(-9.688225,-1.45515594291686E-16,1.8));
#12393=CARTESIAN_POINT('Ctrl Pts',(-9.688225,-3.61932706027801E-14,5.19626312369518));
#12394=CARTESIAN_POINT('Ctrl Pts',(-9.68822500000001,0.298712821306057,
5.18425993690586));
#12395=CARTESIAN_POINT('Ctrl Pts',(-9.57054245632588,0.595858078271496,
5.17225675011654));
#12396=CARTESIAN_POINT('Ctrl Pts',(-9.36601586214937,0.813569405232693,
5.16025356332722));
#12397=CARTESIAN_POINT('Ctrl Pts',(-9.16148926797287,1.03128073219389,5.14825037653791));
#12398=CARTESIAN_POINT('Ctrl Pts',(-8.8722652241285,1.16727314847134,5.13624718974859));
#12399=CARTESIAN_POINT('Ctrl Pts',(-8.57413435701454,1.1859100926019,5.12424400295927));
#12400=CARTESIAN_POINT('Ctrl Pts',(-8.27600348990058,1.20454703673245,5.11224081616995));
#12401=CARTESIAN_POINT('Ctrl Pts',(-7.97209482032099,1.10563290540112,5.10023762938063));
#12402=CARTESIAN_POINT('Ctrl Pts',(-7.74204705372066,0.915087963996613,
5.08823444259132));
#12403=CARTESIAN_POINT('Ctrl Pts',(-7.51199928712033,0.724543022592108,
5.076231255802));
#12404=CARTESIAN_POINT('Ctrl Pts',(-7.35822688079637,0.444367128061532,
5.06422806901268));
#12405=CARTESIAN_POINT('Ctrl Pts',(-7.32102560975818,0.147979855990362,
5.05222488222336));
#12406=CARTESIAN_POINT('Ctrl Pts',(-7.28382433871999,-0.148407416080807,
5.04022169543405));
#12407=CARTESIAN_POINT('Ctrl Pts',(-7.36358464744634,-0.457895344721891,
5.02821850864473));
#12408=CARTESIAN_POINT('Ctrl Pts',(-7.53940549437878,-0.699383189957639,
5.01621532185541));
#12409=CARTESIAN_POINT('Ctrl Pts',(-7.71522634131122,-0.940871035193387,
5.00421213506609));
#12410=CARTESIAN_POINT('Ctrl Pts',(-7.98526240565777,-1.11182427083079,
4.99220894827677));
#12411=CARTESIAN_POINT('Ctrl Pts',(-8.27875123560109,-1.16744491727745,
4.98020576148746));
#12412=CARTESIAN_POINT('Ctrl Pts',(-8.57224006554442,-1.22306556372411,
4.96820257469814));
#12413=CARTESIAN_POINT('Ctrl Pts',(-8.88610136059933,-1.16276985667027,
4.95619938790882));
#12414=CARTESIAN_POINT('Ctrl Pts',(-9.13808834820087,-1.00235817476353,
4.9441962011195));
#12415=CARTESIAN_POINT('Ctrl Pts',(-9.39007533580241,-0.841946492856801,
4.93219301433018));
#12416=CARTESIAN_POINT('Ctrl Pts',(-9.57754329642133,-0.583102430602987,
4.92018982754087));
#12417=CARTESIAN_POINT('Ctrl Pts',(-9.65136659729189,-0.293655596346296,
4.90818664075155));
#12418=CARTESIAN_POINT('Ctrl Pts',(-9.67581103310542,-0.197813707972572,
4.90421213506609));
#12419=CARTESIAN_POINT('Ctrl Pts',(-9.688225,-0.0989100500924382,4.90023762938063));
#12420=CARTESIAN_POINT('Ctrl Pts',(-9.688225,-2.80886425230165E-14,4.89626312369518));
#12421=CARTESIAN_POINT('Ctrl Pts',(-9.69028763874726,8.94605781823637E-5,
4.8537368763049));
#12422=CARTESIAN_POINT('Ctrl Pts',(-9.69029065164093,-0.00381389069076675,
4.85389441790699));
#12423=CARTESIAN_POINT('Ctrl Pts',(-9.69027262936407,-0.00771725416388489,
4.85405195950908));
#12424=CARTESIAN_POINT('Ctrl Pts',(-9.69023347715143,-0.0116204539158122,
4.85420950111117));
#12425=CARTESIAN_POINT('Ctrl Pts',(-9.68628018738611,-0.405735590575178,
4.87011684226279));
#12426=CARTESIAN_POINT('Ctrl Pts',(-9.46689854929461,-0.798181522642429,
4.88602418341442));
#12427=CARTESIAN_POINT('Ctrl Pts',(-9.13347788059196,-1.00774237159632,
4.90193152456604));
#12428=CARTESIAN_POINT('Ctrl Pts',(-8.80005721188931,-1.21730322055022,
4.91783886571766));
#12429=CARTESIAN_POINT('Ctrl Pts',(-8.35259751257551,-1.24397898639076,
4.93374620686927));
#12430=CARTESIAN_POINT('Ctrl Pts',(-7.99517517866866,-1.07733253192674,
4.9496535480209));
#12431=CARTESIAN_POINT('Ctrl Pts',(-7.81646401171523,-0.994009304694722,
4.95760721859671));
#12432=CARTESIAN_POINT('Ctrl Pts',(-7.66026218611355,-0.86235552238656,
4.96556088917252));
#12433=CARTESIAN_POINT('Ctrl Pts',(-7.54281123274328,-0.702270971137819,
4.97351455974833));
#12434=CARTESIAN_POINT('Ctrl Pts',(-7.42536027937301,-0.542186419889074,
4.98146823032414));
#12435=CARTESIAN_POINT('Ctrl Pts',(-7.34666019823415,-0.353671099699739,
4.98942190089995));
#12436=CARTESIAN_POINT('Ctrl Pts',(-7.32081840553957,-0.158190555551361,
4.99737557147576));
#12437=CARTESIAN_POINT('Ctrl Pts',(-7.26913482015041,0.232770532745374,
5.01328291262738));
#12438=CARTESIAN_POINT('Ctrl Pts',(-7.42888438853832,0.651592516878301,
5.029190253779));
#12439=CARTESIAN_POINT('Ctrl Pts',(-7.72885825501123,0.906741044535612,
5.04509759493063));
#12440=CARTESIAN_POINT('Ctrl Pts',(-8.02883212148414,1.16188957219293,5.06100493608225));
#12441=CARTESIAN_POINT('Ctrl Pts',(-8.46903028604204,1.25336464337461,5.07691227723386));
#12442=CARTESIAN_POINT('Ctrl Pts',(-8.84616049271118,1.13884313158887,5.09281961838548));
#12443=CARTESIAN_POINT('Ctrl Pts',(-9.22329069938031,1.02432161980314,5.1087269595371));
#12444=CARTESIAN_POINT('Ctrl Pts',(-9.53735294816069,0.703803525049966,
5.12463430068873));
#12445=CARTESIAN_POINT('Ctrl Pts',(-9.64487175298678,0.324706029258399,
5.14054164184035));
#12446=CARTESIAN_POINT('Ctrl Pts',(-9.67460091651171,0.219884817168954,
5.14494005332854));
#12447=CARTESIAN_POINT('Ctrl Pts',(-9.68853914169805,0.110585013592906,
5.14933846481673));
#12448=CARTESIAN_POINT('Ctrl Pts',(-9.68763172722904,0.00105126113166729,
5.15373687630492));
#12449=CARTESIAN_POINT('Origin',(-8.5,0.,1.8));
#12450=CARTESIAN_POINT('',(-9.688225,-6.12843109593086E-14,5.49626312369518));
#12451=CARTESIAN_POINT('',(-9.68743616841376,-0.000177656540254041,5.45373687630491));
#12452=CARTESIAN_POINT('',(-9.688225,-1.45515594291686E-16,1.8));
#12453=CARTESIAN_POINT('Ctrl Pts',(-9.688225,-4.45199432874688E-14,5.49626312369518));
#12454=CARTESIAN_POINT('Ctrl Pts',(-9.68822500000001,0.298712821306043,
5.48425993690586));
#12455=CARTESIAN_POINT('Ctrl Pts',(-9.57054245632589,0.595858078271478,
5.47225675011654));
#12456=CARTESIAN_POINT('Ctrl Pts',(-9.36601586214939,0.813569405232675,
5.46025356332723));
#12457=CARTESIAN_POINT('Ctrl Pts',(-9.16148926797289,1.03128073219387,5.44825037653791));
#12458=CARTESIAN_POINT('Ctrl Pts',(-8.87226522412853,1.16727314847133,5.43624718974859));
#12459=CARTESIAN_POINT('Ctrl Pts',(-8.57413435701458,1.1859100926019,5.42424400295927));
#12460=CARTESIAN_POINT('Ctrl Pts',(-8.27600348990063,1.20454703673246,5.41224081616995));
#12461=CARTESIAN_POINT('Ctrl Pts',(-7.97209482032104,1.10563290540114,5.40023762938064));
#12462=CARTESIAN_POINT('Ctrl Pts',(-7.7420470537207,0.915087963996651,5.38823444259132));
#12463=CARTESIAN_POINT('Ctrl Pts',(-7.51199928712037,0.724543022592161,
5.376231255802));
#12464=CARTESIAN_POINT('Ctrl Pts',(-7.3582268807964,0.444367128061599,5.36422806901268));
#12465=CARTESIAN_POINT('Ctrl Pts',(-7.32102560975819,0.147979855990437,
5.35222488222337));
#12466=CARTESIAN_POINT('Ctrl Pts',(-7.28382433871998,-0.148407416080724,
5.34022169543405));
#12467=CARTESIAN_POINT('Ctrl Pts',(-7.3635846474463,-0.457895344721807,
5.32821850864473));
#12468=CARTESIAN_POINT('Ctrl Pts',(-7.53940549437872,-0.699383189957564,
5.31621532185541));
#12469=CARTESIAN_POINT('Ctrl Pts',(-7.71522634131115,-0.940871035193321,
5.3042121350661));
#12470=CARTESIAN_POINT('Ctrl Pts',(-7.98526240565767,-1.11182427083074,
5.29220894827678));
#12471=CARTESIAN_POINT('Ctrl Pts',(-8.27875123560099,-1.16744491727743,
5.28020576148746));
#12472=CARTESIAN_POINT('Ctrl Pts',(-8.5722400655443,-1.22306556372412,5.26820257469814));
#12473=CARTESIAN_POINT('Ctrl Pts',(-8.88610136059921,-1.1627698566703,5.25619938790882));
#12474=CARTESIAN_POINT('Ctrl Pts',(-9.13808834820077,-1.0023581747636,5.24419620111951));
#12475=CARTESIAN_POINT('Ctrl Pts',(-9.39007533580232,-0.841946492856899,
5.23219301433019));
#12476=CARTESIAN_POINT('Ctrl Pts',(-9.57754329642126,-0.583102430603111,
5.22018982754087));
#12477=CARTESIAN_POINT('Ctrl Pts',(-9.65136659729185,-0.293655596346435,
5.20818664075155));
#12478=CARTESIAN_POINT('Ctrl Pts',(-9.6758110331054,-0.19781370797267,5.2042121350661));
#12479=CARTESIAN_POINT('Ctrl Pts',(-9.688225,-0.0989100500924914,5.20023762938064));
#12480=CARTESIAN_POINT('Ctrl Pts',(-9.688225,-3.61932706027801E-14,5.19626312369518));
#12481=CARTESIAN_POINT('Ctrl Pts',(-9.68763172722904,0.00105126113166729,
5.15373687630492));
#12482=CARTESIAN_POINT('Ctrl Pts',(-9.68525737700568,-0.285555905167675,
5.16524580596835));
#12483=CARTESIAN_POINT('Ctrl Pts',(-9.58124012083503,-0.573764837715244,
5.17675473563178));
#12484=CARTESIAN_POINT('Ctrl Pts',(-9.39251500118686,-0.787532689948571,
5.18826366529521));
#12485=CARTESIAN_POINT('Ctrl Pts',(-9.13166408368907,-1.08299701653396,
5.20417100644683));
#12486=CARTESIAN_POINT('Ctrl Pts',(-8.7089868878217,-1.23624877287478,5.22007834759846));
#12487=CARTESIAN_POINT('Ctrl Pts',(-8.3197251524468,-1.17657974317491,5.23598568875008));
#12488=CARTESIAN_POINT('Ctrl Pts',(-7.9304634170719,-1.11691071347503,5.25189302990169));
#12489=CARTESIAN_POINT('Ctrl Pts',(-7.57461714218948,-0.844320897734477,
5.26780037105331));
#12490=CARTESIAN_POINT('Ctrl Pts',(-7.4133485788613,-0.484440061841653,
5.28370771220493));
#12491=CARTESIAN_POINT('Ctrl Pts',(-7.33271429719722,-0.304499643895246,
5.29166138278075));
#12492=CARTESIAN_POINT('Ctrl Pts',(-7.30072444342169,-0.102736470910765,
5.29961505335656));
#12493=CARTESIAN_POINT('Ctrl Pts',(-7.31664171845983,0.0951736863613,5.30756872393237));
#12494=CARTESIAN_POINT('Ctrl Pts',(-7.33255899349796,0.29308384363337,5.31552239450818));
#12495=CARTESIAN_POINT('Ctrl Pts',(-7.39638339734975,0.487140985193029,
5.32347606508399));
#12496=CARTESIAN_POINT('Ctrl Pts',(-7.50473925661838,0.651881536219088,
5.33142973565979));
#12497=CARTESIAN_POINT('Ctrl Pts',(-7.72145097515565,0.981362638271211,
5.34733707681141));
#12498=CARTESIAN_POINT('Ctrl Pts',(-8.11628851536029,1.19357737818891,5.36324441796304));
#12499=CARTESIAN_POINT('Ctrl Pts',(-8.51008305302381,1.19026771978055,5.37915175911466));
#12500=CARTESIAN_POINT('Ctrl Pts',(-8.90387759068732,1.18695806137218,5.39505910026629));
#12501=CARTESIAN_POINT('Ctrl Pts',(-9.29662912580972,0.968124004637758,
5.4109664414179));
#12502=CARTESIAN_POINT('Ctrl Pts',(-9.50690608495474,0.6347683838711,5.42687378256952));
#12503=CARTESIAN_POINT('Ctrl Pts',(-9.62527260118696,0.447119943181184,
5.43582814714798));
#12504=CARTESIAN_POINT('Ctrl Pts',(-9.68581929966714,0.2231836200531,5.44478251172644));
#12505=CARTESIAN_POINT('Ctrl Pts',(-9.68639654153517,-0.000411795887354318,
5.45373687630491));
#12506=CARTESIAN_POINT('Origin',(-8.5,0.,1.8));
#12507=CARTESIAN_POINT('',(-9.688225,-6.94999613415348E-14,5.79626312369518));
#12508=CARTESIAN_POINT('',(-9.688225,-1.8036128146548E-12,5.75373687630491));
#12509=CARTESIAN_POINT('',(-9.688225,-1.45515594291686E-16,1.8));
#12510=CARTESIAN_POINT('Ctrl Pts',(-9.688225,-5.26245713672324E-14,5.79626312369518));
#12511=CARTESIAN_POINT('Ctrl Pts',(-9.68822500000001,0.29871282130603,5.78425993690586));
#12512=CARTESIAN_POINT('Ctrl Pts',(-9.5705424563259,0.595858078271459,5.77225675011654));
#12513=CARTESIAN_POINT('Ctrl Pts',(-9.36601586214941,0.813569405232657,
5.76025356332723));
#12514=CARTESIAN_POINT('Ctrl Pts',(-9.16148926797292,1.03128073219385,5.74825037653791));
#12515=CARTESIAN_POINT('Ctrl Pts',(-8.87226522412857,1.16727314847132,5.73624718974859));
#12516=CARTESIAN_POINT('Ctrl Pts',(-8.57413435701462,1.18591009260189,5.72424400295927));
#12517=CARTESIAN_POINT('Ctrl Pts',(-8.27600348990068,1.20454703673247,5.71224081616996));
#12518=CARTESIAN_POINT('Ctrl Pts',(-7.97209482032109,1.10563290540116,5.70023762938064));
#12519=CARTESIAN_POINT('Ctrl Pts',(-7.74204705372075,0.915087963996688,
5.68823444259132));
#12520=CARTESIAN_POINT('Ctrl Pts',(-7.51199928712041,0.724543022592213,
5.676231255802));
#12521=CARTESIAN_POINT('Ctrl Pts',(-7.35822688079642,0.444367128061666,
5.66422806901269));
#12522=CARTESIAN_POINT('Ctrl Pts',(-7.3210256097582,0.147979855990512,5.65222488222337));
#12523=CARTESIAN_POINT('Ctrl Pts',(-7.28382433871997,-0.148407416080641,
5.64022169543405));
#12524=CARTESIAN_POINT('Ctrl Pts',(-7.36358464744627,-0.457895344721723,
5.62821850864473));
#12525=CARTESIAN_POINT('Ctrl Pts',(-7.53940549437867,-0.699383189957489,
5.61621532185542));
#12526=CARTESIAN_POINT('Ctrl Pts',(-7.71522634131107,-0.940871035193256,
5.6042121350661));
#12527=CARTESIAN_POINT('Ctrl Pts',(-7.98526240565758,-1.1118242708307,5.59220894827678));
#12528=CARTESIAN_POINT('Ctrl Pts',(-8.27875123560088,-1.16744491727741,
5.58020576148746));
#12529=CARTESIAN_POINT('Ctrl Pts',(-8.57224006554418,-1.22306556372413,
5.56820257469815));
#12530=CARTESIAN_POINT('Ctrl Pts',(-8.88610136059909,-1.16276985667034,
5.55619938790883));
#12531=CARTESIAN_POINT('Ctrl Pts',(-9.13808834820066,-1.00235817476367,
5.54419620111951));
#12532=CARTESIAN_POINT('Ctrl Pts',(-9.39007533580222,-0.841946492856997,
5.5321930143302));
#12533=CARTESIAN_POINT('Ctrl Pts',(-9.57754329642119,-0.583102430603236,
5.52018982754088));
#12534=CARTESIAN_POINT('Ctrl Pts',(-9.65136659729182,-0.293655596346573,
5.50818664075156));
#12535=CARTESIAN_POINT('Ctrl Pts',(-9.67581103310539,-0.197813707972768,
5.5042121350661));
#12536=CARTESIAN_POINT('Ctrl Pts',(-9.688225,-0.0989100500925447,5.50023762938064));
#12537=CARTESIAN_POINT('Ctrl Pts',(-9.688225,-4.45199432874688E-14,5.49626312369518));
#12538=CARTESIAN_POINT('Ctrl Pts',(-9.688225,-1.76175740662643E-12,5.45373687630491));
#12539=CARTESIAN_POINT('Ctrl Pts',(-9.68822499999956,-0.298712821307844,
5.46574006309423));
#12540=CARTESIAN_POINT('Ctrl Pts',(-9.57054245632499,-0.595858078273094,
5.47774324988354));
#12541=CARTESIAN_POINT('Ctrl Pts',(-9.36601586214817,-0.813569405233979,
5.48974643667286));
#12542=CARTESIAN_POINT('Ctrl Pts',(-9.16148926797134,-1.03128073219486,
5.50174962346218));
#12543=CARTESIAN_POINT('Ctrl Pts',(-8.87226522412679,-1.16727314847189,
5.5137528102515));
#12544=CARTESIAN_POINT('Ctrl Pts',(-8.57413435701281,-1.18591009260201,
5.52575599704081));
#12545=CARTESIAN_POINT('Ctrl Pts',(-8.27600348989884,-1.20454703673212,
5.53775918383013));
#12546=CARTESIAN_POINT('Ctrl Pts',(-7.9720948203194,-1.10563290540036,5.54976237061945));
#12547=CARTESIAN_POINT('Ctrl Pts',(-7.74204705371935,-0.915087963995531,
5.56176555740877));
#12548=CARTESIAN_POINT('Ctrl Pts',(-7.5119992871193,-0.724543022590704,
5.57376874419808));
#12549=CARTESIAN_POINT('Ctrl Pts',(-7.35822688079574,-0.444367128059923,
5.5857719309874));
#12550=CARTESIAN_POINT('Ctrl Pts',(-7.32102560975797,-0.147979855988712,
5.59777511777672));
#12551=CARTESIAN_POINT('Ctrl Pts',(-7.2838243387202,0.148407416082498,5.60977830456603));
#12552=CARTESIAN_POINT('Ctrl Pts',(-7.36358464744697,0.457895344723458,
5.62178149135535));
#12553=CARTESIAN_POINT('Ctrl Pts',(-7.53940549437974,0.699383189958956,
5.63378467814467));
#12554=CARTESIAN_POINT('Ctrl Pts',(-7.71522634131251,0.940871035194454,
5.64578786493399));
#12555=CARTESIAN_POINT('Ctrl Pts',(-7.98526240565927,1.11182427083148,5.65779105172331));
#12556=CARTESIAN_POINT('Ctrl Pts',(-8.27875123560266,1.16744491727775,5.66979423851262));
#12557=CARTESIAN_POINT('Ctrl Pts',(-8.57224006554605,1.22306556372401,5.68179742530194));
#12558=CARTESIAN_POINT('Ctrl Pts',(-8.88610136060087,1.16276985666975,5.69380061209126));
#12559=CARTESIAN_POINT('Ctrl Pts',(-9.13808834820219,1.0023581747627,5.70580379888057));
#12560=CARTESIAN_POINT('Ctrl Pts',(-9.39007533580351,0.841946492855637,
5.71780698566989));
#12561=CARTESIAN_POINT('Ctrl Pts',(-9.57754329642208,0.58310243060159,5.72981017245921));
#12562=CARTESIAN_POINT('Ctrl Pts',(-9.65136659729227,0.293655596344815,
5.74181335924853));
#12563=CARTESIAN_POINT('Ctrl Pts',(-9.67581103310569,0.197813707970967,
5.74578786493399));
#12564=CARTESIAN_POINT('Ctrl Pts',(-9.68822500000015,0.098910050090719,
5.74976237061945));
#12565=CARTESIAN_POINT('Ctrl Pts',(-9.688225,-1.78679293583173E-12,5.75373687630491));
#12566=CARTESIAN_POINT('Origin',(-8.5,0.,1.8));
#12567=CARTESIAN_POINT('',(-9.688225,-7.7715611723761E-14,6.09626312369518));
#12568=CARTESIAN_POINT('',(-9.688225,-1.81177295388579E-12,6.05373687630491));
#12569=CARTESIAN_POINT('',(-9.688225,-1.45515594291686E-16,1.8));
#12570=CARTESIAN_POINT('Ctrl Pts',(-9.688225,-7.7715611723761E-14,6.09626312369518));
#12571=CARTESIAN_POINT('Ctrl Pts',(-9.68822500000002,0.29871282130601,6.08425993690586));
#12572=CARTESIAN_POINT('Ctrl Pts',(-9.5705424563259,0.595858078271448,6.07225675011654));
#12573=CARTESIAN_POINT('Ctrl Pts',(-9.36601586214941,0.813569405232651,
6.06025356332723));
#12574=CARTESIAN_POINT('Ctrl Pts',(-9.16148926797292,1.03128073219385,6.04825037653791));
#12575=CARTESIAN_POINT('Ctrl Pts',(-8.87226522412857,1.16727314847132,6.03624718974859));
#12576=CARTESIAN_POINT('Ctrl Pts',(-8.57413435701461,1.18591009260189,6.02424400295927));
#12577=CARTESIAN_POINT('Ctrl Pts',(-8.27600348990066,1.20454703673246,6.01224081616996));
#12578=CARTESIAN_POINT('Ctrl Pts',(-7.97209482032107,1.10563290540116,6.00023762938064));
#12579=CARTESIAN_POINT('Ctrl Pts',(-7.74204705372073,0.915087963996672,
5.98823444259132));
#12580=CARTESIAN_POINT('Ctrl Pts',(-7.51199928712039,0.724543022592188,
5.976231255802));
#12581=CARTESIAN_POINT('Ctrl Pts',(-7.35822688079641,0.444367128061631,
5.96422806901269));
#12582=CARTESIAN_POINT('Ctrl Pts',(-7.32102560975819,0.14797985599047,5.95222488222337));
#12583=CARTESIAN_POINT('Ctrl Pts',(-7.28382433871998,-0.14840741608069,
5.94022169543405));
#12584=CARTESIAN_POINT('Ctrl Pts',(-7.36358464744629,-0.457895344721775,
5.92821850864473));
#12585=CARTESIAN_POINT('Ctrl Pts',(-7.53940549437871,-0.699383189957538,
5.91621532185541));
#12586=CARTESIAN_POINT('Ctrl Pts',(-7.71522634131112,-0.9408710351933,5.9042121350661));
#12587=CARTESIAN_POINT('Ctrl Pts',(-7.98526240565764,-1.11182427083073,
5.89220894827678));
#12588=CARTESIAN_POINT('Ctrl Pts',(-8.27875123560095,-1.16744491727743,
5.88020576148746));
#12589=CARTESIAN_POINT('Ctrl Pts',(-8.57224006554427,-1.22306556372412,
5.86820257469814));
#12590=CARTESIAN_POINT('Ctrl Pts',(-8.88610136059918,-1.16276985667032,
5.85619938790883));
#12591=CARTESIAN_POINT('Ctrl Pts',(-9.13808834820074,-1.00235817476362,
5.84419620111951));
#12592=CARTESIAN_POINT('Ctrl Pts',(-9.3900753358023,-0.841946492856924,
5.83219301433019));
#12593=CARTESIAN_POINT('Ctrl Pts',(-9.57754329642124,-0.583102430603142,
5.82018982754087));
#12594=CARTESIAN_POINT('Ctrl Pts',(-9.65136659729185,-0.293655596346467,
5.80818664075156));
#12595=CARTESIAN_POINT('Ctrl Pts',(-9.6758110331054,-0.197813707972697,
5.8042121350661));
#12596=CARTESIAN_POINT('Ctrl Pts',(-9.688225,-0.0989100500925134,5.80023762938064));
#12597=CARTESIAN_POINT('Ctrl Pts',(-9.688225,-5.26245713672324E-14,5.79626312369518));
#12598=CARTESIAN_POINT('Ctrl Pts',(-9.688225,-1.78679293583173E-12,5.75373687630491));
#12599=CARTESIAN_POINT('Ctrl Pts',(-9.68822499999955,-0.298712821307875,
5.76574006309423));
#12600=CARTESIAN_POINT('Ctrl Pts',(-9.57054245632497,-0.595858078273127,
5.77774324988355));
#12601=CARTESIAN_POINT('Ctrl Pts',(-9.36601586214814,-0.813569405234009,
5.78974643667286));
#12602=CARTESIAN_POINT('Ctrl Pts',(-9.16148926797131,-1.03128073219489,
5.80174962346218));
#12603=CARTESIAN_POINT('Ctrl Pts',(-8.87226522412674,-1.16727314847191,
5.8137528102515));
#12604=CARTESIAN_POINT('Ctrl Pts',(-8.57413435701275,-1.18591009260201,
5.82575599704082));
#12605=CARTESIAN_POINT('Ctrl Pts',(-8.27600348989877,-1.20454703673211,
5.83775918383013));
#12606=CARTESIAN_POINT('Ctrl Pts',(-7.97209482031934,-1.10563290540033,
5.84976237061945));
#12607=CARTESIAN_POINT('Ctrl Pts',(-7.74204705371929,-0.915087963995482,
5.86176555740877));
#12608=CARTESIAN_POINT('Ctrl Pts',(-7.51199928711925,-0.724543022590638,
5.87376874419809));
#12609=CARTESIAN_POINT('Ctrl Pts',(-7.35822688079571,-0.444367128059839,
5.8857719309874));
#12610=CARTESIAN_POINT('Ctrl Pts',(-7.32102560975796,-0.14797985598862,
5.89777511777672));
#12611=CARTESIAN_POINT('Ctrl Pts',(-7.28382433872021,0.148407416082598,
5.90977830456604));
#12612=CARTESIAN_POINT('Ctrl Pts',(-7.36358464744701,0.457895344723558,
5.92178149135536));
#12613=CARTESIAN_POINT('Ctrl Pts',(-7.5394054943798,0.699383189959045,5.93378467814467));
#12614=CARTESIAN_POINT('Ctrl Pts',(-7.7152263413126,0.940871035194531,5.94578786493399));
#12615=CARTESIAN_POINT('Ctrl Pts',(-7.98526240565939,1.11182427083154,5.95779105172331));
#12616=CARTESIAN_POINT('Ctrl Pts',(-8.27875123560279,1.16744491727777,5.96979423851263));
#12617=CARTESIAN_POINT('Ctrl Pts',(-8.57224006554618,1.22306556372401,5.98179742530195));
#12618=CARTESIAN_POINT('Ctrl Pts',(-8.886101360601,1.16276985666971,5.99380061209126));
#12619=CARTESIAN_POINT('Ctrl Pts',(-9.13808834820231,1.00235817476262,6.00580379888058));
#12620=CARTESIAN_POINT('Ctrl Pts',(-9.39007533580362,0.841946492855527,
6.0178069856699));
#12621=CARTESIAN_POINT('Ctrl Pts',(-9.57754329642215,0.583102430601451,
6.02981017245922));
#12622=CARTESIAN_POINT('Ctrl Pts',(-9.65136659729231,0.29365559634466,6.04181335924853));
#12623=CARTESIAN_POINT('Ctrl Pts',(-9.67581103310571,0.197813707970852,
6.04578786493399));
#12624=CARTESIAN_POINT('Ctrl Pts',(-9.68822500000015,0.098910050090649,
6.04976237061945));
#12625=CARTESIAN_POINT('Ctrl Pts',(-9.688225,-1.81177295388579E-12,6.05373687630491));
#12626=CARTESIAN_POINT('Origin',(-8.5,0.,1.8));
#12627=CARTESIAN_POINT('',(-9.688225,-8.57092175010621E-14,6.39626312369518));
#12628=CARTESIAN_POINT('',(-9.688225,-1.81987758196556E-12,6.35373687630491));
#12629=CARTESIAN_POINT('',(-9.688225,-1.45515594291686E-16,1.8));
#12630=CARTESIAN_POINT('Ctrl Pts',(-9.688225,-8.57092175010621E-14,6.39626312369518));
#12631=CARTESIAN_POINT('Ctrl Pts',(-9.68822500000002,0.298712821306008,
6.38425993690586));
#12632=CARTESIAN_POINT('Ctrl Pts',(-9.5705424563259,0.595858078271451,6.37225675011655));
#12633=CARTESIAN_POINT('Ctrl Pts',(-9.36601586214941,0.813569405232657,
6.36025356332723));
#12634=CARTESIAN_POINT('Ctrl Pts',(-9.16148926797291,1.03128073219386,6.34825037653791));
#12635=CARTESIAN_POINT('Ctrl Pts',(-8.87226522412855,1.16727314847133,6.33624718974859));
#12636=CARTESIAN_POINT('Ctrl Pts',(-8.57413435701459,1.18591009260189,6.32424400295927));
#12637=CARTESIAN_POINT('Ctrl Pts',(-8.27600348990063,1.20454703673246,6.31224081616995));
#12638=CARTESIAN_POINT('Ctrl Pts',(-7.97209482032103,1.10563290540114,6.30023762938064));
#12639=CARTESIAN_POINT('Ctrl Pts',(-7.7420470537207,0.915087963996645,6.28823444259132));
#12640=CARTESIAN_POINT('Ctrl Pts',(-7.51199928712036,0.724543022592149,
6.276231255802));
#12641=CARTESIAN_POINT('Ctrl Pts',(-7.35822688079639,0.444367128061579,
6.26422806901268));
#12642=CARTESIAN_POINT('Ctrl Pts',(-7.32102560975819,0.147979855990411,
6.25222488222337));
#12643=CARTESIAN_POINT('Ctrl Pts',(-7.28382433871999,-0.148407416080757,
6.24022169543405));
#12644=CARTESIAN_POINT('Ctrl Pts',(-7.36358464744632,-0.457895344721844,
6.22821850864473));
#12645=CARTESIAN_POINT('Ctrl Pts',(-7.53940549437875,-0.699383189957599,
6.21621532185541));
#12646=CARTESIAN_POINT('Ctrl Pts',(-7.71522634131118,-0.940871035193355,
6.20421213506609));
#12647=CARTESIAN_POINT('Ctrl Pts',(-7.98526240565772,-1.11182427083077,
6.19220894827678));
#12648=CARTESIAN_POINT('Ctrl Pts',(-8.27875123560104,-1.16744491727744,
6.18020576148746));
#12649=CARTESIAN_POINT('Ctrl Pts',(-8.57224006554437,-1.22306556372412,
6.16820257469814));
#12650=CARTESIAN_POINT('Ctrl Pts',(-8.88610136059928,-1.16276985667028,
6.15619938790882));
#12651=CARTESIAN_POINT('Ctrl Pts',(-9.13808834820083,-1.00235817476356,
6.14419620111951));
#12652=CARTESIAN_POINT('Ctrl Pts',(-9.39007533580238,-0.841946492856838,
6.13219301433019));
#12653=CARTESIAN_POINT('Ctrl Pts',(-9.5775432964213,-0.583102430603032,
6.12018982754087));
#12654=CARTESIAN_POINT('Ctrl Pts',(-9.65136659729188,-0.293655596346344,
6.10818664075155));
#12655=CARTESIAN_POINT('Ctrl Pts',(-9.67581103310541,-0.197813707972621,
6.10421213506609));
#12656=CARTESIAN_POINT('Ctrl Pts',(-9.68822499999999,-0.0989100500924879,
6.10023762938064));
#12657=CARTESIAN_POINT('Ctrl Pts',(-9.688225,-7.7715611723761E-14,6.09626312369518));
#12658=CARTESIAN_POINT('Ctrl Pts',(-9.688225,-1.81177295388579E-12,6.05373687630491));
#12659=CARTESIAN_POINT('Ctrl Pts',(-9.68822499999954,-0.2987128213079,6.06574006309423));
#12660=CARTESIAN_POINT('Ctrl Pts',(-9.57054245632496,-0.59585807827315,
6.07774324988355));
#12661=CARTESIAN_POINT('Ctrl Pts',(-9.36601586214812,-0.813569405234027,
6.08974643667286));
#12662=CARTESIAN_POINT('Ctrl Pts',(-9.16148926797128,-1.03128073219491,
6.10174962346218));
#12663=CARTESIAN_POINT('Ctrl Pts',(-8.87226522412671,-1.16727314847191,
6.1137528102515));
#12664=CARTESIAN_POINT('Ctrl Pts',(-8.57413435701273,-1.18591009260201,
6.12575599704082));
#12665=CARTESIAN_POINT('Ctrl Pts',(-8.27600348989875,-1.20454703673211,
6.13775918383013));
#12666=CARTESIAN_POINT('Ctrl Pts',(-7.97209482031931,-1.10563290540032,
6.14976237061945));
#12667=CARTESIAN_POINT('Ctrl Pts',(-7.74204705371927,-0.915087963995467,
6.16176555740877));
#12668=CARTESIAN_POINT('Ctrl Pts',(-7.51199928711924,-0.724543022590617,
6.17376874419809));
#12669=CARTESIAN_POINT('Ctrl Pts',(-7.3582268807957,-0.444367128059815,
6.18577193098741));
#12670=CARTESIAN_POINT('Ctrl Pts',(-7.32102560975796,-0.147979855988595,
6.19777511777672));
#12671=CARTESIAN_POINT('Ctrl Pts',(-7.28382433872022,0.148407416082624,
6.20977830456604));
#12672=CARTESIAN_POINT('Ctrl Pts',(-7.36358464744702,0.457895344723582,
6.22178149135536));
#12673=CARTESIAN_POINT('Ctrl Pts',(-7.53940549437982,0.699383189959065,
6.23378467814468));
#12674=CARTESIAN_POINT('Ctrl Pts',(-7.71522634131261,0.940871035194547,
6.24578786493399));
#12675=CARTESIAN_POINT('Ctrl Pts',(-7.98526240565941,1.11182427083155,6.25779105172331));
#12676=CARTESIAN_POINT('Ctrl Pts',(-8.27875123560281,1.16744491727778,6.26979423851263));
#12677=CARTESIAN_POINT('Ctrl Pts',(-8.57224006554621,1.22306556372401,6.28179742530195));
#12678=CARTESIAN_POINT('Ctrl Pts',(-8.88610136060103,1.1627698566697,6.29380061209126));
#12679=CARTESIAN_POINT('Ctrl Pts',(-9.13808834820233,1.0023581747626,6.30580379888058));
#12680=CARTESIAN_POINT('Ctrl Pts',(-9.39007533580363,0.841946492855508,
6.3178069856699));
#12681=CARTESIAN_POINT('Ctrl Pts',(-9.57754329642217,0.583102430601428,
6.32981017245922));
#12682=CARTESIAN_POINT('Ctrl Pts',(-9.65136659729231,0.293655596344636,
6.34181335924854));
#12683=CARTESIAN_POINT('Ctrl Pts',(-9.67581103310571,0.197813707970833,
6.34578786493399));
#12684=CARTESIAN_POINT('Ctrl Pts',(-9.68822500000015,0.0989100500906353,
6.34976237061945));
#12685=CARTESIAN_POINT('Ctrl Pts',(-9.688225,-1.81987758196556E-12,6.35373687630491));
#12686=CARTESIAN_POINT('Origin',(-8.5,0.,1.8));
#12687=CARTESIAN_POINT('',(-9.68779459938433,-0.000383426657895316,6.69626312369518));
#12688=CARTESIAN_POINT('',(-9.688225,-1.82809323234778E-12,6.65373687630491));
#12689=CARTESIAN_POINT('',(-9.688225,-1.45515594291686E-16,1.8));
#12690=CARTESIAN_POINT('Ctrl Pts',(-9.688225,-9.39248678832882E-14,6.69626312369518));
#12691=CARTESIAN_POINT('Ctrl Pts',(-9.68822500000002,0.298712821305994,
6.68425993690586));
#12692=CARTESIAN_POINT('Ctrl Pts',(-9.57054245632591,0.595858078271433,
6.67225675011654));
#12693=CARTESIAN_POINT('Ctrl Pts',(-9.36601586214942,0.813569405232639,
6.66025356332723));
#12694=CARTESIAN_POINT('Ctrl Pts',(-9.16148926797294,1.03128073219384,6.64825037653791));
#12695=CARTESIAN_POINT('Ctrl Pts',(-8.87226522412858,1.16727314847132,6.63624718974859));
#12696=CARTESIAN_POINT('Ctrl Pts',(-8.57413435701463,1.18591009260189,6.62424400295927));
#12697=CARTESIAN_POINT('Ctrl Pts',(-8.27600348990068,1.20454703673247,6.61224081616996));
#12698=CARTESIAN_POINT('Ctrl Pts',(-7.97209482032109,1.10563290540116,6.60023762938064));
#12699=CARTESIAN_POINT('Ctrl Pts',(-7.74204705372074,0.915087963996682,
6.58823444259132));
#12700=CARTESIAN_POINT('Ctrl Pts',(-7.5119992871204,0.724543022592202,6.576231255802));
#12701=CARTESIAN_POINT('Ctrl Pts',(-7.35822688079641,0.444367128061646,
6.56422806901269));
#12702=CARTESIAN_POINT('Ctrl Pts',(-7.32102560975819,0.147979855990486,
6.55222488222337));
#12703=CARTESIAN_POINT('Ctrl Pts',(-7.28382433871998,-0.148407416080674,
6.54022169543405));
#12704=CARTESIAN_POINT('Ctrl Pts',(-7.36358464744629,-0.45789534472176,
6.52821850864473));
#12705=CARTESIAN_POINT('Ctrl Pts',(-7.5394054943787,-0.699383189957524,
6.51621532185542));
#12706=CARTESIAN_POINT('Ctrl Pts',(-7.71522634131111,-0.940871035193289,
6.5042121350661));
#12707=CARTESIAN_POINT('Ctrl Pts',(-7.98526240565763,-1.11182427083072,
6.49220894827678));
#12708=CARTESIAN_POINT('Ctrl Pts',(-8.27875123560094,-1.16744491727742,
6.48020576148746));
#12709=CARTESIAN_POINT('Ctrl Pts',(-8.57224006554425,-1.22306556372412,
6.46820257469815));
#12710=CARTESIAN_POINT('Ctrl Pts',(-8.88610136059916,-1.16276985667032,
6.45619938790883));
#12711=CARTESIAN_POINT('Ctrl Pts',(-9.13808834820072,-1.00235817476363,
6.44419620111951));
#12712=CARTESIAN_POINT('Ctrl Pts',(-9.39007533580228,-0.841946492856936,
6.43219301433019));
#12713=CARTESIAN_POINT('Ctrl Pts',(-9.57754329642123,-0.583102430603156,
6.42018982754087));
#12714=CARTESIAN_POINT('Ctrl Pts',(-9.65136659729184,-0.293655596346483,
6.40818664075156));
#12715=CARTESIAN_POINT('Ctrl Pts',(-9.6758110331054,-0.197813707972719,
6.4042121350661));
#12716=CARTESIAN_POINT('Ctrl Pts',(-9.68822499999999,-0.0989100500925409,
6.40023762938064));
#12717=CARTESIAN_POINT('Ctrl Pts',(-9.688225,-8.57092175010621E-14,6.39626312369518));
#12718=CARTESIAN_POINT('Ctrl Pts',(-9.688225,-1.81987758196556E-12,6.35373687630491));
#12719=CARTESIAN_POINT('Ctrl Pts',(-9.68822499999954,-0.298712821307902,
6.36574006309423));
#12720=CARTESIAN_POINT('Ctrl Pts',(-9.57054245632496,-0.595858078273146,
6.37774324988355));
#12721=CARTESIAN_POINT('Ctrl Pts',(-9.36601586214813,-0.813569405234021,
6.38974643667286));
#12722=CARTESIAN_POINT('Ctrl Pts',(-9.16148926797129,-1.0312807321949,6.40174962346218));
#12723=CARTESIAN_POINT('Ctrl Pts',(-8.87226522412673,-1.16727314847191,
6.4137528102515));
#12724=CARTESIAN_POINT('Ctrl Pts',(-8.57413435701275,-1.18591009260201,
6.42575599704082));
#12725=CARTESIAN_POINT('Ctrl Pts',(-8.27600348989878,-1.20454703673211,
6.43775918383013));
#12726=CARTESIAN_POINT('Ctrl Pts',(-7.97209482031935,-1.10563290540033,
6.44976237061945));
#12727=CARTESIAN_POINT('Ctrl Pts',(-7.74204705371931,-0.915087963995493,
6.46176555740877));
#12728=CARTESIAN_POINT('Ctrl Pts',(-7.51199928711927,-0.724543022590656,
6.47376874419809));
#12729=CARTESIAN_POINT('Ctrl Pts',(-7.35822688079572,-0.444367128059867,
6.4857719309874));
#12730=CARTESIAN_POINT('Ctrl Pts',(-7.32102560975797,-0.147979855988654,
6.49777511777672));
#12731=CARTESIAN_POINT('Ctrl Pts',(-7.28382433872021,0.148407416082558,
6.50977830456604));
#12732=CARTESIAN_POINT('Ctrl Pts',(-7.36358464744699,0.457895344723514,
6.52178149135536));
#12733=CARTESIAN_POINT('Ctrl Pts',(-7.53940549437977,0.699383189959003,
6.53378467814467));
#12734=CARTESIAN_POINT('Ctrl Pts',(-7.71522634131255,0.940871035194492,
6.54578786493399));
#12735=CARTESIAN_POINT('Ctrl Pts',(-7.98526240565933,1.11182427083151,6.55779105172331));
#12736=CARTESIAN_POINT('Ctrl Pts',(-8.27875123560272,1.16744491727776,6.56979423851263));
#12737=CARTESIAN_POINT('Ctrl Pts',(-8.57224006554611,1.22306556372401,6.58179742530194));
#12738=CARTESIAN_POINT('Ctrl Pts',(-8.88610136060093,1.16276985666973,6.59380061209126));
#12739=CARTESIAN_POINT('Ctrl Pts',(-9.13808834820224,1.00235817476266,6.60580379888058));
#12740=CARTESIAN_POINT('Ctrl Pts',(-9.39007533580355,0.841946492855594,
6.61780698566989));
#12741=CARTESIAN_POINT('Ctrl Pts',(-9.57754329642211,0.583102430601538,
6.62981017245921));
#12742=CARTESIAN_POINT('Ctrl Pts',(-9.65136659729228,0.293655596344759,
6.64181335924853));
#12743=CARTESIAN_POINT('Ctrl Pts',(-9.6758110331057,0.19781370797092,6.64578786493399));
#12744=CARTESIAN_POINT('Ctrl Pts',(-9.68822500000015,0.0989100500906833,
6.64976237061945));
#12745=CARTESIAN_POINT('Ctrl Pts',(-9.688225,-1.81121784237348E-12,6.65373687630491));
#12746=CARTESIAN_POINT('Origin',(-8.5,0.,1.8));
#12747=CARTESIAN_POINT('',(-9.68888225390868,-0.000138896677983098,6.99626312369518));
#12748=CARTESIAN_POINT('',(-9.688225,-1.83614234927632E-12,6.95373687630491));
#12749=CARTESIAN_POINT('',(-9.688225,-1.45515594291686E-16,1.8));
#12750=CARTESIAN_POINT('Ctrl Pts',(-9.6902066384567,-0.00041877727094708,
6.99626312369518));
#12751=CARTESIAN_POINT('Ctrl Pts',(-9.68899674651061,0.379592025804337,
6.98092963956396));
#12752=CARTESIAN_POINT('Ctrl Pts',(-9.49087722055918,0.761025012956179,
6.96559615543274));
#12753=CARTESIAN_POINT('Ctrl Pts',(-9.1791037192896,0.977577133098408,6.95026267130152));
#12754=CARTESIAN_POINT('Ctrl Pts',(-8.85566206674089,1.20223373578116,6.9343553301499));
#12755=CARTESIAN_POINT('Ctrl Pts',(-8.40990023040919,1.24943717064941,6.91844798899829));
#12756=CARTESIAN_POINT('Ctrl Pts',(-8.0451996812129,1.0993862626989,6.90254064784667));
#12757=CARTESIAN_POINT('Ctrl Pts',(-7.86284940661476,1.02436080872364,6.89458697727086));
#12758=CARTESIAN_POINT('Ctrl Pts',(-7.70076445380047,0.900021769043694,
6.88663330669505));
#12759=CARTESIAN_POINT('Ctrl Pts',(-7.5760833820586,0.745501801578665,6.87867963611924));
#12760=CARTESIAN_POINT('Ctrl Pts',(-7.45140231031673,0.590981834113632,
6.87072596554343));
#12761=CARTESIAN_POINT('Ctrl Pts',(-7.36412511964729,0.406280938863516,
6.86277229496762));
#12762=CARTESIAN_POINT('Ctrl Pts',(-7.32933043709483,0.212193918544567,
6.85481862439181));
#12763=CARTESIAN_POINT('Ctrl Pts',(-7.25974107198991,-0.175980122093319,
6.83891128324018));
#12764=CARTESIAN_POINT('Ctrl Pts',(-7.40008173935293,-0.601698663006534,
6.82300394208856));
#12765=CARTESIAN_POINT('Ctrl Pts',(-7.6880176507503,-0.870358303928216,
6.80709660093694));
#12766=CARTESIAN_POINT('Ctrl Pts',(-7.97595356214767,-1.1390179448499,6.79118925978532));
#12767=CARTESIAN_POINT('Ctrl Pts',(-8.41148471757938,-1.25061868578005,
6.7752819186337));
#12768=CARTESIAN_POINT('Ctrl Pts',(-8.79347776741406,-1.15354304866133,
6.75937457748208));
#12769=CARTESIAN_POINT('Ctrl Pts',(-9.17547081724873,-1.05646741154261,
6.74346723633046));
#12770=CARTESIAN_POINT('Ctrl Pts',(-9.50392576148636,-0.750715396374999,
6.72755989517883));
#12771=CARTESIAN_POINT('Ctrl Pts',(-9.62874639685919,-0.376957434999199,
6.71165255402721));
#12772=CARTESIAN_POINT('Ctrl Pts',(-9.66899863959755,-0.256427715359838,
6.70652274391653));
#12773=CARTESIAN_POINT('Ctrl Pts',(-9.68807417965994,-0.128825799924604,
6.70139293380585));
#12774=CARTESIAN_POINT('Ctrl Pts',(-9.68716172628878,-0.00094722793280222,
6.69626312369518));
#12775=CARTESIAN_POINT('Ctrl Pts',(-9.688225,-1.81121784237348E-12,6.65373687630491));
#12776=CARTESIAN_POINT('Ctrl Pts',(-9.68822499999954,-0.298712821307899,
6.66574006309423));
#12777=CARTESIAN_POINT('Ctrl Pts',(-9.57054245632496,-0.595858078273149,
6.67774324988355));
#12778=CARTESIAN_POINT('Ctrl Pts',(-9.36601586214812,-0.813569405234027,
6.68974643667286));
#12779=CARTESIAN_POINT('Ctrl Pts',(-9.16148926797128,-1.0312807321949,6.70174962346218));
#12780=CARTESIAN_POINT('Ctrl Pts',(-8.87226522412671,-1.16727314847191,
6.7137528102515));
#12781=CARTESIAN_POINT('Ctrl Pts',(-8.57413435701273,-1.18591009260201,
6.72575599704082));
#12782=CARTESIAN_POINT('Ctrl Pts',(-8.27600348989875,-1.20454703673211,
6.73775918383013));
#12783=CARTESIAN_POINT('Ctrl Pts',(-7.97209482031931,-1.10563290540032,
6.74976237061945));
#12784=CARTESIAN_POINT('Ctrl Pts',(-7.74204705371928,-0.915087963995467,
6.76176555740877));
#12785=CARTESIAN_POINT('Ctrl Pts',(-7.51199928711924,-0.724543022590618,
6.77376874419809));
#12786=CARTESIAN_POINT('Ctrl Pts',(-7.3582268807957,-0.444367128059816,
6.78577193098741));
#12787=CARTESIAN_POINT('Ctrl Pts',(-7.32102560975796,-0.147979855988596,
6.79777511777672));
#12788=CARTESIAN_POINT('Ctrl Pts',(-7.28382433872022,0.148407416082623,
6.80977830456604));
#12789=CARTESIAN_POINT('Ctrl Pts',(-7.36358464744702,0.457895344723582,
6.82178149135536));
#12790=CARTESIAN_POINT('Ctrl Pts',(-7.53940549437982,0.699383189959064,
6.83378467814468));
#12791=CARTESIAN_POINT('Ctrl Pts',(-7.71522634131261,0.940871035194547,
6.84578786493399));
#12792=CARTESIAN_POINT('Ctrl Pts',(-7.98526240565941,1.11182427083155,6.85779105172331));
#12793=CARTESIAN_POINT('Ctrl Pts',(-8.27875123560281,1.16744491727778,6.86979423851263));
#12794=CARTESIAN_POINT('Ctrl Pts',(-8.57224006554621,1.22306556372401,6.88179742530195));
#12795=CARTESIAN_POINT('Ctrl Pts',(-8.88610136060103,1.1627698566697,6.89380061209126));
#12796=CARTESIAN_POINT('Ctrl Pts',(-9.13808834820233,1.00235817476261,6.90580379888058));
#12797=CARTESIAN_POINT('Ctrl Pts',(-9.39007533580363,0.841946492855509,
6.9178069856699));
#12798=CARTESIAN_POINT('Ctrl Pts',(-9.57754329642217,0.583102430601429,
6.92981017245922));
#12799=CARTESIAN_POINT('Ctrl Pts',(-9.65136659729231,0.293655596344637,
6.94181335924853));
#12800=CARTESIAN_POINT('Ctrl Pts',(-9.67581103310571,0.197813707970828,
6.94578786493399));
#12801=CARTESIAN_POINT('Ctrl Pts',(-9.68822500000015,0.0989100500906246,
6.94976237061945));
#12802=CARTESIAN_POINT('Ctrl Pts',(-9.688225,-1.83614234927632E-12,6.95373687630491));
#12803=CARTESIAN_POINT('Origin',(-8.5,0.,1.8));
#12804=CARTESIAN_POINT('',(-9.688225,-1.10245146345278E-13,7.29626312369518));
#12805=CARTESIAN_POINT('',(-9.688225,-1.84441351080977E-12,7.25373687630491));
#12806=CARTESIAN_POINT('',(-9.688225,-1.45515594291686E-16,1.8));
#12807=CARTESIAN_POINT('Ctrl Pts',(-9.688225,-1.10245146345278E-13,7.29626312369518));
#12808=CARTESIAN_POINT('Ctrl Pts',(-9.68822500000003,0.298712821305983,
7.28425993690586));
#12809=CARTESIAN_POINT('Ctrl Pts',(-9.57054245632592,0.59585807827143,7.27225675011655));
#12810=CARTESIAN_POINT('Ctrl Pts',(-9.36601586214942,0.813569405232639,
7.26025356332723));
#12811=CARTESIAN_POINT('Ctrl Pts',(-9.16148926797293,1.03128073219385,7.24825037653791));
#12812=CARTESIAN_POINT('Ctrl Pts',(-8.87226522412857,1.16727314847132,7.23624718974859));
#12813=CARTESIAN_POINT('Ctrl Pts',(-8.57413435701461,1.18591009260189,7.22424400295927));
#12814=CARTESIAN_POINT('Ctrl Pts',(-8.27600348990066,1.20454703673246,7.21224081616996));
#12815=CARTESIAN_POINT('Ctrl Pts',(-7.97209482032106,1.10563290540115,7.20023762938064));
#12816=CARTESIAN_POINT('Ctrl Pts',(-7.74204705372072,0.91508796399666,7.18823444259132));
#12817=CARTESIAN_POINT('Ctrl Pts',(-7.51199928712037,0.72454302259217,7.176231255802));
#12818=CARTESIAN_POINT('Ctrl Pts',(-7.35822688079639,0.444367128061603,
7.16422806901268));
#12819=CARTESIAN_POINT('Ctrl Pts',(-7.32102560975819,0.147979855990436,
7.15222488222337));
#12820=CARTESIAN_POINT('Ctrl Pts',(-7.28382433871998,-0.148407416080732,
7.14022169543405));
#12821=CARTESIAN_POINT('Ctrl Pts',(-7.36358464744631,-0.45789534472182,
7.12821850864473));
#12822=CARTESIAN_POINT('Ctrl Pts',(-7.53940549437874,-0.699383189957579,
7.11621532185541));
#12823=CARTESIAN_POINT('Ctrl Pts',(-7.71522634131116,-0.940871035193338,
7.10421213506609));
#12824=CARTESIAN_POINT('Ctrl Pts',(-7.9852624056577,-1.11182427083076,7.09220894827678));
#12825=CARTESIAN_POINT('Ctrl Pts',(-8.27875123560102,-1.16744491727744,
7.08020576148746));
#12826=CARTESIAN_POINT('Ctrl Pts',(-8.57224006554434,-1.22306556372412,
7.06820257469814));
#12827=CARTESIAN_POINT('Ctrl Pts',(-8.88610136059926,-1.16276985667029,
7.05619938790882));
#12828=CARTESIAN_POINT('Ctrl Pts',(-9.13808834820081,-1.00235817476357,
7.04419620111951));
#12829=CARTESIAN_POINT('Ctrl Pts',(-9.39007533580236,-0.841946492856857,
7.03219301433019));
#12830=CARTESIAN_POINT('Ctrl Pts',(-9.57754329642129,-0.583102430603054,
7.02018982754087));
#12831=CARTESIAN_POINT('Ctrl Pts',(-9.65136659729187,-0.293655596346368,
7.00818664075155));
#12832=CARTESIAN_POINT('Ctrl Pts',(-9.6758110331054,-0.197813707972645,
7.0042121350661));
#12833=CARTESIAN_POINT('Ctrl Pts',(-9.68822499999999,-0.0989100500925123,
7.00023762938064));
#12834=CARTESIAN_POINT('Ctrl Pts',(-9.688225,-1.02140518265514E-13,6.99626312369518));
#12835=CARTESIAN_POINT('Ctrl Pts',(-9.688225,-1.83614234927632E-12,6.95373687630491));
#12836=CARTESIAN_POINT('Ctrl Pts',(-9.68822499999954,-0.298712821307918,
6.96574006309423));
#12837=CARTESIAN_POINT('Ctrl Pts',(-9.57054245632495,-0.595858078273161,
6.97774324988355));
#12838=CARTESIAN_POINT('Ctrl Pts',(-9.36601586214811,-0.813569405234033,
6.98974643667286));
#12839=CARTESIAN_POINT('Ctrl Pts',(-9.16148926797128,-1.03128073219491,
7.00174962346218));
#12840=CARTESIAN_POINT('Ctrl Pts',(-8.87226522412671,-1.16727314847191,
7.0137528102515));
#12841=CARTESIAN_POINT('Ctrl Pts',(-8.57413435701274,-1.18591009260201,
7.02575599704082));
#12842=CARTESIAN_POINT('Ctrl Pts',(-8.27600348989876,-1.20454703673211,
7.03775918383013));
#12843=CARTESIAN_POINT('Ctrl Pts',(-7.97209482031933,-1.10563290540032,
7.04976237061945));
#12844=CARTESIAN_POINT('Ctrl Pts',(-7.7420470537193,-0.915087963995483,
7.06176555740877));
#12845=CARTESIAN_POINT('Ctrl Pts',(-7.51199928711926,-0.724543022590642,
7.07376874419809));
#12846=CARTESIAN_POINT('Ctrl Pts',(-7.35822688079572,-0.444367128059851,
7.0857719309874));
#12847=CARTESIAN_POINT('Ctrl Pts',(-7.32102560975796,-0.147979855988638,
7.09777511777672));
#12848=CARTESIAN_POINT('Ctrl Pts',(-7.28382433872021,0.148407416082574,
7.10977830456604));
#12849=CARTESIAN_POINT('Ctrl Pts',(-7.363584647447,0.457895344723529,7.12178149135536));
#12850=CARTESIAN_POINT('Ctrl Pts',(-7.53940549437978,0.699383189959016,
7.13378467814467));
#12851=CARTESIAN_POINT('Ctrl Pts',(-7.71522634131256,0.940871035194503,
7.14578786493399));
#12852=CARTESIAN_POINT('Ctrl Pts',(-7.98526240565934,1.11182427083152,7.15779105172331));
#12853=CARTESIAN_POINT('Ctrl Pts',(-8.27875123560274,1.16744491727776,7.16979423851263));
#12854=CARTESIAN_POINT('Ctrl Pts',(-8.57224006554613,1.22306556372401,7.18179742530194));
#12855=CARTESIAN_POINT('Ctrl Pts',(-8.88610136060094,1.16276985666973,7.19380061209126));
#12856=CARTESIAN_POINT('Ctrl Pts',(-9.13808834820225,1.00235817476266,7.20580379888058));
#12857=CARTESIAN_POINT('Ctrl Pts',(-9.39007533580356,0.841946492855582,
7.2178069856699));
#12858=CARTESIAN_POINT('Ctrl Pts',(-9.57754329642211,0.583102430601523,
7.22981017245921));
#12859=CARTESIAN_POINT('Ctrl Pts',(-9.65136659729228,0.293655596344743,
7.24181335924853));
#12860=CARTESIAN_POINT('Ctrl Pts',(-9.6758110331057,0.197813707970899,7.24578786493399));
#12861=CARTESIAN_POINT('Ctrl Pts',(-9.68822500000015,0.0989100500906558,
7.24976237061945));
#12862=CARTESIAN_POINT('Ctrl Pts',(-9.688225,-1.84441351080977E-12,7.25373687630491));
#12863=CARTESIAN_POINT('Origin',(-8.5,0.,1.8));
#12864=CARTESIAN_POINT('',(-9.688225,-1.18460796727504E-13,7.59626312369518));
#12865=CARTESIAN_POINT('',(-9.688225,-1.85257365004077E-12,7.55373687630491));
#12866=CARTESIAN_POINT('',(-9.688225,-1.45515594291686E-16,1.8));
#12867=CARTESIAN_POINT('Ctrl Pts',(-9.688225,-8.47100167788994E-14,7.59626312369518));
#12868=CARTESIAN_POINT('Ctrl Pts',(-9.68822500000002,0.298712821306009,
7.58425993690586));
#12869=CARTESIAN_POINT('Ctrl Pts',(-9.5705424563259,0.595858078271453,7.57225675011655));
#12870=CARTESIAN_POINT('Ctrl Pts',(-9.36601586214941,0.813569405232658,
7.56025356332723));
#12871=CARTESIAN_POINT('Ctrl Pts',(-9.16148926797291,1.03128073219386,7.54825037653791));
#12872=CARTESIAN_POINT('Ctrl Pts',(-8.87226522412855,1.16727314847133,7.53624718974859));
#12873=CARTESIAN_POINT('Ctrl Pts',(-8.57413435701459,1.18591009260189,7.52424400295927));
#12874=CARTESIAN_POINT('Ctrl Pts',(-8.27600348990063,1.20454703673246,7.51224081616995));
#12875=CARTESIAN_POINT('Ctrl Pts',(-7.97209482032103,1.10563290540114,7.50023762938064));
#12876=CARTESIAN_POINT('Ctrl Pts',(-7.7420470537207,0.915087963996644,7.48823444259132));
#12877=CARTESIAN_POINT('Ctrl Pts',(-7.51199928712036,0.724543022592149,
7.476231255802));
#12878=CARTESIAN_POINT('Ctrl Pts',(-7.35822688079639,0.444367128061578,
7.46422806901268));
#12879=CARTESIAN_POINT('Ctrl Pts',(-7.32102560975819,0.14797985599041,7.45222488222337));
#12880=CARTESIAN_POINT('Ctrl Pts',(-7.28382433871999,-0.148407416080758,
7.44022169543405));
#12881=CARTESIAN_POINT('Ctrl Pts',(-7.36358464744632,-0.457895344721845,
7.42821850864473));
#12882=CARTESIAN_POINT('Ctrl Pts',(-7.53940549437875,-0.6993831899576,7.41621532185541));
#12883=CARTESIAN_POINT('Ctrl Pts',(-7.71522634131118,-0.940871035193355,
7.40421213506609));
#12884=CARTESIAN_POINT('Ctrl Pts',(-7.98526240565772,-1.11182427083077,
7.39220894827678));
#12885=CARTESIAN_POINT('Ctrl Pts',(-8.27875123560105,-1.16744491727744,
7.38020576148746));
#12886=CARTESIAN_POINT('Ctrl Pts',(-8.57224006554437,-1.22306556372412,
7.36820257469814));
#12887=CARTESIAN_POINT('Ctrl Pts',(-8.88610136059928,-1.16276985667028,
7.35619938790882));
#12888=CARTESIAN_POINT('Ctrl Pts',(-9.13808834820083,-1.00235817476356,
7.34419620111951));
#12889=CARTESIAN_POINT('Ctrl Pts',(-9.39007533580238,-0.841946492856837,
7.33219301433019));
#12890=CARTESIAN_POINT('Ctrl Pts',(-9.5775432964213,-0.583102430603031,
7.32018982754087));
#12891=CARTESIAN_POINT('Ctrl Pts',(-9.65136659729188,-0.293655596346343,
7.30818664075155));
#12892=CARTESIAN_POINT('Ctrl Pts',(-9.6758110331054,-0.19781370797263,7.30421213506609));
#12893=CARTESIAN_POINT('Ctrl Pts',(-9.68822499999999,-0.0989100500925091,
7.30023762938064));
#12894=CARTESIAN_POINT('Ctrl Pts',(-9.688225,-1.10245146345278E-13,7.29626312369518));
#12895=CARTESIAN_POINT('Ctrl Pts',(-9.688225,-1.84441351080977E-12,7.25373687630491));
#12896=CARTESIAN_POINT('Ctrl Pts',(-9.68822499999954,-0.298712821307943,
7.26574006309423));
#12897=CARTESIAN_POINT('Ctrl Pts',(-9.57054245632493,-0.595858078273201,
7.27774324988355));
#12898=CARTESIAN_POINT('Ctrl Pts',(-9.36601586214807,-0.813569405234076,
7.28974643667287));
#12899=CARTESIAN_POINT('Ctrl Pts',(-9.16148926797122,-1.03128073219495,
7.30174962346219));
#12900=CARTESIAN_POINT('Ctrl Pts',(-8.87226522412662,-1.16727314847194,
7.3137528102515));
#12901=CARTESIAN_POINT('Ctrl Pts',(-8.57413435701263,-1.18591009260202,
7.32575599704082));
#12902=CARTESIAN_POINT('Ctrl Pts',(-8.27600348989864,-1.20454703673209,
7.33775918383014));
#12903=CARTESIAN_POINT('Ctrl Pts',(-7.9720948203192,-1.10563290540026,7.34976237061946));
#12904=CARTESIAN_POINT('Ctrl Pts',(-7.74204705371917,-0.915087963995381,
7.36176555740878));
#12905=CARTESIAN_POINT('Ctrl Pts',(-7.51199928711915,-0.724543022590499,
7.37376874419809));
#12906=CARTESIAN_POINT('Ctrl Pts',(-7.35822688079564,-0.444367128059665,
7.38577193098741));
#12907=CARTESIAN_POINT('Ctrl Pts',(-7.32102560975794,-0.147979855988429,
7.39777511777673));
#12908=CARTESIAN_POINT('Ctrl Pts',(-7.28382433872024,0.148407416082807,
7.40977830456605));
#12909=CARTESIAN_POINT('Ctrl Pts',(-7.36358464744709,0.457895344723766,
7.42178149135537));
#12910=CARTESIAN_POINT('Ctrl Pts',(-7.53940549437994,0.699383189959228,
7.43378467814468));
#12911=CARTESIAN_POINT('Ctrl Pts',(-7.71522634131278,0.94087103519469,7.445787864934));
#12912=CARTESIAN_POINT('Ctrl Pts',(-7.98526240565962,1.11182427083165,7.45779105172332));
#12913=CARTESIAN_POINT('Ctrl Pts',(-8.27875123560304,1.16744491727782,7.46979423851264));
#12914=CARTESIAN_POINT('Ctrl Pts',(-8.57224006554646,1.22306556372399,7.48179742530196));
#12915=CARTESIAN_POINT('Ctrl Pts',(-8.88610136060128,1.16276985666962,7.49380061209127));
#12916=CARTESIAN_POINT('Ctrl Pts',(-9.13808834820256,1.00235817476246,7.50580379888059));
#12917=CARTESIAN_POINT('Ctrl Pts',(-9.39007533580383,0.841946492855301,
7.51780698566991));
#12918=CARTESIAN_POINT('Ctrl Pts',(-9.57754329642231,0.583102430601164,
7.52981017245923));
#12919=CARTESIAN_POINT('Ctrl Pts',(-9.65136659729239,0.293655596344343,
7.54181335924855));
#12920=CARTESIAN_POINT('Ctrl Pts',(-9.67581103310574,0.197813707970626,
7.545787864934));
#12921=CARTESIAN_POINT('Ctrl Pts',(-9.68822500000015,0.0989100500905238,
7.54976237061946));
#12922=CARTESIAN_POINT('Ctrl Pts',(-9.688225,-1.83564274891523E-12,7.55373687630491));
#12923=CARTESIAN_POINT('Origin',(-8.5,0.,1.8));
#12924=CARTESIAN_POINT('',(-9.688225,-1.26565424807268E-13,7.89626312369518));
#12925=CARTESIAN_POINT('',(-9.688225,-1.86067827812053E-12,7.85373687630491));
#12926=CARTESIAN_POINT('',(-9.688225,-1.45515594291686E-16,1.8));
#12927=CARTESIAN_POINT('Ctrl Pts',(-9.688225,-1.26565424807268E-13,7.89626312369518));
#12928=CARTESIAN_POINT('Ctrl Pts',(-9.68822500000003,0.298712821305967,
7.88425993690586));
#12929=CARTESIAN_POINT('Ctrl Pts',(-9.57054245632592,0.595858078271415,
7.87225675011655));
#12930=CARTESIAN_POINT('Ctrl Pts',(-9.36601586214944,0.813569405232627,
7.86025356332723));
#12931=CARTESIAN_POINT('Ctrl Pts',(-9.16148926797295,1.03128073219384,7.84825037653791));
#12932=CARTESIAN_POINT('Ctrl Pts',(-8.87226522412859,1.16727314847132,7.83624718974859));
#12933=CARTESIAN_POINT('Ctrl Pts',(-8.57413435701463,1.18591009260189,7.82424400295927));
#12934=CARTESIAN_POINT('Ctrl Pts',(-8.27600348990067,1.20454703673247,7.81224081616996));
#12935=CARTESIAN_POINT('Ctrl Pts',(-7.97209482032107,1.10563290540116,7.80023762938064));
#12936=CARTESIAN_POINT('Ctrl Pts',(-7.74204705372073,0.915087963996671,
7.78823444259132));
#12937=CARTESIAN_POINT('Ctrl Pts',(-7.51199928712038,0.724543022592183,
7.776231255802));
#12938=CARTESIAN_POINT('Ctrl Pts',(-7.3582268807964,0.444367128061618,7.76422806901269));
#12939=CARTESIAN_POINT('Ctrl Pts',(-7.32102560975819,0.147979855990452,
7.75222488222337));
#12940=CARTESIAN_POINT('Ctrl Pts',(-7.28382433871998,-0.148407416080715,
7.74022169543405));
#12941=CARTESIAN_POINT('Ctrl Pts',(-7.3635846474463,-0.457895344721805,
7.72821850864473));
#12942=CARTESIAN_POINT('Ctrl Pts',(-7.53940549437873,-0.699383189957566,
7.71621532185541));
#12943=CARTESIAN_POINT('Ctrl Pts',(-7.71522634131115,-0.940871035193328,
7.7042121350661));
#12944=CARTESIAN_POINT('Ctrl Pts',(-7.98526240565768,-1.11182427083075,
7.69220894827678));
#12945=CARTESIAN_POINT('Ctrl Pts',(-8.27875123560101,-1.16744491727744,
7.68020576148746));
#12946=CARTESIAN_POINT('Ctrl Pts',(-8.57224006554432,-1.22306556372412,
7.66820257469814));
#12947=CARTESIAN_POINT('Ctrl Pts',(-8.88610136059924,-1.1627698566703,7.65619938790883));
#12948=CARTESIAN_POINT('Ctrl Pts',(-9.1380883482008,-1.00235817476358,7.64419620111951));
#12949=CARTESIAN_POINT('Ctrl Pts',(-9.39007533580235,-0.841946492856869,
7.63219301433019));
#12950=CARTESIAN_POINT('Ctrl Pts',(-9.57754329642128,-0.583102430603069,
7.62018982754087));
#12951=CARTESIAN_POINT('Ctrl Pts',(-9.65136659729187,-0.293655596346383,
7.60818664075155));
#12952=CARTESIAN_POINT('Ctrl Pts',(-9.6758110331054,-0.19781370797265,7.6042121350661));
#12953=CARTESIAN_POINT('Ctrl Pts',(-9.68822499999999,-0.0989100500925061,
7.60023762938064));
#12954=CARTESIAN_POINT('Ctrl Pts',(-9.688225,-8.47100167788994E-14,7.59626312369518));
#12955=CARTESIAN_POINT('Ctrl Pts',(-9.688225,-1.83564274891523E-12,7.55373687630491));
#12956=CARTESIAN_POINT('Ctrl Pts',(-9.68822499999954,-0.298712821307918,
7.56574006309423));
#12957=CARTESIAN_POINT('Ctrl Pts',(-9.57054245632495,-0.59585807827316,
7.57774324988355));
#12958=CARTESIAN_POINT('Ctrl Pts',(-9.36601586214812,-0.813569405234033,
7.58974643667286));
#12959=CARTESIAN_POINT('Ctrl Pts',(-9.16148926797128,-1.0312807321949,7.60174962346218));
#12960=CARTESIAN_POINT('Ctrl Pts',(-8.87226522412671,-1.16727314847191,
7.6137528102515));
#12961=CARTESIAN_POINT('Ctrl Pts',(-8.57413435701274,-1.18591009260201,
7.62575599704082));
#12962=CARTESIAN_POINT('Ctrl Pts',(-8.27600348989876,-1.20454703673211,
7.63775918383013));
#12963=CARTESIAN_POINT('Ctrl Pts',(-7.97209482031933,-1.10563290540032,
7.64976237061945));
#12964=CARTESIAN_POINT('Ctrl Pts',(-7.7420470537193,-0.915087963995484,
7.66176555740877));
#12965=CARTESIAN_POINT('Ctrl Pts',(-7.51199928711926,-0.724543022590643,
7.67376874419809));
#12966=CARTESIAN_POINT('Ctrl Pts',(-7.35822688079572,-0.444367128059851,
7.6857719309874));
#12967=CARTESIAN_POINT('Ctrl Pts',(-7.32102560975796,-0.147979855988639,
7.69777511777672));
#12968=CARTESIAN_POINT('Ctrl Pts',(-7.28382433872021,0.148407416082574,
7.70977830456604));
#12969=CARTESIAN_POINT('Ctrl Pts',(-7.363584647447,0.457895344723529,7.72178149135536));
#12970=CARTESIAN_POINT('Ctrl Pts',(-7.53940549437978,0.699383189959016,
7.73378467814467));
#12971=CARTESIAN_POINT('Ctrl Pts',(-7.71522634131256,0.940871035194503,
7.74578786493399));
#12972=CARTESIAN_POINT('Ctrl Pts',(-7.98526240565934,1.11182427083152,7.75779105172331));
#12973=CARTESIAN_POINT('Ctrl Pts',(-8.27875123560273,1.16744491727776,7.76979423851263));
#12974=CARTESIAN_POINT('Ctrl Pts',(-8.57224006554613,1.22306556372401,7.78179742530194));
#12975=CARTESIAN_POINT('Ctrl Pts',(-8.88610136060094,1.16276985666973,7.79380061209126));
#12976=CARTESIAN_POINT('Ctrl Pts',(-9.13808834820225,1.00235817476266,7.80580379888058));
#12977=CARTESIAN_POINT('Ctrl Pts',(-9.39007533580356,0.841946492855582,
7.8178069856699));
#12978=CARTESIAN_POINT('Ctrl Pts',(-9.57754329642211,0.583102430601523,
7.82981017245921));
#12979=CARTESIAN_POINT('Ctrl Pts',(-9.65136659729228,0.293655596344744,
7.84181335924853));
#12980=CARTESIAN_POINT('Ctrl Pts',(-9.67581103310571,0.197813707970894,
7.84578786493399));
#12981=CARTESIAN_POINT('Ctrl Pts',(-9.68822500000015,0.0989100500906451,
7.84976237061945));
#12982=CARTESIAN_POINT('Ctrl Pts',(-9.688225,-1.86067827812053E-12,7.85373687630491));
#12983=CARTESIAN_POINT('Origin',(-8.5,0.,1.8));
#12984=CARTESIAN_POINT('',(-9.68879783790665,0.000205673080331772,8.19626312369518));
#12985=CARTESIAN_POINT('',(-9.6886956555678,0.00043025090496092,8.15373687630491));
#12986=CARTESIAN_POINT('',(-9.688225,-1.45515594291686E-16,1.8));
#12987=CARTESIAN_POINT('Ctrl Pts',(-9.688225,-6.7168492989822E-14,8.19626312369518));
#12988=CARTESIAN_POINT('Ctrl Pts',(-9.68822500000002,0.298712821306026,
8.18425993690586));
#12989=CARTESIAN_POINT('Ctrl Pts',(-9.57054245632589,0.595858078271468,
8.17225675011654));
#12990=CARTESIAN_POINT('Ctrl Pts',(-9.36601586214939,0.813569405232671,
8.16025356332723));
#12991=CARTESIAN_POINT('Ctrl Pts',(-9.16148926797289,1.03128073219387,8.14825037653791));
#12992=CARTESIAN_POINT('Ctrl Pts',(-8.87226522412853,1.16727314847133,8.13624718974859));
#12993=CARTESIAN_POINT('Ctrl Pts',(-8.57413435701457,1.1859100926019,8.12424400295927));
#12994=CARTESIAN_POINT('Ctrl Pts',(-8.27600348990061,1.20454703673246,8.11224081616995));
#12995=CARTESIAN_POINT('Ctrl Pts',(-7.97209482032102,1.10563290540113,8.10023762938064));
#12996=CARTESIAN_POINT('Ctrl Pts',(-7.74204705372068,0.915087963996633,
8.08823444259132));
#12997=CARTESIAN_POINT('Ctrl Pts',(-7.51199928712035,0.724543022592134,
8.076231255802));
#12998=CARTESIAN_POINT('Ctrl Pts',(-7.35822688079638,0.444367128061561,
8.06422806901268));
#12999=CARTESIAN_POINT('Ctrl Pts',(-7.32102560975818,0.147979855990393,
8.05222488222337));
#13000=CARTESIAN_POINT('Ctrl Pts',(-7.28382433871999,-0.148407416080776,
8.04022169543405));
#13001=CARTESIAN_POINT('Ctrl Pts',(-7.36358464744632,-0.457895344721862,
8.02821850864473));
#13002=CARTESIAN_POINT('Ctrl Pts',(-7.53940549437876,-0.699383189957614,
8.01621532185541));
#13003=CARTESIAN_POINT('Ctrl Pts',(-7.7152263413112,-0.940871035193367,
8.00421213506609));
#13004=CARTESIAN_POINT('Ctrl Pts',(-7.98526240565774,-1.11182427083078,
7.99220894827678));
#13005=CARTESIAN_POINT('Ctrl Pts',(-8.27875123560106,-1.16744491727745,
7.98020576148746));
#13006=CARTESIAN_POINT('Ctrl Pts',(-8.57224006554439,-1.22306556372412,
7.96820257469814));
#13007=CARTESIAN_POINT('Ctrl Pts',(-8.8861013605993,-1.16276985667028,7.95619938790882));
#13008=CARTESIAN_POINT('Ctrl Pts',(-9.13808834820085,-1.00235817476355,
7.9441962011195));
#13009=CARTESIAN_POINT('Ctrl Pts',(-9.39007533580239,-0.841946492856824,
7.93219301433019));
#13010=CARTESIAN_POINT('Ctrl Pts',(-9.57754329642131,-0.583102430603015,
7.92018982754087));
#13011=CARTESIAN_POINT('Ctrl Pts',(-9.65136659729188,-0.293655596346326,
7.90818664075155));
#13012=CARTESIAN_POINT('Ctrl Pts',(-9.67581103310541,-0.197813707972624,
7.90421213506609));
#13013=CARTESIAN_POINT('Ctrl Pts',(-9.68822499999999,-0.0989100500925142,
7.90023762938064));
#13014=CARTESIAN_POINT('Ctrl Pts',(-9.688225,-1.26565424807268E-13,7.89626312369518));
#13015=CARTESIAN_POINT('Ctrl Pts',(-9.688225,-1.86067827812053E-12,7.85373687630491));
#13016=CARTESIAN_POINT('Ctrl Pts',(-9.68822499999953,-0.298712821307954,
7.86574006309423));
#13017=CARTESIAN_POINT('Ctrl Pts',(-9.57054245632493,-0.595858078273205,
7.87774324988355));
#13018=CARTESIAN_POINT('Ctrl Pts',(-9.36601586214807,-0.813569405234075,
7.88974643667287));
#13019=CARTESIAN_POINT('Ctrl Pts',(-9.16148926797122,-1.03128073219495,
7.90174962346219));
#13020=CARTESIAN_POINT('Ctrl Pts',(-8.87226522412662,-1.16727314847194,
7.9137528102515));
#13021=CARTESIAN_POINT('Ctrl Pts',(-8.57413435701263,-1.18591009260202,
7.92575599704082));
#13022=CARTESIAN_POINT('Ctrl Pts',(-8.27600348989864,-1.20454703673209,
7.93775918383014));
#13023=CARTESIAN_POINT('Ctrl Pts',(-7.97209482031921,-1.10563290540027,
7.94976237061946));
#13024=CARTESIAN_POINT('Ctrl Pts',(-7.74204705371919,-0.915087963995392,
7.96176555740877));
#13025=CARTESIAN_POINT('Ctrl Pts',(-7.51199928711916,-0.724543022590517,
7.97376874419809));
#13026=CARTESIAN_POINT('Ctrl Pts',(-7.35822688079565,-0.444367128059693,
7.98577193098741));
#13027=CARTESIAN_POINT('Ctrl Pts',(-7.32102560975794,-0.147979855988463,
7.99777511777673));
#13028=CARTESIAN_POINT('Ctrl Pts',(-7.28382433872023,0.148407416082766,
8.00977830456605));
#13029=CARTESIAN_POINT('Ctrl Pts',(-7.36358464744707,0.457895344723721,
8.02178149135536));
#13030=CARTESIAN_POINT('Ctrl Pts',(-7.53940549437991,0.699383189959186,
8.03378467814468));
#13031=CARTESIAN_POINT('Ctrl Pts',(-7.71522634131274,0.940871035194651,
8.045787864934));
#13032=CARTESIAN_POINT('Ctrl Pts',(-7.98526240565956,1.11182427083162,8.05779105172332));
#13033=CARTESIAN_POINT('Ctrl Pts',(-8.27875123560298,1.16744491727781,8.06979423851264));
#13034=CARTESIAN_POINT('Ctrl Pts',(-8.57224006554639,1.223065563724,8.08179742530195));
#13035=CARTESIAN_POINT('Ctrl Pts',(-8.8861013606012,1.16276985666964,8.09380061209127));
#13036=CARTESIAN_POINT('Ctrl Pts',(-9.13808834820249,1.00235817476251,8.10580379888059));
#13037=CARTESIAN_POINT('Ctrl Pts',(-9.39007533580377,0.841946492855368,
8.11780698566991));
#13038=CARTESIAN_POINT('Ctrl Pts',(-9.57754329642226,0.583102430601251,
8.12981017245922));
#13039=CARTESIAN_POINT('Ctrl Pts',(-9.65136659729236,0.293655596344441,
8.14181335924854));
#13040=CARTESIAN_POINT('Ctrl Pts',(-9.67581103310573,0.197813707970689,
8.145787864934));
#13041=CARTESIAN_POINT('Ctrl Pts',(-9.68822500000015,0.0989100500905469,
8.14976237061946));
#13042=CARTESIAN_POINT('Ctrl Pts',(-9.688225,-1.85196302737722E-12,8.15373687630491));
#13043=CARTESIAN_POINT('Origin',(-8.5,0.,1.8));
#13044=CARTESIAN_POINT('',(-9.68736610752,0.000385205738155315,8.49626312369518));
#13045=CARTESIAN_POINT('',(-9.68747447047123,0.000180197558070845,8.45373687630491));
#13046=CARTESIAN_POINT('',(-9.688225,-1.45515594291686E-16,1.8));
#13047=CARTESIAN_POINT('Ctrl Pts',(-9.68638374935818,0.000825784751013359,
8.49626312369518));
#13048=CARTESIAN_POINT('Ctrl Pts',(-9.68732027411901,0.157930601934615,
8.48996455641583));
#13049=CARTESIAN_POINT('Ctrl Pts',(-9.65847850514943,0.314731334995638,
8.48366598913647));
#13050=CARTESIAN_POINT('Ctrl Pts',(-9.598408411445,0.458626072499957,8.47736742185712));
#13051=CARTESIAN_POINT('Ctrl Pts',(-9.44669843817874,0.822039302506726,
8.4614600807055));
#13052=CARTESIAN_POINT('Ctrl Pts',(-9.09580176716099,1.10313295059665,8.44555273955388));
#13053=CARTESIAN_POINT('Ctrl Pts',(-8.70773403538356,1.17202275388512,8.42964539840227));
#13054=CARTESIAN_POINT('Ctrl Pts',(-8.31966630360613,1.2409125571736,8.41373805725065));
#13055=CARTESIAN_POINT('Ctrl Pts',(-7.89442751106905,1.09759851566063,8.39783071609902));
#13056=CARTESIAN_POINT('Ctrl Pts',(-7.62673268623578,0.808436475509857,
8.3819233749474));
#13057=CARTESIAN_POINT('Ctrl Pts',(-7.3590378614025,0.519274435359075,8.36601603379578));
#13058=CARTESIAN_POINT('Ctrl Pts',(-7.24888700427306,0.0842643965704531,
8.35010869264415));
#13059=CARTESIAN_POINT('Ctrl Pts',(-7.34744850505387,-0.297347972212119,
8.33420135149253));
#13060=CARTESIAN_POINT('Ctrl Pts',(-7.44601000583468,-0.67896034099468,
8.31829401034092));
#13061=CARTESIAN_POINT('Ctrl Pts',(-7.75328386452571,-1.00717503977121,
8.3023866691893));
#13062=CARTESIAN_POINT('Ctrl Pts',(-8.12729821016773,-1.13045667257339,
8.28647932803768));
#13063=CARTESIAN_POINT('Ctrl Pts',(-8.50131255580976,-1.25373830537556,
8.27057198688606));
#13064=CARTESIAN_POINT('Ctrl Pts',(-8.94206738840278,-1.17208687220337,
8.25466464573443));
#13065=CARTESIAN_POINT('Ctrl Pts',(-9.24895983130622,-0.924420172686451,
8.23875730458281));
#13066=CARTESIAN_POINT('Ctrl Pts',(-9.40240605275795,-0.800586822927992,
8.230803634007));
#13067=CARTESIAN_POINT('Ctrl Pts',(-9.52238667678728,-0.635249656583355,
8.22284996343119));
#13068=CARTESIAN_POINT('Ctrl Pts',(-9.5979190957647,-0.4516287327225,8.21489629285538));
#13069=CARTESIAN_POINT('Ctrl Pts',(-9.65690269444705,-0.308238344471755,
8.20868523646865));
#13070=CARTESIAN_POINT('Ctrl Pts',(-9.68878125811642,-0.153698307161689,
8.20247418008191));
#13071=CARTESIAN_POINT('Ctrl Pts',(-9.6894905109208,0.000454372041894774,
8.19626312369518));
#13072=CARTESIAN_POINT('Ctrl Pts',(-9.68916921325107,0.000863154794381365,
8.15373687630491));
#13073=CARTESIAN_POINT('Ctrl Pts',(-9.68644568297345,-0.338450824757492,
8.16740829852045));
#13074=CARTESIAN_POINT('Ctrl Pts',(-9.53412983057639,-0.679944095139565,
8.181079720736));
#13075=CARTESIAN_POINT('Ctrl Pts',(-9.27761323455168,-0.901170584590548,
8.19475114295154));
#13076=CARTESIAN_POINT('Ctrl Pts',(-8.97914414043077,-1.15857798405419,
8.21065848410316));
#13077=CARTESIAN_POINT('Ctrl Pts',(-8.53960376307625,-1.25316323344806,
8.22656582525477));
#13078=CARTESIAN_POINT('Ctrl Pts',(-8.16201220914371,-1.14131641797617,
8.24247316640639));
#13079=CARTESIAN_POINT('Ctrl Pts',(-7.78442065521116,-1.02946960250427,
8.25838050755802));
#13080=CARTESIAN_POINT('Ctrl Pts',(-7.46877792470057,-0.711190722166612,
8.27428784870964));
#13081=CARTESIAN_POINT('Ctrl Pts',(-7.35774362943076,-0.332782013447075,
8.29019518986126));
#13082=CARTESIAN_POINT('Ctrl Pts',(-7.30222648179586,-0.143577659087295,
8.29814886043707));
#13083=CARTESIAN_POINT('Ctrl Pts',(-7.29786144297115,0.060659152367949,
8.30610253101288));
#13084=CARTESIAN_POINT('Ctrl Pts',(-7.3404400790801,0.254589164854932,8.31405620158869));
#13085=CARTESIAN_POINT('Ctrl Pts',(-7.38301871518904,0.448519177341904,
8.3220098721645));
#13086=CARTESIAN_POINT('Ctrl Pts',(-7.47254102623163,0.632142390860607,
8.32996354274031));
#13087=CARTESIAN_POINT('Ctrl Pts',(-7.60221326400362,0.780687172463381,
8.33791721331612));
#13088=CARTESIAN_POINT('Ctrl Pts',(-7.86155773954761,1.07777673566892,8.35382455446774));
#13089=CARTESIAN_POINT('Ctrl Pts',(-8.28150192200923,1.23455257121074,8.36973189561937));
#13090=CARTESIAN_POINT('Ctrl Pts',(-8.67121870081464,1.17793169122883,8.38563923677099));
#13091=CARTESIAN_POINT('Ctrl Pts',(-9.06093547962008,1.12131081124692,8.40154657792261));
#13092=CARTESIAN_POINT('Ctrl Pts',(-9.42042485476932,0.851293215741264,
8.41745391907422));
#13093=CARTESIAN_POINT('Ctrl Pts',(-9.58360884738056,0.492526781972071,
8.43336126022584));
#13094=CARTESIAN_POINT('Ctrl Pts',(-9.65328264037972,0.339346204382988,
8.4401531322522));
#13095=CARTESIAN_POINT('Ctrl Pts',(-9.68717019866577,0.169986820509775,
8.44694500427855));
#13096=CARTESIAN_POINT('Ctrl Pts',(-9.68650724062112,0.000412423542754418,
8.45373687630491));
#13097=CARTESIAN_POINT('Origin',(-8.5,0.,1.8));
#13098=CARTESIAN_POINT('',(-9.688225,-4.9737991503207E-14,8.79626312369518));
#13099=CARTESIAN_POINT('',(-9.688225,-1.80067072363954E-12,8.75373687630491));
#13100=CARTESIAN_POINT('',(-9.688225,-1.45515594291686E-16,1.8));
#13101=CARTESIAN_POINT('Ctrl Pts',(-9.688225,-1.58761892521397E-14,8.79626312369518));
#13102=CARTESIAN_POINT('Ctrl Pts',(-9.688225,0.298712821306078,8.78425993690586));
#13103=CARTESIAN_POINT('Ctrl Pts',(-9.57054245632587,0.595858078271514,
8.77225675011654));
#13104=CARTESIAN_POINT('Ctrl Pts',(-9.36601586214936,0.813569405232708,
8.76025356332722));
#13105=CARTESIAN_POINT('Ctrl Pts',(-9.16148926797285,1.0312807321939,8.74825037653791));
#13106=CARTESIAN_POINT('Ctrl Pts',(-8.87226522412848,1.16727314847135,8.73624718974859));
#13107=CARTESIAN_POINT('Ctrl Pts',(-8.57413435701452,1.1859100926019,8.72424400295927));
#13108=CARTESIAN_POINT('Ctrl Pts',(-8.27600348990056,1.20454703673245,8.71224081616995));
#13109=CARTESIAN_POINT('Ctrl Pts',(-7.97209482032097,1.10563290540111,8.70023762938063));
#13110=CARTESIAN_POINT('Ctrl Pts',(-7.74204705372064,0.9150879639966,8.68823444259132));
#13111=CARTESIAN_POINT('Ctrl Pts',(-7.51199928712032,0.724543022592091,
8.676231255802));
#13112=CARTESIAN_POINT('Ctrl Pts',(-7.35822688079636,0.444367128061512,
8.66422806901268));
#13113=CARTESIAN_POINT('Ctrl Pts',(-7.32102560975818,0.147979855990342,
8.65222488222336));
#13114=CARTESIAN_POINT('Ctrl Pts',(-7.28382433871999,-0.148407416080828,
8.64022169543404));
#13115=CARTESIAN_POINT('Ctrl Pts',(-7.36358464744634,-0.45789534472191,
8.62821850864473));
#13116=CARTESIAN_POINT('Ctrl Pts',(-7.53940549437879,-0.699383189957656,
8.61621532185541));
#13117=CARTESIAN_POINT('Ctrl Pts',(-7.71522634131124,-0.940871035193401,
8.60421213506609));
#13118=CARTESIAN_POINT('Ctrl Pts',(-7.98526240565779,-1.1118242708308,8.59220894827677));
#13119=CARTESIAN_POINT('Ctrl Pts',(-8.27875123560111,-1.16744491727746,
8.58020576148746));
#13120=CARTESIAN_POINT('Ctrl Pts',(-8.57224006554444,-1.22306556372411,
8.56820257469814));
#13121=CARTESIAN_POINT('Ctrl Pts',(-8.88610136059935,-1.16276985667026,
8.55619938790882));
#13122=CARTESIAN_POINT('Ctrl Pts',(-9.13808834820089,-1.00235817476352,
8.5441962011195));
#13123=CARTESIAN_POINT('Ctrl Pts',(-9.39007533580243,-0.841946492856786,
8.53219301433018));
#13124=CARTESIAN_POINT('Ctrl Pts',(-9.57754329642134,-0.583102430602969,
8.52018982754087));
#13125=CARTESIAN_POINT('Ctrl Pts',(-9.65136659729189,-0.293655596346276,
8.50818664075155));
#13126=CARTESIAN_POINT('Ctrl Pts',(-9.67581103310542,-0.197813707972562,
8.50421213506609));
#13127=CARTESIAN_POINT('Ctrl Pts',(-9.688225,-0.0989100500924404,8.50023762938064));
#13128=CARTESIAN_POINT('Ctrl Pts',(-9.688225,-4.15223411209809E-14,8.49626312369518));
#13129=CARTESIAN_POINT('Ctrl Pts',(-9.688225,-1.82637238665961E-12,8.45373687630491));
#13130=CARTESIAN_POINT('Ctrl Pts',(-9.68822499999954,-0.298712821307931,
8.46574006309423));
#13131=CARTESIAN_POINT('Ctrl Pts',(-9.57054245632493,-0.595858078273196,
8.47774324988355));
#13132=CARTESIAN_POINT('Ctrl Pts',(-9.36601586214807,-0.813569405234075,
8.48974643667287));
#13133=CARTESIAN_POINT('Ctrl Pts',(-9.16148926797121,-1.03128073219495,
8.50174962346219));
#13134=CARTESIAN_POINT('Ctrl Pts',(-8.87226522412661,-1.16727314847195,
8.5137528102515));
#13135=CARTESIAN_POINT('Ctrl Pts',(-8.57413435701261,-1.18591009260202,
8.52575599704082));
#13136=CARTESIAN_POINT('Ctrl Pts',(-8.27600348989861,-1.20454703673209,
8.53775918383014));
#13137=CARTESIAN_POINT('Ctrl Pts',(-7.97209482031917,-1.10563290540025,
8.54976237061946));
#13138=CARTESIAN_POINT('Ctrl Pts',(-7.74204705371915,-0.91508796399536,
8.56176555740878));
#13139=CARTESIAN_POINT('Ctrl Pts',(-7.51199928711912,-0.724543022590468,
8.57376874419809));
#13140=CARTESIAN_POINT('Ctrl Pts',(-7.35822688079562,-0.444367128059623,
8.58577193098741));
#13141=CARTESIAN_POINT('Ctrl Pts',(-7.32102560975793,-0.14797985598838,
8.59777511777673));
#13142=CARTESIAN_POINT('Ctrl Pts',(-7.28382433872024,0.148407416082863,
8.60977830456605));
#13143=CARTESIAN_POINT('Ctrl Pts',(-7.36358464744711,0.457895344723825,
8.62178149135537));
#13144=CARTESIAN_POINT('Ctrl Pts',(-7.53940549437997,0.699383189959281,
8.63378467814469));
#13145=CARTESIAN_POINT('Ctrl Pts',(-7.71522634131284,0.940871035194738,
8.64578786493401));
#13146=CARTESIAN_POINT('Ctrl Pts',(-7.98526240565969,1.11182427083168,8.65779105172332));
#13147=CARTESIAN_POINT('Ctrl Pts',(-8.27875123560312,1.16744491727784,8.66979423851264));
#13148=CARTESIAN_POINT('Ctrl Pts',(-8.57224006554655,1.22306556372399,8.68179742530196));
#13149=CARTESIAN_POINT('Ctrl Pts',(-8.88610136060138,1.16276985666959,8.69380061209128));
#13150=CARTESIAN_POINT('Ctrl Pts',(-9.13808834820264,1.00235817476241,8.7058037988806));
#13151=CARTESIAN_POINT('Ctrl Pts',(-9.39007533580391,0.841946492855223,
8.71780698566991));
#13152=CARTESIAN_POINT('Ctrl Pts',(-9.57754329642237,0.583102430601064,
8.72981017245923));
#13153=CARTESIAN_POINT('Ctrl Pts',(-9.65136659729242,0.293655596344229,
8.74181335924855));
#13154=CARTESIAN_POINT('Ctrl Pts',(-9.67581103310575,0.197813707970559,
8.745787864934));
#13155=CARTESIAN_POINT('Ctrl Pts',(-9.68822500000015,0.0989100500905081,
8.74976237061946));
#13156=CARTESIAN_POINT('Ctrl Pts',(-9.688225,-1.80067072363954E-12,8.75373687630491));
#13157=CARTESIAN_POINT('Origin',(-8.5,0.,1.8));
#13158=CARTESIAN_POINT('',(-9.688225,-2.40918396343659E-14,9.09626312369518));
#13159=CARTESIAN_POINT('',(-9.688225,-1.77513559407316E-12,9.05373687630491));
#13160=CARTESIAN_POINT('',(-9.688225,-1.45515594291686E-16,1.8));
#13161=CARTESIAN_POINT('Ctrl Pts',(-9.688225,9.54791801177635E-15,9.09626312369518));
#13162=CARTESIAN_POINT('Ctrl Pts',(-9.688225,0.298712821306092,9.08425993690586));
#13163=CARTESIAN_POINT('Ctrl Pts',(-9.57054245632587,0.595858078271515,
9.07225675011654));
#13164=CARTESIAN_POINT('Ctrl Pts',(-9.36601586214937,0.813569405232702,
9.06025356332722));
#13165=CARTESIAN_POINT('Ctrl Pts',(-9.16148926797287,1.03128073219389,9.04825037653791));
#13166=CARTESIAN_POINT('Ctrl Pts',(-8.87226522412851,1.16727314847134,9.03624718974859));
#13167=CARTESIAN_POINT('Ctrl Pts',(-8.57413435701456,1.1859100926019,9.02424400295927));
#13168=CARTESIAN_POINT('Ctrl Pts',(-8.27600348990061,1.20454703673245,9.01224081616995));
#13169=CARTESIAN_POINT('Ctrl Pts',(-7.97209482032103,1.10563290540114,9.00023762938064));
#13170=CARTESIAN_POINT('Ctrl Pts',(-7.7420470537207,0.915087963996648,8.98823444259132));
#13171=CARTESIAN_POINT('Ctrl Pts',(-7.51199928712037,0.724543022592161,
8.976231255802));
#13172=CARTESIAN_POINT('Ctrl Pts',(-7.3582268807964,0.444367128061606,8.96422806901269));
#13173=CARTESIAN_POINT('Ctrl Pts',(-7.32102560975819,0.147979855990451,
8.95222488222337));
#13174=CARTESIAN_POINT('Ctrl Pts',(-7.28382433871998,-0.148407416080705,
8.94022169543405));
#13175=CARTESIAN_POINT('Ctrl Pts',(-7.3635846474463,-0.457895344721783,
8.92821850864473));
#13176=CARTESIAN_POINT('Ctrl Pts',(-7.53940549437871,-0.69938318995754,
8.91621532185541));
#13177=CARTESIAN_POINT('Ctrl Pts',(-7.71522634131112,-0.940871035193297,
8.9042121350661));
#13178=CARTESIAN_POINT('Ctrl Pts',(-7.98526240565763,-1.11182427083073,
8.89220894827678));
#13179=CARTESIAN_POINT('Ctrl Pts',(-8.27875123560094,-1.16744491727742,
8.88020576148746));
#13180=CARTESIAN_POINT('Ctrl Pts',(-8.57224006554425,-1.22306556372412,
8.86820257469815));
#13181=CARTESIAN_POINT('Ctrl Pts',(-8.88610136059915,-1.16276985667032,
8.85619938790883));
#13182=CARTESIAN_POINT('Ctrl Pts',(-9.13808834820071,-1.00235817476364,
8.84419620111951));
#13183=CARTESIAN_POINT('Ctrl Pts',(-9.39007533580227,-0.84194649285695,
8.83219301433019));
#13184=CARTESIAN_POINT('Ctrl Pts',(-9.57754329642122,-0.583102430603179,
8.82018982754088));
#13185=CARTESIAN_POINT('Ctrl Pts',(-9.65136659729183,-0.293655596346513,
8.80818664075156));
#13186=CARTESIAN_POINT('Ctrl Pts',(-9.6758110331054,-0.197813707972717,
8.8042121350661));
#13187=CARTESIAN_POINT('Ctrl Pts',(-9.688225,-0.0989100500925048,8.80023762938064));
#13188=CARTESIAN_POINT('Ctrl Pts',(-9.688225,-1.58761892521397E-14,8.79626312369518));
#13189=CARTESIAN_POINT('Ctrl Pts',(-9.688225,-1.80067072363954E-12,8.75373687630491));
#13190=CARTESIAN_POINT('Ctrl Pts',(-9.68822499999955,-0.298712821307894,
8.76574006309423));
#13191=CARTESIAN_POINT('Ctrl Pts',(-9.57054245632496,-0.595858078273151,
8.77774324988355));
#13192=CARTESIAN_POINT('Ctrl Pts',(-9.36601586214812,-0.813569405234032,
8.78974643667286));
#13193=CARTESIAN_POINT('Ctrl Pts',(-9.16148926797127,-1.03128073219491,
8.80174962346218));
#13194=CARTESIAN_POINT('Ctrl Pts',(-8.87226522412669,-1.16727314847192,
8.8137528102515));
#13195=CARTESIAN_POINT('Ctrl Pts',(-8.57413435701271,-1.18591009260201,
8.82575599704082));
#13196=CARTESIAN_POINT('Ctrl Pts',(-8.27600348989872,-1.2045470367321,8.83775918383014));
#13197=CARTESIAN_POINT('Ctrl Pts',(-7.97209482031928,-1.1056329054003,8.84976237061945));
#13198=CARTESIAN_POINT('Ctrl Pts',(-7.74204705371924,-0.915087963995441,
8.86176555740877));
#13199=CARTESIAN_POINT('Ctrl Pts',(-7.51199928711921,-0.724543022590581,
8.87376874419809));
#13200=CARTESIAN_POINT('Ctrl Pts',(-7.35822688079568,-0.444367128059766,
8.88577193098741));
#13201=CARTESIAN_POINT('Ctrl Pts',(-7.32102560975795,-0.147979855988539,
8.89777511777672));
#13202=CARTESIAN_POINT('Ctrl Pts',(-7.28382433872022,0.148407416082687,
8.90977830456604));
#13203=CARTESIAN_POINT('Ctrl Pts',(-7.36358464744704,0.457895344723648,
8.92178149135536));
#13204=CARTESIAN_POINT('Ctrl Pts',(-7.53940549437986,0.699383189959124,
8.93378467814468));
#13205=CARTESIAN_POINT('Ctrl Pts',(-7.71522634131268,0.9408710351946,8.945787864934));
#13206=CARTESIAN_POINT('Ctrl Pts',(-7.98526240565949,1.11182427083159,8.95779105172331));
#13207=CARTESIAN_POINT('Ctrl Pts',(-8.2787512356029,1.16744491727779,8.96979423851263));
#13208=CARTESIAN_POINT('Ctrl Pts',(-8.57224006554631,1.223065563724,8.98179742530195));
#13209=CARTESIAN_POINT('Ctrl Pts',(-8.88610136060113,1.16276985666967,8.99380061209127));
#13210=CARTESIAN_POINT('Ctrl Pts',(-9.13808834820242,1.00235817476255,9.00580379888059));
#13211=CARTESIAN_POINT('Ctrl Pts',(-9.39007533580372,0.841946492855425,
9.01780698566991));
#13212=CARTESIAN_POINT('Ctrl Pts',(-9.57754329642223,0.583102430601321,
9.02981017245922));
#13213=CARTESIAN_POINT('Ctrl Pts',(-9.65136659729234,0.293655596344516,
9.04181335924854));
#13214=CARTESIAN_POINT('Ctrl Pts',(-9.67581103310572,0.197813707970765,
9.045787864934));
#13215=CARTESIAN_POINT('Ctrl Pts',(-9.68822500000015,0.0989100500906238,
9.04976237061945));
#13216=CARTESIAN_POINT('Ctrl Pts',(-9.688225,-1.77513559407316E-12,9.05373687630491));
#13217=CARTESIAN_POINT('Origin',(-8.5,0.,1.8));
#13218=CARTESIAN_POINT('',(-9.68802305040078,0.000608274356598134,9.39626312369518));
#13219=CARTESIAN_POINT('',(-9.688225,-1.74948944220432E-12,9.35373687630491));
#13220=CARTESIAN_POINT('',(-9.688225,-1.45515594291686E-16,1.8));
#13221=CARTESIAN_POINT('Ctrl Pts',(-9.688225,3.530509218308E-14,9.39626312369518));
#13222=CARTESIAN_POINT('Ctrl Pts',(-9.68822499999999,0.298712821306129,
9.38425993690586));
#13223=CARTESIAN_POINT('Ctrl Pts',(-9.57054245632584,0.595858078271561,
9.37225675011654));
#13224=CARTESIAN_POINT('Ctrl Pts',(-9.36601586214933,0.813569405232745,
9.36025356332722));
#13225=CARTESIAN_POINT('Ctrl Pts',(-9.16148926797281,1.03128073219393,9.3482503765379));
#13226=CARTESIAN_POINT('Ctrl Pts',(-8.87226522412843,1.16727314847137,9.33624718974859));
#13227=CARTESIAN_POINT('Ctrl Pts',(-8.57413435701447,1.1859100926019,9.32424400295927));
#13228=CARTESIAN_POINT('Ctrl Pts',(-8.27600348990051,1.20454703673244,9.31224081616995));
#13229=CARTESIAN_POINT('Ctrl Pts',(-7.97209482032092,1.10563290540109,9.30023762938063));
#13230=CARTESIAN_POINT('Ctrl Pts',(-7.7420470537206,0.915087963996567,9.28823444259131));
#13231=CARTESIAN_POINT('Ctrl Pts',(-7.51199928712029,0.724543022592049,
9.276231255802));
#13232=CARTESIAN_POINT('Ctrl Pts',(-7.35822688079634,0.444367128061463,
9.26422806901268));
#13233=CARTESIAN_POINT('Ctrl Pts',(-7.32102560975817,0.147979855990291,
9.25222488222336));
#13234=CARTESIAN_POINT('Ctrl Pts',(-7.28382433872,-0.148407416080881,9.24022169543404));
#13235=CARTESIAN_POINT('Ctrl Pts',(-7.36358464744636,-0.457895344721959,
9.22821850864473));
#13236=CARTESIAN_POINT('Ctrl Pts',(-7.53940549437882,-0.699383189957697,
9.21621532185541));
#13237=CARTESIAN_POINT('Ctrl Pts',(-7.71522634131128,-0.940871035193435,
9.20421213506609));
#13238=CARTESIAN_POINT('Ctrl Pts',(-7.98526240565783,-1.11182427083082,
9.19220894827677));
#13239=CARTESIAN_POINT('Ctrl Pts',(-8.27875123560116,-1.16744491727747,
9.18020576148745));
#13240=CARTESIAN_POINT('Ctrl Pts',(-8.57224006554449,-1.22306556372411,
9.16820257469814));
#13241=CARTESIAN_POINT('Ctrl Pts',(-8.8861013605994,-1.16276985667024,9.15619938790882));
#13242=CARTESIAN_POINT('Ctrl Pts',(-9.13808834820093,-1.0023581747635,9.1441962011195));
#13243=CARTESIAN_POINT('Ctrl Pts',(-9.39007533580246,-0.841946492856748,
9.13219301433018));
#13244=CARTESIAN_POINT('Ctrl Pts',(-9.57754329642136,-0.583102430602922,
9.12018982754086));
#13245=CARTESIAN_POINT('Ctrl Pts',(-9.65136659729191,-0.293655596346227,
9.10818664075155));
#13246=CARTESIAN_POINT('Ctrl Pts',(-9.67581103310543,-0.197813707972512,
9.10421213506609));
#13247=CARTESIAN_POINT('Ctrl Pts',(-9.688225,-0.0989100500923894,9.10023762938063));
#13248=CARTESIAN_POINT('Ctrl Pts',(-9.688225,9.54791801177635E-15,9.09626312369518));
#13249=CARTESIAN_POINT('Ctrl Pts',(-9.688225,-1.77513559407316E-12,9.05373687630491));
#13250=CARTESIAN_POINT('Ctrl Pts',(-9.68822499999955,-0.298712821307869,
9.06574006309423));
#13251=CARTESIAN_POINT('Ctrl Pts',(-9.57054245632497,-0.595858078273128,
9.07774324988354));
#13252=CARTESIAN_POINT('Ctrl Pts',(-9.36601586214813,-0.813569405234013,
9.08974643667286));
#13253=CARTESIAN_POINT('Ctrl Pts',(-9.1614892679713,-1.0312807321949,9.10174962346218));
#13254=CARTESIAN_POINT('Ctrl Pts',(-8.87226522412672,-1.16727314847191,
9.1137528102515));
#13255=CARTESIAN_POINT('Ctrl Pts',(-8.57413435701273,-1.18591009260201,
9.12575599704082));
#13256=CARTESIAN_POINT('Ctrl Pts',(-8.27600348989875,-1.20454703673211,
9.13775918383014));
#13257=CARTESIAN_POINT('Ctrl Pts',(-7.9720948203193,-1.10563290540031,9.14976237061945));
#13258=CARTESIAN_POINT('Ctrl Pts',(-7.74204705371926,-0.915087963995458,
9.16176555740877));
#13259=CARTESIAN_POINT('Ctrl Pts',(-7.51199928711922,-0.724543022590602,
9.17376874419809));
#13260=CARTESIAN_POINT('Ctrl Pts',(-7.35822688079569,-0.444367128059791,
9.18577193098741));
#13261=CARTESIAN_POINT('Ctrl Pts',(-7.32102560975795,-0.147979855988565,
9.19777511777673));
#13262=CARTESIAN_POINT('Ctrl Pts',(-7.28382433872022,0.148407416082661,
9.20977830456604));
#13263=CARTESIAN_POINT('Ctrl Pts',(-7.36358464744704,0.457895344723623,
9.22178149135536));
#13264=CARTESIAN_POINT('Ctrl Pts',(-7.53940549437985,0.699383189959103,
9.23378467814468));
#13265=CARTESIAN_POINT('Ctrl Pts',(-7.71522634131266,0.940871035194583,
9.245787864934));
#13266=CARTESIAN_POINT('Ctrl Pts',(-7.98526240565946,1.11182427083158,9.25779105172331));
#13267=CARTESIAN_POINT('Ctrl Pts',(-8.27875123560287,1.16744491727779,9.26979423851263));
#13268=CARTESIAN_POINT('Ctrl Pts',(-8.57224006554628,1.223065563724,9.28179742530195));
#13269=CARTESIAN_POINT('Ctrl Pts',(-8.8861013606011,1.16276985666968,9.29380061209127));
#13270=CARTESIAN_POINT('Ctrl Pts',(-9.1380883482024,1.00235817476256,9.30580379888059));
#13271=CARTESIAN_POINT('Ctrl Pts',(-9.3900753358037,0.841946492855444,9.3178069856699));
#13272=CARTESIAN_POINT('Ctrl Pts',(-9.57754329642221,0.583102430601344,
9.32981017245922));
#13273=CARTESIAN_POINT('Ctrl Pts',(-9.65136659729234,0.293655596344541,
9.34181335924854));
#13274=CARTESIAN_POINT('Ctrl Pts',(-9.67581103310571,0.197813707970801,
9.34578786493399));
#13275=CARTESIAN_POINT('Ctrl Pts',(-9.68822500000014,0.0989100500906719,
9.34976237061945));
#13276=CARTESIAN_POINT('Ctrl Pts',(-9.688225,-1.71568315110449E-12,9.35373687630491));
#13277=CARTESIAN_POINT('Origin',(-8.5,0.,1.8));
#13278=CARTESIAN_POINT('',(-9.68728951167887,-0.000140790589323958,9.69626312369518));
#13279=CARTESIAN_POINT('',(-9.688225,-1.72389880148671E-12,9.65373687630491));
#13280=CARTESIAN_POINT('',(-9.688225,-1.45515594291686E-16,1.8));
#13281=CARTESIAN_POINT('Ctrl Pts',(-9.68633624213298,-0.000284257245408481,
9.69626312369518));
#13282=CARTESIAN_POINT('Ctrl Pts',(-9.68599772448992,0.214868365865776,
9.68764808520634));
#13283=CARTESIAN_POINT('Ctrl Pts',(-9.63021606168018,0.430233739330785,
9.67903304671751));
#13284=CARTESIAN_POINT('Ctrl Pts',(-9.52020978820705,0.613158016442515,
9.67041800822868));
#13285=CARTESIAN_POINT('Ctrl Pts',(-9.31708738507166,0.950920742018469,
9.65451066707706));
#13286=CARTESIAN_POINT('Ctrl Pts',(-8.92909040695752,1.17807808330892,9.63860332592544));
#13287=CARTESIAN_POINT('Ctrl Pts',(-8.5354559263329,1.18978224478168,9.62269598477382));
#13288=CARTESIAN_POINT('Ctrl Pts',(-8.14182144570827,1.20148640625444,9.6067886436222));
#13289=CARTESIAN_POINT('Ctrl Pts',(-7.74254946257315,0.997737387909526,
9.59088130247057));
#13290=CARTESIAN_POINT('Ctrl Pts',(-7.5188628313805,0.672951217350277,9.57497396131895));
#13291=CARTESIAN_POINT('Ctrl Pts',(-7.40701951578419,0.510558132070666,
9.56702029074314));
#13292=CARTESIAN_POINT('Ctrl Pts',(-7.3390725381735,0.317905758737486,9.55906662016734));
#13293=CARTESIAN_POINT('Ctrl Pts',(-7.31893965943283,0.120379919441194,
9.55111294959153));
#13294=CARTESIAN_POINT('Ctrl Pts',(-7.29880678069217,-0.0771459198551094,
9.54315927901572));
#13295=CARTESIAN_POINT('Ctrl Pts',(-7.32648800082156,-0.279545225114548,
9.5352056084399));
#13296=CARTESIAN_POINT('Ctrl Pts',(-7.40326782979251,-0.461163779379811,
9.52725193786409));
#13297=CARTESIAN_POINT('Ctrl Pts',(-7.55682748773441,-0.824400887910347,
9.51134459671246));
#13298=CARTESIAN_POINT('Ctrl Pts',(-7.90678158104258,-1.10451499246429,
9.49543725556086));
#13299=CARTESIAN_POINT('Ctrl Pts',(-8.29468277135129,-1.1724690820358,9.47952991440923));
#13300=CARTESIAN_POINT('Ctrl Pts',(-8.68258396166,-1.24042317160732,9.46362257325761));
#13301=CARTESIAN_POINT('Ctrl Pts',(-9.10843224896924,-1.09621724619641,
9.44771523210598));
#13302=CARTESIAN_POINT('Ctrl Pts',(-9.37552284820049,-0.806381117933753,
9.43180789095436));
#13303=CARTESIAN_POINT('Ctrl Pts',(-9.57445978547795,-0.590502641361061,
9.4199596352013));
#13304=CARTESIAN_POINT('Ctrl Pts',(-9.68532258180007,-0.293832770251182,
9.40811137944824));
#13305=CARTESIAN_POINT('Ctrl Pts',(-9.68786906204226,0.0010720889423268,
9.39626312369517));
#13306=CARTESIAN_POINT('Ctrl Pts',(-9.688225,-1.71568315110449E-12,9.35373687630491));
#13307=CARTESIAN_POINT('Ctrl Pts',(-9.68822499999957,-0.298712821307787,
9.36574006309422));
#13308=CARTESIAN_POINT('Ctrl Pts',(-9.57054245632502,-0.59585807827303,
9.37774324988354));
#13309=CARTESIAN_POINT('Ctrl Pts',(-9.36601586214822,-0.813569405233921,
9.38974643667286));
#13310=CARTESIAN_POINT('Ctrl Pts',(-9.16148926797142,-1.03128073219481,
9.40174962346217));
#13311=CARTESIAN_POINT('Ctrl Pts',(-8.87226522412689,-1.16727314847185,
9.41375281025149));
#13312=CARTESIAN_POINT('Ctrl Pts',(-8.57413435701293,-1.185910092602,9.42575599704081));
#13313=CARTESIAN_POINT('Ctrl Pts',(-8.27600348989897,-1.20454703673214,
9.43775918383013));
#13314=CARTESIAN_POINT('Ctrl Pts',(-7.97209482031953,-1.10563290540042,
9.44976237061944));
#13315=CARTESIAN_POINT('Ctrl Pts',(-7.74204705371947,-0.915087963995625,
9.46176555740876));
#13316=CARTESIAN_POINT('Ctrl Pts',(-7.5119992871194,-0.724543022590834,
9.47376874419808));
#13317=CARTESIAN_POINT('Ctrl Pts',(-7.35822688079581,-0.444367128060085,
9.4857719309874));
#13318=CARTESIAN_POINT('Ctrl Pts',(-7.321025609758,-0.147979855988892,9.49777511777671));
#13319=CARTESIAN_POINT('Ctrl Pts',(-7.28382433872018,0.148407416082302,
9.50977830456603));
#13320=CARTESIAN_POINT('Ctrl Pts',(-7.3635846474469,0.457895344723262,9.52178149135535));
#13321=CARTESIAN_POINT('Ctrl Pts',(-7.53940549437961,0.699383189958782,
9.53378467814466));
#13322=CARTESIAN_POINT('Ctrl Pts',(-7.71522634131233,0.940871035194303,
9.54578786493398));
#13323=CARTESIAN_POINT('Ctrl Pts',(-7.98526240565905,1.11182427083138,9.5577910517233));
#13324=CARTESIAN_POINT('Ctrl Pts',(-8.27875123560242,1.1674449172777,9.56979423851261));
#13325=CARTESIAN_POINT('Ctrl Pts',(-8.57224006554578,1.22306556372403,9.58179742530193));
#13326=CARTESIAN_POINT('Ctrl Pts',(-8.8861013606006,1.16276985666984,9.59380061209125));
#13327=CARTESIAN_POINT('Ctrl Pts',(-9.13808834820195,1.00235817476285,9.60580379888056));
#13328=CARTESIAN_POINT('Ctrl Pts',(-9.3900753358033,0.841946492855855,9.61780698566988));
#13329=CARTESIAN_POINT('Ctrl Pts',(-9.57754329642193,0.583102430601866,
9.6298101724592));
#13330=CARTESIAN_POINT('Ctrl Pts',(-9.65136659729219,0.293655596345122,
9.64181335924851));
#13331=CARTESIAN_POINT('Ctrl Pts',(-9.67581103310566,0.197813707971209,
9.64578786493398));
#13332=CARTESIAN_POINT('Ctrl Pts',(-9.68822500000014,0.0989100500908889,
9.64976237061944));
#13333=CARTESIAN_POINT('Ctrl Pts',(-9.688225,-1.69009251038688E-12,9.65373687630491));
#13334=CARTESIAN_POINT('Origin',(-8.5,0.,1.8));
#13335=CARTESIAN_POINT('',(-9.688225,5.27355936696949E-14,9.99626312369517));
#13336=CARTESIAN_POINT('',(-9.688225,-1.69825264961787E-12,9.95373687630491));
#13337=CARTESIAN_POINT('',(-9.688225,-1.45515594291686E-16,1.8));
#13338=CARTESIAN_POINT('Ctrl Pts',(-9.688225,8.65973959207622E-14,9.99626312369517));
#13339=CARTESIAN_POINT('Ctrl Pts',(-9.68822499999998,0.29871282130618,9.98425993690586));
#13340=CARTESIAN_POINT('Ctrl Pts',(-9.57054245632582,0.595858078271607,
9.97225675011654));
#13341=CARTESIAN_POINT('Ctrl Pts',(-9.36601586214929,0.813569405232783,
9.96025356332722));
#13342=CARTESIAN_POINT('Ctrl Pts',(-9.16148926797276,1.03128073219396,9.9482503765379));
#13343=CARTESIAN_POINT('Ctrl Pts',(-8.87226522412838,1.16727314847138,9.93624718974858));
#13344=CARTESIAN_POINT('Ctrl Pts',(-8.57413435701442,1.18591009260191,9.92424400295927));
#13345=CARTESIAN_POINT('Ctrl Pts',(-8.27600348990046,1.20454703673243,9.91224081616995));
#13346=CARTESIAN_POINT('Ctrl Pts',(-7.97209482032087,1.10563290540106,9.90023762938063));
#13347=CARTESIAN_POINT('Ctrl Pts',(-7.74204705372056,0.915087963996535,
9.88823444259131));
#13348=CARTESIAN_POINT('Ctrl Pts',(-7.51199928712025,0.724543022592006,
9.87623125580199));
#13349=CARTESIAN_POINT('Ctrl Pts',(-7.35822688079632,0.444367128061413,
9.86422806901268));
#13350=CARTESIAN_POINT('Ctrl Pts',(-7.32102560975816,0.14797985599024,9.85222488222336));
#13351=CARTESIAN_POINT('Ctrl Pts',(-7.28382433872001,-0.148407416080933,
9.84022169543404));
#13352=CARTESIAN_POINT('Ctrl Pts',(-7.36358464744638,-0.457895344722009,
9.82821850864472));
#13353=CARTESIAN_POINT('Ctrl Pts',(-7.53940549437885,-0.699383189957739,
9.8162153218554));
#13354=CARTESIAN_POINT('Ctrl Pts',(-7.71522634131132,-0.940871035193468,
9.80421213506609));
#13355=CARTESIAN_POINT('Ctrl Pts',(-7.98526240565788,-1.11182427083084,
9.79220894827677));
#13356=CARTESIAN_POINT('Ctrl Pts',(-8.27875123560121,-1.16744491727748,
9.78020576148745));
#13357=CARTESIAN_POINT('Ctrl Pts',(-8.57224006554454,-1.22306556372411,
9.76820257469813));
#13358=CARTESIAN_POINT('Ctrl Pts',(-8.88610136059945,-1.16276985667023,
9.75619938790882));
#13359=CARTESIAN_POINT('Ctrl Pts',(-9.13808834820098,-1.00235817476347,
9.7441962011195));
#13360=CARTESIAN_POINT('Ctrl Pts',(-9.3900753358025,-0.841946492856709,
9.73219301433018));
#13361=CARTESIAN_POINT('Ctrl Pts',(-9.57754329642139,-0.583102430602876,
9.72018982754086));
#13362=CARTESIAN_POINT('Ctrl Pts',(-9.65136659729192,-0.293655596346177,
9.70818664075154));
#13363=CARTESIAN_POINT('Ctrl Pts',(-9.67581103310543,-0.197813707972472,
9.70421213506609));
#13364=CARTESIAN_POINT('Ctrl Pts',(-9.688225,-0.0989100500923605,9.70023762938063));
#13365=CARTESIAN_POINT('Ctrl Pts',(-9.688225,2.70894418008538E-14,9.69626312369518));
#13366=CARTESIAN_POINT('Ctrl Pts',(-9.688225,-1.69009251038688E-12,9.65373687630491));
#13367=CARTESIAN_POINT('Ctrl Pts',(-9.68822499999957,-0.298712821307784,
9.66574006309422));
#13368=CARTESIAN_POINT('Ctrl Pts',(-9.57054245632501,-0.595858078273051,
9.67774324988354));
#13369=CARTESIAN_POINT('Ctrl Pts',(-9.36601586214819,-0.813569405233951,
9.68974643667286));
#13370=CARTESIAN_POINT('Ctrl Pts',(-9.16148926797137,-1.03128073219485,
9.70174962346218));
#13371=CARTESIAN_POINT('Ctrl Pts',(-8.8722652241268,-1.16727314847189,9.7137528102515));
#13372=CARTESIAN_POINT('Ctrl Pts',(-8.57413435701282,-1.185910092602,9.72575599704081));
#13373=CARTESIAN_POINT('Ctrl Pts',(-8.27600348989883,-1.20454703673212,
9.73775918383013));
#13374=CARTESIAN_POINT('Ctrl Pts',(-7.97209482031938,-1.10563290540035,
9.74976237061945));
#13375=CARTESIAN_POINT('Ctrl Pts',(-7.74204705371933,-0.915087963995512,
9.76176555740877));
#13376=CARTESIAN_POINT('Ctrl Pts',(-7.51199928711928,-0.724543022590673,
9.77376874419808));
#13377=CARTESIAN_POINT('Ctrl Pts',(-7.35822688079572,-0.444367128059873,
9.7857719309874));
#13378=CARTESIAN_POINT('Ctrl Pts',(-7.32102560975796,-0.147979855988649,
9.79777511777672));
#13379=CARTESIAN_POINT('Ctrl Pts',(-7.28382433872021,0.148407416082574,
9.80977830456604));
#13380=CARTESIAN_POINT('Ctrl Pts',(-7.363584647447,0.457895344723542,9.82178149135536));
#13381=CARTESIAN_POINT('Ctrl Pts',(-7.5394054943798,0.699383189959035,9.83378467814468));
#13382=CARTESIAN_POINT('Ctrl Pts',(-7.71522634131259,0.940871035194527,
9.84578786493399));
#13383=CARTESIAN_POINT('Ctrl Pts',(-7.98526240565938,1.11182427083154,9.85779105172331));
#13384=CARTESIAN_POINT('Ctrl Pts',(-8.27875123560279,1.16744491727777,9.86979423851263));
#13385=CARTESIAN_POINT('Ctrl Pts',(-8.57224006554619,1.22306556372401,9.88179742530195));
#13386=CARTESIAN_POINT('Ctrl Pts',(-8.88610136060102,1.16276985666971,9.89380061209126));
#13387=CARTESIAN_POINT('Ctrl Pts',(-9.13808834820233,1.00235817476261,9.90580379888058));
#13388=CARTESIAN_POINT('Ctrl Pts',(-9.39007533580364,0.841946492855508,
9.9178069856699));
#13389=CARTESIAN_POINT('Ctrl Pts',(-9.57754329642217,0.583102430601421,
9.92981017245922));
#13390=CARTESIAN_POINT('Ctrl Pts',(-9.65136659729231,0.293655596344623,
9.94181335924854));
#13391=CARTESIAN_POINT('Ctrl Pts',(-9.6758110331057,0.197813707970874,9.94578786493399));
#13392=CARTESIAN_POINT('Ctrl Pts',(-9.68822500000014,0.0989100500907344,
9.94976237061945));
#13393=CARTESIAN_POINT('Ctrl Pts',(-9.688225,-1.66444635851803E-12,9.95373687630491));
#13394=CARTESIAN_POINT('Origin',(-8.5,0.,1.8));
#13395=CARTESIAN_POINT('',(-9.688225,7.84927678409986E-14,10.2962631236952));
#13396=CARTESIAN_POINT('',(-9.688225,-1.67266200890026E-12,10.2537368763049));
#13397=CARTESIAN_POINT('',(-9.688225,-1.45515594291686E-16,1.8));
#13398=CARTESIAN_POINT('Ctrl Pts',(-9.688225,1.12132525487141E-13,10.2962631236952));
#13399=CARTESIAN_POINT('Ctrl Pts',(-9.68822499999997,0.298712821306206,
10.2842599369059));
#13400=CARTESIAN_POINT('Ctrl Pts',(-9.57054245632581,0.59585807827163,10.2722567501165));
#13401=CARTESIAN_POINT('Ctrl Pts',(-9.36601586214927,0.813569405232801,
10.2602535633272));
#13402=CARTESIAN_POINT('Ctrl Pts',(-9.16148926797274,1.03128073219397,10.2482503765379));
#13403=CARTESIAN_POINT('Ctrl Pts',(-8.87226522412835,1.16727314847139,10.2362471897486));
#13404=CARTESIAN_POINT('Ctrl Pts',(-8.57413435701439,1.18591009260191,10.2242440029593));
#13405=CARTESIAN_POINT('Ctrl Pts',(-8.27600348990043,1.20454703673242,10.2122408161699));
#13406=CARTESIAN_POINT('Ctrl Pts',(-7.97209482032085,1.10563290540105,10.2002376293806));
#13407=CARTESIAN_POINT('Ctrl Pts',(-7.74204705372054,0.915087963996519,
10.1882344425913));
#13408=CARTESIAN_POINT('Ctrl Pts',(-7.51199928712024,0.724543022591985,
10.176231255802));
#13409=CARTESIAN_POINT('Ctrl Pts',(-7.35822688079631,0.444367128061389,
10.1642280690127));
#13410=CARTESIAN_POINT('Ctrl Pts',(-7.32102560975816,0.147979855990215,
10.1522248822234));
#13411=CARTESIAN_POINT('Ctrl Pts',(-7.28382433872001,-0.148407416080959,
10.140221695434));
#13412=CARTESIAN_POINT('Ctrl Pts',(-7.36358464744639,-0.457895344722033,
10.1282185086447));
#13413=CARTESIAN_POINT('Ctrl Pts',(-7.53940549437887,-0.699383189957759,
10.1162153218554));
#13414=CARTESIAN_POINT('Ctrl Pts',(-7.71522634131134,-0.940871035193485,
10.1042121350661));
#13415=CARTESIAN_POINT('Ctrl Pts',(-7.98526240565791,-1.11182427083086,
10.0922089482768));
#13416=CARTESIAN_POINT('Ctrl Pts',(-8.27875123560124,-1.16744491727748,
10.0802057614875));
#13417=CARTESIAN_POINT('Ctrl Pts',(-8.57224006554457,-1.22306556372411,
10.0682025746981));
#13418=CARTESIAN_POINT('Ctrl Pts',(-8.88610136059948,-1.16276985667022,
10.0561993879088));
#13419=CARTESIAN_POINT('Ctrl Pts',(-9.138088348201,-1.00235817476345,10.0441962011195));
#13420=CARTESIAN_POINT('Ctrl Pts',(-9.39007533580252,-0.84194649285669,
10.0321930143302));
#13421=CARTESIAN_POINT('Ctrl Pts',(-9.5775432964214,-0.583102430602852,
10.0201898275409));
#13422=CARTESIAN_POINT('Ctrl Pts',(-9.65136659729193,-0.293655596346152,
10.0081866407515));
#13423=CARTESIAN_POINT('Ctrl Pts',(-9.67581103310544,-0.197813707972436,
10.0042121350661));
#13424=CARTESIAN_POINT('Ctrl Pts',(-9.68822500000001,-0.0989100500923123,
10.0002376293806));
#13425=CARTESIAN_POINT('Ctrl Pts',(-9.688225,8.65973959207622E-14,9.99626312369517));
#13426=CARTESIAN_POINT('Ctrl Pts',(-9.688225,-1.66444635851803E-12,9.95373687630491));
#13427=CARTESIAN_POINT('Ctrl Pts',(-9.68822499999958,-0.298712821307758,
9.96574006309422));
#13428=CARTESIAN_POINT('Ctrl Pts',(-9.57054245632503,-0.595858078273028,
9.97774324988354));
#13429=CARTESIAN_POINT('Ctrl Pts',(-9.36601586214821,-0.813569405233932,
9.98974643667286));
#13430=CARTESIAN_POINT('Ctrl Pts',(-9.16148926797139,-1.03128073219484,
10.0017496234622));
#13431=CARTESIAN_POINT('Ctrl Pts',(-8.87226522412683,-1.16727314847188,
10.0137528102515));
#13432=CARTESIAN_POINT('Ctrl Pts',(-8.57413435701284,-1.185910092602,10.0257559970408));
#13433=CARTESIAN_POINT('Ctrl Pts',(-8.27600348989886,-1.20454703673213,
10.0377591838301));
#13434=CARTESIAN_POINT('Ctrl Pts',(-7.97209482031941,-1.10563290540036,
10.0497623706194));
#13435=CARTESIAN_POINT('Ctrl Pts',(-7.74204705371935,-0.915087963995528,
10.0617655574088));
#13436=CARTESIAN_POINT('Ctrl Pts',(-7.51199928711929,-0.724543022590694,
10.0737687441981));
#13437=CARTESIAN_POINT('Ctrl Pts',(-7.35822688079573,-0.444367128059897,
10.0857719309874));
#13438=CARTESIAN_POINT('Ctrl Pts',(-7.32102560975797,-0.147979855988675,
10.0977751177767));
#13439=CARTESIAN_POINT('Ctrl Pts',(-7.2838243387202,0.148407416082548,10.109778304566));
#13440=CARTESIAN_POINT('Ctrl Pts',(-7.36358464744699,0.457895344723518,
10.1217814913554));
#13441=CARTESIAN_POINT('Ctrl Pts',(-7.53940549437978,0.699383189959014,
10.1337846781447));
#13442=CARTESIAN_POINT('Ctrl Pts',(-7.71522634131257,0.94087103519451,10.145787864934));
#13443=CARTESIAN_POINT('Ctrl Pts',(-7.98526240565936,1.11182427083153,10.1577910517233));
#13444=CARTESIAN_POINT('Ctrl Pts',(-8.27875123560277,1.16744491727777,10.1697942385126));
#13445=CARTESIAN_POINT('Ctrl Pts',(-8.57224006554617,1.22306556372401,10.1817974253019));
#13446=CARTESIAN_POINT('Ctrl Pts',(-8.88610136060099,1.16276985666971,10.1938006120913));
#13447=CARTESIAN_POINT('Ctrl Pts',(-9.13808834820231,1.00235817476262,10.2058037988806));
#13448=CARTESIAN_POINT('Ctrl Pts',(-9.39007533580362,0.841946492855527,
10.2178069856699));
#13449=CARTESIAN_POINT('Ctrl Pts',(-9.57754329642216,0.583102430601445,
10.2298101724592));
#13450=CARTESIAN_POINT('Ctrl Pts',(-9.65136659729231,0.293655596344648,
10.2418133592485));
#13451=CARTESIAN_POINT('Ctrl Pts',(-9.6758110331057,0.1978137079709,10.245787864934));
#13452=CARTESIAN_POINT('Ctrl Pts',(-9.68822500000014,0.09891005009076,10.2497623706194));
#13453=CARTESIAN_POINT('Ctrl Pts',(-9.688225,-1.63885571780042E-12,10.2537368763049));
#13454=CARTESIAN_POINT('Origin',(-8.5,0.,1.8));
#13455=CARTESIAN_POINT('',(-9.688225,1.0413891970984E-13,10.5962631236952));
#13456=CARTESIAN_POINT('',(-9.688225,-1.64701585703142E-12,10.5537368763049));
#13457=CARTESIAN_POINT('',(-9.688225,-1.45515594291686E-16,1.8));
#13458=CARTESIAN_POINT('Ctrl Pts',(-9.688225,1.37778677355982E-13,10.5962631236952));
#13459=CARTESIAN_POINT('Ctrl Pts',(-9.68822499999997,0.29871282130622,10.5842599369059));
#13460=CARTESIAN_POINT('Ctrl Pts',(-9.5705424563258,0.595858078271631,10.5722567501165));
#13461=CARTESIAN_POINT('Ctrl Pts',(-9.36601586214928,0.813569405232795,
10.5602535633272));
#13462=CARTESIAN_POINT('Ctrl Pts',(-9.16148926797275,1.03128073219396,10.5482503765379));
#13463=CARTESIAN_POINT('Ctrl Pts',(-8.87226522412838,1.16727314847138,10.5362471897486));
#13464=CARTESIAN_POINT('Ctrl Pts',(-8.57413435701443,1.1859100926019,10.5242440029593));
#13465=CARTESIAN_POINT('Ctrl Pts',(-8.27600348990048,1.20454703673243,10.5122408161699));
#13466=CARTESIAN_POINT('Ctrl Pts',(-7.97209482032091,1.10563290540108,10.5002376293806));
#13467=CARTESIAN_POINT('Ctrl Pts',(-7.7420470537206,0.915087963996567,10.4882344425913));
#13468=CARTESIAN_POINT('Ctrl Pts',(-7.51199928712029,0.724543022592055,
10.476231255802));
#13469=CARTESIAN_POINT('Ctrl Pts',(-7.35822688079635,0.444367128061483,
10.4642280690127));
#13470=CARTESIAN_POINT('Ctrl Pts',(-7.32102560975817,0.147979855990323,
10.4522248822234));
#13471=CARTESIAN_POINT('Ctrl Pts',(-7.28382433872,-0.148407416080836,10.440221695434));
#13472=CARTESIAN_POINT('Ctrl Pts',(-7.36358464744634,-0.457895344721905,
10.4282185086447));
#13473=CARTESIAN_POINT('Ctrl Pts',(-7.53940549437878,-0.699383189957643,
10.4162153218554));
#13474=CARTESIAN_POINT('Ctrl Pts',(-7.71522634131122,-0.940871035193382,
10.4042121350661));
#13475=CARTESIAN_POINT('Ctrl Pts',(-7.98526240565775,-1.11182427083078,
10.3922089482768));
#13476=CARTESIAN_POINT('Ctrl Pts',(-8.27875123560107,-1.16744491727745,
10.3802057614875));
#13477=CARTESIAN_POINT('Ctrl Pts',(-8.57224006554438,-1.22306556372411,
10.3682025746981));
#13478=CARTESIAN_POINT('Ctrl Pts',(-8.88610136059928,-1.16276985667028,
10.3561993879088));
#13479=CARTESIAN_POINT('Ctrl Pts',(-9.13808834820082,-1.00235817476357,
10.3441962011195));
#13480=CARTESIAN_POINT('Ctrl Pts',(-9.39007533580236,-0.841946492856854,
10.3321930143302));
#13481=CARTESIAN_POINT('Ctrl Pts',(-9.57754329642128,-0.583102430603063,
10.3201898275409));
#13482=CARTESIAN_POINT('Ctrl Pts',(-9.65136659729187,-0.293655596346389,
10.3081866407516));
#13483=CARTESIAN_POINT('Ctrl Pts',(-9.67581103310542,-0.19781370797259,
10.3042121350661));
#13484=CARTESIAN_POINT('Ctrl Pts',(-9.68822500000001,-0.0989100500923768,
10.3002376293806));
#13485=CARTESIAN_POINT('Ctrl Pts',(-9.688225,1.12132525487141E-13,10.2962631236952));
#13486=CARTESIAN_POINT('Ctrl Pts',(-9.688225,-1.63885571780042E-12,10.2537368763049));
#13487=CARTESIAN_POINT('Ctrl Pts',(-9.68822499999959,-0.298712821307732,
10.2657400630942));
#13488=CARTESIAN_POINT('Ctrl Pts',(-9.57054245632504,-0.595858078273005,
10.2777432498835));
#13489=CARTESIAN_POINT('Ctrl Pts',(-9.36601586214823,-0.813569405233914,
10.2897464366729));
#13490=CARTESIAN_POINT('Ctrl Pts',(-9.16148926797141,-1.03128073219482,
10.3017496234622));
#13491=CARTESIAN_POINT('Ctrl Pts',(-8.87226522412685,-1.16727314847187,
10.3137528102515));
#13492=CARTESIAN_POINT('Ctrl Pts',(-8.57413435701287,-1.185910092602,10.3257559970408));
#13493=CARTESIAN_POINT('Ctrl Pts',(-8.27600348989888,-1.20454703673213,
10.3377591838301));
#13494=CARTESIAN_POINT('Ctrl Pts',(-7.97209482031943,-1.10563290540037,
10.3497623706194));
#13495=CARTESIAN_POINT('Ctrl Pts',(-7.74204705371937,-0.915087963995544,
10.3617655574088));
#13496=CARTESIAN_POINT('Ctrl Pts',(-7.51199928711931,-0.724543022590715,
10.3737687441981));
#13497=CARTESIAN_POINT('Ctrl Pts',(-7.35822688079574,-0.444367128059922,
10.3857719309874));
#13498=CARTESIAN_POINT('Ctrl Pts',(-7.32102560975797,-0.1479798559887,10.3977751177767));
#13499=CARTESIAN_POINT('Ctrl Pts',(-7.2838243387202,0.148407416082522,10.409778304566));
#13500=CARTESIAN_POINT('Ctrl Pts',(-7.36358464744698,0.457895344723493,
10.4217814913554));
#13501=CARTESIAN_POINT('Ctrl Pts',(-7.53940549437977,0.699383189958993,
10.4337846781447));
#13502=CARTESIAN_POINT('Ctrl Pts',(-7.71522634131255,0.940871035194494,
10.445787864934));
#13503=CARTESIAN_POINT('Ctrl Pts',(-7.98526240565934,1.11182427083152,10.4577910517233));
#13504=CARTESIAN_POINT('Ctrl Pts',(-8.27875123560274,1.16744491727776,10.4697942385126));
#13505=CARTESIAN_POINT('Ctrl Pts',(-8.57224006554614,1.22306556372401,10.4817974253019));
#13506=CARTESIAN_POINT('Ctrl Pts',(-8.88610136060097,1.16276985666972,10.4938006120913));
#13507=CARTESIAN_POINT('Ctrl Pts',(-9.13808834820228,1.00235817476263,10.5058037988806));
#13508=CARTESIAN_POINT('Ctrl Pts',(-9.3900753358036,0.841946492855546,10.5178069856699));
#13509=CARTESIAN_POINT('Ctrl Pts',(-9.57754329642215,0.583102430601468,
10.5298101724592));
#13510=CARTESIAN_POINT('Ctrl Pts',(-9.6513665972923,0.293655596344673,10.5418133592485));
#13511=CARTESIAN_POINT('Ctrl Pts',(-9.67581103310569,0.197813707970925,
10.545787864934));
#13512=CARTESIAN_POINT('Ctrl Pts',(-9.68822500000013,0.0989100500907857,
10.5497623706194));
#13513=CARTESIAN_POINT('Ctrl Pts',(-9.688225,-1.61320956593158E-12,10.5537368763049));
#13514=CARTESIAN_POINT('Origin',(-8.5,0.,1.8));
#13515=CARTESIAN_POINT('',(-9.688225,1.29674049276218E-13,10.8962631236952));
#13516=CARTESIAN_POINT('',(-9.688225,-1.62142521631381E-12,10.8537368763049));
#13517=CARTESIAN_POINT('',(-9.688225,-1.45515594291686E-16,1.8));
#13518=CARTESIAN_POINT('Ctrl Pts',(-9.688225,1.29674049276218E-13,10.8962631236952));
#13519=CARTESIAN_POINT('Ctrl Pts',(-9.68822499999997,0.298712821306223,
10.8842599369059));
#13520=CARTESIAN_POINT('Ctrl Pts',(-9.57054245632579,0.595858078271646,
10.8722567501165));
#13521=CARTESIAN_POINT('Ctrl Pts',(-9.36601586214926,0.813569405232814,
10.8602535633272));
#13522=CARTESIAN_POINT('Ctrl Pts',(-9.16148926797272,1.03128073219398,10.8482503765379));
#13523=CARTESIAN_POINT('Ctrl Pts',(-8.87226522412834,1.1672731484714,10.8362471897486));
#13524=CARTESIAN_POINT('Ctrl Pts',(-8.57413435701437,1.18591009260191,10.8242440029593));
#13525=CARTESIAN_POINT('Ctrl Pts',(-8.27600348990041,1.20454703673242,10.8122408161699));
#13526=CARTESIAN_POINT('Ctrl Pts',(-7.97209482032083,1.10563290540104,10.8002376293806));
#13527=CARTESIAN_POINT('Ctrl Pts',(-7.74204705372053,0.915087963996507,
10.7882344425913));
#13528=CARTESIAN_POINT('Ctrl Pts',(-7.51199928712023,0.72454302259197,10.776231255802));
#13529=CARTESIAN_POINT('Ctrl Pts',(-7.35822688079631,0.444367128061372,
10.7642280690127));
#13530=CARTESIAN_POINT('Ctrl Pts',(-7.32102560975816,0.147979855990197,
10.7522248822234));
#13531=CARTESIAN_POINT('Ctrl Pts',(-7.28382433872001,-0.148407416080977,
10.740221695434));
#13532=CARTESIAN_POINT('Ctrl Pts',(-7.3635846474464,-0.45789534472205,10.7282185086447));
#13533=CARTESIAN_POINT('Ctrl Pts',(-7.53940549437888,-0.699383189957773,
10.7162153218554));
#13534=CARTESIAN_POINT('Ctrl Pts',(-7.71522634131135,-0.940871035193497,
10.7042121350661));
#13535=CARTESIAN_POINT('Ctrl Pts',(-7.98526240565793,-1.11182427083086,
10.6922089482768));
#13536=CARTESIAN_POINT('Ctrl Pts',(-8.27875123560126,-1.16744491727748,
10.6802057614874));
#13537=CARTESIAN_POINT('Ctrl Pts',(-8.57224006554459,-1.2230655637241,10.6682025746981));
#13538=CARTESIAN_POINT('Ctrl Pts',(-8.88610136059949,-1.16276985667021,
10.6561993879088));
#13539=CARTESIAN_POINT('Ctrl Pts',(-9.13808834820101,-1.00235817476344,
10.6441962011195));
#13540=CARTESIAN_POINT('Ctrl Pts',(-9.39007533580253,-0.841946492856677,
10.6321930143302));
#13541=CARTESIAN_POINT('Ctrl Pts',(-9.57754329642141,-0.583102430602837,
10.6201898275409));
#13542=CARTESIAN_POINT('Ctrl Pts',(-9.65136659729193,-0.293655596346135,
10.6081866407515));
#13543=CARTESIAN_POINT('Ctrl Pts',(-9.67581103310544,-0.197813707972407,
10.6042121350661));
#13544=CARTESIAN_POINT('Ctrl Pts',(-9.68822500000001,-0.0989100500922724,
10.6002376293806));
#13545=CARTESIAN_POINT('Ctrl Pts',(-9.688225,1.37778677355982E-13,10.5962631236952));
#13546=CARTESIAN_POINT('Ctrl Pts',(-9.688225,-1.61320956593158E-12,10.5537368763049));
#13547=CARTESIAN_POINT('Ctrl Pts',(-9.68822499999959,-0.298712821307707,
10.5657400630942));
#13548=CARTESIAN_POINT('Ctrl Pts',(-9.57054245632505,-0.595858078272982,
10.5777432498835));
#13549=CARTESIAN_POINT('Ctrl Pts',(-9.36601586214824,-0.813569405233895,
10.5897464366729));
#13550=CARTESIAN_POINT('Ctrl Pts',(-9.16148926797144,-1.03128073219481,
10.6017496234622));
#13551=CARTESIAN_POINT('Ctrl Pts',(-8.87226522412688,-1.16727314847186,
10.6137528102515));
#13552=CARTESIAN_POINT('Ctrl Pts',(-8.57413435701289,-1.185910092602,10.6257559970408));
#13553=CARTESIAN_POINT('Ctrl Pts',(-8.27600348989891,-1.20454703673214,
10.6377591838301));
#13554=CARTESIAN_POINT('Ctrl Pts',(-7.97209482031945,-1.10563290540038,
10.6497623706194));
#13555=CARTESIAN_POINT('Ctrl Pts',(-7.74204705371939,-0.915087963995561,
10.6617655574088));
#13556=CARTESIAN_POINT('Ctrl Pts',(-7.51199928711932,-0.724543022590736,
10.6737687441981));
#13557=CARTESIAN_POINT('Ctrl Pts',(-7.35822688079575,-0.444367128059946,
10.6857719309874));
#13558=CARTESIAN_POINT('Ctrl Pts',(-7.32102560975797,-0.147979855988725,
10.6977751177767));
#13559=CARTESIAN_POINT('Ctrl Pts',(-7.2838243387202,0.148407416082496,10.709778304566));
#13560=CARTESIAN_POINT('Ctrl Pts',(-7.36358464744697,0.457895344723468,
10.7217814913554));
#13561=CARTESIAN_POINT('Ctrl Pts',(-7.53940549437975,0.699383189958973,
10.7337846781447));
#13562=CARTESIAN_POINT('Ctrl Pts',(-7.71522634131253,0.940871035194477,
10.745787864934));
#13563=CARTESIAN_POINT('Ctrl Pts',(-7.98526240565931,1.11182427083151,10.7577910517233));
#13564=CARTESIAN_POINT('Ctrl Pts',(-8.27875123560271,1.16744491727776,10.7697942385126));
#13565=CARTESIAN_POINT('Ctrl Pts',(-8.57224006554612,1.22306556372401,10.7817974253019));
#13566=CARTESIAN_POINT('Ctrl Pts',(-8.88610136060094,1.16276985666973,10.7938006120913));
#13567=CARTESIAN_POINT('Ctrl Pts',(-9.13808834820226,1.00235817476265,10.8058037988806));
#13568=CARTESIAN_POINT('Ctrl Pts',(-9.39007533580358,0.841946492855566,
10.8178069856699));
#13569=CARTESIAN_POINT('Ctrl Pts',(-9.57754329642214,0.583102430601491,
10.8298101724592));
#13570=CARTESIAN_POINT('Ctrl Pts',(-9.6513665972923,0.293655596344697,10.8418133592485));
#13571=CARTESIAN_POINT('Ctrl Pts',(-9.67581103310569,0.19781370797095,10.845787864934));
#13572=CARTESIAN_POINT('Ctrl Pts',(-9.68822500000013,0.0989100500908113,
10.8497623706194));
#13573=CARTESIAN_POINT('Ctrl Pts',(-9.688225,-1.58756341406274E-12,10.8537368763049));
#13574=CARTESIAN_POINT('Origin',(-8.5,0.,1.8));
#13575=CARTESIAN_POINT('',(-9.688225,1.55320201145059E-13,11.1962631236952));
#13576=CARTESIAN_POINT('',(-9.688225,-1.59577906444497E-12,11.1537368763049));
#13577=CARTESIAN_POINT('',(-9.688225,-1.45515594291686E-16,1.8));
#13578=CARTESIAN_POINT('Ctrl Pts',(-9.688225,1.55320201145059E-13,11.1962631236952));
#13579=CARTESIAN_POINT('Ctrl Pts',(-9.68822499999996,0.29871282130626,11.1842599369059));
#13580=CARTESIAN_POINT('Ctrl Pts',(-9.57054245632577,0.595858078271691,
11.1722567501165));
#13581=CARTESIAN_POINT('Ctrl Pts',(-9.36601586214922,0.813569405232857,
11.1602535633272));
#13582=CARTESIAN_POINT('Ctrl Pts',(-9.16148926797266,1.03128073219402,11.1482503765379));
#13583=CARTESIAN_POINT('Ctrl Pts',(-8.87226522412826,1.16727314847143,11.1362471897486));
#13584=CARTESIAN_POINT('Ctrl Pts',(-8.57413435701428,1.18591009260191,11.1242440029593));
#13585=CARTESIAN_POINT('Ctrl Pts',(-8.27600348990031,1.2045470367324,11.1122408161699));
#13586=CARTESIAN_POINT('Ctrl Pts',(-7.97209482032072,1.105632905401,11.1002376293806));
#13587=CARTESIAN_POINT('Ctrl Pts',(-7.74204705372043,0.915087963996426,
11.0882344425913));
#13588=CARTESIAN_POINT('Ctrl Pts',(-7.51199928712014,0.724543022591858,
11.076231255802));
#13589=CARTESIAN_POINT('Ctrl Pts',(-7.35822688079625,0.444367128061229,
11.0642280690127));
#13590=CARTESIAN_POINT('Ctrl Pts',(-7.32102560975814,0.147979855990038,
11.0522248822234));
#13591=CARTESIAN_POINT('Ctrl Pts',(-7.28382433872003,-0.148407416081153,
11.040221695434));
#13592=CARTESIAN_POINT('Ctrl Pts',(-7.36358464744647,-0.457895344722227,
11.0282185086447));
#13593=CARTESIAN_POINT('Ctrl Pts',(-7.53940549437899,-0.699383189957931,
11.0162153218554));
#13594=CARTESIAN_POINT('Ctrl Pts',(-7.71522634131151,-0.940871035193635,
11.0042121350661));
#13595=CARTESIAN_POINT('Ctrl Pts',(-7.98526240565813,-1.11182427083096,
10.9922089482768));
#13596=CARTESIAN_POINT('Ctrl Pts',(-8.27875123560148,-1.16744491727753,
10.9802057614874));
#13597=CARTESIAN_POINT('Ctrl Pts',(-8.57224006554484,-1.22306556372409,
10.9682025746981));
#13598=CARTESIAN_POINT('Ctrl Pts',(-8.88610136059974,-1.16276985667013,
10.9561993879088));
#13599=CARTESIAN_POINT('Ctrl Pts',(-9.13808834820123,-1.0023581747633,10.9441962011195));
#13600=CARTESIAN_POINT('Ctrl Pts',(-9.39007533580273,-0.841946492856475,
10.9321930143302));
#13601=CARTESIAN_POINT('Ctrl Pts',(-9.57754329642155,-0.583102430602579,
10.9201898275408));
#13602=CARTESIAN_POINT('Ctrl Pts',(-9.651366597292,-0.293655596345848,10.9081866407515));
#13603=CARTESIAN_POINT('Ctrl Pts',(-9.67581103310547,-0.197813707972213,
10.9042121350661));
#13604=CARTESIAN_POINT('Ctrl Pts',(-9.68822500000001,-0.0989100500921791,
10.9002376293806));
#13605=CARTESIAN_POINT('Ctrl Pts',(-9.688225,1.29674049276218E-13,10.8962631236952));
#13606=CARTESIAN_POINT('Ctrl Pts',(-9.688225,-1.58756341406274E-12,10.8537368763049));
#13607=CARTESIAN_POINT('Ctrl Pts',(-9.6882249999996,-0.298712821307681,
10.8657400630942));
#13608=CARTESIAN_POINT('Ctrl Pts',(-9.57054245632506,-0.595858078272959,
10.8777432498835));
#13609=CARTESIAN_POINT('Ctrl Pts',(-9.36601586214826,-0.813569405233876,
10.8897464366729));
#13610=CARTESIAN_POINT('Ctrl Pts',(-9.16148926797146,-1.03128073219479,
10.9017496234622));
#13611=CARTESIAN_POINT('Ctrl Pts',(-8.8722652241269,-1.16727314847185,10.9137528102515));
#13612=CARTESIAN_POINT('Ctrl Pts',(-8.57413435701292,-1.185910092602,10.9257559970408));
#13613=CARTESIAN_POINT('Ctrl Pts',(-8.27600348989893,-1.20454703673214,
10.9377591838301));
#13614=CARTESIAN_POINT('Ctrl Pts',(-7.97209482031948,-1.1056329054004,10.9497623706194));
#13615=CARTESIAN_POINT('Ctrl Pts',(-7.74204705371941,-0.915087963995577,
10.9617655574088));
#13616=CARTESIAN_POINT('Ctrl Pts',(-7.51199928711934,-0.724543022590758,
10.9737687441981));
#13617=CARTESIAN_POINT('Ctrl Pts',(-7.35822688079576,-0.444367128059971,
10.9857719309874));
#13618=CARTESIAN_POINT('Ctrl Pts',(-7.32102560975798,-0.147979855988751,
10.9977751177767));
#13619=CARTESIAN_POINT('Ctrl Pts',(-7.2838243387202,0.148407416082469,11.009778304566));
#13620=CARTESIAN_POINT('Ctrl Pts',(-7.36358464744696,0.457895344723444,
11.0217814913554));
#13621=CARTESIAN_POINT('Ctrl Pts',(-7.53940549437974,0.699383189958952,
11.0337846781447));
#13622=CARTESIAN_POINT('Ctrl Pts',(-7.71522634131251,0.94087103519446,11.045787864934));
#13623=CARTESIAN_POINT('Ctrl Pts',(-7.98526240565929,1.11182427083149,11.0577910517233));
#13624=CARTESIAN_POINT('Ctrl Pts',(-8.27875123560269,1.16744491727775,11.0697942385126));
#13625=CARTESIAN_POINT('Ctrl Pts',(-8.57224006554609,1.22306556372402,11.0817974253019));
#13626=CARTESIAN_POINT('Ctrl Pts',(-8.88610136060092,1.16276985666974,11.0938006120913));
#13627=CARTESIAN_POINT('Ctrl Pts',(-9.13808834820224,1.00235817476266,11.1058037988806));
#13628=CARTESIAN_POINT('Ctrl Pts',(-9.39007533580356,0.841946492855585,
11.1178069856699));
#13629=CARTESIAN_POINT('Ctrl Pts',(-9.57754329642212,0.583102430601514,
11.1298101724592));
#13630=CARTESIAN_POINT('Ctrl Pts',(-9.65136659729229,0.293655596344722,
11.1418133592485));
#13631=CARTESIAN_POINT('Ctrl Pts',(-9.67581103310568,0.197813707970976,
11.145787864934));
#13632=CARTESIAN_POINT('Ctrl Pts',(-9.68822500000013,0.0989100500908369,
11.1497623706194));
#13633=CARTESIAN_POINT('Ctrl Pts',(-9.688225,-1.56197277334513E-12,11.1537368763049));
#13634=CARTESIAN_POINT('Origin',(-8.5,0.,1.8));
#13635=CARTESIAN_POINT('',(-9.688225,1.80966353013901E-13,11.4962631236952));
#13636=CARTESIAN_POINT('',(-9.688225,-1.57013291257613E-12,11.4537368763049));
#13637=CARTESIAN_POINT('',(-9.688225,-1.45515594291686E-16,1.8));
#13638=CARTESIAN_POINT('Ctrl Pts',(-9.688225,1.80966353013901E-13,11.4962631236952));
#13639=CARTESIAN_POINT('Ctrl Pts',(-9.68822499999995,0.298712821306286,
11.4842599369059));
#13640=CARTESIAN_POINT('Ctrl Pts',(-9.57054245632576,0.595858078271714,
11.4722567501165));
#13641=CARTESIAN_POINT('Ctrl Pts',(-9.3660158621492,0.813569405232876,11.4602535633272));
#13642=CARTESIAN_POINT('Ctrl Pts',(-9.16148926797264,1.03128073219404,11.4482503765379));
#13643=CARTESIAN_POINT('Ctrl Pts',(-8.87226522412823,1.16727314847143,11.4362471897486));
#13644=CARTESIAN_POINT('Ctrl Pts',(-8.57413435701426,1.18591009260192,11.4242440029593));
#13645=CARTESIAN_POINT('Ctrl Pts',(-8.27600348990028,1.2045470367324,11.4122408161699));
#13646=CARTESIAN_POINT('Ctrl Pts',(-7.9720948203207,1.10563290540098,11.4002376293806));
#13647=CARTESIAN_POINT('Ctrl Pts',(-7.74204705372041,0.91508796399641,11.3882344425913));
#13648=CARTESIAN_POINT('Ctrl Pts',(-7.51199928712013,0.724543022591836,
11.376231255802));
#13649=CARTESIAN_POINT('Ctrl Pts',(-7.35822688079624,0.444367128061204,
11.3642280690127));
#13650=CARTESIAN_POINT('Ctrl Pts',(-7.32102560975814,0.147979855990013,
11.3522248822234));
#13651=CARTESIAN_POINT('Ctrl Pts',(-7.28382433872004,-0.148407416081179,
11.340221695434));
#13652=CARTESIAN_POINT('Ctrl Pts',(-7.36358464744648,-0.457895344722251,
11.3282185086447));
#13653=CARTESIAN_POINT('Ctrl Pts',(-7.53940549437901,-0.699383189957951,
11.3162153218554));
#13654=CARTESIAN_POINT('Ctrl Pts',(-7.71522634131153,-0.940871035193652,
11.3042121350661));
#13655=CARTESIAN_POINT('Ctrl Pts',(-7.98526240565815,-1.11182427083097,
11.2922089482768));
#13656=CARTESIAN_POINT('Ctrl Pts',(-8.27875123560151,-1.16744491727753,
11.2802057614874));
#13657=CARTESIAN_POINT('Ctrl Pts',(-8.57224006554486,-1.22306556372409,
11.2682025746981));
#13658=CARTESIAN_POINT('Ctrl Pts',(-8.88610136059977,-1.16276985667013,
11.2561993879088));
#13659=CARTESIAN_POINT('Ctrl Pts',(-9.13808834820125,-1.00235817476329,
11.2441962011195));
#13660=CARTESIAN_POINT('Ctrl Pts',(-9.39007533580274,-0.841946492856455,
11.2321930143302));
#13661=CARTESIAN_POINT('Ctrl Pts',(-9.57754329642156,-0.583102430602556,
11.2201898275408));
#13662=CARTESIAN_POINT('Ctrl Pts',(-9.65136659729201,-0.293655596345824,
11.2081866407515));
#13663=CARTESIAN_POINT('Ctrl Pts',(-9.67581103310547,-0.197813707972188,
11.2042121350661));
#13664=CARTESIAN_POINT('Ctrl Pts',(-9.68822500000001,-0.0989100500921535,
11.2002376293806));
#13665=CARTESIAN_POINT('Ctrl Pts',(-9.688225,1.55320201145059E-13,11.1962631236952));
#13666=CARTESIAN_POINT('Ctrl Pts',(-9.688225,-1.56197277334513E-12,11.1537368763049));
#13667=CARTESIAN_POINT('Ctrl Pts',(-9.68822499999961,-0.298712821307667,
11.1657400630942));
#13668=CARTESIAN_POINT('Ctrl Pts',(-9.57054245632507,-0.595858078272958,
11.1777432498835));
#13669=CARTESIAN_POINT('Ctrl Pts',(-9.36601586214826,-0.813569405233882,
11.1897464366729));
#13670=CARTESIAN_POINT('Ctrl Pts',(-9.16148926797144,-1.03128073219481,
11.2017496234622));
#13671=CARTESIAN_POINT('Ctrl Pts',(-8.87226522412687,-1.16727314847187,
11.2137528102515));
#13672=CARTESIAN_POINT('Ctrl Pts',(-8.57413435701288,-1.185910092602,11.2257559970408));
#13673=CARTESIAN_POINT('Ctrl Pts',(-8.27600348989888,-1.20454703673214,
11.2377591838301));
#13674=CARTESIAN_POINT('Ctrl Pts',(-7.97209482031942,-1.10563290540037,
11.2497623706194));
#13675=CARTESIAN_POINT('Ctrl Pts',(-7.74204705371935,-0.915087963995529,
11.2617655574088));
#13676=CARTESIAN_POINT('Ctrl Pts',(-7.51199928711928,-0.724543022590688,
11.2737687441981));
#13677=CARTESIAN_POINT('Ctrl Pts',(-7.35822688079572,-0.444367128059877,
11.2857719309874));
#13678=CARTESIAN_POINT('Ctrl Pts',(-7.32102560975796,-0.147979855988642,
11.2977751177767));
#13679=CARTESIAN_POINT('Ctrl Pts',(-7.28382433872021,0.148407416082593,
11.309778304566));
#13680=CARTESIAN_POINT('Ctrl Pts',(-7.36358464744701,0.457895344723572,
11.3217814913554));
#13681=CARTESIAN_POINT('Ctrl Pts',(-7.53940549437982,0.699383189959068,
11.3337846781447));
#13682=CARTESIAN_POINT('Ctrl Pts',(-7.71522634131263,0.940871035194563,
11.345787864934));
#13683=CARTESIAN_POINT('Ctrl Pts',(-7.98526240565944,1.11182427083157,11.3577910517233));
#13684=CARTESIAN_POINT('Ctrl Pts',(-8.27875123560286,1.16744491727779,11.3697942385126));
#13685=CARTESIAN_POINT('Ctrl Pts',(-8.57224006554628,1.22306556372401,11.381797425302));
#13686=CARTESIAN_POINT('Ctrl Pts',(-8.88610136060112,1.16276985666968,11.3938006120913));
#13687=CARTESIAN_POINT('Ctrl Pts',(-9.13808834820242,1.00235817476255,11.4058037988806));
#13688=CARTESIAN_POINT('Ctrl Pts',(-9.39007533580372,0.841946492855421,
11.4178069856699));
#13689=CARTESIAN_POINT('Ctrl Pts',(-9.57754329642224,0.583102430601303,
11.4298101724592));
#13690=CARTESIAN_POINT('Ctrl Pts',(-9.65136659729235,0.293655596344485,
11.4418133592485));
#13691=CARTESIAN_POINT('Ctrl Pts',(-9.6758110331057,0.19781370797081,11.445787864934));
#13692=CARTESIAN_POINT('Ctrl Pts',(-9.68822500000013,0.0989100500907499,
11.4497623706194));
#13693=CARTESIAN_POINT('Ctrl Pts',(-9.688225,-1.57013291257613E-12,11.4537368763049));
#13694=CARTESIAN_POINT('Origin',(-8.5,0.,1.8));
#13695=CARTESIAN_POINT('',(-9.688225,2.06501482580279E-13,11.7962631236952));
#13696=CARTESIAN_POINT('',(-9.688225,-1.54454227185852E-12,11.7537368763049));
#13697=CARTESIAN_POINT('',(-9.688225,-1.45515594291686E-16,1.8));
#13698=CARTESIAN_POINT('Ctrl Pts',(-9.688225,2.06501482580279E-13,11.7962631236952));
#13699=CARTESIAN_POINT('Ctrl Pts',(-9.68822499999995,0.298712821306311,
11.7842599369059));
#13700=CARTESIAN_POINT('Ctrl Pts',(-9.57054245632575,0.595858078271737,
11.7722567501165));
#13701=CARTESIAN_POINT('Ctrl Pts',(-9.36601586214918,0.813569405232895,
11.7602535633272));
#13702=CARTESIAN_POINT('Ctrl Pts',(-9.16148926797262,1.03128073219405,11.7482503765379));
#13703=CARTESIAN_POINT('Ctrl Pts',(-8.8722652241282,1.16727314847144,11.7362471897486));
#13704=CARTESIAN_POINT('Ctrl Pts',(-8.57413435701423,1.18591009260192,11.7242440029593));
#13705=CARTESIAN_POINT('Ctrl Pts',(-8.27600348990026,1.20454703673239,11.7122408161699));
#13706=CARTESIAN_POINT('Ctrl Pts',(-7.97209482032068,1.10563290540097,11.7002376293806));
#13707=CARTESIAN_POINT('Ctrl Pts',(-7.74204705372039,0.915087963996394,
11.6882344425913));
#13708=CARTESIAN_POINT('Ctrl Pts',(-7.51199928712011,0.724543022591815,
11.676231255802));
#13709=CARTESIAN_POINT('Ctrl Pts',(-7.35822688079623,0.44436712806118,11.6642280690127));
#13710=CARTESIAN_POINT('Ctrl Pts',(-7.32102560975813,0.147979855989987,
11.6522248822233));
#13711=CARTESIAN_POINT('Ctrl Pts',(-7.28382433872004,-0.148407416081205,
11.640221695434));
#13712=CARTESIAN_POINT('Ctrl Pts',(-7.36358464744649,-0.457895344722276,
11.6282185086447));
#13713=CARTESIAN_POINT('Ctrl Pts',(-7.53940549437902,-0.699383189957972,
11.6162153218554));
#13714=CARTESIAN_POINT('Ctrl Pts',(-7.71522634131155,-0.940871035193668,
11.6042121350661));
#13715=CARTESIAN_POINT('Ctrl Pts',(-7.98526240565817,-1.11182427083098,
11.5922089482768));
#13716=CARTESIAN_POINT('Ctrl Pts',(-8.27875123560153,-1.16744491727754,
11.5802057614874));
#13717=CARTESIAN_POINT('Ctrl Pts',(-8.57224006554489,-1.22306556372409,
11.5682025746981));
#13718=CARTESIAN_POINT('Ctrl Pts',(-8.88610136059979,-1.16276985667012,
11.5561993879088));
#13719=CARTESIAN_POINT('Ctrl Pts',(-9.13808834820128,-1.00235817476328,
11.5441962011195));
#13720=CARTESIAN_POINT('Ctrl Pts',(-9.39007533580276,-0.841946492856436,
11.5321930143302));
#13721=CARTESIAN_POINT('Ctrl Pts',(-9.57754329642158,-0.583102430602533,
11.5201898275408));
#13722=CARTESIAN_POINT('Ctrl Pts',(-9.65136659729202,-0.293655596345799,
11.5081866407515));
#13723=CARTESIAN_POINT('Ctrl Pts',(-9.67581103310548,-0.197813707972162,
11.5042121350661));
#13724=CARTESIAN_POINT('Ctrl Pts',(-9.68822500000002,-0.0989100500921278,
11.5002376293806));
#13725=CARTESIAN_POINT('Ctrl Pts',(-9.688225,1.80966353013901E-13,11.4962631236952));
#13726=CARTESIAN_POINT('Ctrl Pts',(-9.688225,-1.57013291257613E-12,11.4537368763049));
#13727=CARTESIAN_POINT('Ctrl Pts',(-9.6882249999996,-0.298712821307664,
11.4657400630942));
#13728=CARTESIAN_POINT('Ctrl Pts',(-9.57054245632507,-0.595858078272943,
11.4777432498835));
#13729=CARTESIAN_POINT('Ctrl Pts',(-9.36601586214827,-0.813569405233864,
11.4897464366729));
#13730=CARTESIAN_POINT('Ctrl Pts',(-9.16148926797147,-1.03128073219478,
11.5017496234622));
#13731=CARTESIAN_POINT('Ctrl Pts',(-8.87226522412692,-1.16727314847185,
11.5137528102515));
#13732=CARTESIAN_POINT('Ctrl Pts',(-8.57413435701294,-1.185910092602,11.5257559970408));
#13733=CARTESIAN_POINT('Ctrl Pts',(-8.27600348989895,-1.20454703673215,
11.5377591838301));
#13734=CARTESIAN_POINT('Ctrl Pts',(-7.97209482031949,-1.1056329054004,11.5497623706194));
#13735=CARTESIAN_POINT('Ctrl Pts',(-7.74204705371942,-0.915087963995588,
11.5617655574088));
#13736=CARTESIAN_POINT('Ctrl Pts',(-7.51199928711935,-0.724543022590772,
11.5737687441981));
#13737=CARTESIAN_POINT('Ctrl Pts',(-7.35822688079577,-0.444367128059988,
11.5857719309874));
#13738=CARTESIAN_POINT('Ctrl Pts',(-7.32102560975798,-0.147979855988768,
11.5977751177767));
#13739=CARTESIAN_POINT('Ctrl Pts',(-7.28382433872019,0.148407416082451,
11.609778304566));
#13740=CARTESIAN_POINT('Ctrl Pts',(-7.36358464744696,0.457895344723427,
11.6217814913554));
#13741=CARTESIAN_POINT('Ctrl Pts',(-7.53940549437973,0.699383189958938,
11.6337846781447));
#13742=CARTESIAN_POINT('Ctrl Pts',(-7.71522634131249,0.940871035194448,
11.645787864934));
#13743=CARTESIAN_POINT('Ctrl Pts',(-7.98526240565927,1.11182427083149,11.6577910517233));
#13744=CARTESIAN_POINT('Ctrl Pts',(-8.27875123560267,1.16744491727775,11.6697942385126));
#13745=CARTESIAN_POINT('Ctrl Pts',(-8.57224006554607,1.22306556372402,11.6817974253019));
#13746=CARTESIAN_POINT('Ctrl Pts',(-8.8861013606009,1.16276985666974,11.6938006120913));
#13747=CARTESIAN_POINT('Ctrl Pts',(-9.13808834820223,1.00235817476267,11.7058037988806));
#13748=CARTESIAN_POINT('Ctrl Pts',(-9.39007533580355,0.841946492855598,
11.7178069856699));
#13749=CARTESIAN_POINT('Ctrl Pts',(-9.57754329642211,0.58310243060153,11.7298101724592));
#13750=CARTESIAN_POINT('Ctrl Pts',(-9.65136659729228,0.293655596344739,
11.7418133592485));
#13751=CARTESIAN_POINT('Ctrl Pts',(-9.67581103310568,0.197813707970993,
11.745787864934));
#13752=CARTESIAN_POINT('Ctrl Pts',(-9.68822500000013,0.0989100500908544,
11.7497623706194));
#13753=CARTESIAN_POINT('Ctrl Pts',(-9.688225,-1.54454227185852E-12,11.7537368763049));
#13754=CARTESIAN_POINT('Origin',(-8.5,0.,1.8));
#13755=CARTESIAN_POINT('',(-9.688225,2.3214763444912E-13,12.0962631236952));
#13756=CARTESIAN_POINT('',(-9.688225,-1.51884060883845E-12,12.0537368763049));
#13757=CARTESIAN_POINT('',(-9.688225,-1.45515594291686E-16,1.8));
#13758=CARTESIAN_POINT('Ctrl Pts',(-9.688225,2.3214763444912E-13,12.0962631236952));
#13759=CARTESIAN_POINT('Ctrl Pts',(-9.68822499999994,0.298712821306314,
12.0842599369059));
#13760=CARTESIAN_POINT('Ctrl Pts',(-9.57054245632575,0.595858078271716,
12.0722567501165));
#13761=CARTESIAN_POINT('Ctrl Pts',(-9.36601586214921,0.813569405232864,
12.0602535633272));
#13762=CARTESIAN_POINT('Ctrl Pts',(-9.16148926797267,1.03128073219401,12.0482503765379));
#13763=CARTESIAN_POINT('Ctrl Pts',(-8.87226522412829,1.16727314847141,12.0362471897486));
#13764=CARTESIAN_POINT('Ctrl Pts',(-8.57413435701434,1.18591009260191,12.0242440029593));
#13765=CARTESIAN_POINT('Ctrl Pts',(-8.27600348990039,1.20454703673241,12.0122408161699));
#13766=CARTESIAN_POINT('Ctrl Pts',(-7.97209482032082,1.10563290540104,12.0002376293806));
#13767=CARTESIAN_POINT('Ctrl Pts',(-7.74204705372053,0.915087963996507,
11.9882344425913));
#13768=CARTESIAN_POINT('Ctrl Pts',(-7.51199928712024,0.724543022591976,
11.976231255802));
#13769=CARTESIAN_POINT('Ctrl Pts',(-7.35822688079632,0.444367128061392,
11.9642280690127));
#13770=CARTESIAN_POINT('Ctrl Pts',(-7.32102560975816,0.14797985599023,11.9522248822234));
#13771=CARTESIAN_POINT('Ctrl Pts',(-7.28382433872001,-0.148407416080933,
11.940221695434));
#13772=CARTESIAN_POINT('Ctrl Pts',(-7.36358464744638,-0.457895344721995,
11.9282185086447));
#13773=CARTESIAN_POINT('Ctrl Pts',(-7.53940549437884,-0.69938318995772,
11.9162153218554));
#13774=CARTESIAN_POINT('Ctrl Pts',(-7.71522634131129,-0.940871035193444,
11.9042121350661));
#13775=CARTESIAN_POINT('Ctrl Pts',(-7.98526240565784,-1.11182427083082,
11.8922089482768));
#13776=CARTESIAN_POINT('Ctrl Pts',(-8.27875123560116,-1.16744491727747,
11.8802057614875));
#13777=CARTESIAN_POINT('Ctrl Pts',(-8.57224006554447,-1.22306556372411,
11.8682025746981));
#13778=CARTESIAN_POINT('Ctrl Pts',(-8.88610136059937,-1.16276985667025,
11.8561993879088));
#13779=CARTESIAN_POINT('Ctrl Pts',(-9.1380883482009,-1.00235817476352,11.8441962011195));
#13780=CARTESIAN_POINT('Ctrl Pts',(-9.39007533580243,-0.841946492856783,
11.8321930143302));
#13781=CARTESIAN_POINT('Ctrl Pts',(-9.57754329642133,-0.583102430602978,
11.8201898275409));
#13782=CARTESIAN_POINT('Ctrl Pts',(-9.65136659729189,-0.293655596346298,
11.8081866407515));
#13783=CARTESIAN_POINT('Ctrl Pts',(-9.67581103310544,-0.197813707972497,
11.8042121350661));
#13784=CARTESIAN_POINT('Ctrl Pts',(-9.68822500000002,-0.0989100500922825,
11.8002376293806));
#13785=CARTESIAN_POINT('Ctrl Pts',(-9.688225,2.06501482580279E-13,11.7962631236952));
#13786=CARTESIAN_POINT('Ctrl Pts',(-9.688225,-1.54454227185852E-12,11.7537368763049));
#13787=CARTESIAN_POINT('Ctrl Pts',(-9.68822499999961,-0.298712821307638,
11.7657400630942));
#13788=CARTESIAN_POINT('Ctrl Pts',(-9.57054245632509,-0.59585807827292,
11.7777432498835));
#13789=CARTESIAN_POINT('Ctrl Pts',(-9.36601586214829,-0.813569405233845,
11.7897464366729));
#13790=CARTESIAN_POINT('Ctrl Pts',(-9.1614892679715,-1.03128073219477,11.8017496234622));
#13791=CARTESIAN_POINT('Ctrl Pts',(-8.87226522412695,-1.16727314847184,
11.8137528102515));
#13792=CARTESIAN_POINT('Ctrl Pts',(-8.57413435701296,-1.185910092602,11.8257559970408));
#13793=CARTESIAN_POINT('Ctrl Pts',(-8.27600348989898,-1.20454703673215,
11.8377591838301));
#13794=CARTESIAN_POINT('Ctrl Pts',(-7.97209482031952,-1.10563290540042,
11.8497623706194));
#13795=CARTESIAN_POINT('Ctrl Pts',(-7.74204705371944,-0.915087963995605,
11.8617655574088));
#13796=CARTESIAN_POINT('Ctrl Pts',(-7.51199928711937,-0.724543022590794,
11.8737687441981));
#13797=CARTESIAN_POINT('Ctrl Pts',(-7.35822688079578,-0.444367128060013,
11.8857719309874));
#13798=CARTESIAN_POINT('Ctrl Pts',(-7.32102560975798,-0.147979855988794,
11.8977751177767));
#13799=CARTESIAN_POINT('Ctrl Pts',(-7.28382433872019,0.148407416082425,
11.909778304566));
#13800=CARTESIAN_POINT('Ctrl Pts',(-7.36358464744695,0.457895344723403,
11.9217814913554));
#13801=CARTESIAN_POINT('Ctrl Pts',(-7.53940549437971,0.699383189958917,
11.9337846781447));
#13802=CARTESIAN_POINT('Ctrl Pts',(-7.71522634131247,0.940871035194431,
11.945787864934));
#13803=CARTESIAN_POINT('Ctrl Pts',(-7.98526240565925,1.11182427083148,11.9577910517233));
#13804=CARTESIAN_POINT('Ctrl Pts',(-8.27875123560265,1.16744491727775,11.9697942385126));
#13805=CARTESIAN_POINT('Ctrl Pts',(-8.57224006554604,1.22306556372402,11.9817974253019));
#13806=CARTESIAN_POINT('Ctrl Pts',(-8.88610136060088,1.16276985666975,11.9938006120913));
#13807=CARTESIAN_POINT('Ctrl Pts',(-9.13808834820221,1.00235817476268,12.0058037988806));
#13808=CARTESIAN_POINT('Ctrl Pts',(-9.39007533580353,0.841946492855617,
12.0178069856699));
#13809=CARTESIAN_POINT('Ctrl Pts',(-9.5775432964221,0.583102430601553,12.0298101724592));
#13810=CARTESIAN_POINT('Ctrl Pts',(-9.65136659729228,0.293655596344764,
12.0418133592485));
#13811=CARTESIAN_POINT('Ctrl Pts',(-9.67581103310568,0.197813707971018,
12.045787864934));
#13812=CARTESIAN_POINT('Ctrl Pts',(-9.68822500000013,0.0989100500908801,
12.0497623706194));
#13813=CARTESIAN_POINT('Ctrl Pts',(-9.688225,-1.51884060883845E-12,12.0537368763049));
#13814=CARTESIAN_POINT('Origin',(-8.5,0.,1.8));
#13815=CARTESIAN_POINT('',(-9.68878804160158,0.000373206645753347,12.3962631236952));
#13816=CARTESIAN_POINT('',(-9.688225,-1.49330547927207E-12,12.3537368763049));
#13817=CARTESIAN_POINT('',(-9.688225,-1.45515594291686E-16,1.8));
#13818=CARTESIAN_POINT('Ctrl Pts',(-9.688225,2.23931984066894E-13,12.3962631236952));
#13819=CARTESIAN_POINT('Ctrl Pts',(-9.68822499999994,0.298712821306317,
12.3842599369059));
#13820=CARTESIAN_POINT('Ctrl Pts',(-9.57054245632575,0.595858078271731,
12.3722567501165));
#13821=CARTESIAN_POINT('Ctrl Pts',(-9.3660158621492,0.813569405232883,12.3602535633272));
#13822=CARTESIAN_POINT('Ctrl Pts',(-9.16148926797264,1.03128073219403,12.3482503765379));
#13823=CARTESIAN_POINT('Ctrl Pts',(-8.87226522412824,1.16727314847143,12.3362471897486));
#13824=CARTESIAN_POINT('Ctrl Pts',(-8.57413435701428,1.18591009260191,12.3242440029593));
#13825=CARTESIAN_POINT('Ctrl Pts',(-8.27600348990032,1.2045470367324,12.3122408161699));
#13826=CARTESIAN_POINT('Ctrl Pts',(-7.97209482032075,1.105632905401,12.3002376293806));
#13827=CARTESIAN_POINT('Ctrl Pts',(-7.74204705372046,0.915087963996447,
12.2882344425913));
#13828=CARTESIAN_POINT('Ctrl Pts',(-7.51199928712017,0.724543022591892,
12.276231255802));
#13829=CARTESIAN_POINT('Ctrl Pts',(-7.35822688079627,0.444367128061282,
12.2642280690127));
#13830=CARTESIAN_POINT('Ctrl Pts',(-7.32102560975815,0.147979855990104,
12.2522248822234));
#13831=CARTESIAN_POINT('Ctrl Pts',(-7.28382433872002,-0.148407416081074,
12.240221695434));
#13832=CARTESIAN_POINT('Ctrl Pts',(-7.36358464744644,-0.45789534472214,
12.2282185086447));
#13833=CARTESIAN_POINT('Ctrl Pts',(-7.53940549437893,-0.69938318995785,
12.2162153218554));
#13834=CARTESIAN_POINT('Ctrl Pts',(-7.71522634131143,-0.940871035193559,
12.2042121350661));
#13835=CARTESIAN_POINT('Ctrl Pts',(-7.98526240565801,-1.1118242708309,12.1922089482768));
#13836=CARTESIAN_POINT('Ctrl Pts',(-8.27875123560135,-1.1674449172775,12.1802057614874));
#13837=CARTESIAN_POINT('Ctrl Pts',(-8.57224006554469,-1.2230655637241,12.1682025746981));
#13838=CARTESIAN_POINT('Ctrl Pts',(-8.88610136059958,-1.16276985667018,
12.1561993879088));
#13839=CARTESIAN_POINT('Ctrl Pts',(-9.13808834820109,-1.00235817476339,
12.1441962011195));
#13840=CARTESIAN_POINT('Ctrl Pts',(-9.3900753358026,-0.841946492856606,
12.1321930143302));
#13841=CARTESIAN_POINT('Ctrl Pts',(-9.57754329642145,-0.583102430602751,
12.1201898275409));
#13842=CARTESIAN_POINT('Ctrl Pts',(-9.65136659729195,-0.293655596346044,
12.1081866407515));
#13843=CARTESIAN_POINT('Ctrl Pts',(-9.67581103310546,-0.197813707972314,
12.1042121350661));
#13844=CARTESIAN_POINT('Ctrl Pts',(-9.68822500000002,-0.098910050092178,
12.1002376293806));
#13845=CARTESIAN_POINT('Ctrl Pts',(-9.688225,2.3214763444912E-13,12.0962631236952));
#13846=CARTESIAN_POINT('Ctrl Pts',(-9.688225,-1.51884060883845E-12,12.0537368763049));
#13847=CARTESIAN_POINT('Ctrl Pts',(-9.68822499999962,-0.298712821307624,
12.0657400630942));
#13848=CARTESIAN_POINT('Ctrl Pts',(-9.57054245632509,-0.595858078272919,
12.0777432498835));
#13849=CARTESIAN_POINT('Ctrl Pts',(-9.36601586214829,-0.813569405233851,
12.0897464366729));
#13850=CARTESIAN_POINT('Ctrl Pts',(-9.16148926797148,-1.03128073219478,
12.1017496234622));
#13851=CARTESIAN_POINT('Ctrl Pts',(-8.87226522412692,-1.16727314847185,
12.1137528102515));
#13852=CARTESIAN_POINT('Ctrl Pts',(-8.57413435701292,-1.185910092602,12.1257559970408));
#13853=CARTESIAN_POINT('Ctrl Pts',(-8.27600348989893,-1.20454703673215,
12.1377591838301));
#13854=CARTESIAN_POINT('Ctrl Pts',(-7.97209482031946,-1.10563290540039,
12.1497623706194));
#13855=CARTESIAN_POINT('Ctrl Pts',(-7.74204705371938,-0.915087963995556,
12.1617655574088));
#13856=CARTESIAN_POINT('Ctrl Pts',(-7.51199928711931,-0.724543022590723,
12.1737687441981));
#13857=CARTESIAN_POINT('Ctrl Pts',(-7.35822688079574,-0.444367128059919,
12.1857719309874));
#13858=CARTESIAN_POINT('Ctrl Pts',(-7.32102560975797,-0.147979855988685,
12.1977751177767));
#13859=CARTESIAN_POINT('Ctrl Pts',(-7.2838243387202,0.148407416082549,12.209778304566));
#13860=CARTESIAN_POINT('Ctrl Pts',(-7.36358464744699,0.457895344723531,
12.2217814913554));
#13861=CARTESIAN_POINT('Ctrl Pts',(-7.53940549437979,0.699383189959033,
12.2337846781447));
#13862=CARTESIAN_POINT('Ctrl Pts',(-7.71522634131259,0.940871035194535,
12.245787864934));
#13863=CARTESIAN_POINT('Ctrl Pts',(-7.9852624056594,1.11182427083155,12.2577910517233));
#13864=CARTESIAN_POINT('Ctrl Pts',(-8.27875123560282,1.16744491727778,12.2697942385126));
#13865=CARTESIAN_POINT('Ctrl Pts',(-8.57224006554624,1.22306556372401,12.2817974253019));
#13866=CARTESIAN_POINT('Ctrl Pts',(-8.88610136060107,1.16276985666969,12.2938006120913));
#13867=CARTESIAN_POINT('Ctrl Pts',(-9.13808834820238,1.00235817476257,12.3058037988806));
#13868=CARTESIAN_POINT('Ctrl Pts',(-9.39007533580369,0.841946492855453,
12.3178069856699));
#13869=CARTESIAN_POINT('Ctrl Pts',(-9.57754329642222,0.583102430601342,
12.3298101724592));
#13870=CARTESIAN_POINT('Ctrl Pts',(-9.65136659729234,0.293655596344527,
12.3418133592485));
#13871=CARTESIAN_POINT('Ctrl Pts',(-9.6758110331057,0.197813707970863,12.345787864934));
#13872=CARTESIAN_POINT('Ctrl Pts',(-9.68822500000012,0.0989100500908155,
12.3497623706194));
#13873=CARTESIAN_POINT('Ctrl Pts',(-9.688225,-1.49330547927207E-12,12.3537368763049));
#13874=CARTESIAN_POINT('Origin',(-8.5,0.,1.8));
#13875=CARTESIAN_POINT('',(-9.68731827199145,0.000299612246693184,12.6962631236952));
#13876=CARTESIAN_POINT('',(-9.688225,-1.46765932740323E-12,12.6537368763049));
#13877=CARTESIAN_POINT('',(-9.688225,-1.45515594291686E-16,1.8));
#13878=CARTESIAN_POINT('Ctrl Pts',(-9.68662866502971,0.000527480679553827,
12.6962631236952));
#13879=CARTESIAN_POINT('Ctrl Pts',(-9.68740960275973,0.161591526755359,
12.6898105777584));
#13880=CARTESIAN_POINT('Ctrl Pts',(-9.65693800757816,0.322407861474271,
12.6833580318217));
#13881=CARTESIAN_POINT('Ctrl Pts',(-9.59386268769377,0.469313525857254,
12.676905485885));
#13882=CARTESIAN_POINT('Ctrl Pts',(-9.43836427799808,0.831477320328926,
12.6609981447334));
#13883=CARTESIAN_POINT('Ctrl Pts',(-9.08471307556792,1.10909745603158,12.6450908035818));
#13884=CARTESIAN_POINT('Ctrl Pts',(-8.69629196213472,1.17401378965972,12.6291834624301));
#13885=CARTESIAN_POINT('Ctrl Pts',(-8.30787084870153,1.23893012328785,12.6132761212785));
#13886=CARTESIAN_POINT('Ctrl Pts',(-7.88467982426531,1.09114265484149,12.5973687801269));
#13887=CARTESIAN_POINT('Ctrl Pts',(-7.6190606764032,0.799649543688172,12.5814614389753));
#13888=CARTESIAN_POINT('Ctrl Pts',(-7.48625110247213,0.653902988111497,
12.5735077683995));
#13889=CARTESIAN_POINT('Ctrl Pts',(-7.39283449768459,0.472230021858075,
12.5655540978237));
#13890=CARTESIAN_POINT('Ctrl Pts',(-7.34613116947634,0.279251812905948,
12.5576004272478));
#13891=CARTESIAN_POINT('Ctrl Pts',(-7.29942784126808,0.0862736039538323,
12.549646756672));
#13892=CARTESIAN_POINT('Ctrl Pts',(-7.2994377896391,-0.118009847696987,
12.5416930860962));
#13893=CARTESIAN_POINT('Ctrl Pts',(-7.35090869635395,-0.308354763973108,
12.5337394155204));
#13894=CARTESIAN_POINT('Ctrl Pts',(-7.45385050978364,-0.689044596525339,
12.5178320743688));
#13895=CARTESIAN_POINT('Ctrl Pts',(-7.76263615658864,-1.01398028757878,
12.5019247332172));
#13896=CARTESIAN_POINT('Ctrl Pts',(-8.13775744624663,-1.13385150921984,
12.4860173920656));
#13897=CARTESIAN_POINT('Ctrl Pts',(-8.51287873590465,-1.2537227308609,12.4701100509139));
#13898=CARTESIAN_POINT('Ctrl Pts',(-8.95433566841568,-1.16852948308955,
12.4542027097623));
#13899=CARTESIAN_POINT('Ctrl Pts',(-9.25822456392514,-0.917543609722033,
12.4382953686107));
#13900=CARTESIAN_POINT('Ctrl Pts',(-9.52588153985455,-0.696482159767021,
12.4242846203055));
#13901=CARTESIAN_POINT('Ctrl Pts',(-9.6868187133487,-0.346805396004457,
12.4102738720003));
#13902=CARTESIAN_POINT('Ctrl Pts',(-9.68938150757543,0.000766579790317107,
12.3962631236952));
#13903=CARTESIAN_POINT('Ctrl Pts',(-9.688225,-1.49330547927207E-12,12.3537368763049));
#13904=CARTESIAN_POINT('Ctrl Pts',(-9.68822499999962,-0.298712821307587,
12.3657400630942));
#13905=CARTESIAN_POINT('Ctrl Pts',(-9.57054245632511,-0.595858078272874,
12.3777432498835));
#13906=CARTESIAN_POINT('Ctrl Pts',(-9.36601586214833,-0.813569405233808,
12.3897464366729));
#13907=CARTESIAN_POINT('Ctrl Pts',(-9.16148926797154,-1.03128073219474,
12.4017496234622));
#13908=CARTESIAN_POINT('Ctrl Pts',(-8.872265224127,-1.16727314847182,12.4137528102515));
#13909=CARTESIAN_POINT('Ctrl Pts',(-8.57413435701301,-1.18591009260199,
12.4257559970408));
#13910=CARTESIAN_POINT('Ctrl Pts',(-8.27600348989903,-1.20454703673216,
12.4377591838301));
#13911=CARTESIAN_POINT('Ctrl Pts',(-7.97209482031957,-1.10563290540044,
12.4497623706194));
#13912=CARTESIAN_POINT('Ctrl Pts',(-7.74204705371948,-0.915087963995637,
12.4617655574088));
#13913=CARTESIAN_POINT('Ctrl Pts',(-7.5119992871194,-0.724543022590836,
12.4737687441981));
#13914=CARTESIAN_POINT('Ctrl Pts',(-7.3582268807958,-0.444367128060062,
12.4857719309874));
#13915=CARTESIAN_POINT('Ctrl Pts',(-7.32102560975799,-0.147979855988844,
12.4977751177767));
#13916=CARTESIAN_POINT('Ctrl Pts',(-7.28382433872018,0.148407416082373,
12.509778304566));
#13917=CARTESIAN_POINT('Ctrl Pts',(-7.36358464744693,0.457895344723354,
12.5217814913554));
#13918=CARTESIAN_POINT('Ctrl Pts',(-7.53940549437968,0.699383189958875,
12.5337846781447));
#13919=CARTESIAN_POINT('Ctrl Pts',(-7.71522634131243,0.940871035194397,
12.545787864934));
#13920=CARTESIAN_POINT('Ctrl Pts',(-7.9852624056592,1.11182427083145,12.5577910517233));
#13921=CARTESIAN_POINT('Ctrl Pts',(-8.2787512356026,1.16744491727774,12.5697942385126));
#13922=CARTESIAN_POINT('Ctrl Pts',(-8.57224006554599,1.22306556372402,12.5817974253019));
#13923=CARTESIAN_POINT('Ctrl Pts',(-8.88610136060083,1.16276985666977,12.5938006120913));
#13924=CARTESIAN_POINT('Ctrl Pts',(-9.13808834820216,1.00235817476271,12.6058037988806));
#13925=CARTESIAN_POINT('Ctrl Pts',(-9.3900753358035,0.841946492855655,12.6178069856699));
#13926=CARTESIAN_POINT('Ctrl Pts',(-9.57754329642207,0.5831024306016,12.6298101724592));
#13927=CARTESIAN_POINT('Ctrl Pts',(-9.65136659729227,0.293655596344814,
12.6418133592485));
#13928=CARTESIAN_POINT('Ctrl Pts',(-9.67581103310567,0.19781370797108,12.645787864934));
#13929=CARTESIAN_POINT('Ctrl Pts',(-9.68822500000012,0.0989100500909537,
12.6497623706194));
#13930=CARTESIAN_POINT('Ctrl Pts',(-9.688225,-1.43385303630339E-12,12.6537368763049));
#13931=CARTESIAN_POINT('Origin',(-8.5,0.,1.8));
#13932=CARTESIAN_POINT('',(-9.688225,3.08975067753181E-13,12.9962631236952));
#13933=CARTESIAN_POINT('',(-9.688225,-1.44201317553438E-12,12.9537368763049));
#13934=CARTESIAN_POINT('',(-9.688225,-1.45515594291686E-16,1.8));
#13935=CARTESIAN_POINT('Ctrl Pts',(-9.688225,3.42836870004248E-13,12.9962631236952));
#13936=CARTESIAN_POINT('Ctrl Pts',(-9.68822499999991,0.298712821306448,
12.9842599369058));
#13937=CARTESIAN_POINT('Ctrl Pts',(-9.57054245632568,0.59585807827186,12.9722567501165));
#13938=CARTESIAN_POINT('Ctrl Pts',(-9.36601586214909,0.813569405232994,
12.9602535633272));
#13939=CARTESIAN_POINT('Ctrl Pts',(-9.1614892679725,1.03128073219413,12.9482503765379));
#13940=CARTESIAN_POINT('Ctrl Pts',(-8.87226522412807,1.16727314847148,12.9362471897486));
#13941=CARTESIAN_POINT('Ctrl Pts',(-8.57413435701409,1.18591009260193,12.9242440029593));
#13942=CARTESIAN_POINT('Ctrl Pts',(-8.27600348990012,1.20454703673237,12.9122408161699));
#13943=CARTESIAN_POINT('Ctrl Pts',(-7.97209482032055,1.10563290540091,12.9002376293806));
#13944=CARTESIAN_POINT('Ctrl Pts',(-7.74204705372029,0.915087963996307,
12.8882344425913));
#13945=CARTESIAN_POINT('Ctrl Pts',(-7.51199928712003,0.724543022591702,
12.876231255802));
#13946=CARTESIAN_POINT('Ctrl Pts',(-7.35822688079618,0.444367128061049,
12.8642280690127));
#13947=CARTESIAN_POINT('Ctrl Pts',(-7.32102560975812,0.147979855989852,
12.8522248822233));
#13948=CARTESIAN_POINT('Ctrl Pts',(-7.28382433872005,-0.148407416081345,
12.840221695434));
#13949=CARTESIAN_POINT('Ctrl Pts',(-7.36358464744654,-0.457895344722406,
12.8282185086447));
#13950=CARTESIAN_POINT('Ctrl Pts',(-7.5394054943791,-0.699383189958082,
12.8162153218554));
#13951=CARTESIAN_POINT('Ctrl Pts',(-7.71522634131166,-0.940871035193758,
12.8042121350661));
#13952=CARTESIAN_POINT('Ctrl Pts',(-7.9852624056583,-1.11182427083104,12.7922089482768));
#13953=CARTESIAN_POINT('Ctrl Pts',(-8.27875123560167,-1.16744491727756,
12.7802057614874));
#13954=CARTESIAN_POINT('Ctrl Pts',(-8.57224006554503,-1.22306556372408,
12.7682025746981));
#13955=CARTESIAN_POINT('Ctrl Pts',(-8.88610136059992,-1.16276985667007,
12.7561993879088));
#13956=CARTESIAN_POINT('Ctrl Pts',(-9.13808834820139,-1.0023581747632,12.7441962011195));
#13957=CARTESIAN_POINT('Ctrl Pts',(-9.39007533580286,-0.841946492856334,
12.7321930143302));
#13958=CARTESIAN_POINT('Ctrl Pts',(-9.57754329642164,-0.583102430602409,
12.7201898275408));
#13959=CARTESIAN_POINT('Ctrl Pts',(-9.65136659729205,-0.293655596345667,
12.7081866407515));
#13960=CARTESIAN_POINT('Ctrl Pts',(-9.6758110331055,-0.197813707972038,
12.7042121350661));
#13961=CARTESIAN_POINT('Ctrl Pts',(-9.68822500000002,-0.0989100500920141,
12.7002376293806));
#13962=CARTESIAN_POINT('Ctrl Pts',(-9.688225,2.83439938186802E-13,12.6962631236952));
#13963=CARTESIAN_POINT('Ctrl Pts',(-9.688225,-1.43385303630339E-12,12.6537368763049));
#13964=CARTESIAN_POINT('Ctrl Pts',(-9.68822499999964,-0.298712821307539,
12.6657400630942));
#13965=CARTESIAN_POINT('Ctrl Pts',(-9.57054245632513,-0.595858078272843,
12.6777432498835));
#13966=CARTESIAN_POINT('Ctrl Pts',(-9.36601586214834,-0.813569405233789,
12.6897464366729));
#13967=CARTESIAN_POINT('Ctrl Pts',(-9.16148926797156,-1.03128073219474,
12.7017496234622));
#13968=CARTESIAN_POINT('Ctrl Pts',(-8.872265224127,-1.16727314847183,12.7137528102515));
#13969=CARTESIAN_POINT('Ctrl Pts',(-8.574134357013,-1.18591009260199,12.7257559970408));
#13970=CARTESIAN_POINT('Ctrl Pts',(-8.27600348989901,-1.20454703673216,
12.7377591838301));
#13971=CARTESIAN_POINT('Ctrl Pts',(-7.97209482031954,-1.10563290540043,
12.7497623706194));
#13972=CARTESIAN_POINT('Ctrl Pts',(-7.74204705371945,-0.91508796399561,
12.7617655574088));
#13973=CARTESIAN_POINT('Ctrl Pts',(-7.51199928711936,-0.724543022590794,
12.7737687441981));
#13974=CARTESIAN_POINT('Ctrl Pts',(-7.35822688079577,-0.44436712806,12.7857719309874));
#13975=CARTESIAN_POINT('Ctrl Pts',(-7.32102560975798,-0.147979855988769,
12.7977751177767));
#13976=CARTESIAN_POINT('Ctrl Pts',(-7.28382433872019,0.148407416082461,
12.809778304566));
#13977=CARTESIAN_POINT('Ctrl Pts',(-7.36358464744696,0.457895344723449,
12.8217814913554));
#13978=CARTESIAN_POINT('Ctrl Pts',(-7.53940549437974,0.699383189958964,
12.8337846781447));
#13979=CARTESIAN_POINT('Ctrl Pts',(-7.71522634131253,0.940871035194479,
12.845787864934));
#13980=CARTESIAN_POINT('Ctrl Pts',(-7.98526240565932,1.11182427083151,12.8577910517233));
#13981=CARTESIAN_POINT('Ctrl Pts',(-8.27875123560274,1.16744491727776,12.8697942385126));
#13982=CARTESIAN_POINT('Ctrl Pts',(-8.57224006554615,1.22306556372401,12.8817974253019));
#13983=CARTESIAN_POINT('Ctrl Pts',(-8.88610136060099,1.16276985666972,12.8938006120913));
#13984=CARTESIAN_POINT('Ctrl Pts',(-9.13808834820231,1.00235817476262,12.9058037988806));
#13985=CARTESIAN_POINT('Ctrl Pts',(-9.39007533580363,0.841946492855517,
12.9178069856699));
#13986=CARTESIAN_POINT('Ctrl Pts',(-9.57754329642218,0.583102430601419,
12.9298101724592));
#13987=CARTESIAN_POINT('Ctrl Pts',(-9.65136659729232,0.293655596344609,
12.9418133592485));
#13988=CARTESIAN_POINT('Ctrl Pts',(-9.67581103310568,0.197813707970937,
12.945787864934));
#13989=CARTESIAN_POINT('Ctrl Pts',(-9.68822500000012,0.098910050090878,
12.9497623706194));
#13990=CARTESIAN_POINT('Ctrl Pts',(-9.688225,-1.44201317553438E-12,12.9537368763049));
#13991=CARTESIAN_POINT('Origin',(-8.5,0.,1.8));
#13992=CARTESIAN_POINT('',(-9.688225,3.34621219622022E-13,13.2962631236952));
#13993=CARTESIAN_POINT('',(-9.688225,-1.41642253481677E-12,13.2537368763049));
#13994=CARTESIAN_POINT('',(-9.688225,-1.45515594291686E-16,1.8));
#13995=CARTESIAN_POINT('Ctrl Pts',(-9.688225,3.34621219622022E-13,13.2962631236952));
#13996=CARTESIAN_POINT('Ctrl Pts',(-9.68822499999992,0.298712821306428,
13.2842599369058));
#13997=CARTESIAN_POINT('Ctrl Pts',(-9.57054245632569,0.59585807827183,13.2722567501165));
#13998=CARTESIAN_POINT('Ctrl Pts',(-9.36601586214912,0.813569405232963,
13.2602535633272));
#13999=CARTESIAN_POINT('Ctrl Pts',(-9.16148926797255,1.0312807321941,13.2482503765379));
#14000=CARTESIAN_POINT('Ctrl Pts',(-8.87226522412814,1.16727314847146,13.2362471897486));
#14001=CARTESIAN_POINT('Ctrl Pts',(-8.57413435701417,1.18591009260192,13.2242440029593));
#14002=CARTESIAN_POINT('Ctrl Pts',(-8.27600348990021,1.20454703673238,13.2122408161699));
#14003=CARTESIAN_POINT('Ctrl Pts',(-7.97209482032064,1.10563290540095,13.2002376293806));
#14004=CARTESIAN_POINT('Ctrl Pts',(-7.74204705372037,0.915087963996377,
13.1882344425913));
#14005=CARTESIAN_POINT('Ctrl Pts',(-7.5119992871201,0.7245430225918,13.176231255802));
#14006=CARTESIAN_POINT('Ctrl Pts',(-7.35822688079623,0.444367128061175,
13.1642280690127));
#14007=CARTESIAN_POINT('Ctrl Pts',(-7.32102560975813,0.147979855989994,
13.1522248822233));
#14008=CARTESIAN_POINT('Ctrl Pts',(-7.28382433872004,-0.148407416081187,
13.140221695434));
#14009=CARTESIAN_POINT('Ctrl Pts',(-7.36358464744648,-0.457895344722246,
13.1282185086447));
#14010=CARTESIAN_POINT('Ctrl Pts',(-7.539405494379,-0.699383189957939,13.1162153218554));
#14011=CARTESIAN_POINT('Ctrl Pts',(-7.71522634131152,-0.940871035193632,
13.1042121350661));
#14012=CARTESIAN_POINT('Ctrl Pts',(-7.98526240565812,-1.11182427083095,
13.0922089482768));
#14013=CARTESIAN_POINT('Ctrl Pts',(-8.27875123560146,-1.16744491727752,
13.0802057614874));
#14014=CARTESIAN_POINT('Ctrl Pts',(-8.5722400655448,-1.22306556372409,13.0682025746981));
#14015=CARTESIAN_POINT('Ctrl Pts',(-8.88610136059969,-1.16276985667015,
13.0561993879088));
#14016=CARTESIAN_POINT('Ctrl Pts',(-9.13808834820118,-1.00235817476333,
13.0441962011195));
#14017=CARTESIAN_POINT('Ctrl Pts',(-9.39007533580268,-0.841946492856523,
13.0321930143302));
#14018=CARTESIAN_POINT('Ctrl Pts',(-9.57754329642151,-0.583102430602651,
13.0201898275409));
#14019=CARTESIAN_POINT('Ctrl Pts',(-9.65136659729198,-0.293655596345937,
13.0081866407515));
#14020=CARTESIAN_POINT('Ctrl Pts',(-9.67581103310548,-0.197813707972205,
13.0042121350661));
#14021=CARTESIAN_POINT('Ctrl Pts',(-9.68822500000003,-0.0989100500920673,
13.0002376293806));
#14022=CARTESIAN_POINT('Ctrl Pts',(-9.688225,3.42836870004248E-13,12.9962631236952));
#14023=CARTESIAN_POINT('Ctrl Pts',(-9.688225,-1.44201317553438E-12,12.9537368763049));
#14024=CARTESIAN_POINT('Ctrl Pts',(-9.68822499999964,-0.298712821307535,
12.9657400630942));
#14025=CARTESIAN_POINT('Ctrl Pts',(-9.57054245632514,-0.595858078272828,
12.9777432498835));
#14026=CARTESIAN_POINT('Ctrl Pts',(-9.36601586214836,-0.81356940523377,
12.9897464366729));
#14027=CARTESIAN_POINT('Ctrl Pts',(-9.16148926797158,-1.03128073219471,
13.0017496234622));
#14028=CARTESIAN_POINT('Ctrl Pts',(-8.87226522412705,-1.16727314847181,
13.0137528102515));
#14029=CARTESIAN_POINT('Ctrl Pts',(-8.57413435701307,-1.18591009260199,
13.0257559970408));
#14030=CARTESIAN_POINT('Ctrl Pts',(-8.27600348989908,-1.20454703673217,
13.0377591838301));
#14031=CARTESIAN_POINT('Ctrl Pts',(-7.97209482031961,-1.10563290540046,
13.0497623706194));
#14032=CARTESIAN_POINT('Ctrl Pts',(-7.74204705371952,-0.91508796399567,
13.0617655574088));
#14033=CARTESIAN_POINT('Ctrl Pts',(-7.51199928711943,-0.724543022590879,
13.0737687441981));
#14034=CARTESIAN_POINT('Ctrl Pts',(-7.35822688079581,-0.444367128060111,
13.0857719309874));
#14035=CARTESIAN_POINT('Ctrl Pts',(-7.321025609758,-0.147979855988895,13.0977751177767));
#14036=CARTESIAN_POINT('Ctrl Pts',(-7.28382433872018,0.14840741608232,13.109778304566));
#14037=CARTESIAN_POINT('Ctrl Pts',(-7.36358464744691,0.457895344723305,
13.1217814913553));
#14038=CARTESIAN_POINT('Ctrl Pts',(-7.53940549437965,0.699383189958834,
13.1337846781447));
#14039=CARTESIAN_POINT('Ctrl Pts',(-7.71522634131239,0.940871035194364,
13.145787864934));
#14040=CARTESIAN_POINT('Ctrl Pts',(-7.98526240565915,1.11182427083143,13.1577910517233));
#14041=CARTESIAN_POINT('Ctrl Pts',(-8.27875123560255,1.16744491727773,13.1697942385126));
#14042=CARTESIAN_POINT('Ctrl Pts',(-8.57224006554594,1.22306556372402,13.1817974253019));
#14043=CARTESIAN_POINT('Ctrl Pts',(-8.88610136060078,1.16276985666979,13.1938006120913));
#14044=CARTESIAN_POINT('Ctrl Pts',(-9.13808834820212,1.00235817476274,13.2058037988806));
#14045=CARTESIAN_POINT('Ctrl Pts',(-9.39007533580346,0.841946492855694,
13.2178069856699));
#14046=CARTESIAN_POINT('Ctrl Pts',(-9.57754329642205,0.583102430601646,
13.2298101724592));
#14047=CARTESIAN_POINT('Ctrl Pts',(-9.65136659729225,0.293655596344863,
13.2418133592485));
#14048=CARTESIAN_POINT('Ctrl Pts',(-9.67581103310566,0.19781370797112,13.245787864934));
#14049=CARTESIAN_POINT('Ctrl Pts',(-9.68822500000012,0.0989100500909825,
13.2497623706194));
#14050=CARTESIAN_POINT('Ctrl Pts',(-9.688225,-1.41642253481677E-12,13.2537368763049));
#14051=CARTESIAN_POINT('Origin',(-8.5,0.,1.8));
#14052=CARTESIAN_POINT('',(-9.688225,3.60267371490863E-13,13.5962631236952));
#14053=CARTESIAN_POINT('',(-9.688225,-1.39083189409916E-12,13.5537368763049));
#14054=CARTESIAN_POINT('',(-9.688225,-1.45515594291686E-16,1.8));
#14055=CARTESIAN_POINT('Ctrl Pts',(-9.688225,3.93907129137006E-13,13.5962631236952));
#14056=CARTESIAN_POINT('Ctrl Pts',(-9.6882249999999,0.29871282130651,13.5842599369058));
#14057=CARTESIAN_POINT('Ctrl Pts',(-9.57054245632564,0.595858078271928,
13.5722567501165));
#14058=CARTESIAN_POINT('Ctrl Pts',(-9.36601586214903,0.813569405233056,
13.5602535633272));
#14059=CARTESIAN_POINT('Ctrl Pts',(-9.16148926797242,1.03128073219418,13.5482503765379));
#14060=CARTESIAN_POINT('Ctrl Pts',(-8.87226522412797,1.16727314847152,13.5362471897486));
#14061=CARTESIAN_POINT('Ctrl Pts',(-8.57413435701398,1.18591009260193,13.5242440029592));
#14062=CARTESIAN_POINT('Ctrl Pts',(-8.27600348989999,1.20454703673235,13.5122408161699));
#14063=CARTESIAN_POINT('Ctrl Pts',(-7.97209482032042,1.10563290540085,13.5002376293806));
#14064=CARTESIAN_POINT('Ctrl Pts',(-7.74204705372017,0.91508796399621,13.4882344425913));
#14065=CARTESIAN_POINT('Ctrl Pts',(-7.51199928711992,0.724543022591568,
13.476231255802));
#14066=CARTESIAN_POINT('Ctrl Pts',(-7.35822688079611,0.444367128060881,
13.4642280690127));
#14067=CARTESIAN_POINT('Ctrl Pts',(-7.32102560975809,0.147979855989667,
13.4522248822233));
#14068=CARTESIAN_POINT('Ctrl Pts',(-7.28382433872008,-0.148407416081547,
13.440221695434));
#14069=CARTESIAN_POINT('Ctrl Pts',(-7.36358464744662,-0.457895344722607,
13.4282185086447));
#14070=CARTESIAN_POINT('Ctrl Pts',(-7.53940549437923,-0.69938318995826,
13.4162153218554));
#14071=CARTESIAN_POINT('Ctrl Pts',(-7.71522634131184,-0.940871035193913,
13.4042121350661));
#14072=CARTESIAN_POINT('Ctrl Pts',(-7.98526240565853,-1.11182427083115,
13.3922089482767));
#14073=CARTESIAN_POINT('Ctrl Pts',(-8.27875123560191,-1.16744491727761,
13.3802057614874));
#14074=CARTESIAN_POINT('Ctrl Pts',(-8.5722400655453,-1.22306556372407,13.3682025746981));
#14075=CARTESIAN_POINT('Ctrl Pts',(-8.8861013606002,-1.16276985666999,13.3561993879088));
#14076=CARTESIAN_POINT('Ctrl Pts',(-9.13808834820163,-1.00235817476305,
13.3441962011195));
#14077=CARTESIAN_POINT('Ctrl Pts',(-9.39007533580307,-0.841946492856113,
13.3321930143301));
#14078=CARTESIAN_POINT('Ctrl Pts',(-9.5775432964218,-0.583102430602129,
13.3201898275408));
#14079=CARTESIAN_POINT('Ctrl Pts',(-9.65136659729213,-0.293655596345355,
13.3081866407515));
#14080=CARTESIAN_POINT('Ctrl Pts',(-9.67581103310553,-0.197813707971808,
13.3042121350661));
#14081=CARTESIAN_POINT('Ctrl Pts',(-9.68822500000003,-0.0989100500918729,
13.3002376293806));
#14082=CARTESIAN_POINT('Ctrl Pts',(-9.688225,3.34621219622022E-13,13.2962631236952));
#14083=CARTESIAN_POINT('Ctrl Pts',(-9.688225,-1.41642253481677E-12,13.2537368763049));
#14084=CARTESIAN_POINT('Ctrl Pts',(-9.68822499999964,-0.298712821307499,
13.2657400630942));
#14085=CARTESIAN_POINT('Ctrl Pts',(-9.57054245632516,-0.595858078272782,
13.2777432498835));
#14086=CARTESIAN_POINT('Ctrl Pts',(-9.3660158621484,-0.813569405233727,
13.2897464366728));
#14087=CARTESIAN_POINT('Ctrl Pts',(-9.16148926797164,-1.03128073219467,
13.3017496234622));
#14088=CARTESIAN_POINT('Ctrl Pts',(-8.87226522412713,-1.16727314847178,
13.3137528102515));
#14089=CARTESIAN_POINT('Ctrl Pts',(-8.57413435701316,-1.18591009260198,
13.3257559970408));
#14090=CARTESIAN_POINT('Ctrl Pts',(-8.27600348989919,-1.20454703673219,
13.3377591838301));
#14091=CARTESIAN_POINT('Ctrl Pts',(-7.97209482031972,-1.10563290540051,
13.3497623706194));
#14092=CARTESIAN_POINT('Ctrl Pts',(-7.74204705371962,-0.915087963995751,
13.3617655574088));
#14093=CARTESIAN_POINT('Ctrl Pts',(-7.51199928711951,-0.724543022590991,
13.3737687441981));
#14094=CARTESIAN_POINT('Ctrl Pts',(-7.35822688079587,-0.444367128060254,
13.3857719309874));
#14095=CARTESIAN_POINT('Ctrl Pts',(-7.32102560975802,-0.147979855989055,
13.3977751177767));
#14096=CARTESIAN_POINT('Ctrl Pts',(-7.28382433872016,0.148407416082145,
13.409778304566));
#14097=CARTESIAN_POINT('Ctrl Pts',(-7.36358464744684,0.457895344723128,
13.4217814913553));
#14098=CARTESIAN_POINT('Ctrl Pts',(-7.53940549437953,0.699383189958677,
13.4337846781447));
#14099=CARTESIAN_POINT('Ctrl Pts',(-7.71522634131223,0.940871035194226,
13.445787864934));
#14100=CARTESIAN_POINT('Ctrl Pts',(-7.98526240565895,1.11182427083133,13.4577910517233));
#14101=CARTESIAN_POINT('Ctrl Pts',(-8.27875123560232,1.16744491727769,13.4697942385126));
#14102=CARTESIAN_POINT('Ctrl Pts',(-8.57224006554569,1.22306556372404,13.4817974253019));
#14103=CARTESIAN_POINT('Ctrl Pts',(-8.88610136060053,1.16276985666987,13.4938006120912));
#14104=CARTESIAN_POINT('Ctrl Pts',(-9.1380883482019,1.00235817476288,13.5058037988806));
#14105=CARTESIAN_POINT('Ctrl Pts',(-9.39007533580327,0.841946492855896,
13.5178069856699));
#14106=CARTESIAN_POINT('Ctrl Pts',(-9.57754329642191,0.583102430601903,
13.5298101724592));
#14107=CARTESIAN_POINT('Ctrl Pts',(-9.65136659729218,0.29365559634515,13.5418133592485));
#14108=CARTESIAN_POINT('Ctrl Pts',(-9.67581103310563,0.197813707971336,
13.545787864934));
#14109=CARTESIAN_POINT('Ctrl Pts',(-9.68822500000011,0.0989100500911206,
13.5497623706194));
#14110=CARTESIAN_POINT('Ctrl Pts',(-9.688225,-1.35702560299933E-12,13.5537368763049));
#14111=CARTESIAN_POINT('Origin',(-8.5,0.,1.8));
#14112=CARTESIAN_POINT('',(-9.688225,3.85913523359704E-13,13.8962631236952));
#14113=CARTESIAN_POINT('',(-9.6873777234388,-0.000235261270365428,13.8537368763049));
#14114=CARTESIAN_POINT('',(-9.688225,-1.45515594291686E-16,1.8));
#14115=CARTESIAN_POINT('Ctrl Pts',(-9.688225,4.53415083256914E-13,13.8962631236952));
#14116=CARTESIAN_POINT('Ctrl Pts',(-9.68822499999989,0.298712821306558,
13.8842599369058));
#14117=CARTESIAN_POINT('Ctrl Pts',(-9.57054245632563,0.595858078271959,
13.8722567501165));
#14118=CARTESIAN_POINT('Ctrl Pts',(-9.36601586214902,0.813569405233075,
13.8602535633272));
#14119=CARTESIAN_POINT('Ctrl Pts',(-9.16148926797241,1.03128073219419,13.8482503765379));
#14120=CARTESIAN_POINT('Ctrl Pts',(-8.87226522412796,1.16727314847152,13.8362471897486));
#14121=CARTESIAN_POINT('Ctrl Pts',(-8.57413435701398,1.18591009260193,13.8242440029592));
#14122=CARTESIAN_POINT('Ctrl Pts',(-8.2760034899,1.20454703673235,13.8122408161699));
#14123=CARTESIAN_POINT('Ctrl Pts',(-7.97209482032045,1.10563290540086,13.8002376293806));
#14124=CARTESIAN_POINT('Ctrl Pts',(-7.7420470537202,0.915087963996236,13.7882344425913));
#14125=CARTESIAN_POINT('Ctrl Pts',(-7.51199928711996,0.72454302259161,13.776231255802));
#14126=CARTESIAN_POINT('Ctrl Pts',(-7.35822688079613,0.444367128060942,
13.7642280690127));
#14127=CARTESIAN_POINT('Ctrl Pts',(-7.3210256097581,0.147979855989742,13.7522248822233));
#14128=CARTESIAN_POINT('Ctrl Pts',(-7.28382433872007,-0.148407416081458,
13.740221695434));
#14129=CARTESIAN_POINT('Ctrl Pts',(-7.36358464744658,-0.457895344722512,
13.7282185086447));
#14130=CARTESIAN_POINT('Ctrl Pts',(-7.53940549437917,-0.699383189958172,
13.7162153218554));
#14131=CARTESIAN_POINT('Ctrl Pts',(-7.71522634131175,-0.940871035193831,
13.7042121350661));
#14132=CARTESIAN_POINT('Ctrl Pts',(-7.98526240565841,-1.11182427083109,
13.6922089482767));
#14133=CARTESIAN_POINT('Ctrl Pts',(-8.27875123560177,-1.16744491727758,
13.6802057614874));
#14134=CARTESIAN_POINT('Ctrl Pts',(-8.57224006554514,-1.22306556372407,
13.6682025746981));
#14135=CARTESIAN_POINT('Ctrl Pts',(-8.88610136060003,-1.16276985667004,
13.6561993879088));
#14136=CARTESIAN_POINT('Ctrl Pts',(-9.13808834820149,-1.00235817476314,
13.6441962011195));
#14137=CARTESIAN_POINT('Ctrl Pts',(-9.39007533580294,-0.841946492856251,
13.6321930143302));
#14138=CARTESIAN_POINT('Ctrl Pts',(-9.57754329642169,-0.583102430602309,
13.6201898275408));
#14139=CARTESIAN_POINT('Ctrl Pts',(-9.65136659729208,-0.29365559634556,
13.6081866407515));
#14140=CARTESIAN_POINT('Ctrl Pts',(-9.67581103310551,-0.197813707971929,
13.6042121350661));
#14141=CARTESIAN_POINT('Ctrl Pts',(-9.68822500000003,-0.0989100500919037,
13.6002376293806));
#14142=CARTESIAN_POINT('Ctrl Pts',(-9.688225,3.93907129137006E-13,13.5962631236952));
#14143=CARTESIAN_POINT('Ctrl Pts',(-9.688225,-1.35702560299933E-12,13.5537368763049));
#14144=CARTESIAN_POINT('Ctrl Pts',(-9.68822499999966,-0.298712821307417,
13.5657400630942));
#14145=CARTESIAN_POINT('Ctrl Pts',(-9.57054245632521,-0.595858078272685,
13.5777432498835));
#14146=CARTESIAN_POINT('Ctrl Pts',(-9.36601586214849,-0.813569405233634,
13.5897464366728));
#14147=CARTESIAN_POINT('Ctrl Pts',(-9.16148926797177,-1.03128073219458,
13.6017496234622));
#14148=CARTESIAN_POINT('Ctrl Pts',(-8.8722652241273,-1.16727314847172,13.6137528102515));
#14149=CARTESIAN_POINT('Ctrl Pts',(-8.57413435701335,-1.18591009260197,
13.6257559970408));
#14150=CARTESIAN_POINT('Ctrl Pts',(-8.27600348989941,-1.20454703673222,
13.6377591838301));
#14151=CARTESIAN_POINT('Ctrl Pts',(-7.97209482031995,-1.10563290540061,
13.6497623706194));
#14152=CARTESIAN_POINT('Ctrl Pts',(-7.74204705371982,-0.915087963995918,
13.6617655574087));
#14153=CARTESIAN_POINT('Ctrl Pts',(-7.51199928711969,-0.724543022591224,
13.6737687441981));
#14154=CARTESIAN_POINT('Ctrl Pts',(-7.35822688079599,-0.444367128060549,
13.6857719309874));
#14155=CARTESIAN_POINT('Ctrl Pts',(-7.32102560975806,-0.147979855989382,
13.6977751177767));
#14156=CARTESIAN_POINT('Ctrl Pts',(-7.28382433872012,0.148407416081785,
13.709778304566));
#14157=CARTESIAN_POINT('Ctrl Pts',(-7.3635846474467,0.457895344722766,13.7217814913553));
#14158=CARTESIAN_POINT('Ctrl Pts',(-7.5394054943793,0.699383189958356,13.7337846781446));
#14159=CARTESIAN_POINT('Ctrl Pts',(-7.7152263413119,0.940871035193946,13.745787864934));
#14160=CARTESIAN_POINT('Ctrl Pts',(-7.98526240565854,1.11182427083114,13.7577910517233));
#14161=CARTESIAN_POINT('Ctrl Pts',(-8.27875123560186,1.1674449172776,13.7697942385126));
#14162=CARTESIAN_POINT('Ctrl Pts',(-8.57224006554519,1.22306556372406,13.7817974253019));
#14163=CARTESIAN_POINT('Ctrl Pts',(-8.88610136060003,1.16276985667003,13.7938006120912));
#14164=CARTESIAN_POINT('Ctrl Pts',(-9.13808834820145,1.00235817476317,13.8058037988805));
#14165=CARTESIAN_POINT('Ctrl Pts',(-9.39007533580287,0.841946492856307,
13.8178069856699));
#14166=CARTESIAN_POINT('Ctrl Pts',(-9.57754329642162,0.583102430602426,
13.8298101724592));
#14167=CARTESIAN_POINT('Ctrl Pts',(-9.65136659729203,0.293655596345731,
13.8418133592485));
#14168=CARTESIAN_POINT('Ctrl Pts',(-9.67581103310558,0.197813707971733,
13.845787864934));
#14169=CARTESIAN_POINT('Ctrl Pts',(-9.68822500000011,0.0989100500913151,
13.8497623706194));
#14170=CARTESIAN_POINT('Ctrl Pts',(-9.688225,-1.36513023107909E-12,13.8537368763049));
#14171=CARTESIAN_POINT('Origin',(-8.5,0.,1.8));
#14172=CARTESIAN_POINT('',(-9.688225,3.77808895279941E-13,14.1962631236952));
#14173=CARTESIAN_POINT('',(-9.68865868051598,-0.000343891003544964,14.1537368763049));
#14174=CARTESIAN_POINT('',(-9.688225,-1.45515594291686E-16,1.8));
#14175=CARTESIAN_POINT('Ctrl Pts',(-9.688225,3.77808895279941E-13,14.1962631236952));
#14176=CARTESIAN_POINT('Ctrl Pts',(-9.68822499999991,0.29871282130646,14.1842599369058));
#14177=CARTESIAN_POINT('Ctrl Pts',(-9.57054245632568,0.595858078271847,
14.1722567501165));
#14178=CARTESIAN_POINT('Ctrl Pts',(-9.36601586214911,0.81356940523297,14.1602535633272));
#14179=CARTESIAN_POINT('Ctrl Pts',(-9.16148926797255,1.03128073219409,14.1482503765379));
#14180=CARTESIAN_POINT('Ctrl Pts',(-8.87226522412815,1.16727314847145,14.1362471897486));
#14181=CARTESIAN_POINT('Ctrl Pts',(-8.5741343570142,1.18591009260192,14.1242440029593));
#14182=CARTESIAN_POINT('Ctrl Pts',(-8.27600348990024,1.20454703673238,14.1122408161699));
#14183=CARTESIAN_POINT('Ctrl Pts',(-7.97209482032069,1.10563290540097,14.1002376293806));
#14184=CARTESIAN_POINT('Ctrl Pts',(-7.74204705372042,0.915087963996414,
14.0882344425913));
#14185=CARTESIAN_POINT('Ctrl Pts',(-7.51199928712015,0.724543022591856,
14.076231255802));
#14186=CARTESIAN_POINT('Ctrl Pts',(-7.35822688079626,0.444367128061253,
14.0642280690127));
#14187=CARTESIAN_POINT('Ctrl Pts',(-7.32102560975814,0.147979855990085,
14.0522248822234));
#14188=CARTESIAN_POINT('Ctrl Pts',(-7.28382433872003,-0.148407416081082,
14.040221695434));
#14189=CARTESIAN_POINT('Ctrl Pts',(-7.36358464744644,-0.457895344722135,
14.0282185086447));
#14190=CARTESIAN_POINT('Ctrl Pts',(-7.53940549437892,-0.699383189957837,
14.0162153218554));
#14191=CARTESIAN_POINT('Ctrl Pts',(-7.71522634131141,-0.94087103519354,
14.0042121350661));
#14192=CARTESIAN_POINT('Ctrl Pts',(-7.98526240565798,-1.11182427083088,
13.9922089482768));
#14193=CARTESIAN_POINT('Ctrl Pts',(-8.2787512356013,-1.16744491727749,13.9802057614874));
#14194=CARTESIAN_POINT('Ctrl Pts',(-8.57224006554462,-1.2230655637241,13.9682025746981));
#14195=CARTESIAN_POINT('Ctrl Pts',(-8.88610136059951,-1.1627698566702,13.9561993879088));
#14196=CARTESIAN_POINT('Ctrl Pts',(-9.13808834820102,-1.00235817476344,
13.9441962011195));
#14197=CARTESIAN_POINT('Ctrl Pts',(-9.39007533580253,-0.841946492856674,
13.9321930143302));
#14198=CARTESIAN_POINT('Ctrl Pts',(-9.5775432964214,-0.583102430602846,
13.9201898275409));
#14199=CARTESIAN_POINT('Ctrl Pts',(-9.65136659729192,-0.293655596346157,
13.9081866407515));
#14200=CARTESIAN_POINT('Ctrl Pts',(-9.67581103310547,-0.19781370797232,
13.9042121350661));
#14201=CARTESIAN_POINT('Ctrl Pts',(-9.68822500000004,-0.0989100500920693,
13.9002376293806));
#14202=CARTESIAN_POINT('Ctrl Pts',(-9.688225,4.53415083256914E-13,13.8962631236952));
#14203=CARTESIAN_POINT('Ctrl Pts',(-9.68655655853903,-0.000463272172757516,
13.8537368763049));
#14204=CARTESIAN_POINT('Ctrl Pts',(-9.68727352946558,-0.166355206423755,
13.8603818955633));
#14205=CARTESIAN_POINT('Ctrl Pts',(-9.65488880874086,-0.332016339541931,
13.8670269148217));
#14206=CARTESIAN_POINT('Ctrl Pts',(-9.58810721516616,-0.482507464589454,
13.8736719340801));
#14207=CARTESIAN_POINT('Ctrl Pts',(-9.42824047131953,-0.842764308599199,
13.8895792752318));
#14208=CARTESIAN_POINT('Ctrl Pts',(-9.07125782470074,-1.1160873825261,13.9054866163834));
#14209=CARTESIAN_POINT('Ctrl Pts',(-8.68208007088468,-1.17630173021062,
13.921393957535));
#14210=CARTESIAN_POINT('Ctrl Pts',(-8.29290231706859,-1.23651607789514,
13.9373012986866));
#14211=CARTESIAN_POINT('Ctrl Pts',(-7.87152945605521,-1.08362169933721,
13.9532086398383));
#14212=CARTESIAN_POINT('Ctrl Pts',(-7.60945480461122,-0.78893772856281,
13.9691159809899));
#14213=CARTESIAN_POINT('Ctrl Pts',(-7.47841747888923,-0.641595743175621,
13.9770696515657));
#14214=CARTESIAN_POINT('Ctrl Pts',(-7.38720470555958,-0.458806359734322,
13.9850233221415));
#14215=CARTESIAN_POINT('Ctrl Pts',(-7.34283850902019,-0.265277471449604,
13.9929769927173));
#14216=CARTESIAN_POINT('Ctrl Pts',(-7.2984723124808,-0.0717485831648862,
14.0009306632931));
#14217=CARTESIAN_POINT('Ctrl Pts',(-7.30095269273168,0.132519809963242,
14.0088843338689));
#14218=CARTESIAN_POINT('Ctrl Pts',(-7.35472170729873,0.322228361332696,
14.0168380044447));
#14219=CARTESIAN_POINT('Ctrl Pts',(-7.46225973643285,0.701645464071678,
14.0327453455964));
#14220=CARTESIAN_POINT('Ctrl Pts',(-7.7749523028318,1.02282319977593,14.048652686748));
#14221=CARTESIAN_POINT('Ctrl Pts',(-8.1514957837131,1.13814925380642,14.0645600278996));
#14222=CARTESIAN_POINT('Ctrl Pts',(-8.52803926459432,1.25347530783689,14.0804673690512));
#14223=CARTESIAN_POINT('Ctrl Pts',(-8.96843365995786,1.16294968019372,14.0963747102028));
#14224=CARTESIAN_POINT('Ctrl Pts',(-9.2692651211118,0.908307182907879,14.1122820513545));
#14225=CARTESIAN_POINT('Ctrl Pts',(-9.53058923645479,0.687106165312514,
14.1261003263379));
#14226=CARTESIAN_POINT('Ctrl Pts',(-9.6866002114824,0.342063792426944,14.1399186013214));
#14227=CARTESIAN_POINT('Ctrl Pts',(-9.68926336417008,-0.000823380536053999,
14.1537368763049));
#14228=CARTESIAN_POINT('Origin',(-8.5,0.,1.8));
#14229=CARTESIAN_POINT('',(-9.688225,4.03344024846319E-13,14.4962631236952));
#14230=CARTESIAN_POINT('',(-9.688225,-1.31394894964387E-12,14.4537368763049));
#14231=CARTESIAN_POINT('',(-9.688225,-1.45515594291686E-16,1.8));
#14232=CARTESIAN_POINT('Ctrl Pts',(-9.688225,4.03344024846319E-13,14.4962631236952));
#14233=CARTESIAN_POINT('Ctrl Pts',(-9.6882249999999,0.298712821306486,14.4842599369058));
#14234=CARTESIAN_POINT('Ctrl Pts',(-9.57054245632567,0.59585807827187,14.4722567501165));
#14235=CARTESIAN_POINT('Ctrl Pts',(-9.3660158621491,0.813569405232989,14.4602535633272));
#14236=CARTESIAN_POINT('Ctrl Pts',(-9.16148926797252,1.03128073219411,14.4482503765379));
#14237=CARTESIAN_POINT('Ctrl Pts',(-8.87226522412812,1.16727314847146,14.4362471897486));
#14238=CARTESIAN_POINT('Ctrl Pts',(-8.57413435701417,1.18591009260192,14.4242440029593));
#14239=CARTESIAN_POINT('Ctrl Pts',(-8.27600348990022,1.20454703673238,14.4122408161699));
#14240=CARTESIAN_POINT('Ctrl Pts',(-7.97209482032066,1.10563290540096,14.4002376293806));
#14241=CARTESIAN_POINT('Ctrl Pts',(-7.7420470537204,0.915087963996397,14.3882344425913));
#14242=CARTESIAN_POINT('Ctrl Pts',(-7.51199928712013,0.724543022591834,
14.376231255802));
#14243=CARTESIAN_POINT('Ctrl Pts',(-7.35822688079625,0.444367128061228,
14.3642280690127));
#14244=CARTESIAN_POINT('Ctrl Pts',(-7.32102560975814,0.14797985599006,14.3522248822234));
#14245=CARTESIAN_POINT('Ctrl Pts',(-7.28382433872003,-0.148407416081108,
14.340221695434));
#14246=CARTESIAN_POINT('Ctrl Pts',(-7.36358464744645,-0.457895344722159,
14.3282185086447));
#14247=CARTESIAN_POINT('Ctrl Pts',(-7.53940549437894,-0.699383189957858,
14.3162153218554));
#14248=CARTESIAN_POINT('Ctrl Pts',(-7.71522634131143,-0.940871035193557,
14.3042121350661));
#14249=CARTESIAN_POINT('Ctrl Pts',(-7.985262405658,-1.1118242708309,14.2922089482768));
#14250=CARTESIAN_POINT('Ctrl Pts',(-8.27875123560133,-1.1674449172775,14.2802057614874));
#14251=CARTESIAN_POINT('Ctrl Pts',(-8.57224006554465,-1.2230655637241,14.2682025746981));
#14252=CARTESIAN_POINT('Ctrl Pts',(-8.88610136059954,-1.16276985667019,
14.2561993879088));
#14253=CARTESIAN_POINT('Ctrl Pts',(-9.13808834820104,-1.00235817476342,
14.2441962011195));
#14254=CARTESIAN_POINT('Ctrl Pts',(-9.39007533580255,-0.841946492856655,
14.2321930143302));
#14255=CARTESIAN_POINT('Ctrl Pts',(-9.57754329642141,-0.583102430602823,
14.2201898275409));
#14256=CARTESIAN_POINT('Ctrl Pts',(-9.65136659729193,-0.293655596346132,
14.2081866407515));
#14257=CARTESIAN_POINT('Ctrl Pts',(-9.67581103310546,-0.197813707972328,
14.2042121350661));
#14258=CARTESIAN_POINT('Ctrl Pts',(-9.68822500000003,-0.0989100500921112,
14.2002376293806));
#14259=CARTESIAN_POINT('Ctrl Pts',(-9.688225,3.77808895279941E-13,14.1962631236952));
#14260=CARTESIAN_POINT('Ctrl Pts',(-9.688225,-1.27203803046427E-12,14.1537368763049));
#14261=CARTESIAN_POINT('Ctrl Pts',(-9.68822499999968,-0.298712821307377,
14.1657400630942));
#14262=CARTESIAN_POINT('Ctrl Pts',(-9.57054245632521,-0.595858078272697,
14.1777432498835));
#14263=CARTESIAN_POINT('Ctrl Pts',(-9.36601586214845,-0.813569405233671,
14.1897464366728));
#14264=CARTESIAN_POINT('Ctrl Pts',(-9.1614892679717,-1.03128073219465,14.2017496234622));
#14265=CARTESIAN_POINT('Ctrl Pts',(-8.87226522412716,-1.16727314847177,
14.2137528102515));
#14266=CARTESIAN_POINT('Ctrl Pts',(-8.57413435701317,-1.18591009260198,
14.2257559970408));
#14267=CARTESIAN_POINT('Ctrl Pts',(-8.27600348989917,-1.20454703673219,
14.2377591838301));
#14268=CARTESIAN_POINT('Ctrl Pts',(-7.97209482031969,-1.1056329054005,14.2497623706194));
#14269=CARTESIAN_POINT('Ctrl Pts',(-7.74204705371957,-0.915087963995714,
14.2617655574088));
#14270=CARTESIAN_POINT('Ctrl Pts',(-7.51199928711946,-0.724543022590929,
14.2737687441981));
#14271=CARTESIAN_POINT('Ctrl Pts',(-7.35822688079583,-0.444367128060156,
14.2857719309874));
#14272=CARTESIAN_POINT('Ctrl Pts',(-7.321025609758,-0.14797985598893,14.2977751177767));
#14273=CARTESIAN_POINT('Ctrl Pts',(-7.28382433872017,0.148407416082296,
14.309778304566));
#14274=CARTESIAN_POINT('Ctrl Pts',(-7.3635846474469,0.457895344723294,14.3217814913553));
#14275=CARTESIAN_POINT('Ctrl Pts',(-7.53940549437965,0.699383189958833,
14.3337846781447));
#14276=CARTESIAN_POINT('Ctrl Pts',(-7.7152263413124,0.940871035194372,14.345787864934));
#14277=CARTESIAN_POINT('Ctrl Pts',(-7.98526240565917,1.11182427083144,14.3577910517233));
#14278=CARTESIAN_POINT('Ctrl Pts',(-8.27875123560258,1.16744491727773,14.3697942385126));
#14279=CARTESIAN_POINT('Ctrl Pts',(-8.57224006554599,1.22306556372402,14.3817974253019));
#14280=CARTESIAN_POINT('Ctrl Pts',(-8.88610136060083,1.16276985666977,14.3938006120913));
#14281=CARTESIAN_POINT('Ctrl Pts',(-9.13808834820217,1.0023581747627,14.4058037988806));
#14282=CARTESIAN_POINT('Ctrl Pts',(-9.39007533580352,0.841946492855638,
14.4178069856699));
#14283=CARTESIAN_POINT('Ctrl Pts',(-9.5775432964221,0.583102430601566,14.4298101724592));
#14284=CARTESIAN_POINT('Ctrl Pts',(-9.65136659729228,0.293655596344766,
14.4418133592485));
#14285=CARTESIAN_POINT('Ctrl Pts',(-9.67581103310566,0.197813707971086,
14.445787864934));
#14286=CARTESIAN_POINT('Ctrl Pts',(-9.68822500000011,0.0989100500910174,
14.4497623706194));
#14287=CARTESIAN_POINT('Ctrl Pts',(-9.688225,-1.31394894964387E-12,14.4537368763049));
#14288=CARTESIAN_POINT('Origin',(-8.5,0.,1.8));
#14289=CARTESIAN_POINT('',(-9.688225,4.28879154412698E-13,14.7962631236952));
#14290=CARTESIAN_POINT('',(-9.688225,-1.28830279777503E-12,14.7537368763049));
#14291=CARTESIAN_POINT('',(-9.688225,-1.45515594291686E-16,1.8));
#14292=CARTESIAN_POINT('Ctrl Pts',(-9.688225,4.96602758914833E-13,14.7962631236952));
#14293=CARTESIAN_POINT('Ctrl Pts',(-9.68822499999988,0.298712821306624,
14.7842599369058));
#14294=CARTESIAN_POINT('Ctrl Pts',(-9.57054245632558,0.595858078272043,
14.7722567501165));
#14295=CARTESIAN_POINT('Ctrl Pts',(-9.36601586214894,0.813569405233155,
14.7602535633272));
#14296=CARTESIAN_POINT('Ctrl Pts',(-9.16148926797229,1.03128073219427,14.7482503765379));
#14297=CARTESIAN_POINT('Ctrl Pts',(-8.87226522412781,1.16727314847157,14.7362471897486));
#14298=CARTESIAN_POINT('Ctrl Pts',(-8.57413435701381,1.18591009260194,14.7242440029592));
#14299=CARTESIAN_POINT('Ctrl Pts',(-8.2760034898998,1.20454703673231,14.7122408161699));
#14300=CARTESIAN_POINT('Ctrl Pts',(-7.97209482032024,1.10563290540077,14.7002376293806));
#14301=CARTESIAN_POINT('Ctrl Pts',(-7.74204705372001,0.915087963996079,
14.6882344425913));
#14302=CARTESIAN_POINT('Ctrl Pts',(-7.51199928711979,0.724543022591391,
14.676231255802));
#14303=CARTESIAN_POINT('Ctrl Pts',(-7.35822688079602,0.444367128060664,
14.6642280690126));
#14304=CARTESIAN_POINT('Ctrl Pts',(-7.32102560975806,0.147979855989431,
14.6522248822233));
#14305=CARTESIAN_POINT('Ctrl Pts',(-7.2838243387201,-0.148407416081801,
14.640221695434));
#14306=CARTESIAN_POINT('Ctrl Pts',(-7.36358464744672,-0.457895344722858,
14.6282185086447));
#14307=CARTESIAN_POINT('Ctrl Pts',(-7.53940549437939,-0.699383189958479,
14.6162153218554));
#14308=CARTESIAN_POINT('Ctrl Pts',(-7.71522634131207,-0.940871035194101,
14.604212135066));
#14309=CARTESIAN_POINT('Ctrl Pts',(-7.9852624056588,-1.11182427083128,14.5922089482767));
#14310=CARTESIAN_POINT('Ctrl Pts',(-8.27875123560221,-1.16744491727767,
14.5802057614874));
#14311=CARTESIAN_POINT('Ctrl Pts',(-8.57224006554563,-1.22306556372405,
14.5682025746981));
#14312=CARTESIAN_POINT('Ctrl Pts',(-8.88610136060052,-1.16276985666988,
14.5561993879088));
#14313=CARTESIAN_POINT('Ctrl Pts',(-9.13808834820192,-1.00235817476287,
14.5441962011195));
#14314=CARTESIAN_POINT('Ctrl Pts',(-9.39007533580332,-0.841946492855853,
14.5321930143301));
#14315=CARTESIAN_POINT('Ctrl Pts',(-9.57754329642198,-0.583102430601802,
14.5201898275408));
#14316=CARTESIAN_POINT('Ctrl Pts',(-9.65136659729222,-0.293655596344994,
14.5081866407515));
#14317=CARTESIAN_POINT('Ctrl Pts',(-9.67581103310556,-0.197813707971537,
14.5042121350661));
#14318=CARTESIAN_POINT('Ctrl Pts',(-9.68822500000003,-0.0989100500917029,
14.5002376293806));
#14319=CARTESIAN_POINT('Ctrl Pts',(-9.688225,4.03344024846319E-13,14.4962631236952));
#14320=CARTESIAN_POINT('Ctrl Pts',(-9.688225,-1.31394894964387E-12,14.4537368763049));
#14321=CARTESIAN_POINT('Ctrl Pts',(-9.68822499999967,-0.298712821307396,
14.4657400630942));
#14322=CARTESIAN_POINT('Ctrl Pts',(-9.57054245632521,-0.59585807827269,
14.4777432498835));
#14323=CARTESIAN_POINT('Ctrl Pts',(-9.36601586214847,-0.813569405233652,
14.4897464366728));
#14324=CARTESIAN_POINT('Ctrl Pts',(-9.16148926797173,-1.03128073219461,
14.5017496234622));
#14325=CARTESIAN_POINT('Ctrl Pts',(-8.87226522412723,-1.16727314847175,
14.5137528102515));
#14326=CARTESIAN_POINT('Ctrl Pts',(-8.57413435701326,-1.18591009260198,
14.5257559970408));
#14327=CARTESIAN_POINT('Ctrl Pts',(-8.27600348989929,-1.20454703673221,
14.5377591838301));
#14328=CARTESIAN_POINT('Ctrl Pts',(-7.97209482031982,-1.10563290540056,
14.5497623706194));
#14329=CARTESIAN_POINT('Ctrl Pts',(-7.7420470537197,-0.915087963995816,
14.5617655574087));
#14330=CARTESIAN_POINT('Ctrl Pts',(-7.51199928711958,-0.724543022591077,
14.5737687441981));
#14331=CARTESIAN_POINT('Ctrl Pts',(-7.35822688079591,-0.444367128060353,
14.5857719309874));
#14332=CARTESIAN_POINT('Ctrl Pts',(-7.32102560975803,-0.147979855989156,
14.5977751177767));
#14333=CARTESIAN_POINT('Ctrl Pts',(-7.28382433872015,0.14840741608204,14.609778304566));
#14334=CARTESIAN_POINT('Ctrl Pts',(-7.3635846474468,0.45789534472303,14.6217814913553));
#14335=CARTESIAN_POINT('Ctrl Pts',(-7.53940549437947,0.699383189958594,
14.6337846781447));
#14336=CARTESIAN_POINT('Ctrl Pts',(-7.71522634131215,0.940871035194158,
14.645787864934));
#14337=CARTESIAN_POINT('Ctrl Pts',(-7.98526240565885,1.11182427083129,14.6577910517233));
#14338=CARTESIAN_POINT('Ctrl Pts',(-8.27875123560222,1.16744491727767,14.6697942385126));
#14339=CARTESIAN_POINT('Ctrl Pts',(-8.57224006554559,1.22306556372404,14.6817974253019));
#14340=CARTESIAN_POINT('Ctrl Pts',(-8.88610136060043,1.1627698566699,14.6938006120912));
#14341=CARTESIAN_POINT('Ctrl Pts',(-9.13808834820181,1.00235817476294,14.7058037988806));
#14342=CARTESIAN_POINT('Ctrl Pts',(-9.39007533580319,0.841946492855973,
14.7178069856699));
#14343=CARTESIAN_POINT('Ctrl Pts',(-9.57754329642186,0.583102430601997,
14.7298101724592));
#14344=CARTESIAN_POINT('Ctrl Pts',(-9.65136659729215,0.293655596345249,
14.7418133592485));
#14345=CARTESIAN_POINT('Ctrl Pts',(-9.67581103310561,0.197813707971427,
14.745787864934));
#14346=CARTESIAN_POINT('Ctrl Pts',(-9.68822500000011,0.0989100500912006,
14.7497623706194));
#14347=CARTESIAN_POINT('Ctrl Pts',(-9.688225,-1.28830279777503E-12,14.7537368763049));
#14348=CARTESIAN_POINT('Origin',(-8.5,0.,1.8));
#14349=CARTESIAN_POINT('',(-9.688225,4.54525306281539E-13,15.0962631236952));
#14350=CARTESIAN_POINT('',(-9.688225,-1.26271215705742E-12,15.0537368763049));
#14351=CARTESIAN_POINT('',(-9.688225,-1.45515594291686E-16,1.8));
#14352=CARTESIAN_POINT('Ctrl Pts',(-9.688225,4.54525306281539E-13,15.0962631236952));
#14353=CARTESIAN_POINT('Ctrl Pts',(-9.68822499999989,0.298712821306559,
15.0842599369058));
#14354=CARTESIAN_POINT('Ctrl Pts',(-9.57054245632562,0.595858078271961,
15.0722567501165));
#14355=CARTESIAN_POINT('Ctrl Pts',(-9.36601586214901,0.813569405233076,
15.0602535633272));
#14356=CARTESIAN_POINT('Ctrl Pts',(-9.1614892679724,1.03128073219419,15.0482503765379));
#14357=CARTESIAN_POINT('Ctrl Pts',(-8.87226522412796,1.16727314847152,15.0362471897486));
#14358=CARTESIAN_POINT('Ctrl Pts',(-8.57413435701398,1.18591009260193,15.0242440029593));
#14359=CARTESIAN_POINT('Ctrl Pts',(-8.2760034899,1.20454703673235,15.0122408161699));
#14360=CARTESIAN_POINT('Ctrl Pts',(-7.97209482032045,1.10563290540086,15.0002376293806));
#14361=CARTESIAN_POINT('Ctrl Pts',(-7.7420470537202,0.915087963996235,14.9882344425913));
#14362=CARTESIAN_POINT('Ctrl Pts',(-7.51199928711996,0.724543022591609,
14.976231255802));
#14363=CARTESIAN_POINT('Ctrl Pts',(-7.35822688079613,0.444367128060941,
14.9642280690127));
#14364=CARTESIAN_POINT('Ctrl Pts',(-7.3210256097581,0.147979855989741,14.9522248822233));
#14365=CARTESIAN_POINT('Ctrl Pts',(-7.28382433872007,-0.148407416081459,
14.940221695434));
#14366=CARTESIAN_POINT('Ctrl Pts',(-7.36358464744658,-0.457895344722513,
14.9282185086447));
#14367=CARTESIAN_POINT('Ctrl Pts',(-7.53940549437917,-0.699383189958172,
14.9162153218554));
#14368=CARTESIAN_POINT('Ctrl Pts',(-7.71522634131175,-0.940871035193832,
14.9042121350661));
#14369=CARTESIAN_POINT('Ctrl Pts',(-7.98526240565841,-1.11182427083109,
14.8922089482767));
#14370=CARTESIAN_POINT('Ctrl Pts',(-8.27875123560177,-1.16744491727758,
14.8802057614874));
#14371=CARTESIAN_POINT('Ctrl Pts',(-8.57224006554514,-1.22306556372407,
14.8682025746981));
#14372=CARTESIAN_POINT('Ctrl Pts',(-8.88610136060003,-1.16276985667004,
14.8561993879088));
#14373=CARTESIAN_POINT('Ctrl Pts',(-9.13808834820149,-1.00235817476314,
14.8441962011195));
#14374=CARTESIAN_POINT('Ctrl Pts',(-9.39007533580294,-0.841946492856251,
14.8321930143302));
#14375=CARTESIAN_POINT('Ctrl Pts',(-9.5775432964217,-0.583102430602308,
14.8201898275408));
#14376=CARTESIAN_POINT('Ctrl Pts',(-9.65136659729208,-0.293655596345558,
14.8081866407515));
#14377=CARTESIAN_POINT('Ctrl Pts',(-9.67581103310552,-0.197813707971895,
14.8042121350661));
#14378=CARTESIAN_POINT('Ctrl Pts',(-9.68822500000004,-0.0989100500918347,
14.8002376293806));
#14379=CARTESIAN_POINT('Ctrl Pts',(-9.688225,4.96602758914833E-13,14.7962631236952));
#14380=CARTESIAN_POINT('Ctrl Pts',(-9.688225,-1.28830279777503E-12,14.7537368763049));
#14381=CARTESIAN_POINT('Ctrl Pts',(-9.68822499999968,-0.298712821307393,
14.7657400630942));
#14382=CARTESIAN_POINT('Ctrl Pts',(-9.57054245632521,-0.595858078272712,
14.7777432498835));
#14383=CARTESIAN_POINT('Ctrl Pts',(-9.36601586214844,-0.813569405233683,
14.7897464366728));
#14384=CARTESIAN_POINT('Ctrl Pts',(-9.16148926797168,-1.03128073219465,
14.8017496234622));
#14385=CARTESIAN_POINT('Ctrl Pts',(-8.87226522412714,-1.16727314847178,
14.8137528102515));
#14386=CARTESIAN_POINT('Ctrl Pts',(-8.57413435701315,-1.18591009260198,
14.8257559970408));
#14387=CARTESIAN_POINT('Ctrl Pts',(-8.27600348989916,-1.20454703673219,
14.8377591838301));
#14388=CARTESIAN_POINT('Ctrl Pts',(-7.97209482031967,-1.10563290540049,
14.8497623706194));
#14389=CARTESIAN_POINT('Ctrl Pts',(-7.74204705371956,-0.915087963995703,
14.8617655574088));
#14390=CARTESIAN_POINT('Ctrl Pts',(-7.51199928711945,-0.724543022590915,
14.8737687441981));
#14391=CARTESIAN_POINT('Ctrl Pts',(-7.35822688079582,-0.44436712806014,
14.8857719309874));
#14392=CARTESIAN_POINT('Ctrl Pts',(-7.321025609758,-0.147979855988914,14.8977751177767));
#14393=CARTESIAN_POINT('Ctrl Pts',(-7.28382433872017,0.148407416082312,
14.909778304566));
#14394=CARTESIAN_POINT('Ctrl Pts',(-7.36358464744691,0.45789534472331,14.9217814913553));
#14395=CARTESIAN_POINT('Ctrl Pts',(-7.53940549437966,0.699383189958846,
14.9337846781447));
#14396=CARTESIAN_POINT('Ctrl Pts',(-7.71522634131241,0.940871035194383,
14.945787864934));
#14397=CARTESIAN_POINT('Ctrl Pts',(-7.98526240565919,1.11182427083145,14.9577910517233));
#14398=CARTESIAN_POINT('Ctrl Pts',(-8.27875123560259,1.16744491727774,14.9697942385126));
#14399=CARTESIAN_POINT('Ctrl Pts',(-8.572240065546,1.22306556372402,14.9817974253019));
#14400=CARTESIAN_POINT('Ctrl Pts',(-8.88610136060085,1.16276985666977,14.9938006120913));
#14401=CARTESIAN_POINT('Ctrl Pts',(-9.13808834820219,1.0023581747627,15.0058037988806));
#14402=CARTESIAN_POINT('Ctrl Pts',(-9.39007533580353,0.841946492855626,
15.0178069856699));
#14403=CARTESIAN_POINT('Ctrl Pts',(-9.57754329642211,0.583102430601552,
15.0298101724592));
#14404=CARTESIAN_POINT('Ctrl Pts',(-9.65136659729228,0.293655596344751,
15.0418133592485));
#14405=CARTESIAN_POINT('Ctrl Pts',(-9.67581103310565,0.197813707971113,
15.045787864934));
#14406=CARTESIAN_POINT('Ctrl Pts',(-9.6882250000001,0.0989100500910911,
15.0497623706194));
#14407=CARTESIAN_POINT('Ctrl Pts',(-9.688225,-1.19515508600898E-12,15.0537368763049));
#14408=CARTESIAN_POINT('Origin',(-8.5,0.,1.8));
#14409=CARTESIAN_POINT('',(-9.688225,4.8017145815038E-13,15.3962631236952));
#14410=CARTESIAN_POINT('',(-9.688225,-1.23712151633981E-12,15.3537368763049));
#14411=CARTESIAN_POINT('',(-9.688225,-1.45515594291686E-16,1.8));
#14412=CARTESIAN_POINT('Ctrl Pts',(-9.688225,5.4767301804759E-13,15.3962631236952));
#14413=CARTESIAN_POINT('Ctrl Pts',(-9.68822499999986,0.298712821306675,
15.3842599369058));
#14414=CARTESIAN_POINT('Ctrl Pts',(-9.57054245632556,0.595858078272089,
15.3722567501165));
#14415=CARTESIAN_POINT('Ctrl Pts',(-9.3660158621489,0.813569405233193,15.3602535633272));
#14416=CARTESIAN_POINT('Ctrl Pts',(-9.16148926797225,1.0312807321943,15.3482503765379));
#14417=CARTESIAN_POINT('Ctrl Pts',(-8.87226522412776,1.16727314847159,15.3362471897486));
#14418=CARTESIAN_POINT('Ctrl Pts',(-8.57413435701375,1.18591009260195,15.3242440029592));
#14419=CARTESIAN_POINT('Ctrl Pts',(-8.27600348989975,1.2045470367323,15.3122408161699));
#14420=CARTESIAN_POINT('Ctrl Pts',(-7.97209482032019,1.10563290540075,15.3002376293806));
#14421=CARTESIAN_POINT('Ctrl Pts',(-7.74204705371997,0.915087963996047,
15.2882344425913));
#14422=CARTESIAN_POINT('Ctrl Pts',(-7.51199928711976,0.724543022591348,
15.276231255802));
#14423=CARTESIAN_POINT('Ctrl Pts',(-7.358226880796,0.444367128060615,15.2642280690126));
#14424=CARTESIAN_POINT('Ctrl Pts',(-7.32102560975806,0.147979855989381,
15.2522248822233));
#14425=CARTESIAN_POINT('Ctrl Pts',(-7.28382433872011,-0.148407416081853,
15.240221695434));
#14426=CARTESIAN_POINT('Ctrl Pts',(-7.36358464744674,-0.457895344722907,
15.2282185086447));
#14427=CARTESIAN_POINT('Ctrl Pts',(-7.53940549437942,-0.699383189958521,
15.2162153218554));
#14428=CARTESIAN_POINT('Ctrl Pts',(-7.71522634131211,-0.940871035194135,
15.204212135066));
#14429=CARTESIAN_POINT('Ctrl Pts',(-7.98526240565885,-1.1118242708313,15.1922089482767));
#14430=CARTESIAN_POINT('Ctrl Pts',(-8.27875123560226,-1.16744491727767,
15.1802057614874));
#14431=CARTESIAN_POINT('Ctrl Pts',(-8.57224006554568,-1.22306556372405,
15.1682025746981));
#14432=CARTESIAN_POINT('Ctrl Pts',(-8.88610136060057,-1.16276985666986,
15.1561993879088));
#14433=CARTESIAN_POINT('Ctrl Pts',(-9.13808834820196,-1.00235817476284,
15.1441962011195));
#14434=CARTESIAN_POINT('Ctrl Pts',(-9.39007533580336,-0.841946492855815,
15.1321930143301));
#14435=CARTESIAN_POINT('Ctrl Pts',(-9.577543296422,-0.583102430601755,15.1201898275408));
#14436=CARTESIAN_POINT('Ctrl Pts',(-9.65136659729223,-0.293655596344945,
15.1081866407515));
#14437=CARTESIAN_POINT('Ctrl Pts',(-9.67581103310557,-0.197813707971486,
15.104212135066));
#14438=CARTESIAN_POINT('Ctrl Pts',(-9.68822500000004,-0.0989100500916517,
15.1002376293806));
#14439=CARTESIAN_POINT('Ctrl Pts',(-9.688225,4.54525306281539E-13,15.0962631236952));
#14440=CARTESIAN_POINT('Ctrl Pts',(-9.688225,-1.19515508600898E-12,15.0537368763049));
#14441=CARTESIAN_POINT('Ctrl Pts',(-9.6882249999997,-0.298712821307277,
15.0657400630942));
#14442=CARTESIAN_POINT('Ctrl Pts',(-9.57054245632527,-0.595858078272583,
15.0777432498835));
#14443=CARTESIAN_POINT('Ctrl Pts',(-9.36601586214855,-0.813569405233566,
15.0897464366728));
#14444=CARTESIAN_POINT('Ctrl Pts',(-9.16148926797184,-1.03128073219455,
15.1017496234622));
#14445=CARTESIAN_POINT('Ctrl Pts',(-8.87226522412734,-1.16727314847171,
15.1137528102515));
#14446=CARTESIAN_POINT('Ctrl Pts',(-8.57413435701338,-1.18591009260197,
15.1257559970408));
#14447=CARTESIAN_POINT('Ctrl Pts',(-8.27600348989941,-1.20454703673223,
15.1377591838301));
#14448=CARTESIAN_POINT('Ctrl Pts',(-7.97209482031993,-1.10563290540061,
15.1497623706194));
#14449=CARTESIAN_POINT('Ctrl Pts',(-7.74204705371979,-0.915087963995892,
15.1617655574087));
#14450=CARTESIAN_POINT('Ctrl Pts',(-7.51199928711965,-0.724543022591176,
15.1737687441981));
#14451=CARTESIAN_POINT('Ctrl Pts',(-7.35822688079596,-0.444367128060467,
15.1857719309874));
#14452=CARTESIAN_POINT('Ctrl Pts',(-7.32102560975804,-0.147979855989274,
15.1977751177767));
#14453=CARTESIAN_POINT('Ctrl Pts',(-7.28382433872013,0.148407416081918,
15.209778304566));
#14454=CARTESIAN_POINT('Ctrl Pts',(-7.36358464744675,0.457895344722916,
15.2217814913553));
#14455=CARTESIAN_POINT('Ctrl Pts',(-7.5394054943794,0.699383189958498,15.2337846781446));
#14456=CARTESIAN_POINT('Ctrl Pts',(-7.71522634131206,0.94087103519408,15.245787864934));
#14457=CARTESIAN_POINT('Ctrl Pts',(-7.98526240565874,1.11182427083124,15.2577910517233));
#14458=CARTESIAN_POINT('Ctrl Pts',(-8.2787512356021,1.16744491727764,15.2697942385126));
#14459=CARTESIAN_POINT('Ctrl Pts',(-8.57224006554547,1.22306556372405,15.2817974253019));
#14460=CARTESIAN_POINT('Ctrl Pts',(-8.88610136060031,1.16276985666994,15.2938006120912));
#14461=CARTESIAN_POINT('Ctrl Pts',(-9.13808834820171,1.002358174763,15.3058037988806));
#14462=CARTESIAN_POINT('Ctrl Pts',(-9.39007533580311,0.841946492856062,
15.3178069856699));
#14463=CARTESIAN_POINT('Ctrl Pts',(-9.5775432964218,0.583102430602104,15.3298101724592));
#14464=CARTESIAN_POINT('Ctrl Pts',(-9.65136659729213,0.293655596345364,
15.3418133592485));
#14465=CARTESIAN_POINT('Ctrl Pts',(-9.6758110331056,0.197813707971522,15.345787864934));
#14466=CARTESIAN_POINT('Ctrl Pts',(-9.6882250000001,0.0989100500912743,
15.3497623706194));
#14467=CARTESIAN_POINT('Ctrl Pts',(-9.688225,-1.23712151633981E-12,15.3537368763049));
#14468=CARTESIAN_POINT('Origin',(-8.5,0.,1.8));
#14469=CARTESIAN_POINT('',(-9.688225,5.05817610019221E-13,15.6962631236952));
#14470=CARTESIAN_POINT('',(-9.688225,-1.21141985331974E-12,15.6537368763049));
#14471=CARTESIAN_POINT('',(-9.688225,-1.45515594291686E-16,1.8));
#14472=CARTESIAN_POINT('Ctrl Pts',(-9.688225,5.05817610019221E-13,15.6962631236952));
#14473=CARTESIAN_POINT('Ctrl Pts',(-9.68822499999987,0.298712821306611,
15.6842599369058));
#14474=CARTESIAN_POINT('Ctrl Pts',(-9.5705424563256,0.595858078272007,15.6722567501165));
#14475=CARTESIAN_POINT('Ctrl Pts',(-9.36601586214898,0.813569405233113,
15.6602535633272));
#14476=CARTESIAN_POINT('Ctrl Pts',(-9.16148926797236,1.03128073219422,15.6482503765379));
#14477=CARTESIAN_POINT('Ctrl Pts',(-8.87226522412791,1.16727314847153,15.6362471897486));
#14478=CARTESIAN_POINT('Ctrl Pts',(-8.57413435701393,1.18591009260194,15.6242440029592));
#14479=CARTESIAN_POINT('Ctrl Pts',(-8.27600348989995,1.20454703673234,15.6122408161699));
#14480=CARTESIAN_POINT('Ctrl Pts',(-7.9720948203204,1.10563290540084,15.6002376293806));
#14481=CARTESIAN_POINT('Ctrl Pts',(-7.74204705372016,0.915087963996203,
15.5882344425913));
#14482=CARTESIAN_POINT('Ctrl Pts',(-7.51199928711993,0.724543022591566,
15.576231255802));
#14483=CARTESIAN_POINT('Ctrl Pts',(-7.35822688079612,0.444367128060892,
15.5642280690127));
#14484=CARTESIAN_POINT('Ctrl Pts',(-7.3210256097581,0.14797985598969,15.5522248822233));
#14485=CARTESIAN_POINT('Ctrl Pts',(-7.28382433872008,-0.148407416081511,
15.540221695434));
#14486=CARTESIAN_POINT('Ctrl Pts',(-7.3635846474466,-0.457895344722562,
15.5282185086447));
#14487=CARTESIAN_POINT('Ctrl Pts',(-7.5394054943792,-0.699383189958214,
15.5162153218554));
#14488=CARTESIAN_POINT('Ctrl Pts',(-7.71522634131179,-0.940871035193866,
15.5042121350661));
#14489=CARTESIAN_POINT('Ctrl Pts',(-7.98526240565846,-1.11182427083111,
15.4922089482767));
#14490=CARTESIAN_POINT('Ctrl Pts',(-8.27875123560183,-1.16744491727759,
15.4802057614874));
#14491=CARTESIAN_POINT('Ctrl Pts',(-8.5722400655452,-1.22306556372407,15.4682025746981));
#14492=CARTESIAN_POINT('Ctrl Pts',(-8.88610136060008,-1.16276985667002,
15.4561993879088));
#14493=CARTESIAN_POINT('Ctrl Pts',(-9.13808834820153,-1.00235817476312,
15.4441962011195));
#14494=CARTESIAN_POINT('Ctrl Pts',(-9.39007533580298,-0.841946492856212,
15.4321930143302));
#14495=CARTESIAN_POINT('Ctrl Pts',(-9.57754329642172,-0.583102430602261,
15.4201898275408));
#14496=CARTESIAN_POINT('Ctrl Pts',(-9.65136659729209,-0.293655596345509,
15.4081866407515));
#14497=CARTESIAN_POINT('Ctrl Pts',(-9.67581103310553,-0.197813707971844,
15.4042121350661));
#14498=CARTESIAN_POINT('Ctrl Pts',(-9.68822500000005,-0.0989100500917836,
15.4002376293806));
#14499=CARTESIAN_POINT('Ctrl Pts',(-9.688225,5.4767301804759E-13,15.3962631236952));
#14500=CARTESIAN_POINT('Ctrl Pts',(-9.688225,-1.23712151633981E-12,15.3537368763049));
#14501=CARTESIAN_POINT('Ctrl Pts',(-9.68822499999969,-0.298712821307319,
15.3657400630942));
#14502=CARTESIAN_POINT('Ctrl Pts',(-9.57054245632525,-0.595858078272621,
15.3777432498835));
#14503=CARTESIAN_POINT('Ctrl Pts',(-9.36601586214852,-0.813569405233596,
15.3897464366728));
#14504=CARTESIAN_POINT('Ctrl Pts',(-9.1614892679718,-1.03128073219457,15.4017496234622));
#14505=CARTESIAN_POINT('Ctrl Pts',(-8.8722652241273,-1.16727314847172,15.4137528102515));
#14506=CARTESIAN_POINT('Ctrl Pts',(-8.57413435701334,-1.18591009260197,
15.4257559970408));
#14507=CARTESIAN_POINT('Ctrl Pts',(-8.27600348989937,-1.20454703673222,
15.4377591838301));
#14508=CARTESIAN_POINT('Ctrl Pts',(-7.97209482031989,-1.10563290540059,
15.4497623706194));
#14509=CARTESIAN_POINT('Ctrl Pts',(-7.74204705371976,-0.915087963995865,
15.4617655574087));
#14510=CARTESIAN_POINT('Ctrl Pts',(-7.51199928711962,-0.724543022591141,
15.4737687441981));
#14511=CARTESIAN_POINT('Ctrl Pts',(-7.35822688079594,-0.444367128060427,
15.4857719309874));
#14512=CARTESIAN_POINT('Ctrl Pts',(-7.32102560975804,-0.147979855989233,
15.4977751177767));
#14513=CARTESIAN_POINT('Ctrl Pts',(-7.28382433872014,0.148407416081961,
15.509778304566));
#14514=CARTESIAN_POINT('Ctrl Pts',(-7.36358464744677,0.457895344722956,
15.5217814913553));
#14515=CARTESIAN_POINT('Ctrl Pts',(-7.53940549437943,0.699383189958532,
15.5337846781447));
#14516=CARTESIAN_POINT('Ctrl Pts',(-7.71522634131209,0.940871035194107,
15.545787864934));
#14517=CARTESIAN_POINT('Ctrl Pts',(-7.98526240565878,1.11182427083126,15.5577910517233));
#14518=CARTESIAN_POINT('Ctrl Pts',(-8.27875123560215,1.16744491727765,15.5697942385126));
#14519=CARTESIAN_POINT('Ctrl Pts',(-8.57224006554551,1.22306556372405,15.5817974253019));
#14520=CARTESIAN_POINT('Ctrl Pts',(-8.88610136060035,1.16276985666992,15.5938006120912));
#14521=CARTESIAN_POINT('Ctrl Pts',(-9.13808834820175,1.00235817476298,15.6058037988806));
#14522=CARTESIAN_POINT('Ctrl Pts',(-9.39007533580314,0.84194649285603,15.6178069856699));
#14523=CARTESIAN_POINT('Ctrl Pts',(-9.57754329642182,0.583102430602066,
15.6298101724592));
#14524=CARTESIAN_POINT('Ctrl Pts',(-9.65136659729214,0.293655596345324,
15.6418133592485));
#14525=CARTESIAN_POINT('Ctrl Pts',(-9.6758110331056,0.197813707971524,15.645787864934));
#14526=CARTESIAN_POINT('Ctrl Pts',(-9.6882250000001,0.0989100500913225,
15.6497623706194));
#14527=CARTESIAN_POINT('Ctrl Pts',(-9.688225,-1.14391829342253E-12,15.6537368763049));
#14528=CARTESIAN_POINT('Origin',(-8.5,0.,1.8));
#14529=CARTESIAN_POINT('',(-9.68731278632248,-0.000152542232196749,15.9962631236952));
#14530=CARTESIAN_POINT('',(-9.688225,-1.18588472375336E-12,15.9537368763049));
#14531=CARTESIAN_POINT('',(-9.688225,-1.45515594291686E-16,1.8));
#14532=CARTESIAN_POINT('Ctrl Pts',(-9.688225,5.98965321785272E-13,15.9962631236952));
#14533=CARTESIAN_POINT('Ctrl Pts',(-9.68822499999985,0.298712821306659,
15.9842599369058));
#14534=CARTESIAN_POINT('Ctrl Pts',(-9.57054245632559,0.595858078272002,
15.9722567501165));
#14535=CARTESIAN_POINT('Ctrl Pts',(-9.36601586214901,0.813569405233082,
15.9602535633272));
#14536=CARTESIAN_POINT('Ctrl Pts',(-9.16148926797243,1.03128073219416,15.9482503765379));
#14537=CARTESIAN_POINT('Ctrl Pts',(-8.87226522412804,1.16727314847148,15.9362471897486));
#14538=CARTESIAN_POINT('Ctrl Pts',(-8.57413435701411,1.18591009260192,15.9242440029593));
#14539=CARTESIAN_POINT('Ctrl Pts',(-8.27600348990018,1.20454703673237,15.9122408161699));
#14540=CARTESIAN_POINT('Ctrl Pts',(-7.97209482032065,1.10563290540095,15.9002376293806));
#14541=CARTESIAN_POINT('Ctrl Pts',(-7.7420470537204,0.915087963996402,15.8882344425913));
#14542=CARTESIAN_POINT('Ctrl Pts',(-7.51199928712015,0.724543022591854,
15.876231255802));
#14543=CARTESIAN_POINT('Ctrl Pts',(-7.35822688079628,0.444367128061277,
15.8642280690127));
#14544=CARTESIAN_POINT('Ctrl Pts',(-7.32102560975815,0.147979855990134,
15.8522248822234));
#14545=CARTESIAN_POINT('Ctrl Pts',(-7.28382433872002,-0.148407416081009,
15.840221695434));
#14546=CARTESIAN_POINT('Ctrl Pts',(-7.36358464744641,-0.457895344722041,
15.8282185086447));
#14547=CARTESIAN_POINT('Ctrl Pts',(-7.53940549437885,-0.699383189957743,
15.8162153218554));
#14548=CARTESIAN_POINT('Ctrl Pts',(-7.7152263413113,-0.940871035193445,
15.8042121350661));
#14549=CARTESIAN_POINT('Ctrl Pts',(-7.98526240565783,-1.11182427083081,
15.7922089482768));
#14550=CARTESIAN_POINT('Ctrl Pts',(-8.27875123560112,-1.16744491727746,
15.7802057614875));
#14551=CARTESIAN_POINT('Ctrl Pts',(-8.57224006554441,-1.22306556372411,
15.7682025746981));
#14552=CARTESIAN_POINT('Ctrl Pts',(-8.88610136059929,-1.16276985667027,
15.7561993879088));
#14553=CARTESIAN_POINT('Ctrl Pts',(-9.13808834820081,-1.00235817476357,
15.7441962011195));
#14554=CARTESIAN_POINT('Ctrl Pts',(-9.39007533580233,-0.841946492856875,
15.7321930143302));
#14555=CARTESIAN_POINT('Ctrl Pts',(-9.57754329642125,-0.583102430603113,
15.7201898275409));
#14556=CARTESIAN_POINT('Ctrl Pts',(-9.65136659729185,-0.293655596346466,
15.7081866407516));
#14557=CARTESIAN_POINT('Ctrl Pts',(-9.67581103310544,-0.197813707972516,
15.7042121350661));
#14558=CARTESIAN_POINT('Ctrl Pts',(-9.68822500000004,-0.0989100500921407,
15.7002376293806));
#14559=CARTESIAN_POINT('Ctrl Pts',(-9.688225,5.05817610019221E-13,15.6962631236952));
#14560=CARTESIAN_POINT('Ctrl Pts',(-9.688225,-1.14391829342253E-12,15.6537368763049));
#14561=CARTESIAN_POINT('Ctrl Pts',(-9.68822499999971,-0.298712821307226,
15.6657400630942));
#14562=CARTESIAN_POINT('Ctrl Pts',(-9.5705424563253,-0.595858078272537,
15.6777432498835));
#14563=CARTESIAN_POINT('Ctrl Pts',(-9.36601586214859,-0.813569405233528,
15.6897464366728));
#14564=CARTESIAN_POINT('Ctrl Pts',(-9.16148926797188,-1.03128073219452,
15.7017496234622));
#14565=CARTESIAN_POINT('Ctrl Pts',(-8.87226522412739,-1.16727314847169,
15.7137528102515));
#14566=CARTESIAN_POINT('Ctrl Pts',(-8.57413435701343,-1.18591009260197,
15.7257559970408));
#14567=CARTESIAN_POINT('Ctrl Pts',(-8.27600348989946,-1.20454703673224,
15.7377591838301));
#14568=CARTESIAN_POINT('Ctrl Pts',(-7.97209482031998,-1.10563290540063,
15.7497623706194));
#14569=CARTESIAN_POINT('Ctrl Pts',(-7.74204705371983,-0.915087963995925,
15.7617655574087));
#14570=CARTESIAN_POINT('Ctrl Pts',(-7.51199928711968,-0.724543022591218,
15.7737687441981));
#14571=CARTESIAN_POINT('Ctrl Pts',(-7.35822688079597,-0.444367128060516,
15.7857719309874));
#14572=CARTESIAN_POINT('Ctrl Pts',(-7.32102560975805,-0.147979855989325,
15.7977751177767));
#14573=CARTESIAN_POINT('Ctrl Pts',(-7.28382433872012,0.148407416081866,
15.809778304566));
#14574=CARTESIAN_POINT('Ctrl Pts',(-7.36358464744673,0.457895344722867,
15.8217814913553));
#14575=CARTESIAN_POINT('Ctrl Pts',(-7.53940549437938,0.699383189958457,
15.8337846781446));
#14576=CARTESIAN_POINT('Ctrl Pts',(-7.71522634131202,0.940871035194046,
15.845787864934));
#14577=CARTESIAN_POINT('Ctrl Pts',(-7.9852624056587,1.11182427083122,15.8577910517233));
#14578=CARTESIAN_POINT('Ctrl Pts',(-8.27875123560205,1.16744491727763,15.8697942385126));
#14579=CARTESIAN_POINT('Ctrl Pts',(-8.57224006554541,1.22306556372405,15.8817974253019));
#14580=CARTESIAN_POINT('Ctrl Pts',(-8.88610136060026,1.16276985666995,15.8938006120912));
#14581=CARTESIAN_POINT('Ctrl Pts',(-9.13808834820167,1.00235817476303,15.9058037988806));
#14582=CARTESIAN_POINT('Ctrl Pts',(-9.39007533580307,0.8419464928561,15.9178069856699));
#14583=CARTESIAN_POINT('Ctrl Pts',(-9.57754329642177,0.583102430602151,
15.9298101724592));
#14584=CARTESIAN_POINT('Ctrl Pts',(-9.65136659729211,0.293655596345414,
15.9418133592485));
#14585=CARTESIAN_POINT('Ctrl Pts',(-9.67581103310559,0.197813707971573,
15.945787864934));
#14586=CARTESIAN_POINT('Ctrl Pts',(-9.6882250000001,0.0989100500913255,
15.9497623706194));
#14587=CARTESIAN_POINT('Ctrl Pts',(-9.688225,-1.18588472375336E-12,15.9537368763049));
#14588=CARTESIAN_POINT('Origin',(-8.5,0.,1.8));
#14589=CARTESIAN_POINT('',(-9.68853128499928,-0.000371837973163785,16.2962631236952));
#14590=CARTESIAN_POINT('',(-9.688225,-1.16018306073329E-12,16.2537368763049));
#14591=CARTESIAN_POINT('',(-9.688225,-1.45515594291686E-16,1.8));
#14592=CARTESIAN_POINT('Ctrl Pts',(-9.68898909271114,-0.000927628473370801,
16.2962631236952));
#14593=CARTESIAN_POINT('Ctrl Pts',(-9.68618839456819,0.331830806210976,
16.28286116413));
#14594=CARTESIAN_POINT('Ctrl Pts',(-9.54051002256345,0.666783184116169,
16.2694592045648));
#14595=CARTESIAN_POINT('Ctrl Pts',(-9.29275770219925,0.88787589629704,16.2560572449997));
#14596=CARTESIAN_POINT('Ctrl Pts',(-8.99869020692162,1.1502999979143,16.240149903848));
#14597=CARTESIAN_POINT('Ctrl Pts',(-8.56081787342036,1.25231518939494,16.2242425626964));
#14598=CARTESIAN_POINT('Ctrl Pts',(-8.18138465234568,1.14687580809469,16.2083352215448));
#14599=CARTESIAN_POINT('Ctrl Pts',(-7.801951431271,1.04143642679444,16.1924278803932));
#14600=CARTESIAN_POINT('Ctrl Pts',(-7.48095732262289,0.728542472713292,
16.1765205392416));
#14601=CARTESIAN_POINT('Ctrl Pts',(-7.36353983692846,0.352071909547143,
16.1606131980899));
#14602=CARTESIAN_POINT('Ctrl Pts',(-7.30483109408124,0.163836627964079,
16.1526595275141));
#14603=CARTESIAN_POINT('Ctrl Pts',(-7.29701650697244,-0.0402928058902354,
16.1447058569383));
#14604=CARTESIAN_POINT('Ctrl Pts',(-7.33630215661051,-0.234917907606526,
16.1367521863625));
#14605=CARTESIAN_POINT('Ctrl Pts',(-7.37558780624859,-0.42954300932284,
16.1287985157867));
#14606=CARTESIAN_POINT('Ctrl Pts',(-7.46197369263355,-0.614663778901128,
16.1208448452109));
#14607=CARTESIAN_POINT('Ctrl Pts',(-7.58911134538717,-0.76538325520993,
16.1128911746351));
#14608=CARTESIAN_POINT('Ctrl Pts',(-7.84338665089437,-1.06682220782752,
16.0969838334835));
#14609=CARTESIAN_POINT('Ctrl Pts',(-8.26066902187615,-1.23065598736718,
16.0810764923318));
#14610=CARTESIAN_POINT('Ctrl Pts',(-8.65127494800788,-1.18064869785899,
16.0651691511802));
#14611=CARTESIAN_POINT('Ctrl Pts',(-9.04188087413961,-1.1306414083508,16.0492618100286));
#14612=CARTESIAN_POINT('Ctrl Pts',(-9.40581035542129,-0.866793049794769,
16.033354468877));
#14613=CARTESIAN_POINT('Ctrl Pts',(-9.57507559972748,-0.510823660624535,
16.0174471277254));
#14614=CARTESIAN_POINT('Ctrl Pts',(-9.65021314331775,-0.352807373198149,
16.0103857930486));
#14615=CARTESIAN_POINT('Ctrl Pts',(-9.6869919257318,-0.176638554687772,
16.0033244583719));
#14616=CARTESIAN_POINT('Ctrl Pts',(-9.68646940363724,-0.000293574405992758,
15.9962631236952));
#14617=CARTESIAN_POINT('Ctrl Pts',(-9.688225,-1.18588472375336E-12,15.9537368763049));
#14618=CARTESIAN_POINT('Ctrl Pts',(-9.6882249999997,-0.298712821307291,
15.9657400630942));
#14619=CARTESIAN_POINT('Ctrl Pts',(-9.57054245632526,-0.595858078272619,
15.9777432498835));
#14620=CARTESIAN_POINT('Ctrl Pts',(-9.36601586214851,-0.813569405233608,
15.9897464366728));
#14621=CARTESIAN_POINT('Ctrl Pts',(-9.16148926797177,-1.0312807321946,16.0017496234622));
#14622=CARTESIAN_POINT('Ctrl Pts',(-8.87226522412724,-1.16727314847175,
16.0137528102515));
#14623=CARTESIAN_POINT('Ctrl Pts',(-8.57413435701325,-1.18591009260198,
16.0257559970408));
#14624=CARTESIAN_POINT('Ctrl Pts',(-8.27600348989926,-1.20454703673221,
16.0377591838301));
#14625=CARTESIAN_POINT('Ctrl Pts',(-7.97209482031977,-1.10563290540054,
16.0497623706194));
#14626=CARTESIAN_POINT('Ctrl Pts',(-7.74204705371964,-0.915087963995769,
16.0617655574088));
#14627=CARTESIAN_POINT('Ctrl Pts',(-7.51199928711951,-0.724543022591,16.0737687441981));
#14628=CARTESIAN_POINT('Ctrl Pts',(-7.35822688079586,-0.444367128060239,
16.0857719309874));
#14629=CARTESIAN_POINT('Ctrl Pts',(-7.32102560975801,-0.147979855989016,
16.0977751177767));
#14630=CARTESIAN_POINT('Ctrl Pts',(-7.28382433872016,0.148407416082207,
16.109778304566));
#14631=CARTESIAN_POINT('Ctrl Pts',(-7.36358464744687,0.457895344723212,
16.1217814913553));
#14632=CARTESIAN_POINT('Ctrl Pts',(-7.5394054943796,0.699383189958763,16.1337846781447));
#14633=CARTESIAN_POINT('Ctrl Pts',(-7.71522634131233,0.940871035194315,
16.145787864934));
#14634=CARTESIAN_POINT('Ctrl Pts',(-7.98526240565909,1.11182427083141,16.1577910517233));
#14635=CARTESIAN_POINT('Ctrl Pts',(-8.27875123560249,1.16744491727772,16.1697942385126));
#14636=CARTESIAN_POINT('Ctrl Pts',(-8.5722400655459,1.22306556372403,16.1817974253019));
#14637=CARTESIAN_POINT('Ctrl Pts',(-8.88610136060075,1.1627698566698,16.1938006120913));
#14638=CARTESIAN_POINT('Ctrl Pts',(-9.1380883482021,1.00235817476275,16.2058037988806));
#14639=CARTESIAN_POINT('Ctrl Pts',(-9.39007533580346,0.841946492855702,
16.2178069856699));
#14640=CARTESIAN_POINT('Ctrl Pts',(-9.57754329642206,0.583102430601644,
16.2298101724592));
#14641=CARTESIAN_POINT('Ctrl Pts',(-9.65136659729226,0.29365559634485,16.2418133592485));
#14642=CARTESIAN_POINT('Ctrl Pts',(-9.67581103310564,0.197813707971193,
16.245787864934));
#14643=CARTESIAN_POINT('Ctrl Pts',(-9.6882250000001,0.0989100500911486,
16.2497623706194));
#14644=CARTESIAN_POINT('Ctrl Pts',(-9.688225,-1.16018306073329E-12,16.2537368763049));
#14645=CARTESIAN_POINT('Origin',(-8.5,0.,1.8));
#14646=CARTESIAN_POINT('',(-9.688225,5.82645043323282E-13,16.5962631236952));
#14647=CARTESIAN_POINT('',(-9.688225,-1.13453690886445E-12,16.5537368763049));
#14648=CARTESIAN_POINT('',(-9.688225,-1.45515594291686E-16,1.8));
#14649=CARTESIAN_POINT('Ctrl Pts',(-9.688225,5.82645043323282E-13,16.5962631236952));
#14650=CARTESIAN_POINT('Ctrl Pts',(-9.68822499999986,0.298712821306687,
16.5842599369058));
#14651=CARTESIAN_POINT('Ctrl Pts',(-9.57054245632556,0.595858078272076,
16.5722567501165));
#14652=CARTESIAN_POINT('Ctrl Pts',(-9.36601586214893,0.813569405233169,
16.5602535633272));
#14653=CARTESIAN_POINT('Ctrl Pts',(-9.16148926797229,1.03128073219426,16.5482503765379));
#14654=CARTESIAN_POINT('Ctrl Pts',(-8.87226522412784,1.16727314847156,16.5362471897486));
#14655=CARTESIAN_POINT('Ctrl Pts',(-8.57413435701386,1.18591009260194,16.5242440029592));
#14656=CARTESIAN_POINT('Ctrl Pts',(-8.27600348989987,1.20454703673232,16.5122408161699));
#14657=CARTESIAN_POINT('Ctrl Pts',(-7.97209482032033,1.10563290540081,16.5002376293806));
#14658=CARTESIAN_POINT('Ctrl Pts',(-7.7420470537201,0.915087963996154,16.4882344425913));
#14659=CARTESIAN_POINT('Ctrl Pts',(-7.51199928711988,0.724543022591502,
16.476231255802));
#14660=CARTESIAN_POINT('Ctrl Pts',(-7.35822688079609,0.444367128060818,
16.4642280690127));
#14661=CARTESIAN_POINT('Ctrl Pts',(-7.32102560975809,0.147979855989614,
16.4522248822233));
#14662=CARTESIAN_POINT('Ctrl Pts',(-7.28382433872008,-0.14840741608159,
16.440221695434));
#14663=CARTESIAN_POINT('Ctrl Pts',(-7.36358464744663,-0.457895344722635,
16.4282185086447));
#14664=CARTESIAN_POINT('Ctrl Pts',(-7.53940549437924,-0.699383189958276,
16.4162153218554));
#14665=CARTESIAN_POINT('Ctrl Pts',(-7.71522634131185,-0.940871035193917,
16.4042121350661));
#14666=CARTESIAN_POINT('Ctrl Pts',(-7.98526240565853,-1.11182427083114,
16.3922089482767));
#14667=CARTESIAN_POINT('Ctrl Pts',(-8.2787512356019,-1.16744491727761,16.3802057614874));
#14668=CARTESIAN_POINT('Ctrl Pts',(-8.57224006554527,-1.22306556372407,
16.3682025746981));
#14669=CARTESIAN_POINT('Ctrl Pts',(-8.88610136060016,-1.16276985666999,
16.3561993879088));
#14670=CARTESIAN_POINT('Ctrl Pts',(-9.13808834820159,-1.00235817476307,
16.3441962011195));
#14671=CARTESIAN_POINT('Ctrl Pts',(-9.39007533580303,-0.841946492856155,
16.3321930143302));
#14672=CARTESIAN_POINT('Ctrl Pts',(-9.57754329642176,-0.583102430602191,
16.3201898275408));
#14673=CARTESIAN_POINT('Ctrl Pts',(-9.65136659729211,-0.293655596345434,
16.3081866407515));
#14674=CARTESIAN_POINT('Ctrl Pts',(-9.67581103310554,-0.197813707971768,
16.3042121350661));
#14675=CARTESIAN_POINT('Ctrl Pts',(-9.68822500000005,-0.0989100500917069,
16.3002376293806));
#14676=CARTESIAN_POINT('Ctrl Pts',(-9.688225,6.24500451351651E-13,16.2962631236952));
#14677=CARTESIAN_POINT('Ctrl Pts',(-9.688225,-1.16018306073329E-12,16.2537368763049));
#14678=CARTESIAN_POINT('Ctrl Pts',(-9.68822499999971,-0.298712821307242,
16.2657400630942));
#14679=CARTESIAN_POINT('Ctrl Pts',(-9.57054245632529,-0.595858078272552,
16.2777432498835));
#14680=CARTESIAN_POINT('Ctrl Pts',(-9.36601586214858,-0.81356940523354,
16.2897464366728));
#14681=CARTESIAN_POINT('Ctrl Pts',(-9.16148926797187,-1.03128073219453,
16.3017496234622));
#14682=CARTESIAN_POINT('Ctrl Pts',(-8.87226522412738,-1.1672731484717,16.3137528102515));
#14683=CARTESIAN_POINT('Ctrl Pts',(-8.57413435701341,-1.18591009260197,
16.3257559970408));
#14684=CARTESIAN_POINT('Ctrl Pts',(-8.27600348989945,-1.20454703673224,
16.3377591838301));
#14685=CARTESIAN_POINT('Ctrl Pts',(-7.97209482031996,-1.10563290540062,
16.3497623706194));
#14686=CARTESIAN_POINT('Ctrl Pts',(-7.74204705371982,-0.915087963995914,
16.3617655574087));
#14687=CARTESIAN_POINT('Ctrl Pts',(-7.51199928711967,-0.724543022591205,
16.3737687441981));
#14688=CARTESIAN_POINT('Ctrl Pts',(-7.35822688079597,-0.4443671280605,16.3857719309874));
#14689=CARTESIAN_POINT('Ctrl Pts',(-7.32102560975805,-0.147979855989309,
16.3977751177767));
#14690=CARTESIAN_POINT('Ctrl Pts',(-7.28382433872013,0.148407416081883,
16.409778304566));
#14691=CARTESIAN_POINT('Ctrl Pts',(-7.36358464744674,0.457895344722883,
16.4217814913553));
#14692=CARTESIAN_POINT('Ctrl Pts',(-7.53940549437938,0.69938318995847,16.4337846781446));
#14693=CARTESIAN_POINT('Ctrl Pts',(-7.71522634131203,0.940871035194057,
16.445787864934));
#14694=CARTESIAN_POINT('Ctrl Pts',(-7.98526240565871,1.11182427083122,16.4577910517233));
#14695=CARTESIAN_POINT('Ctrl Pts',(-8.27875123560207,1.16744491727764,16.4697942385126));
#14696=CARTESIAN_POINT('Ctrl Pts',(-8.57224006554543,1.22306556372405,16.4817974253019));
#14697=CARTESIAN_POINT('Ctrl Pts',(-8.88610136060028,1.16276985666995,16.4938006120912));
#14698=CARTESIAN_POINT('Ctrl Pts',(-9.13808834820168,1.00235817476302,16.5058037988806));
#14699=CARTESIAN_POINT('Ctrl Pts',(-9.39007533580308,0.841946492856088,
16.5178069856699));
#14700=CARTESIAN_POINT('Ctrl Pts',(-9.57754329642178,0.583102430602136,
16.5298101724592));
#14701=CARTESIAN_POINT('Ctrl Pts',(-9.65136659729212,0.293655596345398,
16.5418133592485));
#14702=CARTESIAN_POINT('Ctrl Pts',(-9.67581103310558,0.1978137079716,16.545787864934));
#14703=CARTESIAN_POINT('Ctrl Pts',(-9.68822500000009,0.0989100500913994,
16.5497623706194));
#14704=CARTESIAN_POINT('Ctrl Pts',(-9.688225,-1.06703534896724E-12,16.5537368763049));
#14705=CARTESIAN_POINT('Origin',(-8.5,0.,1.8));
#14706=CARTESIAN_POINT('',(-9.688225,6.08291195192123E-13,16.8962631236952));
#14707=CARTESIAN_POINT('',(-9.688225,-1.10900177929807E-12,16.8537368763049));
#14708=CARTESIAN_POINT('',(-9.688225,-1.45515594291686E-16,1.8));
#14709=CARTESIAN_POINT('Ctrl Pts',(-9.688225,5.40789635294914E-13,16.8962631236952));
#14710=CARTESIAN_POINT('Ctrl Pts',(-9.68822499999986,0.298712821306646,
16.8842599369058));
#14711=CARTESIAN_POINT('Ctrl Pts',(-9.57054245632558,0.595858078272038,
16.8722567501165));
#14712=CARTESIAN_POINT('Ctrl Pts',(-9.36601586214896,0.813569405233138,
16.8602535633272));
#14713=CARTESIAN_POINT('Ctrl Pts',(-9.16148926797233,1.03128073219424,16.8482503765379));
#14714=CARTESIAN_POINT('Ctrl Pts',(-8.87226522412788,1.16727314847155,16.8362471897486));
#14715=CARTESIAN_POINT('Ctrl Pts',(-8.5741343570139,1.18591009260194,16.8242440029592));
#14716=CARTESIAN_POINT('Ctrl Pts',(-8.27600348989992,1.20454703673233,16.8122408161699));
#14717=CARTESIAN_POINT('Ctrl Pts',(-7.97209482032037,1.10563290540082,16.8002376293806));
#14718=CARTESIAN_POINT('Ctrl Pts',(-7.74204705372014,0.915087963996181,
16.7882344425913));
#14719=CARTESIAN_POINT('Ctrl Pts',(-7.51199928711991,0.724543022591537,
16.776231255802));
#14720=CARTESIAN_POINT('Ctrl Pts',(-7.3582268807961,0.444367128060859,16.7642280690127));
#14721=CARTESIAN_POINT('Ctrl Pts',(-7.32102560975809,0.147979855989656,
16.7522248822233));
#14722=CARTESIAN_POINT('Ctrl Pts',(-7.28382433872008,-0.148407416081547,
16.740221695434));
#14723=CARTESIAN_POINT('Ctrl Pts',(-7.36358464744662,-0.457895344722595,
16.7282185086447));
#14724=CARTESIAN_POINT('Ctrl Pts',(-7.53940549437922,-0.699383189958242,
16.7162153218554));
#14725=CARTESIAN_POINT('Ctrl Pts',(-7.71522634131182,-0.940871035193889,
16.7042121350661));
#14726=CARTESIAN_POINT('Ctrl Pts',(-7.98526240565849,-1.11182427083113,
16.6922089482767));
#14727=CARTESIAN_POINT('Ctrl Pts',(-8.27875123560186,-1.1674449172776,16.6802057614874));
#14728=CARTESIAN_POINT('Ctrl Pts',(-8.57224006554523,-1.22306556372407,
16.6682025746981));
#14729=CARTESIAN_POINT('Ctrl Pts',(-8.88610136060012,-1.16276985667001,
16.6561993879088));
#14730=CARTESIAN_POINT('Ctrl Pts',(-9.13808834820156,-1.0023581747631,16.6441962011195));
#14731=CARTESIAN_POINT('Ctrl Pts',(-9.390075335803,-0.841946492856186,16.6321930143302));
#14732=CARTESIAN_POINT('Ctrl Pts',(-9.57754329642174,-0.58310243060223,
16.6201898275408));
#14733=CARTESIAN_POINT('Ctrl Pts',(-9.6513665972921,-0.293655596345475,
16.6081866407515));
#14734=CARTESIAN_POINT('Ctrl Pts',(-9.67581103310554,-0.19781370797181,
16.6042121350661));
#14735=CARTESIAN_POINT('Ctrl Pts',(-9.68822500000005,-0.0989100500917488,
16.6002376293806));
#14736=CARTESIAN_POINT('Ctrl Pts',(-9.688225,5.82645043323282E-13,16.5962631236952));
#14737=CARTESIAN_POINT('Ctrl Pts',(-9.688225,-1.06703534896724E-12,16.5537368763049));
#14738=CARTESIAN_POINT('Ctrl Pts',(-9.68822499999973,-0.298712821307149,
16.5657400630942));
#14739=CARTESIAN_POINT('Ctrl Pts',(-9.57054245632533,-0.595858078272468,
16.5777432498835));
#14740=CARTESIAN_POINT('Ctrl Pts',(-9.36601586214864,-0.813569405233472,
16.5897464366728));
#14741=CARTESIAN_POINT('Ctrl Pts',(-9.16148926797195,-1.03128073219448,
16.6017496234622));
#14742=CARTESIAN_POINT('Ctrl Pts',(-8.87226522412747,-1.16727314847167,
16.6137528102515));
#14743=CARTESIAN_POINT('Ctrl Pts',(-8.57413435701351,-1.18591009260196,
16.6257559970408));
#14744=CARTESIAN_POINT('Ctrl Pts',(-8.27600348989954,-1.20454703673225,
16.6377591838301));
#14745=CARTESIAN_POINT('Ctrl Pts',(-7.97209482032005,-1.10563290540067,
16.6497623706194));
#14746=CARTESIAN_POINT('Ctrl Pts',(-7.74204705371989,-0.915087963995974,
16.6617655574087));
#14747=CARTESIAN_POINT('Ctrl Pts',(-7.51199928711973,-0.724543022591282,
16.6737687441981));
#14748=CARTESIAN_POINT('Ctrl Pts',(-7.358226880796,-0.44436712806059,16.6857719309874));
#14749=CARTESIAN_POINT('Ctrl Pts',(-7.32102560975806,-0.147979855989401,
16.6977751177767));
#14750=CARTESIAN_POINT('Ctrl Pts',(-7.28382433872012,0.148407416081787,
16.709778304566));
#14751=CARTESIAN_POINT('Ctrl Pts',(-7.3635846474467,0.457895344722794,16.7217814913553));
#14752=CARTESIAN_POINT('Ctrl Pts',(-7.53940549437933,0.699383189958394,
16.7337846781446));
#14753=CARTESIAN_POINT('Ctrl Pts',(-7.71522634131196,0.940871035193995,
16.745787864934));
#14754=CARTESIAN_POINT('Ctrl Pts',(-7.98526240565862,1.11182427083118,16.7577910517233));
#14755=CARTESIAN_POINT('Ctrl Pts',(-8.27875123560198,1.16744491727762,16.7697942385126));
#14756=CARTESIAN_POINT('Ctrl Pts',(-8.57224006554533,1.22306556372406,16.7817974253019));
#14757=CARTESIAN_POINT('Ctrl Pts',(-8.88610136060019,1.16276985666998,16.7938006120912));
#14758=CARTESIAN_POINT('Ctrl Pts',(-9.1380883482016,1.00235817476307,16.8058037988806));
#14759=CARTESIAN_POINT('Ctrl Pts',(-9.39007533580302,0.841946492856158,
16.8178069856699));
#14760=CARTESIAN_POINT('Ctrl Pts',(-9.57754329642174,0.58310243060222,16.8298101724592));
#14761=CARTESIAN_POINT('Ctrl Pts',(-9.65136659729209,0.293655596345488,
16.8418133592485));
#14762=CARTESIAN_POINT('Ctrl Pts',(-9.67581103310557,0.197813707971671,
16.845787864934));
#14763=CARTESIAN_POINT('Ctrl Pts',(-9.68822500000009,0.0989100500914474,
16.8497623706194));
#14764=CARTESIAN_POINT('Ctrl Pts',(-9.688225,-1.04144470824963E-12,16.8537368763049));
#14765=CARTESIAN_POINT('Origin',(-8.5,0.,1.8));
#14766=CARTESIAN_POINT('',(-9.688225,6.33826324758502E-13,17.1962631236952));
#14767=CARTESIAN_POINT('',(-9.688225,-1.083300116278E-12,17.1537368763049));
#14768=CARTESIAN_POINT('',(-9.688225,-1.45515594291686E-16,1.8));
#14769=CARTESIAN_POINT('Ctrl Pts',(-9.688225,6.33826324758502E-13,17.1962631236952));
#14770=CARTESIAN_POINT('Ctrl Pts',(-9.68822499999984,0.298712821306739,
17.1842599369058));
#14771=CARTESIAN_POINT('Ctrl Pts',(-9.57054245632553,0.595858078272122,
17.1722567501165));
#14772=CARTESIAN_POINT('Ctrl Pts',(-9.36601586214889,0.813569405233206,
17.1602535633272));
#14773=CARTESIAN_POINT('Ctrl Pts',(-9.16148926797225,1.03128073219429,17.1482503765379));
#14774=CARTESIAN_POINT('Ctrl Pts',(-8.87226522412779,1.16727314847158,17.1362471897486));
#14775=CARTESIAN_POINT('Ctrl Pts',(-8.5741343570138,1.18591009260194,17.1242440029592));
#14776=CARTESIAN_POINT('Ctrl Pts',(-8.27600348989982,1.20454703673231,17.1122408161699));
#14777=CARTESIAN_POINT('Ctrl Pts',(-7.97209482032028,1.10563290540078,17.1002376293806));
#14778=CARTESIAN_POINT('Ctrl Pts',(-7.74204705372006,0.915087963996121,
17.0882344425913));
#14779=CARTESIAN_POINT('Ctrl Pts',(-7.51199928711985,0.72454302259146,17.076231255802));
#14780=CARTESIAN_POINT('Ctrl Pts',(-7.35822688079607,0.444367128060769,
17.0642280690127));
#14781=CARTESIAN_POINT('Ctrl Pts',(-7.32102560975808,0.147979855989563,
17.0522248822233));
#14782=CARTESIAN_POINT('Ctrl Pts',(-7.28382433872009,-0.148407416081643,
17.040221695434));
#14783=CARTESIAN_POINT('Ctrl Pts',(-7.36358464744665,-0.457895344722684,
17.0282185086447));
#14784=CARTESIAN_POINT('Ctrl Pts',(-7.53940549437927,-0.699383189958317,
17.0162153218554));
#14785=CARTESIAN_POINT('Ctrl Pts',(-7.71522634131189,-0.94087103519395,
17.0042121350661));
#14786=CARTESIAN_POINT('Ctrl Pts',(-7.98526240565858,-1.11182427083117,
16.9922089482767));
#14787=CARTESIAN_POINT('Ctrl Pts',(-8.27875123560195,-1.16744491727762,
16.9802057614874));
#14788=CARTESIAN_POINT('Ctrl Pts',(-8.57224006554533,-1.22306556372406,
16.9682025746981));
#14789=CARTESIAN_POINT('Ctrl Pts',(-8.88610136060021,-1.16276985666998,
16.9561993879088));
#14790=CARTESIAN_POINT('Ctrl Pts',(-9.13808834820164,-1.00235817476305,
16.9441962011195));
#14791=CARTESIAN_POINT('Ctrl Pts',(-9.39007533580307,-0.841946492856116,
16.9321930143301));
#14792=CARTESIAN_POINT('Ctrl Pts',(-9.57754329642178,-0.583102430602145,
16.9201898275408));
#14793=CARTESIAN_POINT('Ctrl Pts',(-9.65136659729212,-0.293655596345385,
16.9081866407515));
#14794=CARTESIAN_POINT('Ctrl Pts',(-9.67581103310554,-0.197813707971761,
16.9042121350661));
#14795=CARTESIAN_POINT('Ctrl Pts',(-9.68822500000005,-0.0989100500917455,
16.9002376293806));
#14796=CARTESIAN_POINT('Ctrl Pts',(-9.688225,5.40789635294914E-13,16.8962631236952));
#14797=CARTESIAN_POINT('Ctrl Pts',(-9.688225,-1.04144470824963E-12,16.8537368763049));
#14798=CARTESIAN_POINT('Ctrl Pts',(-9.68822499999974,-0.298712821307124,
16.8657400630942));
#14799=CARTESIAN_POINT('Ctrl Pts',(-9.57054245632535,-0.595858078272445,
16.8777432498835));
#14800=CARTESIAN_POINT('Ctrl Pts',(-9.36601586214866,-0.813569405233454,
16.8897464366728));
#14801=CARTESIAN_POINT('Ctrl Pts',(-9.16148926797197,-1.03128073219446,
16.9017496234622));
#14802=CARTESIAN_POINT('Ctrl Pts',(-8.8722652241275,-1.16727314847166,16.9137528102515));
#14803=CARTESIAN_POINT('Ctrl Pts',(-8.57413435701353,-1.18591009260196,
16.9257559970408));
#14804=CARTESIAN_POINT('Ctrl Pts',(-8.27600348989957,-1.20454703673226,
16.9377591838301));
#14805=CARTESIAN_POINT('Ctrl Pts',(-7.97209482032007,-1.10563290540068,
16.9497623706194));
#14806=CARTESIAN_POINT('Ctrl Pts',(-7.74204705371991,-0.91508796399599,
16.9617655574087));
#14807=CARTESIAN_POINT('Ctrl Pts',(-7.51199928711974,-0.724543022591304,
16.9737687441981));
#14808=CARTESIAN_POINT('Ctrl Pts',(-7.35822688079601,-0.444367128060615,
16.9857719309874));
#14809=CARTESIAN_POINT('Ctrl Pts',(-7.32102560975806,-0.147979855989427,
16.9977751177767));
#14810=CARTESIAN_POINT('Ctrl Pts',(-7.28382433872011,0.148407416081761,
17.009778304566));
#14811=CARTESIAN_POINT('Ctrl Pts',(-7.36358464744669,0.457895344722769,
17.0217814913553));
#14812=CARTESIAN_POINT('Ctrl Pts',(-7.53940549437931,0.699383189958374,
17.0337846781446));
#14813=CARTESIAN_POINT('Ctrl Pts',(-7.71522634131194,0.940871035193978,
17.045787864934));
#14814=CARTESIAN_POINT('Ctrl Pts',(-7.9852624056586,1.11182427083117,17.0577910517233));
#14815=CARTESIAN_POINT('Ctrl Pts',(-8.27875123560195,1.16744491727762,17.0697942385126));
#14816=CARTESIAN_POINT('Ctrl Pts',(-8.57224006554531,1.22306556372406,17.0817974253019));
#14817=CARTESIAN_POINT('Ctrl Pts',(-8.88610136060016,1.16276985666999,17.0938006120912));
#14818=CARTESIAN_POINT('Ctrl Pts',(-9.13808834820158,1.00235817476308,17.1058037988805));
#14819=CARTESIAN_POINT('Ctrl Pts',(-9.390075335803,0.841946492856177,17.1178069856699));
#14820=CARTESIAN_POINT('Ctrl Pts',(-9.57754329642172,0.583102430602244,
17.1298101724592));
#14821=CARTESIAN_POINT('Ctrl Pts',(-9.65136659729209,0.293655596345513,
17.1418133592485));
#14822=CARTESIAN_POINT('Ctrl Pts',(-9.67581103310557,0.197813707971696,
17.145787864934));
#14823=CARTESIAN_POINT('Ctrl Pts',(-9.68822500000008,0.0989100500914731,
17.1497623706194));
#14824=CARTESIAN_POINT('Ctrl Pts',(-9.688225,-1.01579855638079E-12,17.1537368763049));
#14825=CARTESIAN_POINT('Origin',(-8.5,0.,1.8));
#14826=CARTESIAN_POINT('',(-9.688225,6.59472476627343E-13,17.4962631236952));
#14827=CARTESIAN_POINT('',(-9.68910276879127,0.000129087185285244,17.4537368763049));
#14828=CARTESIAN_POINT('',(-9.688225,-1.45515594291686E-16,1.8));
#14829=CARTESIAN_POINT('Ctrl Pts',(-9.688225,6.59472476627343E-13,17.4962631236952));
#14830=CARTESIAN_POINT('Ctrl Pts',(-9.68822499999984,0.298712821306742,
17.4842599369058));
#14831=CARTESIAN_POINT('Ctrl Pts',(-9.57054245632554,0.595858078272101,
17.4722567501165));
#14832=CARTESIAN_POINT('Ctrl Pts',(-9.36601586214892,0.813569405233176,
17.4602535633272));
#14833=CARTESIAN_POINT('Ctrl Pts',(-9.1614892679723,1.03128073219425,17.4482503765379));
#14834=CARTESIAN_POINT('Ctrl Pts',(-8.87226522412787,1.16727314847154,17.4362471897486));
#14835=CARTESIAN_POINT('Ctrl Pts',(-8.57413435701391,1.18591009260194,17.4242440029592));
#14836=CARTESIAN_POINT('Ctrl Pts',(-8.27600348989995,1.20454703673233,17.4122408161699));
#14837=CARTESIAN_POINT('Ctrl Pts',(-7.97209482032043,1.10563290540085,17.4002376293806));
#14838=CARTESIAN_POINT('Ctrl Pts',(-7.7420470537202,0.915087963996234,17.3882344425913));
#14839=CARTESIAN_POINT('Ctrl Pts',(-7.51199928711998,0.724543022591621,
17.376231255802));
#14840=CARTESIAN_POINT('Ctrl Pts',(-7.35822688079616,0.444367128060982,
17.3642280690127));
#14841=CARTESIAN_POINT('Ctrl Pts',(-7.32102560975811,0.147979855989806,
17.3522248822233));
#14842=CARTESIAN_POINT('Ctrl Pts',(-7.28382433872006,-0.14840741608137,
17.340221695434));
#14843=CARTESIAN_POINT('Ctrl Pts',(-7.36358464744655,-0.457895344722404,
17.3282185086447));
#14844=CARTESIAN_POINT('Ctrl Pts',(-7.53940549437909,-0.699383189958065,
17.3162153218554));
#14845=CARTESIAN_POINT('Ctrl Pts',(-7.71522634131163,-0.940871035193726,
17.3042121350661));
#14846=CARTESIAN_POINT('Ctrl Pts',(-7.98526240565824,-1.11182427083101,
17.2922089482768));
#14847=CARTESIAN_POINT('Ctrl Pts',(-8.27875123560158,-1.16744491727754,
17.2802057614874));
#14848=CARTESIAN_POINT('Ctrl Pts',(-8.57224006554492,-1.22306556372408,
17.2682025746981));
#14849=CARTESIAN_POINT('Ctrl Pts',(-8.88610136059979,-1.16276985667011,
17.2561993879088));
#14850=CARTESIAN_POINT('Ctrl Pts',(-9.13808834820126,-1.00235817476329,
17.2441962011195));
#14851=CARTESIAN_POINT('Ctrl Pts',(-9.39007533580273,-0.841946492856463,
17.2321930143302));
#14852=CARTESIAN_POINT('Ctrl Pts',(-9.57754329642154,-0.58310243060259,
17.2201898275409));
#14853=CARTESIAN_POINT('Ctrl Pts',(-9.65136659729199,-0.293655596345883,
17.2081866407515));
#14854=CARTESIAN_POINT('Ctrl Pts',(-9.67581103310551,-0.197813707972074,
17.2042121350661));
#14855=CARTESIAN_POINT('Ctrl Pts',(-9.68822500000005,-0.0989100500918551,
17.2002376293806));
#14856=CARTESIAN_POINT('Ctrl Pts',(-9.688225,6.33826324758502E-13,17.1962631236952));
#14857=CARTESIAN_POINT('Ctrl Pts',(-9.688225,-1.01579855638079E-12,17.1537368763049));
#14858=CARTESIAN_POINT('Ctrl Pts',(-9.68822499999974,-0.298712821307098,
17.1657400630942));
#14859=CARTESIAN_POINT('Ctrl Pts',(-9.57054245632536,-0.595858078272422,
17.1777432498835));
#14860=CARTESIAN_POINT('Ctrl Pts',(-9.36601586214868,-0.813569405233435,
17.1897464366728));
#14861=CARTESIAN_POINT('Ctrl Pts',(-9.16148926797199,-1.03128073219445,
17.2017496234622));
#14862=CARTESIAN_POINT('Ctrl Pts',(-8.87226522412752,-1.16727314847165,
17.2137528102515));
#14863=CARTESIAN_POINT('Ctrl Pts',(-8.57413435701356,-1.18591009260196,
17.2257559970408));
#14864=CARTESIAN_POINT('Ctrl Pts',(-8.27600348989959,-1.20454703673226,
17.2377591838301));
#14865=CARTESIAN_POINT('Ctrl Pts',(-7.9720948203201,-1.10563290540069,17.2497623706194));
#14866=CARTESIAN_POINT('Ctrl Pts',(-7.74204705371993,-0.915087963996007,
17.2617655574087));
#14867=CARTESIAN_POINT('Ctrl Pts',(-7.51199928711976,-0.724543022591325,
17.2737687441981));
#14868=CARTESIAN_POINT('Ctrl Pts',(-7.35822688079602,-0.444367128060639,
17.2857719309874));
#14869=CARTESIAN_POINT('Ctrl Pts',(-7.32102560975807,-0.147979855989452,
17.2977751177767));
#14870=CARTESIAN_POINT('Ctrl Pts',(-7.28382433872011,0.148407416081735,
17.309778304566));
#14871=CARTESIAN_POINT('Ctrl Pts',(-7.36358464744668,0.457895344722745,
17.3217814913553));
#14872=CARTESIAN_POINT('Ctrl Pts',(-7.5394054943793,0.699383189958353,17.3337846781446));
#14873=CARTESIAN_POINT('Ctrl Pts',(-7.71522634131192,0.940871035193961,
17.345787864934));
#14874=CARTESIAN_POINT('Ctrl Pts',(-7.98526240565858,1.11182427083116,17.3577910517233));
#14875=CARTESIAN_POINT('Ctrl Pts',(-8.27875123560193,1.16744491727761,17.3697942385126));
#14876=CARTESIAN_POINT('Ctrl Pts',(-8.57224006554528,1.22306556372406,17.3817974253019));
#14877=CARTESIAN_POINT('Ctrl Pts',(-8.88610136060014,1.16276985667,17.3938006120912));
#14878=CARTESIAN_POINT('Ctrl Pts',(-9.13808834820156,1.0023581747631,17.4058037988805));
#14879=CARTESIAN_POINT('Ctrl Pts',(-9.39007533580298,0.841946492856196,
17.4178069856699));
#14880=CARTESIAN_POINT('Ctrl Pts',(-9.57754329642171,0.583102430602267,
17.4298101724592));
#14881=CARTESIAN_POINT('Ctrl Pts',(-9.65136659729208,0.293655596345538,
17.4418133592485));
#14882=CARTESIAN_POINT('Ctrl Pts',(-9.67581103310557,0.1978137079717,17.445787864934));
#14883=CARTESIAN_POINT('Ctrl Pts',(-9.68822500000009,0.0989100500914538,
17.4497623706194));
#14884=CARTESIAN_POINT('Ctrl Pts',(-9.688225,-1.05770947556039E-12,17.4537368763049));
#14885=CARTESIAN_POINT('Origin',(-8.5,0.,1.8));
#14886=CARTESIAN_POINT('',(-9.688225,6.85118628496184E-13,17.7962631236952));
#14887=CARTESIAN_POINT('',(-9.68776597122061,0.000508313949723295,17.7537368763049));
#14888=CARTESIAN_POINT('',(-9.688225,-1.45515594291686E-16,1.8));
#14889=CARTESIAN_POINT('Ctrl Pts',(-9.688225,6.85118628496184E-13,17.7962631236952));
#14890=CARTESIAN_POINT('Ctrl Pts',(-9.68822499999983,0.298712821306812,
17.7842599369058));
#14891=CARTESIAN_POINT('Ctrl Pts',(-9.57054245632549,0.595858078272213,
17.7722567501165));
#14892=CARTESIAN_POINT('Ctrl Pts',(-9.36601586214881,0.813569405233293,
17.7602535633272));
#14893=CARTESIAN_POINT('Ctrl Pts',(-9.16148926797213,1.03128073219437,17.7482503765379));
#14894=CARTESIAN_POINT('Ctrl Pts',(-8.87226522412762,1.16727314847163,17.7362471897486));
#14895=CARTESIAN_POINT('Ctrl Pts',(-8.57413435701362,1.18591009260196,17.7242440029592));
#14896=CARTESIAN_POINT('Ctrl Pts',(-8.27600348989961,1.20454703673228,17.7122408161699));
#14897=CARTESIAN_POINT('Ctrl Pts',(-7.97209482032006,1.10563290540068,17.7002376293806));
#14898=CARTESIAN_POINT('Ctrl Pts',(-7.74204705371987,0.915087963995959,
17.6882344425913));
#14899=CARTESIAN_POINT('Ctrl Pts',(-7.51199928711968,0.724543022591234,
17.676231255802));
#14900=CARTESIAN_POINT('Ctrl Pts',(-7.35822688079595,0.444367128060483,
17.6642280690126));
#14901=CARTESIAN_POINT('Ctrl Pts',(-7.32102560975804,0.147979855989244,
17.6522248822233));
#14902=CARTESIAN_POINT('Ctrl Pts',(-7.28382433872013,-0.148407416081994,
17.640221695434));
#14903=CARTESIAN_POINT('Ctrl Pts',(-7.36358464744679,-0.457895344723038,
17.6282185086447));
#14904=CARTESIAN_POINT('Ctrl Pts',(-7.5394054943795,-0.699383189958632,
17.6162153218554));
#14905=CARTESIAN_POINT('Ctrl Pts',(-7.71522634131221,-0.940871035194226,
17.604212135066));
#14906=CARTESIAN_POINT('Ctrl Pts',(-7.98526240565898,-1.11182427083136,
17.5922089482767));
#14907=CARTESIAN_POINT('Ctrl Pts',(-8.2787512356024,-1.1674449172777,17.5802057614874));
#14908=CARTESIAN_POINT('Ctrl Pts',(-8.57224006554582,-1.22306556372404,
17.5682025746981));
#14909=CARTESIAN_POINT('Ctrl Pts',(-8.8861013606007,-1.16276985666982,17.5561993879088));
#14910=CARTESIAN_POINT('Ctrl Pts',(-9.13808834820208,-1.00235817476277,
17.5441962011194));
#14911=CARTESIAN_POINT('Ctrl Pts',(-9.39007533580346,-0.841946492855711,
17.5321930143301));
#14912=CARTESIAN_POINT('Ctrl Pts',(-9.57754329642207,-0.58310243060163,
17.5201898275408));
#14913=CARTESIAN_POINT('Ctrl Pts',(-9.65136659729227,-0.293655596344811,
17.5081866407515));
#14914=CARTESIAN_POINT('Ctrl Pts',(-9.6758110331056,-0.197813707971328,
17.504212135066));
#14915=CARTESIAN_POINT('Ctrl Pts',(-9.68822500000006,-0.0989100500914692,
17.5002376293806));
#14916=CARTESIAN_POINT('Ctrl Pts',(-9.688225,6.59472476627343E-13,17.4962631236952));
#14917=CARTESIAN_POINT('Ctrl Pts',(-9.69026320655127,0.00029974448077278,
17.4537368763049));
#14918=CARTESIAN_POINT('Ctrl Pts',(-9.68955486729688,-0.386329465614491,
17.4693398230865));
#14919=CARTESIAN_POINT('Ctrl Pts',(-9.48339361754863,-0.77397925042195,
17.4849427698681));
#14920=CARTESIAN_POINT('Ctrl Pts',(-9.16245597895801,-0.988934269126449,
17.5005457166497));
#14921=CARTESIAN_POINT('Ctrl Pts',(-8.83525724035327,-1.20808279681468,
17.5164530578013));
#14922=CARTESIAN_POINT('Ctrl Pts',(-8.38876013652682,-1.24773270561251,
17.5323603989529));
#14923=CARTESIAN_POINT('Ctrl Pts',(-8.02665222357482,-1.09152891264187,
17.5482677401045));
#14924=CARTESIAN_POINT('Ctrl Pts',(-7.84559826709884,-1.01342701615656,
17.5562214106804));
#14925=CARTESIAN_POINT('Ctrl Pts',(-7.68564160834148,-0.886361694229139,
17.5641750812562));
#14926=CARTESIAN_POINT('Ctrl Pts',(-7.56359443378863,-0.729753018927428,
17.572128751832));
#14927=CARTESIAN_POINT('Ctrl Pts',(-7.44154725923576,-0.573144343625699,
17.5800824224078));
#14928=CARTESIAN_POINT('Ctrl Pts',(-7.35740956888742,-0.386992314949683,
17.5880360929836));
#14929=CARTESIAN_POINT('Ctrl Pts',(-7.32590577206228,-0.192344036827784,
17.5959897635594));
#14930=CARTESIAN_POINT('Ctrl Pts',(-7.26289817841198,0.196952519416013,
17.611897104711));
#14931=CARTESIAN_POINT('Ctrl Pts',(-7.41042615885448,0.62023407344335,17.6278044458627));
#14932=CARTESIAN_POINT('Ctrl Pts',(-7.70286921780885,0.883980445933719,
17.6437117870143));
#14933=CARTESIAN_POINT('Ctrl Pts',(-7.99531227676318,1.14772681842406,17.6596191281659));
#14934=CARTESIAN_POINT('Ctrl Pts',(-8.43267041422935,1.25193800937752,17.6755264693175));
#14935=CARTESIAN_POINT('Ctrl Pts',(-8.81296522226336,1.14840913211923,17.6914338104691));
#14936=CARTESIAN_POINT('Ctrl Pts',(-9.19326003029737,1.04488025486095,17.7073411516207));
#14937=CARTESIAN_POINT('Ctrl Pts',(-9.5164915088992,0.733611309390916,17.7232484927724));
#14938=CARTESIAN_POINT('Ctrl Pts',(-9.63496652153152,0.357793699254791,
17.739155833924));
#14939=CARTESIAN_POINT('Ctrl Pts',(-9.67116551426496,0.242965950886986,
17.7440161813843));
#14940=CARTESIAN_POINT('Ctrl Pts',(-9.6882493851827,0.122112236099562,17.7488765288446));
#14941=CARTESIAN_POINT('Ctrl Pts',(-9.68732689617031,0.000994531771981839,
17.7537368763049));
#14942=CARTESIAN_POINT('Origin',(-8.5,0.,1.8));
#14943=CARTESIAN_POINT('',(-9.688225,7.10764780365025E-13,18.0962631236951));
#14944=CARTESIAN_POINT('',(-9.688225,-1.00647268297394E-12,18.0537368763049));
#14945=CARTESIAN_POINT('',(-9.688225,-1.45515594291686E-16,1.8));
#14946=CARTESIAN_POINT('Ctrl Pts',(-9.688225,7.78266340262235E-13,18.0962631236951));
#14947=CARTESIAN_POINT('Ctrl Pts',(-9.68822499999981,0.298712821306883,
18.0842599369058));
#14948=CARTESIAN_POINT('Ctrl Pts',(-9.57054245632546,0.595858078272252,
18.0722567501165));
#14949=CARTESIAN_POINT('Ctrl Pts',(-9.36601586214879,0.813569405233311,
18.0602535633272));
#14950=CARTESIAN_POINT('Ctrl Pts',(-9.16148926797212,1.03128073219437,18.0482503765379));
#14951=CARTESIAN_POINT('Ctrl Pts',(-8.87226522412764,1.16727314847162,18.0362471897486));
#14952=CARTESIAN_POINT('Ctrl Pts',(-8.57413435701366,1.18591009260195,18.0242440029592));
#14953=CARTESIAN_POINT('Ctrl Pts',(-8.27600348989968,1.20454703673229,18.0122408161699));
#14954=CARTESIAN_POINT('Ctrl Pts',(-7.97209482032015,1.10563290540072,18.0002376293806));
#14955=CARTESIAN_POINT('Ctrl Pts',(-7.74204705371995,0.915087963996029,
17.9882344425913));
#14956=CARTESIAN_POINT('Ctrl Pts',(-7.51199928711976,0.72454302259134,17.976231255802));
#14957=CARTESIAN_POINT('Ctrl Pts',(-7.35822688079601,0.44436712806063,17.9642280690126));
#14958=CARTESIAN_POINT('Ctrl Pts',(-7.32102560975806,0.14797985598942,17.9522248822233));
#14959=CARTESIAN_POINT('Ctrl Pts',(-7.28382433872011,-0.148407416081791,
17.940221695434));
#14960=CARTESIAN_POINT('Ctrl Pts',(-7.36358464744671,-0.457895344722822,
17.9282185086447));
#14961=CARTESIAN_POINT('Ctrl Pts',(-7.53940549437936,-0.699383189958434,
17.9162153218554));
#14962=CARTESIAN_POINT('Ctrl Pts',(-7.71522634131201,-0.940871035194046,
17.9042121350661));
#14963=CARTESIAN_POINT('Ctrl Pts',(-7.98526240565871,-1.11182427083123,
17.8922089482767));
#14964=CARTESIAN_POINT('Ctrl Pts',(-8.27875123560209,-1.16744491727764,
17.8802057614874));
#14965=CARTESIAN_POINT('Ctrl Pts',(-8.57224006554548,-1.22306556372405,
17.8682025746981));
#14966=CARTESIAN_POINT('Ctrl Pts',(-8.88610136060035,-1.16276985666993,
17.8561993879088));
#14967=CARTESIAN_POINT('Ctrl Pts',(-9.13808834820176,-1.00235817476297,
17.8441962011195));
#14968=CARTESIAN_POINT('Ctrl Pts',(-9.39007533580317,-0.841946492856008,
17.8321930143301));
#14969=CARTESIAN_POINT('Ctrl Pts',(-9.57754329642185,-0.583102430602014,
17.8201898275408));
#14970=CARTESIAN_POINT('Ctrl Pts',(-9.65136659729216,-0.293655596345245,
17.8081866407515));
#14971=CARTESIAN_POINT('Ctrl Pts',(-9.67581103310557,-0.197813707971618,
17.8042121350661));
#14972=CARTESIAN_POINT('Ctrl Pts',(-9.68822500000006,-0.0989100500916012,
17.8002376293806));
#14973=CARTESIAN_POINT('Ctrl Pts',(-9.688225,6.85118628496184E-13,17.7962631236952));
#14974=CARTESIAN_POINT('Ctrl Pts',(-9.688225,-9.64561763794336E-13,17.7537368763049));
#14975=CARTESIAN_POINT('Ctrl Pts',(-9.68822499999976,-0.298712821307047,
17.7657400630942));
#14976=CARTESIAN_POINT('Ctrl Pts',(-9.57054245632539,-0.595858078272375,
17.7777432498835));
#14977=CARTESIAN_POINT('Ctrl Pts',(-9.36601586214871,-0.813569405233398,
17.7897464366728));
#14978=CARTESIAN_POINT('Ctrl Pts',(-9.16148926797204,-1.03128073219442,
17.8017496234622));
#14979=CARTESIAN_POINT('Ctrl Pts',(-8.87226522412757,-1.16727314847164,
17.8137528102515));
#14980=CARTESIAN_POINT('Ctrl Pts',(-8.57413435701361,-1.18591009260196,
17.8257559970408));
#14981=CARTESIAN_POINT('Ctrl Pts',(-8.27600348989965,-1.20454703673227,
17.8377591838301));
#14982=CARTESIAN_POINT('Ctrl Pts',(-7.97209482032014,-1.10563290540071,
17.8497623706194));
#14983=CARTESIAN_POINT('Ctrl Pts',(-7.74204705371997,-0.915087963996039,
17.8617655574087));
#14984=CARTESIAN_POINT('Ctrl Pts',(-7.51199928711979,-0.724543022591367,
17.8737687441981));
#14985=CARTESIAN_POINT('Ctrl Pts',(-7.35822688079604,-0.444367128060688,
17.8857719309874));
#14986=CARTESIAN_POINT('Ctrl Pts',(-7.32102560975807,-0.147979855989503,
17.8977751177767));
#14987=CARTESIAN_POINT('Ctrl Pts',(-7.2838243387201,0.148407416081682,17.909778304566));
#14988=CARTESIAN_POINT('Ctrl Pts',(-7.36358464744666,0.457895344722696,
17.9217814913553));
#14989=CARTESIAN_POINT('Ctrl Pts',(-7.53940549437927,0.699383189958312,
17.9337846781446));
#14990=CARTESIAN_POINT('Ctrl Pts',(-7.71522634131187,0.940871035193927,
17.945787864934));
#14991=CARTESIAN_POINT('Ctrl Pts',(-7.98526240565853,1.11182427083114,17.9577910517233));
#14992=CARTESIAN_POINT('Ctrl Pts',(-8.27875123560188,1.1674449172776,17.9697942385126));
#14993=CARTESIAN_POINT('Ctrl Pts',(-8.57224006554523,1.22306556372406,17.9817974253019));
#14994=CARTESIAN_POINT('Ctrl Pts',(-8.88610136060009,1.16276985667001,17.9938006120912));
#14995=CARTESIAN_POINT('Ctrl Pts',(-9.13808834820152,1.00235817476312,18.0058037988805));
#14996=CARTESIAN_POINT('Ctrl Pts',(-9.39007533580295,0.841946492856234,
18.0178069856699));
#14997=CARTESIAN_POINT('Ctrl Pts',(-9.57754329642169,0.583102430602313,
18.0298101724592));
#14998=CARTESIAN_POINT('Ctrl Pts',(-9.65136659729207,0.293655596345588,
18.0418133592485));
#14999=CARTESIAN_POINT('Ctrl Pts',(-9.67581103310556,0.197813707971772,
18.045787864934));
#15000=CARTESIAN_POINT('Ctrl Pts',(-9.68822500000008,0.0989100500915499,
18.0497623706194));
#15001=CARTESIAN_POINT('Ctrl Pts',(-9.688225,-9.39026634227957E-13,18.0537368763049));
#15002=CARTESIAN_POINT('Origin',(-8.5,0.,1.8));
#15003=CARTESIAN_POINT('',(-9.688225,7.36299909931404E-13,18.3962631236951));
#15004=CARTESIAN_POINT('',(-9.688225,-9.80826531105095E-13,18.3537368763049));
#15005=CARTESIAN_POINT('',(-9.688225,-1.45515594291686E-16,1.8));
#15006=CARTESIAN_POINT('Ctrl Pts',(-9.688225,7.36299909931404E-13,18.3962631236951));
#15007=CARTESIAN_POINT('Ctrl Pts',(-9.68822499999982,0.298712821306841,
18.3842599369058));
#15008=CARTESIAN_POINT('Ctrl Pts',(-9.57054245632548,0.595858078272214,
18.3722567501165));
#15009=CARTESIAN_POINT('Ctrl Pts',(-9.36601586214882,0.813569405233281,
18.3602535633272));
#15010=CARTESIAN_POINT('Ctrl Pts',(-9.16148926797216,1.03128073219435,18.3482503765379));
#15011=CARTESIAN_POINT('Ctrl Pts',(-8.87226522412768,1.16727314847161,18.3362471897486));
#15012=CARTESIAN_POINT('Ctrl Pts',(-8.5741343570137,1.18591009260195,18.3242440029592));
#15013=CARTESIAN_POINT('Ctrl Pts',(-8.27600348989972,1.20454703673229,18.3122408161699));
#15014=CARTESIAN_POINT('Ctrl Pts',(-7.97209482032018,1.10563290540074,18.3002376293806));
#15015=CARTESIAN_POINT('Ctrl Pts',(-7.74204705371999,0.915087963996056,
18.2882344425913));
#15016=CARTESIAN_POINT('Ctrl Pts',(-7.51199928711979,0.724543022591374,
18.276231255802));
#15017=CARTESIAN_POINT('Ctrl Pts',(-7.35822688079603,0.444367128060671,
18.2642280690126));
#15018=CARTESIAN_POINT('Ctrl Pts',(-7.32102560975807,0.147979855989462,
18.2522248822233));
#15019=CARTESIAN_POINT('Ctrl Pts',(-7.2838243387201,-0.148407416081748,
18.240221695434));
#15020=CARTESIAN_POINT('Ctrl Pts',(-7.36358464744669,-0.457895344722782,
18.2282185086447));
#15021=CARTESIAN_POINT('Ctrl Pts',(-7.53940549437933,-0.6993831899584,18.2162153218554));
#15022=CARTESIAN_POINT('Ctrl Pts',(-7.71522634131197,-0.940871035194018,
18.2042121350661));
#15023=CARTESIAN_POINT('Ctrl Pts',(-7.98526240565867,-1.11182427083121,
18.1922089482767));
#15024=CARTESIAN_POINT('Ctrl Pts',(-8.27875123560205,-1.16744491727763,
18.1802057614874));
#15025=CARTESIAN_POINT('Ctrl Pts',(-8.57224006554543,-1.22306556372406,
18.1682025746981));
#15026=CARTESIAN_POINT('Ctrl Pts',(-8.88610136060031,-1.16276985666994,
18.1561993879088));
#15027=CARTESIAN_POINT('Ctrl Pts',(-9.13808834820172,-1.00235817476299,
18.1441962011195));
#15028=CARTESIAN_POINT('Ctrl Pts',(-9.39007533580314,-0.841946492856039,
18.1321930143301));
#15029=CARTESIAN_POINT('Ctrl Pts',(-9.57754329642183,-0.583102430602052,
18.1201898275408));
#15030=CARTESIAN_POINT('Ctrl Pts',(-9.65136659729215,-0.293655596345285,
18.1081866407515));
#15031=CARTESIAN_POINT('Ctrl Pts',(-9.67581103310557,-0.197813707971616,
18.1042121350661));
#15032=CARTESIAN_POINT('Ctrl Pts',(-9.68822500000006,-0.0989100500915531,
18.1002376293806));
#15033=CARTESIAN_POINT('Ctrl Pts',(-9.688225,7.78266340262235E-13,18.0962631236951));
#15034=CARTESIAN_POINT('Ctrl Pts',(-9.688225,-9.39026634227957E-13,18.0537368763049));
#15035=CARTESIAN_POINT('Ctrl Pts',(-9.68822499999976,-0.298712821307044,
18.0657400630942));
#15036=CARTESIAN_POINT('Ctrl Pts',(-9.57054245632538,-0.595858078272397,
18.0777432498835));
#15037=CARTESIAN_POINT('Ctrl Pts',(-9.36601586214868,-0.813569405233428,
18.0897464366728));
#15038=CARTESIAN_POINT('Ctrl Pts',(-9.16148926797198,-1.03128073219446,
18.1017496234622));
#15039=CARTESIAN_POINT('Ctrl Pts',(-8.87226522412749,-1.16727314847167,
18.1137528102515));
#15040=CARTESIAN_POINT('Ctrl Pts',(-8.5741343570135,-1.18591009260196,18.1257559970408));
#15041=CARTESIAN_POINT('Ctrl Pts',(-8.27600348989951,-1.20454703673225,
18.1377591838301));
#15042=CARTESIAN_POINT('Ctrl Pts',(-7.97209482032,-1.10563290540065,18.1497623706194));
#15043=CARTESIAN_POINT('Ctrl Pts',(-7.74204705371983,-0.915087963995926,
18.1617655574087));
#15044=CARTESIAN_POINT('Ctrl Pts',(-7.51199928711966,-0.724543022591206,
18.1737687441981));
#15045=CARTESIAN_POINT('Ctrl Pts',(-7.35822688079595,-0.444367128060476,
18.1857719309874));
#15046=CARTESIAN_POINT('Ctrl Pts',(-7.32102560975804,-0.147979855989261,
18.1977751177767));
#15047=CARTESIAN_POINT('Ctrl Pts',(-7.28382433872013,0.148407416081955,
18.209778304566));
#15048=CARTESIAN_POINT('Ctrl Pts',(-7.36358464744677,0.457895344722976,
18.2217814913553));
#15049=CARTESIAN_POINT('Ctrl Pts',(-7.53940549437945,0.699383189958564,
18.2337846781447));
#15050=CARTESIAN_POINT('Ctrl Pts',(-7.71522634131214,0.940871035194152,
18.245787864934));
#15051=CARTESIAN_POINT('Ctrl Pts',(-7.98526240565886,1.1118242708313,18.2577910517233));
#15052=CARTESIAN_POINT('Ctrl Pts',(-8.27875123560225,1.16744491727767,18.2697942385126));
#15053=CARTESIAN_POINT('Ctrl Pts',(-8.57224006554564,1.22306556372404,18.2817974253019));
#15054=CARTESIAN_POINT('Ctrl Pts',(-8.88610136060051,1.16276985666988,18.2938006120912));
#15055=CARTESIAN_POINT('Ctrl Pts',(-9.13808834820189,1.00235817476288,18.3058037988806));
#15056=CARTESIAN_POINT('Ctrl Pts',(-9.39007533580328,0.841946492855888,
18.3178069856699));
#15057=CARTESIAN_POINT('Ctrl Pts',(-9.57754329642193,0.583102430601868,
18.3298101724592));
#15058=CARTESIAN_POINT('Ctrl Pts',(-9.6513665972922,0.293655596345089,18.3418133592485));
#15059=CARTESIAN_POINT('Ctrl Pts',(-9.6758110331056,0.197813707971437,18.345787864934));
#15060=CARTESIAN_POINT('Ctrl Pts',(-9.68822500000008,0.0989100500913954,
18.3497623706194));
#15061=CARTESIAN_POINT('Ctrl Pts',(-9.688225,-9.13324971207885E-13,18.3537368763049));
#15062=CARTESIAN_POINT('Origin',(-8.5,0.,1.8));
#15063=CARTESIAN_POINT('',(-9.688225,7.61946061800245E-13,18.6962631236951));
#15064=CARTESIAN_POINT('',(-9.688225,-9.55291401538716E-13,18.6537368763049));
#15065=CARTESIAN_POINT('',(-9.688225,-1.45515594291686E-16,1.8));
#15066=CARTESIAN_POINT('Ctrl Pts',(-9.688225,8.29447621697454E-13,18.6962631236951));
#15067=CARTESIAN_POINT('Ctrl Pts',(-9.68822499999979,0.298712821306934,
18.6842599369058));
#15068=CARTESIAN_POINT('Ctrl Pts',(-9.57054245632543,0.595858078272298,
18.6722567501165));
#15069=CARTESIAN_POINT('Ctrl Pts',(-9.36601586214876,0.813569405233349,
18.6602535633272));
#15070=CARTESIAN_POINT('Ctrl Pts',(-9.16148926797208,1.0312807321944,18.6482503765379));
#15071=CARTESIAN_POINT('Ctrl Pts',(-8.87226522412759,1.16727314847164,18.6362471897486));
#15072=CARTESIAN_POINT('Ctrl Pts',(-8.57413435701361,1.18591009260196,18.6242440029592));
#15073=CARTESIAN_POINT('Ctrl Pts',(-8.27600348989962,1.20454703673228,18.6122408161699));
#15074=CARTESIAN_POINT('Ctrl Pts',(-7.9720948203201,1.1056329054007,18.6002376293806));
#15075=CARTESIAN_POINT('Ctrl Pts',(-7.74204705371991,0.915087963995996,
18.5882344425913));
#15076=CARTESIAN_POINT('Ctrl Pts',(-7.51199928711973,0.724543022591297,
18.576231255802));
#15077=CARTESIAN_POINT('Ctrl Pts',(-7.35822688079599,0.444367128060581,
18.5642280690126));
#15078=CARTESIAN_POINT('Ctrl Pts',(-7.32102560975805,0.147979855989369,
18.5522248822233));
#15079=CARTESIAN_POINT('Ctrl Pts',(-7.28382433872012,-0.148407416081843,
18.540221695434));
#15080=CARTESIAN_POINT('Ctrl Pts',(-7.36358464744673,-0.457895344722872,
18.5282185086447));
#15081=CARTESIAN_POINT('Ctrl Pts',(-7.53940549437939,-0.699383189958476,
18.5162153218554));
#15082=CARTESIAN_POINT('Ctrl Pts',(-7.71522634131205,-0.94087103519408,
18.5042121350661));
#15083=CARTESIAN_POINT('Ctrl Pts',(-7.98526240565876,-1.11182427083125,
18.4922089482767));
#15084=CARTESIAN_POINT('Ctrl Pts',(-8.27875123560214,-1.16744491727765,
18.4802057614874));
#15085=CARTESIAN_POINT('Ctrl Pts',(-8.57224006554553,-1.22306556372405,
18.4682025746981));
#15086=CARTESIAN_POINT('Ctrl Pts',(-8.8861013606004,-1.16276985666991,18.4561993879088));
#15087=CARTESIAN_POINT('Ctrl Pts',(-9.1380883482018,-1.00235817476294,18.4441962011195));
#15088=CARTESIAN_POINT('Ctrl Pts',(-9.3900753358032,-0.84194649285597,18.4321930143301));
#15089=CARTESIAN_POINT('Ctrl Pts',(-9.57754329642188,-0.583102430601968,
18.4201898275408));
#15090=CARTESIAN_POINT('Ctrl Pts',(-9.65136659729217,-0.293655596345195,
18.4081866407515));
#15091=CARTESIAN_POINT('Ctrl Pts',(-9.67581103310557,-0.197813707971568,
18.4042121350661));
#15092=CARTESIAN_POINT('Ctrl Pts',(-9.68822500000006,-0.09891005009155,
18.4002376293806));
#15093=CARTESIAN_POINT('Ctrl Pts',(-9.688225,7.36299909931404E-13,18.3962631236951));
#15094=CARTESIAN_POINT('Ctrl Pts',(-9.688225,-9.13324971207885E-13,18.3537368763049));
#15095=CARTESIAN_POINT('Ctrl Pts',(-9.68822499999977,-0.298712821306996,
18.3657400630942));
#15096=CARTESIAN_POINT('Ctrl Pts',(-9.57054245632541,-0.595858078272329,
18.3777432498835));
#15097=CARTESIAN_POINT('Ctrl Pts',(-9.36601586214875,-0.81356940523336,
18.3897464366728));
#15098=CARTESIAN_POINT('Ctrl Pts',(-9.16148926797208,-1.03128073219439,
18.4017496234621));
#15099=CARTESIAN_POINT('Ctrl Pts',(-8.87226522412762,-1.16727314847162,
18.4137528102515));
#15100=CARTESIAN_POINT('Ctrl Pts',(-8.57413435701366,-1.18591009260195,
18.4257559970408));
#15101=CARTESIAN_POINT('Ctrl Pts',(-8.2760034898997,-1.20454703673228,18.4377591838301));
#15102=CARTESIAN_POINT('Ctrl Pts',(-7.97209482032019,-1.10563290540073,
18.4497623706194));
#15103=CARTESIAN_POINT('Ctrl Pts',(-7.74204705372001,-0.915087963996072,
18.4617655574087));
#15104=CARTESIAN_POINT('Ctrl Pts',(-7.51199928711982,-0.72454302259141,
18.4737687441981));
#15105=CARTESIAN_POINT('Ctrl Pts',(-7.35822688079606,-0.444367128060738,
18.4857719309874));
#15106=CARTESIAN_POINT('Ctrl Pts',(-7.32102560975808,-0.147979855989554,
18.4977751177767));
#15107=CARTESIAN_POINT('Ctrl Pts',(-7.2838243387201,0.14840741608163,18.509778304566));
#15108=CARTESIAN_POINT('Ctrl Pts',(-7.36358464744664,0.457895344722647,
18.5217814913553));
#15109=CARTESIAN_POINT('Ctrl Pts',(-7.53940549437924,0.69938318995827,18.5337846781446));
#15110=CARTESIAN_POINT('Ctrl Pts',(-7.71522634131183,0.940871035193894,
18.545787864934));
#15111=CARTESIAN_POINT('Ctrl Pts',(-7.98526240565848,1.11182427083112,18.5577910517233));
#15112=CARTESIAN_POINT('Ctrl Pts',(-8.27875123560183,1.16744491727759,18.5697942385126));
#15113=CARTESIAN_POINT('Ctrl Pts',(-8.57224006554518,1.22306556372407,18.5817974253019));
#15114=CARTESIAN_POINT('Ctrl Pts',(-8.88610136060004,1.16276985667003,18.5938006120912));
#15115=CARTESIAN_POINT('Ctrl Pts',(-9.13808834820147,1.00235817476315,18.6058037988805));
#15116=CARTESIAN_POINT('Ctrl Pts',(-9.39007533580291,0.841946492856273,
18.6178069856699));
#15117=CARTESIAN_POINT('Ctrl Pts',(-9.57754329642166,0.58310243060236,18.6298101724592));
#15118=CARTESIAN_POINT('Ctrl Pts',(-9.65136659729206,0.293655596345638,
18.6418133592485));
#15119=CARTESIAN_POINT('Ctrl Pts',(-9.67581103310556,0.197813707971779,
18.645787864934));
#15120=CARTESIAN_POINT('Ctrl Pts',(-9.68822500000008,0.0989100500915112,
18.6497623706194));
#15121=CARTESIAN_POINT('Ctrl Pts',(-9.688225,-1.02273745028469E-12,18.6537368763049));
#15122=CARTESIAN_POINT('Origin',(-8.5,0.,1.8));
#15123=CARTESIAN_POINT('',(-9.688225,7.87592213669086E-13,18.9962631236951));
#15124=CARTESIAN_POINT('',(-9.688225,-9.29589738518644E-13,18.9537368763049));
#15125=CARTESIAN_POINT('',(-9.688225,-1.45515594291686E-16,1.8));
#15126=CARTESIAN_POINT('Ctrl Pts',(-9.688225,7.87592213669086E-13,18.9962631236951));
#15127=CARTESIAN_POINT('Ctrl Pts',(-9.6882249999998,0.29871282130687,18.9842599369058));
#15128=CARTESIAN_POINT('Ctrl Pts',(-9.57054245632547,0.595858078272216,
18.9722567501165));
#15129=CARTESIAN_POINT('Ctrl Pts',(-9.36601586214883,0.813569405233269,
18.9602535633272));
#15130=CARTESIAN_POINT('Ctrl Pts',(-9.16148926797219,1.03128073219432,18.9482503765379));
#15131=CARTESIAN_POINT('Ctrl Pts',(-8.87226522412774,1.16727314847158,18.9362471897486));
#15132=CARTESIAN_POINT('Ctrl Pts',(-8.57413435701378,1.18591009260194,18.9242440029592));
#15133=CARTESIAN_POINT('Ctrl Pts',(-8.27600348989982,1.20454703673231,18.9122408161699));
#15134=CARTESIAN_POINT('Ctrl Pts',(-7.97209482032031,1.10563290540079,18.9002376293806));
#15135=CARTESIAN_POINT('Ctrl Pts',(-7.7420470537201,0.915087963996152,18.8882344425913));
#15136=CARTESIAN_POINT('Ctrl Pts',(-7.5119992871199,0.724543022591515,18.876231255802));
#15137=CARTESIAN_POINT('Ctrl Pts',(-7.35822688079611,0.444367128060859,
18.8642280690127));
#15138=CARTESIAN_POINT('Ctrl Pts',(-7.32102560975809,0.147979855989679,
18.8522248822233));
#15139=CARTESIAN_POINT('Ctrl Pts',(-7.28382433872008,-0.148407416081501,
18.840221695434));
#15140=CARTESIAN_POINT('Ctrl Pts',(-7.3635846474466,-0.457895344722527,
18.8282185086447));
#15141=CARTESIAN_POINT('Ctrl Pts',(-7.53940549437916,-0.699383189958169,
18.8162153218554));
#15142=CARTESIAN_POINT('Ctrl Pts',(-7.71522634131173,-0.940871035193811,
18.8042121350661));
#15143=CARTESIAN_POINT('Ctrl Pts',(-7.98526240565836,-1.11182427083106,
18.7922089482768));
#15144=CARTESIAN_POINT('Ctrl Pts',(-8.27875123560171,-1.16744491727757,
18.7802057614874));
#15145=CARTESIAN_POINT('Ctrl Pts',(-8.57224006554505,-1.22306556372407,
18.7682025746981));
#15146=CARTESIAN_POINT('Ctrl Pts',(-8.88610136059992,-1.16276985667007,
18.7561993879088));
#15147=CARTESIAN_POINT('Ctrl Pts',(-9.13808834820137,-1.00235817476322,
18.7441962011195));
#15148=CARTESIAN_POINT('Ctrl Pts',(-9.39007533580282,-0.841946492856367,
18.7321930143302));
#15149=CARTESIAN_POINT('Ctrl Pts',(-9.5775432964216,-0.583102430602474,
18.7201898275408));
#15150=CARTESIAN_POINT('Ctrl Pts',(-9.65136659729203,-0.293655596345759,
18.7081866407515));
#15151=CARTESIAN_POINT('Ctrl Pts',(-9.67581103310553,-0.197813707971926,
18.7042121350661));
#15152=CARTESIAN_POINT('Ctrl Pts',(-9.68822500000007,-0.0989100500916821,
18.7002376293806));
#15153=CARTESIAN_POINT('Ctrl Pts',(-9.688225,8.29447621697454E-13,18.6962631236951));
#15154=CARTESIAN_POINT('Ctrl Pts',(-9.688225,-1.02273745028469E-12,18.6537368763049));
#15155=CARTESIAN_POINT('Ctrl Pts',(-9.68822499999974,-0.298712821307128,
18.6657400630942));
#15156=CARTESIAN_POINT('Ctrl Pts',(-9.57054245632534,-0.595858078272472,
18.6777432498835));
#15157=CARTESIAN_POINT('Ctrl Pts',(-9.36601586214863,-0.813569405233489,
18.6897464366728));
#15158=CARTESIAN_POINT('Ctrl Pts',(-9.16148926797191,-1.03128073219451,
18.7017496234622));
#15159=CARTESIAN_POINT('Ctrl Pts',(-8.8722652241274,-1.1672731484717,18.7137528102515));
#15160=CARTESIAN_POINT('Ctrl Pts',(-8.57413435701342,-1.18591009260197,
18.7257559970408));
#15161=CARTESIAN_POINT('Ctrl Pts',(-8.27600348989943,-1.20454703673224,
18.7377591838301));
#15162=CARTESIAN_POINT('Ctrl Pts',(-7.97209482031992,-1.10563290540061,
18.7497623706194));
#15163=CARTESIAN_POINT('Ctrl Pts',(-7.74204705371976,-0.915087963995873,
18.7617655574087));
#15164=CARTESIAN_POINT('Ctrl Pts',(-7.51199928711961,-0.724543022591136,
18.7737687441981));
#15165=CARTESIAN_POINT('Ctrl Pts',(-7.35822688079592,-0.444367128060395,
18.7857719309874));
#15166=CARTESIAN_POINT('Ctrl Pts',(-7.32102560975803,-0.147979855989177,
18.7977751177767));
#15167=CARTESIAN_POINT('Ctrl Pts',(-7.28382433872014,0.148407416082041,
18.809778304566));
#15168=CARTESIAN_POINT('Ctrl Pts',(-7.3635846474468,0.457895344723056,18.8217814913553));
#15169=CARTESIAN_POINT('Ctrl Pts',(-7.5394054943795,0.699383189958632,18.8337846781447));
#15170=CARTESIAN_POINT('Ctrl Pts',(-7.7152263413122,0.940871035194207,18.845787864934));
#15171=CARTESIAN_POINT('Ctrl Pts',(-7.98526240565894,1.11182427083134,18.8577910517233));
#15172=CARTESIAN_POINT('Ctrl Pts',(-8.27875123560233,1.16744491727769,18.8697942385126));
#15173=CARTESIAN_POINT('Ctrl Pts',(-8.57224006554573,1.22306556372404,18.8817974253019));
#15174=CARTESIAN_POINT('Ctrl Pts',(-8.88610136060059,1.16276985666985,18.8938006120912));
#15175=CARTESIAN_POINT('Ctrl Pts',(-9.13808834820196,1.00235817476284,18.9058037988806));
#15176=CARTESIAN_POINT('Ctrl Pts',(-9.39007533580334,0.841946492855824,
18.9178069856699));
#15177=CARTESIAN_POINT('Ctrl Pts',(-9.57754329642197,0.583102430601792,
18.9298101724592));
#15178=CARTESIAN_POINT('Ctrl Pts',(-9.65136659729222,0.293655596345008,
18.9418133592485));
#15179=CARTESIAN_POINT('Ctrl Pts',(-9.6758110331056,0.197813707971398,18.945787864934));
#15180=CARTESIAN_POINT('Ctrl Pts',(-9.68822500000007,0.0989100500914017,
18.9497623706194));
#15181=CARTESIAN_POINT('Ctrl Pts',(-9.688225,-8.62088178621434E-13,18.9537368763049));
#15182=CARTESIAN_POINT('Origin',(-8.5,0.,1.8));
#15183=CARTESIAN_POINT('',(-9.68783295262227,-0.000517608156923501,19.2962631236951));
#15184=CARTESIAN_POINT('',(-9.688225,-9.03999097801034E-13,19.2537368763049));
#15185=CARTESIAN_POINT('',(-9.688225,-1.45515594291686E-16,1.8));
#15186=CARTESIAN_POINT('Ctrl Pts',(-9.688225,8.80739925435137E-13,19.2962631236951));
#15187=CARTESIAN_POINT('Ctrl Pts',(-9.68822499999978,0.298712821306963,
19.2842599369058));
#15188=CARTESIAN_POINT('Ctrl Pts',(-9.57054245632543,0.5958580782723,19.2722567501165));
#15189=CARTESIAN_POINT('Ctrl Pts',(-9.36601586214877,0.813569405233337,
19.2602535633272));
#15190=CARTESIAN_POINT('Ctrl Pts',(-9.16148926797211,1.03128073219437,19.2482503765379));
#15191=CARTESIAN_POINT('Ctrl Pts',(-8.87226522412765,1.16727314847161,19.2362471897486));
#15192=CARTESIAN_POINT('Ctrl Pts',(-8.57413435701369,1.18591009260195,19.2242440029592));
#15193=CARTESIAN_POINT('Ctrl Pts',(-8.27600348989973,1.20454703673229,19.2122408161699));
#15194=CARTESIAN_POINT('Ctrl Pts',(-7.97209482032022,1.10563290540075,19.2002376293806));
#15195=CARTESIAN_POINT('Ctrl Pts',(-7.74204705372003,0.915087963996093,
19.1882344425913));
#15196=CARTESIAN_POINT('Ctrl Pts',(-7.51199928711984,0.724543022591437,
19.176231255802));
#15197=CARTESIAN_POINT('Ctrl Pts',(-7.35822688079607,0.444367128060769,
19.1642280690127));
#15198=CARTESIAN_POINT('Ctrl Pts',(-7.32102560975808,0.147979855989586,
19.1522248822233));
#15199=CARTESIAN_POINT('Ctrl Pts',(-7.28382433872009,-0.148407416081596,
19.140221695434));
#15200=CARTESIAN_POINT('Ctrl Pts',(-7.36358464744663,-0.457895344722616,
19.1282185086447));
#15201=CARTESIAN_POINT('Ctrl Pts',(-7.53940549437922,-0.699383189958244,
19.1162153218554));
#15202=CARTESIAN_POINT('Ctrl Pts',(-7.71522634131181,-0.940871035193872,
19.1042121350661));
#15203=CARTESIAN_POINT('Ctrl Pts',(-7.98526240565845,-1.1118242708311,19.0922089482767));
#15204=CARTESIAN_POINT('Ctrl Pts',(-8.2787512356018,-1.16744491727759,19.0802057614874));
#15205=CARTESIAN_POINT('Ctrl Pts',(-8.57224006554514,-1.22306556372407,
19.0682025746981));
#15206=CARTESIAN_POINT('Ctrl Pts',(-8.88610136060001,-1.16276985667004,
19.0561993879088));
#15207=CARTESIAN_POINT('Ctrl Pts',(-9.13808834820145,-1.00235817476317,
19.0441962011195));
#15208=CARTESIAN_POINT('Ctrl Pts',(-9.39007533580289,-0.841946492856298,
19.0321930143302));
#15209=CARTESIAN_POINT('Ctrl Pts',(-9.57754329642164,-0.583102430602389,
19.0201898275408));
#15210=CARTESIAN_POINT('Ctrl Pts',(-9.65136659729205,-0.293655596345669,
19.0081866407515));
#15211=CARTESIAN_POINT('Ctrl Pts',(-9.67581103310554,-0.197813707971877,
19.0042121350661));
#15212=CARTESIAN_POINT('Ctrl Pts',(-9.68822500000007,-0.0989100500916788,
19.0002376293806));
#15213=CARTESIAN_POINT('Ctrl Pts',(-9.688225,7.87592213669086E-13,18.9962631236951));
#15214=CARTESIAN_POINT('Ctrl Pts',(-9.688225,-8.62088178621434E-13,18.9537368763049));
#15215=CARTESIAN_POINT('Ctrl Pts',(-9.68822499999978,-0.298712821306989,
18.9657400630942));
#15216=CARTESIAN_POINT('Ctrl Pts',(-9.5705424563254,-0.595858078272372,
18.9777432498835));
#15217=CARTESIAN_POINT('Ctrl Pts',(-9.36601586214869,-0.813569405233421,
18.9897464366728));
#15218=CARTESIAN_POINT('Ctrl Pts',(-9.16148926797198,-1.03128073219447,
19.0017496234621));
#15219=CARTESIAN_POINT('Ctrl Pts',(-8.87226522412745,-1.16727314847169,
19.0137528102515));
#15220=CARTESIAN_POINT('Ctrl Pts',(-8.57413435701344,-1.18591009260197,
19.0257559970408));
#15221=CARTESIAN_POINT('Ctrl Pts',(-8.27600348989943,-1.20454703673225,
19.0377591838301));
#15222=CARTESIAN_POINT('Ctrl Pts',(-7.9720948203199,-1.10563290540061,19.0497623706194));
#15223=CARTESIAN_POINT('Ctrl Pts',(-7.74204705371973,-0.915087963995846,
19.0617655574087));
#15224=CARTESIAN_POINT('Ctrl Pts',(-7.51199928711957,-0.724543022591087,
19.0737687441981));
#15225=CARTESIAN_POINT('Ctrl Pts',(-7.35822688079588,-0.444367128060312,
19.0857719309874));
#15226=CARTESIAN_POINT('Ctrl Pts',(-7.32102560975802,-0.147979855989069,
19.0977751177767));
#15227=CARTESIAN_POINT('Ctrl Pts',(-7.28382433872015,0.148407416082175,
19.109778304566));
#15228=CARTESIAN_POINT('Ctrl Pts',(-7.36358464744686,0.457895344723207,
19.1217814913553));
#15229=CARTESIAN_POINT('Ctrl Pts',(-7.53940549437961,0.699383189958775,
19.1337846781447));
#15230=CARTESIAN_POINT('Ctrl Pts',(-7.71522634131235,0.940871035194342,
19.145787864934));
#15231=CARTESIAN_POINT('Ctrl Pts',(-7.98526240565915,1.11182427083144,19.1577910517233));
#15232=CARTESIAN_POINT('Ctrl Pts',(-8.27875123560257,1.16744491727773,19.1697942385126));
#15233=CARTESIAN_POINT('Ctrl Pts',(-8.572240065546,1.22306556372403,19.1817974253019));
#15234=CARTESIAN_POINT('Ctrl Pts',(-8.88610136060088,1.16276985666976,19.1938006120913));
#15235=CARTESIAN_POINT('Ctrl Pts',(-9.13808834820223,1.00235817476267,19.2058037988806));
#15236=CARTESIAN_POINT('Ctrl Pts',(-9.39007533580358,0.841946492855579,
19.2178069856699));
#15237=CARTESIAN_POINT('Ctrl Pts',(-9.57754329642215,0.58310243060147,19.2298101724592));
#15238=CARTESIAN_POINT('Ctrl Pts',(-9.65136659729231,0.29365559634464,19.2418133592485));
#15239=CARTESIAN_POINT('Ctrl Pts',(-9.67581103310564,0.197813707971131,
19.245787864934));
#15240=CARTESIAN_POINT('Ctrl Pts',(-9.68822500000007,0.0989100500912471,
19.2497623706194));
#15241=CARTESIAN_POINT('Ctrl Pts',(-9.688225,-9.03999097801034E-13,19.2537368763049));
#15242=CARTESIAN_POINT('Origin',(-8.5,0.,1.8));
#15243=CARTESIAN_POINT('',(-9.68921750296084,-0.000102469561994563,19.5962631236951));
#15244=CARTESIAN_POINT('',(-9.688225,-8.78408457083424E-13,19.5537368763049));
#15245=CARTESIAN_POINT('',(-9.688225,-1.45515594291686E-16,1.8));
#15246=CARTESIAN_POINT('Ctrl Pts',(-9.69028507049178,-0.000212689062328297,
19.5962631236951));
#15247=CARTESIAN_POINT('Ctrl Pts',(-9.68998036389171,0.391158548490939,
19.5804677035918));
#15248=CARTESIAN_POINT('Ctrl Pts',(-9.4779526199623,0.783211439565971,19.5646722834885));
#15249=CARTESIAN_POINT('Ctrl Pts',(-9.15044819587364,0.996873139970471,
19.5488768633852));
#15250=CARTESIAN_POINT('Ctrl Pts',(-8.82062318529691,1.21204877551144,19.5329695222336));
#15251=CARTESIAN_POINT('Ctrl Pts',(-8.37367923882642,1.24629622368731,19.5170621810819));
#15252=CARTESIAN_POINT('Ctrl Pts',(-8.01348680256335,1.08572482393094,19.5011548399303));
#15253=CARTESIAN_POINT('Ctrl Pts',(-7.83339058443181,1.00543912405275,19.4932011693545));
#15254=CARTESIAN_POINT('Ctrl Pts',(-7.67498224385212,0.87644871219149,19.4852474987787));
#15255=CARTESIAN_POINT('Ctrl Pts',(-7.55483788786785,0.718375552796157,
19.4772938282029));
#15256=CARTESIAN_POINT('Ctrl Pts',(-7.43469353188358,0.560302393400842,
19.4693401576271));
#15257=CARTESIAN_POINT('Ctrl Pts',(-7.35281316049472,0.373146486471458,
19.4613864870513));
#15258=CARTESIAN_POINT('Ctrl Pts',(-7.32366558028848,0.178131461516125,
19.4534328164754));
#15259=CARTESIAN_POINT('Ctrl Pts',(-7.26537041987601,-0.211898588394563,
19.4375254753238));
#15260=CARTESIAN_POINT('Ctrl Pts',(-7.41800642419409,-0.633365110409051,
19.4216181341722));
#15261=CARTESIAN_POINT('Ctrl Pts',(-7.71361762553116,-0.893555635556405,
19.4057107930206));
#15262=CARTESIAN_POINT('Ctrl Pts',(-8.00922882686823,-1.15374616070376,
19.389803451869));
#15263=CARTESIAN_POINT('Ctrl Pts',(-8.44781522522429,-1.25266068898398,
19.3738961107173));
#15264=CARTESIAN_POINT('Ctrl Pts',(-8.8268302328739,-1.14454041604515,19.3579887695657));
#15265=CARTESIAN_POINT('Ctrl Pts',(-9.20584524052351,-1.03642014310631,
19.3420814284141));
#15266=CARTESIAN_POINT('Ctrl Pts',(-9.52528885746666,-0.721265068948423,
19.3261740872625));
#15267=CARTESIAN_POINT('Ctrl Pts',(-9.6392103838706,-0.344042203087319,
19.3102667461109));
#15268=CARTESIAN_POINT('Ctrl Pts',(-9.6726396881056,-0.233349357359851,
19.3055988719723));
#15269=CARTESIAN_POINT('Ctrl Pts',(-9.6883719131767,-0.117311983360903,
19.3009309978337));
#15270=CARTESIAN_POINT('Ctrl Pts',(-9.68745089909105,-0.00102202174496036,
19.2962631236951));
#15271=CARTESIAN_POINT('Ctrl Pts',(-9.688225,-9.03999097801034E-13,19.2537368763049));
#15272=CARTESIAN_POINT('Ctrl Pts',(-9.68822499999977,-0.298712821307009,
19.2657400630942));
#15273=CARTESIAN_POINT('Ctrl Pts',(-9.5705424563254,-0.595858078272365,
19.2777432498835));
#15274=CARTESIAN_POINT('Ctrl Pts',(-9.36601586214871,-0.813569405233403,
19.2897464366728));
#15275=CARTESIAN_POINT('Ctrl Pts',(-9.16148926797202,-1.03128073219444,
19.3017496234622));
#15276=CARTESIAN_POINT('Ctrl Pts',(-8.87226522412752,-1.16727314847166,
19.3137528102515));
#15277=CARTESIAN_POINT('Ctrl Pts',(-8.57413435701353,-1.18591009260196,
19.3257559970408));
#15278=CARTESIAN_POINT('Ctrl Pts',(-8.27600348989955,-1.20454703673226,
19.3377591838301));
#15279=CARTESIAN_POINT('Ctrl Pts',(-7.97209482032003,-1.10563290540066,
19.3497623706194));
#15280=CARTESIAN_POINT('Ctrl Pts',(-7.74204705371986,-0.915087963995949,
19.3617655574087));
#15281=CARTESIAN_POINT('Ctrl Pts',(-7.51199928711968,-0.724543022591235,
19.3737687441981));
#15282=CARTESIAN_POINT('Ctrl Pts',(-7.35822688079597,-0.444367128060509,
19.3857719309874));
#15283=CARTESIAN_POINT('Ctrl Pts',(-7.32102560975805,-0.147979855989295,
19.3977751177767));
#15284=CARTESIAN_POINT('Ctrl Pts',(-7.28382433872012,0.148407416081919,
19.409778304566));
#15285=CARTESIAN_POINT('Ctrl Pts',(-7.36358464744676,0.457895344722943,
19.4217814913553));
#15286=CARTESIAN_POINT('Ctrl Pts',(-7.53940549437943,0.699383189958536,
19.4337846781447));
#15287=CARTESIAN_POINT('Ctrl Pts',(-7.71522634131211,0.940871035194129,
19.445787864934));
#15288=CARTESIAN_POINT('Ctrl Pts',(-7.98526240565883,1.11182427083128,19.4577910517233));
#15289=CARTESIAN_POINT('Ctrl Pts',(-8.27875123560222,1.16744491727767,19.4697942385126));
#15290=CARTESIAN_POINT('Ctrl Pts',(-8.57224006554561,1.22306556372405,19.4817974253019));
#15291=CARTESIAN_POINT('Ctrl Pts',(-8.88610136060047,1.16276985666989,19.4938006120912));
#15292=CARTESIAN_POINT('Ctrl Pts',(-9.13808834820187,1.0023581747629,19.5058037988806));
#15293=CARTESIAN_POINT('Ctrl Pts',(-9.39007533580326,0.841946492855913,
19.5178069856699));
#15294=CARTESIAN_POINT('Ctrl Pts',(-9.57754329642192,0.5831024306019,19.5298101724592));
#15295=CARTESIAN_POINT('Ctrl Pts',(-9.65136659729219,0.293655596345123,
19.5418133592485));
#15296=CARTESIAN_POINT('Ctrl Pts',(-9.67581103310559,0.197813707971494,
19.545787864934));
#15297=CARTESIAN_POINT('Ctrl Pts',(-9.68822500000007,0.0989100500914754,
19.5497623706194));
#15298=CARTESIAN_POINT('Ctrl Pts',(-9.688225,-8.10851386034983E-13,19.5537368763049));
#15299=CARTESIAN_POINT('Origin',(-8.5,0.,1.8));
#15300=CARTESIAN_POINT('',(-9.688225,8.64530669275609E-13,19.8962631236951));
#15301=CARTESIAN_POINT('',(-9.688225,-8.52762305214583E-13,19.8537368763049));
#15302=CARTESIAN_POINT('',(-9.688225,-1.45515594291686E-16,1.8));
#15303=CARTESIAN_POINT('Ctrl Pts',(-9.688225,7.96918087075937E-13,19.8962631236951));
#15304=CARTESIAN_POINT('Ctrl Pts',(-9.6882249999998,0.298712821306902,19.8842599369058));
#15305=CARTESIAN_POINT('Ctrl Pts',(-9.57054245632545,0.595858078272269,
19.8722567501165));
#15306=CARTESIAN_POINT('Ctrl Pts',(-9.36601586214878,0.813569405233325,
19.8602535633272));
#15307=CARTESIAN_POINT('Ctrl Pts',(-9.16148926797211,1.03128073219438,19.8482503765379));
#15308=CARTESIAN_POINT('Ctrl Pts',(-8.87226522412763,1.16727314847163,19.8362471897486));
#15309=CARTESIAN_POINT('Ctrl Pts',(-8.57413435701364,1.18591009260195,19.8242440029592));
#15310=CARTESIAN_POINT('Ctrl Pts',(-8.27600348989966,1.20454703673228,19.8122408161699));
#15311=CARTESIAN_POINT('Ctrl Pts',(-7.97209482032013,1.10563290540071,19.8002376293806));
#15312=CARTESIAN_POINT('Ctrl Pts',(-7.74204705371994,0.915087963996017,
19.7882344425913));
#15313=CARTESIAN_POINT('Ctrl Pts',(-7.51199928711975,0.724543022591324,
19.776231255802));
#15314=CARTESIAN_POINT('Ctrl Pts',(-7.35822688079601,0.444367128060612,
19.7642280690126));
#15315=CARTESIAN_POINT('Ctrl Pts',(-7.32102560975806,0.147979855989401,
19.7522248822233));
#15316=CARTESIAN_POINT('Ctrl Pts',(-7.28382433872011,-0.14840741608181,
19.740221695434));
#15317=CARTESIAN_POINT('Ctrl Pts',(-7.36358464744672,-0.45789534472284,
19.7282185086447));
#15318=CARTESIAN_POINT('Ctrl Pts',(-7.53940549437937,-0.699383189958449,
19.7162153218554));
#15319=CARTESIAN_POINT('Ctrl Pts',(-7.71522634131202,-0.940871035194058,
19.7042121350661));
#15320=CARTESIAN_POINT('Ctrl Pts',(-7.98526240565873,-1.11182427083124,
19.6922089482767));
#15321=CARTESIAN_POINT('Ctrl Pts',(-8.27875123560211,-1.16744491727765,
19.6802057614874));
#15322=CARTESIAN_POINT('Ctrl Pts',(-8.5722400655455,-1.22306556372405,19.6682025746981));
#15323=CARTESIAN_POINT('Ctrl Pts',(-8.88610136060037,-1.16276985666993,
19.6561993879088));
#15324=CARTESIAN_POINT('Ctrl Pts',(-9.13808834820177,-1.00235817476296,
19.6441962011195));
#15325=CARTESIAN_POINT('Ctrl Pts',(-9.39007533580318,-0.841946492855994,
19.6321930143301));
#15326=CARTESIAN_POINT('Ctrl Pts',(-9.57754329642186,-0.583102430601997,
19.6201898275408));
#15327=CARTESIAN_POINT('Ctrl Pts',(-9.65136659729216,-0.293655596345227,
19.6081866407515));
#15328=CARTESIAN_POINT('Ctrl Pts',(-9.67581103310559,-0.197813707971534,
19.6042121350661));
#15329=CARTESIAN_POINT('Ctrl Pts',(-9.68822500000008,-0.0989100500914475,
19.6002376293806));
#15330=CARTESIAN_POINT('Ctrl Pts',(-9.688225,9.06386077303978E-13,19.5962631236951));
#15331=CARTESIAN_POINT('Ctrl Pts',(-9.688225,-8.10851386034983E-13,19.5537368763049));
#15332=CARTESIAN_POINT('Ctrl Pts',(-9.68822499999979,-0.298712821306893,
19.5657400630942));
#15333=CARTESIAN_POINT('Ctrl Pts',(-9.57054245632546,-0.595858078272237,
19.5777432498835));
#15334=CARTESIAN_POINT('Ctrl Pts',(-9.36601586214882,-0.813569405233286,
19.5897464366728));
#15335=CARTESIAN_POINT('Ctrl Pts',(-9.16148926797217,-1.03128073219433,
19.6017496234621));
#15336=CARTESIAN_POINT('Ctrl Pts',(-8.87226522412772,-1.16727314847159,
19.6137528102515));
#15337=CARTESIAN_POINT('Ctrl Pts',(-8.57413435701376,-1.18591009260195,
19.6257559970408));
#15338=CARTESIAN_POINT('Ctrl Pts',(-8.2760034898998,-1.2045470367323,19.6377591838301));
#15339=CARTESIAN_POINT('Ctrl Pts',(-7.97209482032029,-1.10563290540078,
19.6497623706194));
#15340=CARTESIAN_POINT('Ctrl Pts',(-7.74204705372008,-0.915087963996137,
19.6617655574087));
#15341=CARTESIAN_POINT('Ctrl Pts',(-7.51199928711988,-0.724543022591495,
19.673768744198));
#15342=CARTESIAN_POINT('Ctrl Pts',(-7.3582268807961,-0.444367128060836,
19.6857719309874));
#15343=CARTESIAN_POINT('Ctrl Pts',(-7.32102560975809,-0.147979855989656,
19.6977751177767));
#15344=CARTESIAN_POINT('Ctrl Pts',(-7.28382433872008,0.148407416081525,
19.709778304566));
#15345=CARTESIAN_POINT('Ctrl Pts',(-7.36358464744661,0.457895344722549,
19.7217814913553));
#15346=CARTESIAN_POINT('Ctrl Pts',(-7.53940549437918,0.699383189958187,
19.7337846781446));
#15347=CARTESIAN_POINT('Ctrl Pts',(-7.71522634131175,0.940871035193826,
19.745787864934));
#15348=CARTESIAN_POINT('Ctrl Pts',(-7.98526240565838,1.11182427083107,19.7577910517233));
#15349=CARTESIAN_POINT('Ctrl Pts',(-8.27875123560173,1.16744491727757,19.7697942385126));
#15350=CARTESIAN_POINT('Ctrl Pts',(-8.57224006554507,1.22306556372407,19.7817974253019));
#15351=CARTESIAN_POINT('Ctrl Pts',(-8.88610136059994,1.16276985667006,19.7938006120912));
#15352=CARTESIAN_POINT('Ctrl Pts',(-9.13808834820139,1.00235817476321,19.8058037988805));
#15353=CARTESIAN_POINT('Ctrl Pts',(-9.39007533580284,0.84194649285635,19.8178069856699));
#15354=CARTESIAN_POINT('Ctrl Pts',(-9.57754329642161,0.583102430602453,
19.8298101724592));
#15355=CARTESIAN_POINT('Ctrl Pts',(-9.65136659729203,0.293655596345737,
19.8418133592485));
#15356=CARTESIAN_POINT('Ctrl Pts',(-9.67581103310554,0.197813707971903,
19.845787864934));
#15357=CARTESIAN_POINT('Ctrl Pts',(-9.68822500000007,0.0989100500916587,
19.8497623706194));
#15358=CARTESIAN_POINT('Ctrl Pts',(-9.688225,-8.52762305214583E-13,19.8537368763049));
#15359=CARTESIAN_POINT('Origin',(-8.5,0.,1.8));
#15360=CARTESIAN_POINT('',(-9.688225,8.90176821144451E-13,20.1962631236951));
#15361=CARTESIAN_POINT('',(-9.688225,-8.27171664496973E-13,20.1537368763049));
#15362=CARTESIAN_POINT('',(-9.688225,-1.45515594291686E-16,1.8));
#15363=CARTESIAN_POINT('Ctrl Pts',(-9.688225,9.5767838104166E-13,20.1962631236951));
#15364=CARTESIAN_POINT('Ctrl Pts',(-9.68822499999976,0.29871282130704,20.1842599369058));
#15365=CARTESIAN_POINT('Ctrl Pts',(-9.57054245632539,0.595858078272369,
20.1722567501165));
#15366=CARTESIAN_POINT('Ctrl Pts',(-9.36601586214872,0.813569405233393,
20.1602535633272));
#15367=CARTESIAN_POINT('Ctrl Pts',(-9.16148926797204,1.03128073219442,20.1482503765379));
#15368=CARTESIAN_POINT('Ctrl Pts',(-8.87226522412758,1.16727314847164,20.1362471897486));
#15369=CARTESIAN_POINT('Ctrl Pts',(-8.57413435701362,1.18591009260196,20.1242440029592));
#15370=CARTESIAN_POINT('Ctrl Pts',(-8.27600348989965,1.20454703673228,20.1122408161699));
#15371=CARTESIAN_POINT('Ctrl Pts',(-7.97209482032015,1.10563290540071,20.1002376293806));
#15372=CARTESIAN_POINT('Ctrl Pts',(-7.74204705371997,0.915087963996044,
20.0882344425913));
#15373=CARTESIAN_POINT('Ctrl Pts',(-7.51199928711979,0.724543022591373,
20.076231255802));
#15374=CARTESIAN_POINT('Ctrl Pts',(-7.35822688079604,0.444367128060695,
20.0642280690126));
#15375=CARTESIAN_POINT('Ctrl Pts',(-7.32102560975807,0.14797985598951,20.0522248822233));
#15376=CARTESIAN_POINT('Ctrl Pts',(-7.2838243387201,-0.148407416081675,
20.040221695434));
#15377=CARTESIAN_POINT('Ctrl Pts',(-7.36358464744666,-0.457895344722689,
20.0282185086447));
#15378=CARTESIAN_POINT('Ctrl Pts',(-7.53940549437926,-0.699383189958306,
20.0162153218554));
#15379=CARTESIAN_POINT('Ctrl Pts',(-7.71522634131187,-0.940871035193923,
20.0042121350661));
#15380=CARTESIAN_POINT('Ctrl Pts',(-7.98526240565852,-1.11182427083114,
19.9922089482767));
#15381=CARTESIAN_POINT('Ctrl Pts',(-8.27875123560187,-1.1674449172776,19.9802057614874));
#15382=CARTESIAN_POINT('Ctrl Pts',(-8.57224006554522,-1.22306556372406,
19.9682025746981));
#15383=CARTESIAN_POINT('Ctrl Pts',(-8.88610136060008,-1.16276985667001,
19.9561993879088));
#15384=CARTESIAN_POINT('Ctrl Pts',(-9.13808834820151,-1.00235817476313,
19.9441962011195));
#15385=CARTESIAN_POINT('Ctrl Pts',(-9.39007533580294,-0.84194649285624,
19.9321930143302));
#15386=CARTESIAN_POINT('Ctrl Pts',(-9.57754329642168,-0.58310243060232,
19.9201898275408));
#15387=CARTESIAN_POINT('Ctrl Pts',(-9.65136659729207,-0.293655596345595,
19.9081866407515));
#15388=CARTESIAN_POINT('Ctrl Pts',(-9.67581103310554,-0.197813707971823,
19.9042121350661));
#15389=CARTESIAN_POINT('Ctrl Pts',(-9.68822500000007,-0.098910050091647,
19.9002376293806));
#15390=CARTESIAN_POINT('Ctrl Pts',(-9.688225,7.96918087075937E-13,19.8962631236951));
#15391=CARTESIAN_POINT('Ctrl Pts',(-9.688225,-8.52762305214583E-13,19.8537368763049));
#15392=CARTESIAN_POINT('Ctrl Pts',(-9.68822499999978,-0.298712821306935,
19.8657400630942));
#15393=CARTESIAN_POINT('Ctrl Pts',(-9.57054245632544,-0.595858078272275,
19.8777432498835));
#15394=CARTESIAN_POINT('Ctrl Pts',(-9.36601586214879,-0.813569405233316,
19.8897464366728));
#15395=CARTESIAN_POINT('Ctrl Pts',(-9.16148926797213,-1.03128073219436,
19.9017496234621));
#15396=CARTESIAN_POINT('Ctrl Pts',(-8.87226522412768,-1.1672731484716,19.9137528102515));
#15397=CARTESIAN_POINT('Ctrl Pts',(-8.57413435701372,-1.18591009260195,
19.9257559970408));
#15398=CARTESIAN_POINT('Ctrl Pts',(-8.27600348989976,-1.20454703673229,
19.9377591838301));
#15399=CARTESIAN_POINT('Ctrl Pts',(-7.97209482032025,-1.10563290540076,
19.9497623706194));
#15400=CARTESIAN_POINT('Ctrl Pts',(-7.74204705372005,-0.915087963996111,
19.9617655574087));
#15401=CARTESIAN_POINT('Ctrl Pts',(-7.51199928711986,-0.72454302259146,
19.9737687441981));
#15402=CARTESIAN_POINT('Ctrl Pts',(-7.35822688079608,-0.444367128060796,
19.9857719309874));
#15403=CARTESIAN_POINT('Ctrl Pts',(-7.32102560975809,-0.147979855989614,
19.9977751177767));
#15404=CARTESIAN_POINT('Ctrl Pts',(-7.28382433872009,0.148407416081568,
20.009778304566));
#15405=CARTESIAN_POINT('Ctrl Pts',(-7.36358464744662,0.457895344722589,
20.0217814913553));
#15406=CARTESIAN_POINT('Ctrl Pts',(-7.5394054943792,0.699383189958221,20.0337846781446));
#15407=CARTESIAN_POINT('Ctrl Pts',(-7.71522634131179,0.940871035193854,
20.045787864934));
#15408=CARTESIAN_POINT('Ctrl Pts',(-7.98526240565842,1.11182427083109,20.0577910517233));
#15409=CARTESIAN_POINT('Ctrl Pts',(-8.27875123560177,1.16744491727758,20.0697942385126));
#15410=CARTESIAN_POINT('Ctrl Pts',(-8.57224006554511,1.22306556372407,20.0817974253019));
#15411=CARTESIAN_POINT('Ctrl Pts',(-8.88610136059998,1.16276985667005,20.0938006120912));
#15412=CARTESIAN_POINT('Ctrl Pts',(-9.13808834820142,1.00235817476318,20.1058037988805));
#15413=CARTESIAN_POINT('Ctrl Pts',(-9.39007533580287,0.841946492856318,
20.1178069856699));
#15414=CARTESIAN_POINT('Ctrl Pts',(-9.57754329642163,0.583102430602415,
20.1298101724592));
#15415=CARTESIAN_POINT('Ctrl Pts',(-9.65136659729204,0.293655596345696,
20.1418133592485));
#15416=CARTESIAN_POINT('Ctrl Pts',(-9.67581103310554,0.197813707971883,
20.145787864934));
#15417=CARTESIAN_POINT('Ctrl Pts',(-9.68822500000007,0.0989100500916617,
20.1497623706194));
#15418=CARTESIAN_POINT('Ctrl Pts',(-9.688225,-8.27171664496973E-13,20.1537368763049));
#15419=CARTESIAN_POINT('Origin',(-8.5,0.,1.8));
#15420=CARTESIAN_POINT('',(-9.688225,9.15711950710829E-13,20.4962631236951));
#15421=CARTESIAN_POINT('',(-9.688225,-8.01581023779363E-13,20.4537368763049));
#15422=CARTESIAN_POINT('',(-9.688225,-1.45515594291686E-16,1.8));
#15423=CARTESIAN_POINT('Ctrl Pts',(-9.688225,9.15711950710829E-13,20.4962631236951));
#15424=CARTESIAN_POINT('Ctrl Pts',(-9.68822499999977,0.298712821306998,
20.4842599369058));
#15425=CARTESIAN_POINT('Ctrl Pts',(-9.57054245632541,0.595858078272332,
20.4722567501165));
#15426=CARTESIAN_POINT('Ctrl Pts',(-9.36601586214874,0.813569405233362,
20.4602535633272));
#15427=CARTESIAN_POINT('Ctrl Pts',(-9.16148926797208,1.03128073219439,20.4482503765379));
#15428=CARTESIAN_POINT('Ctrl Pts',(-8.87226522412762,1.16727314847162,20.4362471897486));
#15429=CARTESIAN_POINT('Ctrl Pts',(-8.57413435701366,1.18591009260195,20.4242440029592));
#15430=CARTESIAN_POINT('Ctrl Pts',(-8.2760034898997,1.20454703673228,20.4122408161699));
#15431=CARTESIAN_POINT('Ctrl Pts',(-7.97209482032019,1.10563290540073,20.4002376293806));
#15432=CARTESIAN_POINT('Ctrl Pts',(-7.74204705372,0.915087963996071,20.3882344425913));
#15433=CARTESIAN_POINT('Ctrl Pts',(-7.51199928711982,0.724543022591408,
20.376231255802));
#15434=CARTESIAN_POINT('Ctrl Pts',(-7.35822688079606,0.444367128060736,
20.3642280690127));
#15435=CARTESIAN_POINT('Ctrl Pts',(-7.32102560975808,0.147979855989552,
20.3522248822233));
#15436=CARTESIAN_POINT('Ctrl Pts',(-7.28382433872009,-0.148407416081632,
20.340221695434));
#15437=CARTESIAN_POINT('Ctrl Pts',(-7.36358464744665,-0.457895344722649,
20.3282185086447));
#15438=CARTESIAN_POINT('Ctrl Pts',(-7.53940549437924,-0.699383189958272,
20.3162153218554));
#15439=CARTESIAN_POINT('Ctrl Pts',(-7.71522634131184,-0.940871035193895,
20.3042121350661));
#15440=CARTESIAN_POINT('Ctrl Pts',(-7.98526240565848,-1.11182427083112,
20.2922089482767));
#15441=CARTESIAN_POINT('Ctrl Pts',(-8.27875123560183,-1.16744491727759,
20.2802057614874));
#15442=CARTESIAN_POINT('Ctrl Pts',(-8.57224006554518,-1.22306556372407,
20.2682025746981));
#15443=CARTESIAN_POINT('Ctrl Pts',(-8.88610136060004,-1.16276985667003,
20.2561993879088));
#15444=CARTESIAN_POINT('Ctrl Pts',(-9.13808834820148,-1.00235817476315,
20.2441962011195));
#15445=CARTESIAN_POINT('Ctrl Pts',(-9.39007533580291,-0.841946492856271,
20.2321930143302));
#15446=CARTESIAN_POINT('Ctrl Pts',(-9.57754329642166,-0.583102430602358,
20.2201898275408));
#15447=CARTESIAN_POINT('Ctrl Pts',(-9.65136659729206,-0.293655596345635,
20.2081866407515));
#15448=CARTESIAN_POINT('Ctrl Pts',(-9.67581103310556,-0.197813707971799,
20.2042121350661));
#15449=CARTESIAN_POINT('Ctrl Pts',(-9.68822500000008,-0.0989100500915538,
20.2002376293806));
#15450=CARTESIAN_POINT('Ctrl Pts',(-9.688225,9.5767838104166E-13,20.1962631236951));
#15451=CARTESIAN_POINT('Ctrl Pts',(-9.688225,-8.27171664496973E-13,20.1537368763049));
#15452=CARTESIAN_POINT('Ctrl Pts',(-9.68822499999979,-0.298712821306932,
20.1657400630942));
#15453=CARTESIAN_POINT('Ctrl Pts',(-9.57054245632544,-0.595858078272296,
20.1777432498835));
#15454=CARTESIAN_POINT('Ctrl Pts',(-9.36601586214876,-0.813569405233347,
20.1897464366728));
#15455=CARTESIAN_POINT('Ctrl Pts',(-9.16148926797208,-1.0312807321944,20.2017496234621));
#15456=CARTESIAN_POINT('Ctrl Pts',(-8.8722652241276,-1.16727314847164,20.2137528102515));
#15457=CARTESIAN_POINT('Ctrl Pts',(-8.57413435701361,-1.18591009260196,
20.2257559970408));
#15458=CARTESIAN_POINT('Ctrl Pts',(-8.27600348989963,-1.20454703673228,
20.2377591838301));
#15459=CARTESIAN_POINT('Ctrl Pts',(-7.9720948203201,-1.1056329054007,20.2497623706194));
#15460=CARTESIAN_POINT('Ctrl Pts',(-7.74204705371992,-0.915087963995998,
20.2617655574087));
#15461=CARTESIAN_POINT('Ctrl Pts',(-7.51199928711973,-0.724543022591299,
20.2737687441981));
#15462=CARTESIAN_POINT('Ctrl Pts',(-7.358226880796,-0.444367128060583,20.2857719309874));
#15463=CARTESIAN_POINT('Ctrl Pts',(-7.32102560975806,-0.147979855989371,
20.2977751177767));
#15464=CARTESIAN_POINT('Ctrl Pts',(-7.28382433872012,0.14840741608184,20.309778304566));
#15465=CARTESIAN_POINT('Ctrl Pts',(-7.36358464744673,0.457895344722869,
20.3217814913553));
#15466=CARTESIAN_POINT('Ctrl Pts',(-7.53940549437939,0.699383189958473,
20.3337846781446));
#15467=CARTESIAN_POINT('Ctrl Pts',(-7.71522634131205,0.940871035194078,
20.345787864934));
#15468=CARTESIAN_POINT('Ctrl Pts',(-7.98526240565876,1.11182427083125,20.3577910517233));
#15469=CARTESIAN_POINT('Ctrl Pts',(-8.27875123560214,1.16744491727765,20.3697942385126));
#15470=CARTESIAN_POINT('Ctrl Pts',(-8.57224006554553,1.22306556372405,20.3817974253019));
#15471=CARTESIAN_POINT('Ctrl Pts',(-8.8861013606004,1.16276985666991,20.3938006120912));
#15472=CARTESIAN_POINT('Ctrl Pts',(-9.1380883482018,1.00235817476294,20.4058037988806));
#15473=CARTESIAN_POINT('Ctrl Pts',(-9.3900753358032,0.841946492855971,20.4178069856699));
#15474=CARTESIAN_POINT('Ctrl Pts',(-9.57754329642188,0.58310243060197,20.4298101724592));
#15475=CARTESIAN_POINT('Ctrl Pts',(-9.65136659729217,0.293655596345198,
20.4418133592485));
#15476=CARTESIAN_POINT('Ctrl Pts',(-9.67581103310558,0.197813707971548,
20.445787864934));
#15477=CARTESIAN_POINT('Ctrl Pts',(-9.68822500000007,0.0989100500915072,
20.4497623706194));
#15478=CARTESIAN_POINT('Ctrl Pts',(-9.688225,-8.01581023779363E-13,20.4537368763049));
#15479=CARTESIAN_POINT('Origin',(-8.5,0.,1.8));
#15480=CARTESIAN_POINT('',(-9.688225,9.41247080277208E-13,20.7962631236951));
#15481=CARTESIAN_POINT('',(-9.68836223994391,0.000210585078932092,20.7537368763049));
#15482=CARTESIAN_POINT('',(-9.688225,-1.45515594291686E-16,1.8));
#15483=CARTESIAN_POINT('Ctrl Pts',(-9.688225,1.00885966247688E-12,20.7962631236951));
#15484=CARTESIAN_POINT('Ctrl Pts',(-9.68822499999975,0.298712821307114,
20.7842599369058));
#15485=CARTESIAN_POINT('Ctrl Pts',(-9.57054245632535,0.59585807827246,20.7722567501165));
#15486=CARTESIAN_POINT('Ctrl Pts',(-9.36601586214863,0.813569405233479,
20.7602535633272));
#15487=CARTESIAN_POINT('Ctrl Pts',(-9.16148926797192,1.0312807321945,20.7482503765379));
#15488=CARTESIAN_POINT('Ctrl Pts',(-8.87226522412742,1.16727314847169,20.7362471897485));
#15489=CARTESIAN_POINT('Ctrl Pts',(-8.57413435701343,1.18591009260197,20.7242440029592));
#15490=CARTESIAN_POINT('Ctrl Pts',(-8.27600348989944,1.20454703673224,20.7122408161699));
#15491=CARTESIAN_POINT('Ctrl Pts',(-7.97209482031993,1.10563290540062,20.7002376293806));
#15492=CARTESIAN_POINT('Ctrl Pts',(-7.74204705371978,0.915087963995882,
20.6882344425913));
#15493=CARTESIAN_POINT('Ctrl Pts',(-7.51199928711962,0.724543022591148,
20.676231255802));
#15494=CARTESIAN_POINT('Ctrl Pts',(-7.35822688079593,0.444367128060409,
20.6642280690126));
#15495=CARTESIAN_POINT('Ctrl Pts',(-7.32102560975803,0.147979855989191,
20.6522248822233));
#15496=CARTESIAN_POINT('Ctrl Pts',(-7.28382433872014,-0.148407416082027,
20.640221695434));
#15497=CARTESIAN_POINT('Ctrl Pts',(-7.3635846474468,-0.457895344723043,
20.6282185086447));
#15498=CARTESIAN_POINT('Ctrl Pts',(-7.53940549437949,-0.699383189958621,
20.6162153218554));
#15499=CARTESIAN_POINT('Ctrl Pts',(-7.71522634131219,-0.940871035194198,
20.604212135066));
#15500=CARTESIAN_POINT('Ctrl Pts',(-7.98526240565893,-1.11182427083133,
20.5922089482767));
#15501=CARTESIAN_POINT('Ctrl Pts',(-8.27875123560232,-1.16744491727769,
20.5802057614874));
#15502=CARTESIAN_POINT('Ctrl Pts',(-8.57224006554571,-1.22306556372404,
20.5682025746981));
#15503=CARTESIAN_POINT('Ctrl Pts',(-8.88610136060058,-1.16276985666986,
20.5561993879088));
#15504=CARTESIAN_POINT('Ctrl Pts',(-9.13808834820195,-1.00235817476285,
20.5441962011195));
#15505=CARTESIAN_POINT('Ctrl Pts',(-9.39007533580333,-0.841946492855835,
20.5321930143301));
#15506=CARTESIAN_POINT('Ctrl Pts',(-9.57754329642197,-0.583102430601805,
20.5201898275408));
#15507=CARTESIAN_POINT('Ctrl Pts',(-9.65136659729221,-0.293655596345021,
20.5081866407515));
#15508=CARTESIAN_POINT('Ctrl Pts',(-9.6758110331056,-0.19781370797139,20.504212135066));
#15509=CARTESIAN_POINT('Ctrl Pts',(-9.68822500000008,-0.0989100500913706,
20.5002376293806));
#15510=CARTESIAN_POINT('Ctrl Pts',(-9.688225,9.15711950710829E-13,20.4962631236951));
#15511=CARTESIAN_POINT('Ctrl Pts',(-9.688225,-8.01581023779363E-13,20.4537368763049));
#15512=CARTESIAN_POINT('Ctrl Pts',(-9.6882249999998,-0.298712821306884,
20.4657400630942));
#15513=CARTESIAN_POINT('Ctrl Pts',(-9.57054245632547,-0.595858078272229,
20.4777432498835));
#15514=CARTESIAN_POINT('Ctrl Pts',(-9.36601586214882,-0.813569405233279,
20.4897464366728));
#15515=CARTESIAN_POINT('Ctrl Pts',(-9.16148926797218,-1.03128073219433,
20.5017496234621));
#15516=CARTESIAN_POINT('Ctrl Pts',(-8.87226522412773,-1.16727314847159,
20.5137528102515));
#15517=CARTESIAN_POINT('Ctrl Pts',(-8.57413435701377,-1.18591009260195,
20.5257559970408));
#15518=CARTESIAN_POINT('Ctrl Pts',(-8.27600348989981,-1.2045470367323,20.5377591838301));
#15519=CARTESIAN_POINT('Ctrl Pts',(-7.97209482032029,-1.10563290540078,
20.5497623706194));
#15520=CARTESIAN_POINT('Ctrl Pts',(-7.74204705372009,-0.915087963996143,
20.5617655574087));
#15521=CARTESIAN_POINT('Ctrl Pts',(-7.51199928711989,-0.724543022591503,
20.573768744198));
#15522=CARTESIAN_POINT('Ctrl Pts',(-7.3582268807961,-0.444367128060845,
20.5857719309874));
#15523=CARTESIAN_POINT('Ctrl Pts',(-7.32102560975809,-0.147979855989665,
20.5977751177767));
#15524=CARTESIAN_POINT('Ctrl Pts',(-7.28382433872008,0.148407416081515,
20.609778304566));
#15525=CARTESIAN_POINT('Ctrl Pts',(-7.3635846474466,0.45789534472254,20.6217814913553));
#15526=CARTESIAN_POINT('Ctrl Pts',(-7.53940549437917,0.69938318995818,20.6337846781446));
#15527=CARTESIAN_POINT('Ctrl Pts',(-7.71522634131175,0.94087103519382,20.645787864934));
#15528=CARTESIAN_POINT('Ctrl Pts',(-7.98526240565837,1.11182427083107,20.6577910517233));
#15529=CARTESIAN_POINT('Ctrl Pts',(-8.27875123560172,1.16744491727757,20.6697942385126));
#15530=CARTESIAN_POINT('Ctrl Pts',(-8.57224006554506,1.22306556372407,20.6817974253019));
#15531=CARTESIAN_POINT('Ctrl Pts',(-8.88610136059993,1.16276985667007,20.6938006120912));
#15532=CARTESIAN_POINT('Ctrl Pts',(-9.13808834820138,1.00235817476321,20.7058037988805));
#15533=CARTESIAN_POINT('Ctrl Pts',(-9.39007533580283,0.841946492856357,
20.7178069856699));
#15534=CARTESIAN_POINT('Ctrl Pts',(-9.57754329642161,0.583102430602461,
20.7298101724592));
#15535=CARTESIAN_POINT('Ctrl Pts',(-9.65136659729203,0.293655596345746,
20.7418133592485));
#15536=CARTESIAN_POINT('Ctrl Pts',(-9.67581103310553,0.197813707971934,
20.7457878649339));
#15537=CARTESIAN_POINT('Ctrl Pts',(-9.68822500000006,0.098910050091713,
20.7497623706194));
#15538=CARTESIAN_POINT('Ctrl Pts',(-9.688225,-7.75879360759291E-13,20.7537368763049));
#15539=CARTESIAN_POINT('Origin',(-8.5,0.,1.8));
#15540=CARTESIAN_POINT('',(-9.688225,9.66893232146049E-13,21.0962631236951));
#15541=CARTESIAN_POINT('',(-9.6874221426744,0.000106455689637072,21.0537368763049));
#15542=CARTESIAN_POINT('',(-9.688225,-1.45515594291686E-16,1.8));
#15543=CARTESIAN_POINT('Ctrl Pts',(-9.688225,9.66893232146049E-13,21.0962631236951));
#15544=CARTESIAN_POINT('Ctrl Pts',(-9.68822499999976,0.298712821307072,
21.0842599369058));
#15545=CARTESIAN_POINT('Ctrl Pts',(-9.57054245632537,0.595858078272422,
21.0722567501165));
#15546=CARTESIAN_POINT('Ctrl Pts',(-9.36601586214866,0.813569405233449,
21.0602535633272));
#15547=CARTESIAN_POINT('Ctrl Pts',(-9.16148926797196,1.03128073219448,21.0482503765379));
#15548=CARTESIAN_POINT('Ctrl Pts',(-8.87226522412746,1.16727314847168,21.0362471897485));
#15549=CARTESIAN_POINT('Ctrl Pts',(-8.57413435701347,1.18591009260196,21.0242440029592));
#15550=CARTESIAN_POINT('Ctrl Pts',(-8.27600348989949,1.20454703673225,21.0122408161699));
#15551=CARTESIAN_POINT('Ctrl Pts',(-7.97209482031997,1.10563290540063,21.0002376293806));
#15552=CARTESIAN_POINT('Ctrl Pts',(-7.74204705371981,0.915087963995909,
20.9882344425913));
#15553=CARTESIAN_POINT('Ctrl Pts',(-7.51199928711965,0.724543022591183,
20.976231255802));
#15554=CARTESIAN_POINT('Ctrl Pts',(-7.35822688079594,0.444367128060449,
20.9642280690126));
#15555=CARTESIAN_POINT('Ctrl Pts',(-7.32102560975804,0.147979855989233,
20.9522248822233));
#15556=CARTESIAN_POINT('Ctrl Pts',(-7.28382433872013,-0.148407416081984,
20.940221695434));
#15557=CARTESIAN_POINT('Ctrl Pts',(-7.36358464744678,-0.457895344723003,
20.9282185086447));
#15558=CARTESIAN_POINT('Ctrl Pts',(-7.53940549437947,-0.699383189958587,
20.9162153218554));
#15559=CARTESIAN_POINT('Ctrl Pts',(-7.71522634131216,-0.940871035194171,
20.904212135066));
#15560=CARTESIAN_POINT('Ctrl Pts',(-7.98526240565889,-1.11182427083131,
20.8922089482767));
#15561=CARTESIAN_POINT('Ctrl Pts',(-8.27875123560228,-1.16744491727768,
20.8802057614874));
#15562=CARTESIAN_POINT('Ctrl Pts',(-8.57224006554567,-1.22306556372404,
20.8682025746981));
#15563=CARTESIAN_POINT('Ctrl Pts',(-8.88610136060053,-1.16276985666987,
20.8561993879088));
#15564=CARTESIAN_POINT('Ctrl Pts',(-9.13808834820192,-1.00235817476287,
20.8441962011195));
#15565=CARTESIAN_POINT('Ctrl Pts',(-9.3900753358033,-0.841946492855867,
20.8321930143301));
#15566=CARTESIAN_POINT('Ctrl Pts',(-9.57754329642195,-0.583102430601843,
20.8201898275408));
#15567=CARTESIAN_POINT('Ctrl Pts',(-9.6513665972922,-0.293655596345062,
20.8081866407515));
#15568=CARTESIAN_POINT('Ctrl Pts',(-9.67581103310561,-0.197813707971388,
20.804212135066));
#15569=CARTESIAN_POINT('Ctrl Pts',(-9.68822500000008,-0.0989100500913225,
20.8002376293806));
#15570=CARTESIAN_POINT('Ctrl Pts',(-9.688225,1.00885966247688E-12,20.7962631236951));
#15571=CARTESIAN_POINT('Ctrl Pts',(-9.68885519676553,0.00096699279630702,
20.7537368763049));
#15572=CARTESIAN_POINT('Ctrl Pts',(-9.68602600941174,-0.327109604903285,
20.7669463625483));
#15573=CARTESIAN_POINT('Ctrl Pts',(-9.54497968579521,-0.657370321733589,
20.7801558487917));
#15574=CARTESIAN_POINT('Ctrl Pts',(-9.30343789015976,-0.878224528088828,
20.7933653350352));
#15575=CARTESIAN_POINT('Ctrl Pts',(-9.01256452273736,-1.14418515218266,
20.8092726761868));
#15576=CARTESIAN_POINT('Ctrl Pts',(-8.57595415348136,-1.25148612229012,
20.8251800173384));
#15577=CARTESIAN_POINT('Ctrl Pts',(-8.1952758127627,-1.1506442032281,20.84108735849));
#15578=CARTESIAN_POINT('Ctrl Pts',(-7.81459747204409,-1.0498022841661,20.8569946996417));
#15579=CARTESIAN_POINT('Ctrl Pts',(-7.48985115986283,-0.740817475934675,
20.8729020407933));
#15580=CARTESIAN_POINT('Ctrl Pts',(-7.36788212617543,-0.365790383070442,
20.8888093819449));
#15581=CARTESIAN_POINT('Ctrl Pts',(-7.30689760933172,-0.178276836638304,
20.8967630525207));
#15582=CARTESIAN_POINT('Ctrl Pts',(-7.2966074121115,0.025747280952097,20.9047167230965));
#15583=CARTESIAN_POINT('Ctrl Pts',(-7.33354022386741,0.220831256234288,
20.9126703936723));
#15584=CARTESIAN_POINT('Ctrl Pts',(-7.37047303562331,0.415915231516458,
20.9206240642481));
#15585=CARTESIAN_POINT('Ctrl Pts',(-7.45462885635533,0.602059064490469,
20.928577734824));
#15586=CARTESIAN_POINT('Ctrl Pts',(-7.57993567741204,0.754304399351246,
20.9365314053998));
#15587=CARTESIAN_POINT('Ctrl Pts',(-7.83054931952548,1.05879506907282,20.9524387465514));
#15588=CARTESIAN_POINT('Ctrl Pts',(-8.2457669629377,1.2276917463414,20.968346087703));
#15589=CARTESIAN_POINT('Ctrl Pts',(-8.63696275298426,1.18240437964549,20.9842534288546));
#15590=CARTESIAN_POINT('Ctrl Pts',(-9.02815854303084,1.13711701294958,21.0001607700063));
#15591=CARTESIAN_POINT('Ctrl Pts',(-9.39533247971174,0.87764560228914,21.0160681111579));
#15592=CARTESIAN_POINT('Ctrl Pts',(-9.56885922347405,0.523765907133755,
21.0319754523095));
#15593=CARTESIAN_POINT('Ctrl Pts',(-9.64798807787227,0.362395421724354,
21.039229260308));
#15594=CARTESIAN_POINT('Ctrl Pts',(-9.68685003861911,0.181393728166409,
21.0464830683064));
#15595=CARTESIAN_POINT('Ctrl Pts',(-9.68638548896517,0.000243911851261936,
21.0537368763049));
#15596=CARTESIAN_POINT('Origin',(-8.5,0.,1.8));
#15597=CARTESIAN_POINT('',(-9.688225,9.92650406317352E-13,21.3962631236951));
#15598=CARTESIAN_POINT('',(-9.688225,-7.2464256817284E-13,21.3537368763049));
#15599=CARTESIAN_POINT('',(-9.688225,-1.45515594291686E-16,1.8));
#15600=CARTESIAN_POINT('Ctrl Pts',(-9.688225,1.0600409439121E-12,21.3962631236951));
#15601=CARTESIAN_POINT('Ctrl Pts',(-9.68822499999973,0.298712821307165,
21.3842599369058));
#15602=CARTESIAN_POINT('Ctrl Pts',(-9.57054245632532,0.595858078272506,
21.3722567501165));
#15603=CARTESIAN_POINT('Ctrl Pts',(-9.3660158621486,0.813569405233517,21.3602535633272));
#15604=CARTESIAN_POINT('Ctrl Pts',(-9.16148926797188,1.03128073219453,21.3482503765379));
#15605=CARTESIAN_POINT('Ctrl Pts',(-8.87226522412737,1.16727314847171,21.3362471897485));
#15606=CARTESIAN_POINT('Ctrl Pts',(-8.57413435701338,1.18591009260197,21.3242440029592));
#15607=CARTESIAN_POINT('Ctrl Pts',(-8.27600348989939,1.20454703673223,21.3122408161699));
#15608=CARTESIAN_POINT('Ctrl Pts',(-7.97209482031988,1.10563290540059,21.3002376293806));
#15609=CARTESIAN_POINT('Ctrl Pts',(-7.74204705371974,0.915087963995849,
21.2882344425913));
#15610=CARTESIAN_POINT('Ctrl Pts',(-7.51199928711959,0.724543022591105,
21.276231255802));
#15611=CARTESIAN_POINT('Ctrl Pts',(-7.35822688079591,0.444367128060359,
21.2642280690126));
#15612=CARTESIAN_POINT('Ctrl Pts',(-7.32102560975803,0.14797985598914,21.2522248822233));
#15613=CARTESIAN_POINT('Ctrl Pts',(-7.28382433872014,-0.148407416082079,
21.240221695434));
#15614=CARTESIAN_POINT('Ctrl Pts',(-7.36358464744682,-0.457895344723092,
21.2282185086447));
#15615=CARTESIAN_POINT('Ctrl Pts',(-7.53940549437952,-0.699383189958662,
21.2162153218554));
#15616=CARTESIAN_POINT('Ctrl Pts',(-7.71522634131223,-0.940871035194232,
21.204212135066));
#15617=CARTESIAN_POINT('Ctrl Pts',(-7.98526240565897,-1.11182427083135,
21.1922089482767));
#15618=CARTESIAN_POINT('Ctrl Pts',(-8.27875123560237,-1.16744491727769,
21.1802057614874));
#15619=CARTESIAN_POINT('Ctrl Pts',(-8.57224006554577,-1.22306556372404,
21.1682025746981));
#15620=CARTESIAN_POINT('Ctrl Pts',(-8.88610136060063,-1.16276985666984,
21.1561993879088));
#15621=CARTESIAN_POINT('Ctrl Pts',(-9.138088348202,-1.00235817476282,21.1441962011195));
#15622=CARTESIAN_POINT('Ctrl Pts',(-9.39007533580337,-0.841946492855797,
21.1321930143301));
#15623=CARTESIAN_POINT('Ctrl Pts',(-9.57754329642199,-0.583102430601759,
21.1201898275408));
#15624=CARTESIAN_POINT('Ctrl Pts',(-9.65136659729223,-0.293655596344972,
21.1081866407515));
#15625=CARTESIAN_POINT('Ctrl Pts',(-9.67581103310561,-0.197813707971339,
21.104212135066));
#15626=CARTESIAN_POINT('Ctrl Pts',(-9.68822500000008,-0.0989100500913194,
21.1002376293806));
#15627=CARTESIAN_POINT('Ctrl Pts',(-9.688225,9.66893232146049E-13,21.0962631236951));
#15628=CARTESIAN_POINT('Ctrl Pts',(-9.688225,-7.50344231192912E-13,21.0537368763049));
#15629=CARTESIAN_POINT('Ctrl Pts',(-9.68822499999981,-0.298712821306855,
21.0657400630942));
#15630=CARTESIAN_POINT('Ctrl Pts',(-9.57054245632547,-0.595858078272227,
21.0777432498835));
#15631=CARTESIAN_POINT('Ctrl Pts',(-9.36601586214881,-0.813569405233291,
21.0897464366728));
#15632=CARTESIAN_POINT('Ctrl Pts',(-9.16148926797215,-1.03128073219435,
21.1017496234621));
#15633=CARTESIAN_POINT('Ctrl Pts',(-8.87226522412767,-1.16727314847161,
21.1137528102515));
#15634=CARTESIAN_POINT('Ctrl Pts',(-8.57413435701369,-1.18591009260195,
21.1257559970408));
#15635=CARTESIAN_POINT('Ctrl Pts',(-8.2760034898997,-1.20454703673229,21.1377591838301));
#15636=CARTESIAN_POINT('Ctrl Pts',(-7.97209482032017,-1.10563290540073,
21.1497623706194));
#15637=CARTESIAN_POINT('Ctrl Pts',(-7.74204705371998,-0.915087963996047,
21.1617655574087));
#15638=CARTESIAN_POINT('Ctrl Pts',(-7.51199928711978,-0.724543022591362,
21.1737687441981));
#15639=CARTESIAN_POINT('Ctrl Pts',(-7.35822688079602,-0.444367128060657,
21.1857719309874));
#15640=CARTESIAN_POINT('Ctrl Pts',(-7.32102560975807,-0.147979855989448,
21.1977751177767));
#15641=CARTESIAN_POINT('Ctrl Pts',(-7.28382433872011,0.148407416081762,
21.209778304566));
#15642=CARTESIAN_POINT('Ctrl Pts',(-7.3635846474467,0.457895344722796,21.2217814913553));
#15643=CARTESIAN_POINT('Ctrl Pts',(-7.53940549437934,0.699383189958411,
21.2337846781446));
#15644=CARTESIAN_POINT('Ctrl Pts',(-7.71522634131199,0.940871035194027,
21.245787864934));
#15645=CARTESIAN_POINT('Ctrl Pts',(-7.98526240565868,1.11182427083122,21.2577910517233));
#15646=CARTESIAN_POINT('Ctrl Pts',(-8.27875123560207,1.16744491727764,21.2697942385126));
#15647=CARTESIAN_POINT('Ctrl Pts',(-8.57224006554545,1.22306556372406,21.2817974253019));
#15648=CARTESIAN_POINT('Ctrl Pts',(-8.88610136060032,1.16276985666994,21.2938006120912));
#15649=CARTESIAN_POINT('Ctrl Pts',(-9.13808834820174,1.00235817476298,21.3058037988806));
#15650=CARTESIAN_POINT('Ctrl Pts',(-9.39007533580315,0.841946492856029,
21.3178069856699));
#15651=CARTESIAN_POINT('Ctrl Pts',(-9.57754329642184,0.583102430602039,
21.3298101724592));
#15652=CARTESIAN_POINT('Ctrl Pts',(-9.65136659729215,0.293655596345272,
21.3418133592485));
#15653=CARTESIAN_POINT('Ctrl Pts',(-9.67581103310556,0.197813707971646,
21.345787864934));
#15654=CARTESIAN_POINT('Ctrl Pts',(-9.68822500000005,0.0989100500916291,
21.3497623706194));
#15655=CARTESIAN_POINT('Ctrl Pts',(-9.688225,-6.5714100827563E-13,21.3537368763049));
#15656=CARTESIAN_POINT('Origin',(-8.5,0.,1.8));
#15657=CARTESIAN_POINT('',(-9.68941361091145,8.37946601863416E-5,21.6962631236951));
#15658=CARTESIAN_POINT('',(-9.688225,-6.9905192745523E-13,21.6537368763049));
#15659=CARTESIAN_POINT('',(-9.688225,-1.45515594291686E-16,1.8));
#15660=CARTESIAN_POINT('Ctrl Pts',(-9.688225,1.01829655818619E-12,21.6962631236951));
#15661=CARTESIAN_POINT('Ctrl Pts',(-9.68822499999975,0.298712821307101,
21.6842599369058));
#15662=CARTESIAN_POINT('Ctrl Pts',(-9.57054245632536,0.595858078272424,
21.6722567501165));
#15663=CARTESIAN_POINT('Ctrl Pts',(-9.36601586214868,0.813569405233437,
21.6602535633272));
#15664=CARTESIAN_POINT('Ctrl Pts',(-9.16148926797199,1.03128073219445,21.6482503765379));
#15665=CARTESIAN_POINT('Ctrl Pts',(-8.87226522412752,1.16727314847165,21.6362471897486));
#15666=CARTESIAN_POINT('Ctrl Pts',(-8.57413435701356,1.18591009260196,21.6242440029592));
#15667=CARTESIAN_POINT('Ctrl Pts',(-8.27600348989959,1.20454703673226,21.6122408161699));
#15668=CARTESIAN_POINT('Ctrl Pts',(-7.97209482032009,1.10563290540069,21.6002376293806));
#15669=CARTESIAN_POINT('Ctrl Pts',(-7.74204705371992,0.915087963996005,
21.5882344425913));
#15670=CARTESIAN_POINT('Ctrl Pts',(-7.51199928711976,0.724543022591323,
21.576231255802));
#15671=CARTESIAN_POINT('Ctrl Pts',(-7.35822688079602,0.444367128060637,
21.5642280690126));
#15672=CARTESIAN_POINT('Ctrl Pts',(-7.32102560975807,0.14797985598945,21.5522248822233));
#15673=CARTESIAN_POINT('Ctrl Pts',(-7.28382433872011,-0.148407416081737,
21.540221695434));
#15674=CARTESIAN_POINT('Ctrl Pts',(-7.36358464744668,-0.457895344722747,
21.5282185086447));
#15675=CARTESIAN_POINT('Ctrl Pts',(-7.5394054943793,-0.699383189958355,
21.5162153218554));
#15676=CARTESIAN_POINT('Ctrl Pts',(-7.71522634131192,-0.940871035193963,
21.5042121350661));
#15677=CARTESIAN_POINT('Ctrl Pts',(-7.98526240565858,-1.11182427083116,
21.4922089482767));
#15678=CARTESIAN_POINT('Ctrl Pts',(-8.27875123560193,-1.16744491727761,
21.4802057614874));
#15679=CARTESIAN_POINT('Ctrl Pts',(-8.57224006554528,-1.22306556372406,
21.4682025746981));
#15680=CARTESIAN_POINT('Ctrl Pts',(-8.88610136060014,-1.16276985666999,
21.4561993879088));
#15681=CARTESIAN_POINT('Ctrl Pts',(-9.13808834820156,-1.00235817476309,
21.4441962011195));
#15682=CARTESIAN_POINT('Ctrl Pts',(-9.39007533580298,-0.841946492856195,
21.4321930143302));
#15683=CARTESIAN_POINT('Ctrl Pts',(-9.57754329642171,-0.583102430602265,
21.4201898275408));
#15684=CARTESIAN_POINT('Ctrl Pts',(-9.65136659729208,-0.293655596345536,
21.4081866407515));
#15685=CARTESIAN_POINT('Ctrl Pts',(-9.67581103310557,-0.197813707971697,
21.4042121350661));
#15686=CARTESIAN_POINT('Ctrl Pts',(-9.68822500000009,-0.0989100500914515,
21.4002376293806));
#15687=CARTESIAN_POINT('Ctrl Pts',(-9.688225,1.0600409439121E-12,21.3962631236951));
#15688=CARTESIAN_POINT('Ctrl Pts',(-9.688225,-6.5714100827563E-13,21.3537368763049));
#15689=CARTESIAN_POINT('Ctrl Pts',(-9.68822499999983,-0.298712821306739,
21.3657400630942));
#15690=CARTESIAN_POINT('Ctrl Pts',(-9.57054245632554,-0.595858078272098,
21.3777432498835));
#15691=CARTESIAN_POINT('Ctrl Pts',(-9.36601586214892,-0.813569405233174,
21.3897464366728));
#15692=CARTESIAN_POINT('Ctrl Pts',(-9.1614892679723,-1.03128073219425,21.4017496234621));
#15693=CARTESIAN_POINT('Ctrl Pts',(-8.87226522412787,-1.16727314847154,
21.4137528102515));
#15694=CARTESIAN_POINT('Ctrl Pts',(-8.57413435701392,-1.18591009260194,
21.4257559970408));
#15695=CARTESIAN_POINT('Ctrl Pts',(-8.27600348989996,-1.20454703673233,
21.4377591838301));
#15696=CARTESIAN_POINT('Ctrl Pts',(-7.97209482032043,-1.10563290540085,
21.4497623706194));
#15697=CARTESIAN_POINT('Ctrl Pts',(-7.7420470537202,-0.915087963996235,
21.4617655574087));
#15698=CARTESIAN_POINT('Ctrl Pts',(-7.51199928711998,-0.724543022591623,
21.473768744198));
#15699=CARTESIAN_POINT('Ctrl Pts',(-7.35822688079616,-0.444367128060984,
21.4857719309874));
#15700=CARTESIAN_POINT('Ctrl Pts',(-7.32102560975811,-0.147979855989808,
21.4977751177767));
#15701=CARTESIAN_POINT('Ctrl Pts',(-7.28382433872006,0.148407416081368,
21.509778304566));
#15702=CARTESIAN_POINT('Ctrl Pts',(-7.36358464744655,0.457895344722402,
21.5217814913553));
#15703=CARTESIAN_POINT('Ctrl Pts',(-7.53940549437909,0.699383189958063,
21.5337846781446));
#15704=CARTESIAN_POINT('Ctrl Pts',(-7.71522634131163,0.940871035193724,
21.5457878649339));
#15705=CARTESIAN_POINT('Ctrl Pts',(-7.98526240565824,1.11182427083101,21.5577910517233));
#15706=CARTESIAN_POINT('Ctrl Pts',(-8.27875123560158,1.16744491727754,21.5697942385126));
#15707=CARTESIAN_POINT('Ctrl Pts',(-8.57224006554491,1.22306556372408,21.5817974253019));
#15708=CARTESIAN_POINT('Ctrl Pts',(-8.88610136059979,1.16276985667011,21.5938006120912));
#15709=CARTESIAN_POINT('Ctrl Pts',(-9.13808834820126,1.00235817476329,21.6058037988805));
#15710=CARTESIAN_POINT('Ctrl Pts',(-9.39007533580273,0.841946492856465,
21.6178069856699));
#15711=CARTESIAN_POINT('Ctrl Pts',(-9.57754329642153,0.583102430602592,
21.6298101724592));
#15712=CARTESIAN_POINT('Ctrl Pts',(-9.65136659729199,0.293655596345886,
21.6418133592485));
#15713=CARTESIAN_POINT('Ctrl Pts',(-9.67581103310551,0.197813707972055,
21.6457878649339));
#15714=CARTESIAN_POINT('Ctrl Pts',(-9.68822500000006,0.0989100500918124,
21.6497623706194));
#15715=CARTESIAN_POINT('Ctrl Pts',(-9.688225,-6.9905192745523E-13,21.6537368763049));
#15716=CARTESIAN_POINT('Origin',(-8.5,0.,1.8));
#15717=CARTESIAN_POINT('',(-9.68754848723268,0.00103932034338594,21.9962631236951));
#15718=CARTESIAN_POINT('',(-9.688225,-6.7346128673762E-13,21.9537368763049));
#15719=CARTESIAN_POINT('',(-9.688225,-1.45515594291686E-16,1.8));
#15720=CARTESIAN_POINT('Ctrl Pts',(-9.68754848723268,0.00103932034338594,
21.9962631236951));
#15721=CARTESIAN_POINT('Ctrl Pts',(-9.68846371561513,0.113646838372302,
21.9917421023245));
#15722=CARTESIAN_POINT('Ctrl Pts',(-9.67372334216155,0.22601158102592,21.9872210809538));
#15723=CARTESIAN_POINT('Ctrl Pts',(-9.64233633231695,0.333516176657786,
21.9827000595831));
#15724=CARTESIAN_POINT('Ctrl Pts',(-9.53190025330015,0.711774127212782,
21.9667927184315));
#15725=CARTESIAN_POINT('Ctrl Pts',(-9.21537813921845,1.02986326011492,21.9508853772799));
#15726=CARTESIAN_POINT('Ctrl Pts',(-8.83737688077721,1.14147606431245,21.9349780361283));
#15727=CARTESIAN_POINT('Ctrl Pts',(-8.45937562233595,1.25308886850999,21.9190706949767));
#15728=CARTESIAN_POINT('Ctrl Pts',(-8.01989521953514,1.15822534400289,21.903163353825));
#15729=CARTESIAN_POINT('Ctrl Pts',(-7.72189584988414,0.900773470014709,
21.8872560126734));
#15730=CARTESIAN_POINT('Ctrl Pts',(-7.42389648023317,0.643321596026557,
21.8713486715218));
#15731=CARTESIAN_POINT('Ctrl Pts',(-7.26737814373198,0.223281372557366,
21.8554413303702));
#15732=CARTESIAN_POINT('Ctrl Pts',(-7.32207205408808,-0.16726995791123,
21.8395339892186));
#15733=CARTESIAN_POINT('Ctrl Pts',(-7.34941900926613,-0.36254562314555,
21.8315803186428));
#15734=CARTESIAN_POINT('Ctrl Pts',(-7.42956902615852,-0.55044906512972,
21.823626648067));
#15735=CARTESIAN_POINT('Ctrl Pts',(-7.54824974241705,-0.70962405557879,
21.8156729774911));
#15736=CARTESIAN_POINT('Ctrl Pts',(-7.66693045867558,-0.86879904602786,
21.8077193069153));
#15737=CARTESIAN_POINT('Ctrl Pts',(-7.82414187430025,-0.999245584941831,
21.7997656363395));
#15738=CARTESIAN_POINT('Ctrl Pts',(-8.00348963778739,-1.08118959706215,
21.7918119657637));
#15739=CARTESIAN_POINT('Ctrl Pts',(-8.36218516476167,-1.24507762130277,
21.7759046246121));
#15740=CARTESIAN_POINT('Ctrl Pts',(-8.80942608318585,-1.21495553836879,
21.7599972834604));
#15741=CARTESIAN_POINT('Ctrl Pts',(-9.14122245772507,-1.00283232517649,
21.7440899423088));
#15742=CARTESIAN_POINT('Ctrl Pts',(-9.4730188322643,-0.790709111984192,
21.7281826011572));
#15743=CARTESIAN_POINT('Ctrl Pts',(-9.68937066291857,-0.396584768533572,
21.7122752600056));
#15744=CARTESIAN_POINT('Ctrl Pts',(-9.69028767880224,-0.00245087183618204,
21.696367918854));
#15745=CARTESIAN_POINT('Ctrl Pts',(-9.69028969252292,-0.00158537365915197,
21.6963329871344));
#15746=CARTESIAN_POINT('Ctrl Pts',(-9.69029066737497,-0.000719875436054535,
21.6962980554148));
#15747=CARTESIAN_POINT('Ctrl Pts',(-9.6902906044062,0.000145620923329259,
21.6962631236951));
#15748=CARTESIAN_POINT('Ctrl Pts',(-9.688225,-6.9905192745523E-13,21.6537368763049));
#15749=CARTESIAN_POINT('Ctrl Pts',(-9.68822499999982,-0.298712821306781,
21.6657400630942));
#15750=CARTESIAN_POINT('Ctrl Pts',(-9.57054245632552,-0.595858078272136,
21.6777432498835));
#15751=CARTESIAN_POINT('Ctrl Pts',(-9.36601586214889,-0.813569405233204,
21.6897464366728));
#15752=CARTESIAN_POINT('Ctrl Pts',(-9.16148926797227,-1.03128073219427,
21.7017496234621));
#15753=CARTESIAN_POINT('Ctrl Pts',(-8.87226522412783,-1.16727314847155,
21.7137528102515));
#15754=CARTESIAN_POINT('Ctrl Pts',(-8.57413435701387,-1.18591009260194,
21.7257559970408));
#15755=CARTESIAN_POINT('Ctrl Pts',(-8.27600348989992,-1.20454703673232,
21.7377591838301));
#15756=CARTESIAN_POINT('Ctrl Pts',(-7.97209482032039,-1.10563290540083,
21.7497623706194));
#15757=CARTESIAN_POINT('Ctrl Pts',(-7.74204705372017,-0.915087963996209,
21.7617655574087));
#15758=CARTESIAN_POINT('Ctrl Pts',(-7.51199928711995,-0.724543022591588,
21.773768744198));
#15759=CARTESIAN_POINT('Ctrl Pts',(-7.35822688079614,-0.444367128060944,
21.7857719309874));
#15760=CARTESIAN_POINT('Ctrl Pts',(-7.32102560975811,-0.147979855989767,
21.7977751177767));
#15761=CARTESIAN_POINT('Ctrl Pts',(-7.28382433872007,0.14840741608141,21.809778304566));
#15762=CARTESIAN_POINT('Ctrl Pts',(-7.36358464744656,0.457895344722442,
21.8217814913553));
#15763=CARTESIAN_POINT('Ctrl Pts',(-7.53940549437911,0.699383189958097,
21.8337846781446));
#15764=CARTESIAN_POINT('Ctrl Pts',(-7.71522634131166,0.940871035193752,
21.8457878649339));
#15765=CARTESIAN_POINT('Ctrl Pts',(-7.98526240565828,1.11182427083102,21.8577910517233));
#15766=CARTESIAN_POINT('Ctrl Pts',(-8.27875123560162,1.16744491727755,21.8697942385126));
#15767=CARTESIAN_POINT('Ctrl Pts',(-8.57224006554496,1.22306556372408,21.8817974253019));
#15768=CARTESIAN_POINT('Ctrl Pts',(-8.88610136059983,1.1627698566701,21.8938006120912));
#15769=CARTESIAN_POINT('Ctrl Pts',(-9.13808834820129,1.00235817476327,21.9058037988805));
#15770=CARTESIAN_POINT('Ctrl Pts',(-9.39007533580276,0.841946492856433,
21.9178069856699));
#15771=CARTESIAN_POINT('Ctrl Pts',(-9.57754329642156,0.583102430602554,
21.9298101724592));
#15772=CARTESIAN_POINT('Ctrl Pts',(-9.651366597292,0.293655596345845,21.9418133592485));
#15773=CARTESIAN_POINT('Ctrl Pts',(-9.67581103310551,0.197813707972057,
21.9457878649339));
#15774=CARTESIAN_POINT('Ctrl Pts',(-9.68822500000005,0.0989100500918605,
21.9497623706194));
#15775=CARTESIAN_POINT('Ctrl Pts',(-9.688225,-6.05904215689179E-13,21.9537368763049));
#15776=CARTESIAN_POINT('Origin',(-8.5,0.,1.8));
#15777=CARTESIAN_POINT('',(-9.6873844249699,-0.000213222977800639,22.2962631236951));
#15778=CARTESIAN_POINT('',(-9.688225,-6.47759623717548E-13,22.2537368763049));
#15779=CARTESIAN_POINT('',(-9.688225,-1.45515594291686E-16,1.8));
#15780=CARTESIAN_POINT('Ctrl Pts',(-9.68642524001508,-0.000456532936506715,
22.2962631236951));
#15781=CARTESIAN_POINT('Ctrl Pts',(-9.68575927361135,0.226185688933078,
22.2871861492342));
#15782=CARTESIAN_POINT('Ctrl Pts',(-9.62343522762896,0.453218610314175,
22.2781091747733));
#15783=CARTESIAN_POINT('Ctrl Pts',(-9.50198612166228,0.642506480183205,
22.2690322003123));
#15784=CARTESIAN_POINT('Ctrl Pts',(-9.28914732064055,0.974232291997172,
22.2531248591607));
#15785=CARTESIAN_POINT('Ctrl Pts',(-8.89472160162217,1.19003420325999,22.2372175180091));
#15786=CARTESIAN_POINT('Ctrl Pts',(-8.50091325276927,1.19031007669399,22.2213101768575));
#15787=CARTESIAN_POINT('Ctrl Pts',(-8.10710490391636,1.19058595012799,22.2054028357058));
#15788=CARTESIAN_POINT('Ctrl Pts',(-7.71391392522893,0.975335785733172,
22.1894954945542));
#15789=CARTESIAN_POINT('Ctrl Pts',(-7.49974687085622,0.644194972207926,
22.1735881534026));
#15790=CARTESIAN_POINT('Ctrl Pts',(-7.39266334366985,0.478624565445293,
22.1656344828268));
#15791=CARTESIAN_POINT('Ctrl Pts',(-7.33033579756217,0.28408149640005,22.157680812251));
#15792=CARTESIAN_POINT('Ctrl Pts',(-7.31594364125642,0.0860545895591625,
22.1497271416752));
#15793=CARTESIAN_POINT('Ctrl Pts',(-7.30155148495066,-0.111972317281703,
22.1417734710994));
#15794=CARTESIAN_POINT('Ctrl Pts',(-7.33509471844682,-0.313483061918211,
22.1338198005235));
#15795=CARTESIAN_POINT('Ctrl Pts',(-7.41711281973766,-0.492796955554075,
22.1258661299477));
#15796=CARTESIAN_POINT('Ctrl Pts',(-7.58114902231934,-0.851424742825822,
22.1099587887961));
#15797=CARTESIAN_POINT('Ctrl Pts',(-7.93908469607976,-1.12126512609498,
22.0940514476445));
#15798=CARTESIAN_POINT('Ctrl Pts',(-8.32879455452619,-1.17793361788769,
22.0781441064929));
#15799=CARTESIAN_POINT('Ctrl Pts',(-8.71850441297263,-1.2346021096804,22.0622367653413));
#15800=CARTESIAN_POINT('Ctrl Pts',(-9.13998845610508,-1.07809870999666,
22.0463294241896));
#15801=CARTESIAN_POINT('Ctrl Pts',(-9.39855545569536,-0.780633626050859,
22.030422083038));
#15802=CARTESIAN_POINT('Ctrl Pts',(-9.58363519429373,-0.567711017728565,
22.019035763257));
#15803=CARTESIAN_POINT('Ctrl Pts',(-9.68524345874889,-0.282565888500901,
22.0076494434761));
#15804=CARTESIAN_POINT('Ctrl Pts',(-9.68754848723268,0.00103932034338594,
21.9962631236951));
#15805=CARTESIAN_POINT('Ctrl Pts',(-9.688225,-6.05904215689179E-13,21.9537368763049));
#15806=CARTESIAN_POINT('Ctrl Pts',(-9.68822499999985,-0.298712821306711,
21.9657400630942));
#15807=CARTESIAN_POINT('Ctrl Pts',(-9.57054245632555,-0.595858078272097,
21.9777432498835));
#15808=CARTESIAN_POINT('Ctrl Pts',(-9.36601586214891,-0.813569405233185,
21.9897464366728));
#15809=CARTESIAN_POINT('Ctrl Pts',(-9.16148926797228,-1.03128073219427,
22.0017496234621));
#15810=CARTESIAN_POINT('Ctrl Pts',(-8.87226522412781,-1.16727314847157,
22.0137528102515));
#15811=CARTESIAN_POINT('Ctrl Pts',(-8.57413435701383,-1.18591009260194,
22.0257559970408));
#15812=CARTESIAN_POINT('Ctrl Pts',(-8.27600348989985,-1.20454703673232,
22.0377591838301));
#15813=CARTESIAN_POINT('Ctrl Pts',(-7.97209482032031,-1.10563290540079,
22.0497623706194));
#15814=CARTESIAN_POINT('Ctrl Pts',(-7.74204705372009,-0.915087963996139,
22.0617655574087));
#15815=CARTESIAN_POINT('Ctrl Pts',(-7.51199928711987,-0.724543022591483,
22.073768744198));
#15816=CARTESIAN_POINT('Ctrl Pts',(-7.35822688079608,-0.444367128060796,
22.0857719309874));
#15817=CARTESIAN_POINT('Ctrl Pts',(-7.32102560975808,-0.147979855989591,
22.0977751177767));
#15818=CARTESIAN_POINT('Ctrl Pts',(-7.28382433872009,0.148407416081614,
22.109778304566));
#15819=CARTESIAN_POINT('Ctrl Pts',(-7.36358464744664,0.457895344722657,
22.1217814913553));
#15820=CARTESIAN_POINT('Ctrl Pts',(-7.53940549437926,0.699383189958295,
22.1337846781446));
#15821=CARTESIAN_POINT('Ctrl Pts',(-7.71522634131187,0.940871035193932,
22.145787864934));
#15822=CARTESIAN_POINT('Ctrl Pts',(-7.98526240565855,1.11182427083115,22.1577910517233));
#15823=CARTESIAN_POINT('Ctrl Pts',(-8.27875123560192,1.16744491727761,22.1697942385126));
#15824=CARTESIAN_POINT('Ctrl Pts',(-8.5722400655453,1.22306556372406,22.1817974253019));
#15825=CARTESIAN_POINT('Ctrl Pts',(-8.88610136060018,1.16276985666999,22.1938006120912));
#15826=CARTESIAN_POINT('Ctrl Pts',(-9.13808834820161,1.00235817476306,22.2058037988805));
#15827=CARTESIAN_POINT('Ctrl Pts',(-9.39007533580305,0.841946492856137,
22.2178069856699));
#15828=CARTESIAN_POINT('Ctrl Pts',(-9.57754329642177,0.58310243060217,22.2298101724592));
#15829=CARTESIAN_POINT('Ctrl Pts',(-9.65136659729211,0.293655596345412,
22.2418133592485));
#15830=CARTESIAN_POINT('Ctrl Pts',(-9.67581103310554,0.197813707971767,
22.245787864934));
#15831=CARTESIAN_POINT('Ctrl Pts',(-9.68822500000005,0.0989100500917286,
22.2497623706194));
#15832=CARTESIAN_POINT('Ctrl Pts',(-9.688225,-5.80202552669107E-13,22.2537368763049));
#15833=CARTESIAN_POINT('Origin',(-8.5,0.,1.8));
#15834=CARTESIAN_POINT('',(-9.688225,1.09501296918779E-12,22.5962631236951));
#15835=CARTESIAN_POINT('',(-9.688225,-6.22168982999938E-13,22.5537368763049));
#15836=CARTESIAN_POINT('',(-9.688225,-1.45515594291686E-16,1.8));
#15837=CARTESIAN_POINT('Ctrl Pts',(-9.688225,1.16262555138746E-12,22.5962631236951));
#15838=CARTESIAN_POINT('Ctrl Pts',(-9.68822499999971,0.298712821307267,
22.5842599369058));
#15839=CARTESIAN_POINT('Ctrl Pts',(-9.57054245632527,0.595858078272598,
22.5722567501165));
#15840=CARTESIAN_POINT('Ctrl Pts',(-9.36601586214853,0.813569405233591,
22.5602535633272));
#15841=CARTESIAN_POINT('Ctrl Pts',(-9.16148926797179,1.03128073219458,22.5482503765379));
#15842=CARTESIAN_POINT('Ctrl Pts',(-8.87226522412727,1.16727314847174,22.5362471897485));
#15843=CARTESIAN_POINT('Ctrl Pts',(-8.57413435701328,1.18591009260198,22.5242440029592));
#15844=CARTESIAN_POINT('Ctrl Pts',(-8.27600348989929,1.20454703673221,22.5122408161699));
#15845=CARTESIAN_POINT('Ctrl Pts',(-7.97209482031979,1.10563290540055,22.5002376293806));
#15846=CARTESIAN_POINT('Ctrl Pts',(-7.74204705371966,0.915087963995784,
22.4882344425913));
#15847=CARTESIAN_POINT('Ctrl Pts',(-7.51199928711953,0.72454302259102,22.4762312558019));
#15848=CARTESIAN_POINT('Ctrl Pts',(-7.35822688079587,0.444367128060261,
22.4642280690126));
#15849=CARTESIAN_POINT('Ctrl Pts',(-7.32102560975801,0.147979855989039,
22.4522248822233));
#15850=CARTESIAN_POINT('Ctrl Pts',(-7.28382433872016,-0.148407416082184,
22.440221695434));
#15851=CARTESIAN_POINT('Ctrl Pts',(-7.36358464744686,-0.45789534472319,
22.4282185086447));
#15852=CARTESIAN_POINT('Ctrl Pts',(-7.53940549437958,-0.699383189958745,
22.4162153218554));
#15853=CARTESIAN_POINT('Ctrl Pts',(-7.71522634131231,-0.9408710351943,22.404212135066));
#15854=CARTESIAN_POINT('Ctrl Pts',(-7.98526240565907,-1.1118242708314,22.3922089482767));
#15855=CARTESIAN_POINT('Ctrl Pts',(-8.27875123560247,-1.16744491727771,
22.3802057614874));
#15856=CARTESIAN_POINT('Ctrl Pts',(-8.57224006554587,-1.22306556372403,
22.3682025746981));
#15857=CARTESIAN_POINT('Ctrl Pts',(-8.88610136060073,-1.16276985666981,
22.3561993879088));
#15858=CARTESIAN_POINT('Ctrl Pts',(-9.13808834820208,-1.00235817476276,
22.3441962011194));
#15859=CARTESIAN_POINT('Ctrl Pts',(-9.39007533580344,-0.84194649285572,
22.3321930143301));
#15860=CARTESIAN_POINT('Ctrl Pts',(-9.57754329642204,-0.583102430601666,
22.3201898275408));
#15861=CARTESIAN_POINT('Ctrl Pts',(-9.65136659729225,-0.293655596344872,
22.3081866407515));
#15862=CARTESIAN_POINT('Ctrl Pts',(-9.67581103310563,-0.197813707971238,
22.304212135066));
#15863=CARTESIAN_POINT('Ctrl Pts',(-9.68822500000009,-0.0989100500912168,
22.3002376293806));
#15864=CARTESIAN_POINT('Ctrl Pts',(-9.688225,1.06947783962141E-12,22.2962631236951));
#15865=CARTESIAN_POINT('Ctrl Pts',(-9.688225,-5.80202552669107E-13,22.2537368763049));
#15866=CARTESIAN_POINT('Ctrl Pts',(-9.68822499999985,-0.298712821306662,
22.2657400630942));
#15867=CARTESIAN_POINT('Ctrl Pts',(-9.57054245632558,-0.595858078272029,
22.2777432498835));
#15868=CARTESIAN_POINT('Ctrl Pts',(-9.36601586214897,-0.813569405233117,
22.2897464366728));
#15869=CARTESIAN_POINT('Ctrl Pts',(-9.16148926797237,-1.03128073219421,
22.3017496234621));
#15870=CARTESIAN_POINT('Ctrl Pts',(-8.87226522412795,-1.16727314847152,
22.3137528102515));
#15871=CARTESIAN_POINT('Ctrl Pts',(-8.57413435701399,-1.18591009260193,
22.3257559970408));
#15872=CARTESIAN_POINT('Ctrl Pts',(-8.27600348990004,-1.20454703673235,
22.3377591838301));
#15873=CARTESIAN_POINT('Ctrl Pts',(-7.9720948203205,-1.10563290540088,22.3497623706194));
#15874=CARTESIAN_POINT('Ctrl Pts',(-7.74204705372026,-0.915087963996284,
22.3617655574087));
#15875=CARTESIAN_POINT('Ctrl Pts',(-7.51199928712002,-0.724543022591687,
22.373768744198));
#15876=CARTESIAN_POINT('Ctrl Pts',(-7.35822688079619,-0.444367128061058,
22.3857719309874));
#15877=CARTESIAN_POINT('Ctrl Pts',(-7.32102560975812,-0.147979855989884,
22.3977751177767));
#15878=CARTESIAN_POINT('Ctrl Pts',(-7.28382433872005,0.148407416081289,
22.409778304566));
#15879=CARTESIAN_POINT('Ctrl Pts',(-7.36358464744652,0.457895344722328,
22.4217814913553));
#15880=CARTESIAN_POINT('Ctrl Pts',(-7.53940549437904,0.699383189958001,
22.4337846781446));
#15881=CARTESIAN_POINT('Ctrl Pts',(-7.71522634131157,0.940871035193674,
22.4457878649339));
#15882=CARTESIAN_POINT('Ctrl Pts',(-7.98526240565817,1.11182427083097,22.4577910517233));
#15883=CARTESIAN_POINT('Ctrl Pts',(-8.2787512356015,1.16744491727753,22.4697942385126));
#15884=CARTESIAN_POINT('Ctrl Pts',(-8.57224006554483,1.22306556372409,22.4817974253019));
#15885=CARTESIAN_POINT('Ctrl Pts',(-8.88610136059971,1.16276985667014,22.4938006120912));
#15886=CARTESIAN_POINT('Ctrl Pts',(-9.13808834820119,1.00235817476333,22.5058037988805));
#15887=CARTESIAN_POINT('Ctrl Pts',(-9.39007533580267,0.841946492856522,
22.5178069856698));
#15888=CARTESIAN_POINT('Ctrl Pts',(-9.5775432964215,0.583102430602662,22.5298101724592));
#15889=CARTESIAN_POINT('Ctrl Pts',(-9.65136659729197,0.29365559634596,22.5418133592485));
#15890=CARTESIAN_POINT('Ctrl Pts',(-9.67581103310549,0.197813707972153,
22.5457878649339));
#15891=CARTESIAN_POINT('Ctrl Pts',(-9.68822500000005,0.0989100500919342,
22.5497623706194));
#15892=CARTESIAN_POINT('Ctrl Pts',(-9.688225,-5.54667423102728E-13,22.5537368763049));
#15893=CARTESIAN_POINT('Origin',(-8.5,0.,1.8));
#15894=CARTESIAN_POINT('',(-9.688225,1.12065912105663E-12,22.8962631236951));
#15895=CARTESIAN_POINT('',(-9.688225,-5.96633853433559E-13,22.8537368763049));
#15896=CARTESIAN_POINT('',(-9.688225,-1.45515594291686E-16,1.8));
#15897=CARTESIAN_POINT('Ctrl Pts',(-9.688225,1.12065912105663E-12,22.8962631236951));
#15898=CARTESIAN_POINT('Ctrl Pts',(-9.68822499999972,0.298712821307135,
22.8842599369058));
#15899=CARTESIAN_POINT('Ctrl Pts',(-9.57054245632536,0.595858078272383,
22.8722567501165));
#15900=CARTESIAN_POINT('Ctrl Pts',(-9.36601586214874,0.813569405233364,
22.8602535633272));
#15901=CARTESIAN_POINT('Ctrl Pts',(-9.16148926797212,1.03128073219435,22.8482503765379));
#15902=CARTESIAN_POINT('Ctrl Pts',(-8.87226522412775,1.16727314847156,22.8362471897486));
#15903=CARTESIAN_POINT('Ctrl Pts',(-8.57413435701386,1.18591009260194,22.8242440029592));
#15904=CARTESIAN_POINT('Ctrl Pts',(-8.27600348989997,1.20454703673232,22.8122408161699));
#15905=CARTESIAN_POINT('Ctrl Pts',(-7.97209482032051,1.10563290540087,22.8002376293806));
#15906=CARTESIAN_POINT('Ctrl Pts',(-7.74204705372031,0.915087963996328,
22.7882344425913));
#15907=CARTESIAN_POINT('Ctrl Pts',(-7.51199928712012,0.724543022591786,
22.776231255802));
#15908=CARTESIAN_POINT('Ctrl Pts',(-7.35822688079628,0.44436712806125,22.7642280690127));
#15909=CARTESIAN_POINT('Ctrl Pts',(-7.32102560975815,0.147979855990152,
22.7522248822234));
#15910=CARTESIAN_POINT('Ctrl Pts',(-7.28382433872003,-0.148407416080945,
22.740221695434));
#15911=CARTESIAN_POINT('Ctrl Pts',(-7.36358464744637,-0.457895344721931,
22.7282185086447));
#15912=CARTESIAN_POINT('Ctrl Pts',(-7.53940549437876,-0.699383189957619,
22.7162153218554));
#15913=CARTESIAN_POINT('Ctrl Pts',(-7.71522634131116,-0.940871035193307,
22.7042121350661));
#15914=CARTESIAN_POINT('Ctrl Pts',(-7.9852624056576,-1.11182427083069,22.6922089482768));
#15915=CARTESIAN_POINT('Ctrl Pts',(-8.27875123560084,-1.1674449172774,22.6802057614875));
#15916=CARTESIAN_POINT('Ctrl Pts',(-8.57224006554407,-1.22306556372412,
22.6682025746982));
#15917=CARTESIAN_POINT('Ctrl Pts',(-8.88610136059891,-1.16276985667039,
22.6561993879088));
#15918=CARTESIAN_POINT('Ctrl Pts',(-9.13808834820045,-1.0023581747638,22.6441962011195));
#15919=CARTESIAN_POINT('Ctrl Pts',(-9.39007533580199,-0.841946492857216,
22.6321930143302));
#15920=CARTESIAN_POINT('Ctrl Pts',(-9.57754329642098,-0.583102430603576,
22.6201898275409));
#15921=CARTESIAN_POINT('Ctrl Pts',(-9.65136659729171,-0.293655596347007,
22.6081866407516));
#15922=CARTESIAN_POINT('Ctrl Pts',(-9.67581103310545,-0.197813707972676,
22.6042121350661));
#15923=CARTESIAN_POINT('Ctrl Pts',(-9.6882250000001,-0.0989100500918892,
22.6002376293806));
#15924=CARTESIAN_POINT('Ctrl Pts',(-9.688225,1.16262555138746E-12,22.5962631236951));
#15925=CARTESIAN_POINT('Ctrl Pts',(-9.688225,-5.54667423102728E-13,22.5537368763049));
#15926=CARTESIAN_POINT('Ctrl Pts',(-9.68822499999986,-0.298712821306682,
22.5657400630942));
#15927=CARTESIAN_POINT('Ctrl Pts',(-9.57054245632555,-0.595858078272095,
22.5777432498835));
#15928=CARTESIAN_POINT('Ctrl Pts',(-9.3660158621489,-0.813569405233197,
22.5897464366728));
#15929=CARTESIAN_POINT('Ctrl Pts',(-9.16148926797224,-1.0312807321943,22.6017496234621));
#15930=CARTESIAN_POINT('Ctrl Pts',(-8.87226522412775,-1.16727314847159,
22.6137528102515));
#15931=CARTESIAN_POINT('Ctrl Pts',(-8.57413435701375,-1.18591009260195,
22.6257559970408));
#15932=CARTESIAN_POINT('Ctrl Pts',(-8.27600348989974,-1.2045470367323,22.6377591838301));
#15933=CARTESIAN_POINT('Ctrl Pts',(-7.97209482032018,-1.10563290540074,
22.6497623706194));
#15934=CARTESIAN_POINT('Ctrl Pts',(-7.74204705371997,-0.915087963996042,
22.6617655574087));
#15935=CARTESIAN_POINT('Ctrl Pts',(-7.51199928711976,-0.724543022591342,
22.6737687441981));
#15936=CARTESIAN_POINT('Ctrl Pts',(-7.358226880796,-0.444367128060608,22.6857719309874));
#15937=CARTESIAN_POINT('Ctrl Pts',(-7.32102560975806,-0.147979855989374,
22.6977751177767));
#15938=CARTESIAN_POINT('Ctrl Pts',(-7.28382433872011,0.14840741608186,22.709778304566));
#15939=CARTESIAN_POINT('Ctrl Pts',(-7.36358464744674,0.457895344722913,
22.7217814913553));
#15940=CARTESIAN_POINT('Ctrl Pts',(-7.53940549437942,0.699383189958526,
22.7337846781447));
#15941=CARTESIAN_POINT('Ctrl Pts',(-7.71522634131211,0.940871035194139,
22.745787864934));
#15942=CARTESIAN_POINT('Ctrl Pts',(-7.98526240565886,1.1118242708313,22.7577910517233));
#15943=CARTESIAN_POINT('Ctrl Pts',(-8.27875123560227,1.16744491727768,22.7697942385126));
#15944=CARTESIAN_POINT('Ctrl Pts',(-8.57224006554569,1.22306556372405,22.7817974253019));
#15945=CARTESIAN_POINT('Ctrl Pts',(-8.88610136060057,1.16276985666986,22.7938006120912));
#15946=CARTESIAN_POINT('Ctrl Pts',(-9.13808834820197,1.00235817476284,22.8058037988806));
#15947=CARTESIAN_POINT('Ctrl Pts',(-9.39007533580336,0.841946492855809,
22.8178069856699));
#15948=CARTESIAN_POINT('Ctrl Pts',(-9.577543296422,0.583102430601749,22.8298101724592));
#15949=CARTESIAN_POINT('Ctrl Pts',(-9.65136659729223,0.293655596344938,
22.8418133592485));
#15950=CARTESIAN_POINT('Ctrl Pts',(-9.67581103310559,0.197813707971436,
22.845787864934));
#15951=CARTESIAN_POINT('Ctrl Pts',(-9.68822500000005,0.0989100500915545,
22.8497623706194));
#15952=CARTESIAN_POINT('Ctrl Pts',(-9.688225,-5.96633853433559E-13,22.8537368763049));
#15953=CARTESIAN_POINT('Origin',(-8.5,0.,1.8));
#15954=CARTESIAN_POINT('',(-9.688225,1.14630527292547E-12,23.1962631236951));
#15955=CARTESIAN_POINT('',(-9.688225,-5.70987701564718E-13,23.1537368763049));
#15956=CARTESIAN_POINT('',(-9.688225,-1.45515594291686E-16,1.8));
#15957=CARTESIAN_POINT('Ctrl Pts',(-9.688225,1.21391785512515E-12,23.1962631236951));
#15958=CARTESIAN_POINT('Ctrl Pts',(-9.6882249999997,0.298712821307319,23.1842599369058));
#15959=CARTESIAN_POINT('Ctrl Pts',(-9.57054245632524,0.595858078272645,
23.1722567501165));
#15960=CARTESIAN_POINT('Ctrl Pts',(-9.36601586214849,0.813569405233629,
23.1602535633272));
#15961=CARTESIAN_POINT('Ctrl Pts',(-9.16148926797175,1.03128073219461,23.1482503765379));
#15962=CARTESIAN_POINT('Ctrl Pts',(-8.87226522412722,1.16727314847176,23.1362471897485));
#15963=CARTESIAN_POINT('Ctrl Pts',(-8.57413435701323,1.18591009260198,23.1242440029592));
#15964=CARTESIAN_POINT('Ctrl Pts',(-8.27600348989924,1.2045470367322,23.1122408161699));
#15965=CARTESIAN_POINT('Ctrl Pts',(-7.97209482031974,1.10563290540052,23.1002376293806));
#15966=CARTESIAN_POINT('Ctrl Pts',(-7.74204705371962,0.915087963995751,
23.0882344425913));
#15967=CARTESIAN_POINT('Ctrl Pts',(-7.5119992871195,0.724543022590977,23.0762312558019));
#15968=CARTESIAN_POINT('Ctrl Pts',(-7.35822688079585,0.444367128060212,
23.0642280690126));
#15969=CARTESIAN_POINT('Ctrl Pts',(-7.32102560975801,0.147979855988988,
23.0522248822233));
#15970=CARTESIAN_POINT('Ctrl Pts',(-7.28382433872016,-0.148407416082236,
23.040221695434));
#15971=CARTESIAN_POINT('Ctrl Pts',(-7.36358464744688,-0.457895344723239,
23.0282185086447));
#15972=CARTESIAN_POINT('Ctrl Pts',(-7.53940549437961,-0.699383189958786,
23.0162153218554));
#15973=CARTESIAN_POINT('Ctrl Pts',(-7.71522634131235,-0.940871035194334,
23.004212135066));
#15974=CARTESIAN_POINT('Ctrl Pts',(-7.98526240565912,-1.11182427083142,
22.9922089482767));
#15975=CARTESIAN_POINT('Ctrl Pts',(-8.27875123560252,-1.16744491727772,
22.9802057614874));
#15976=CARTESIAN_POINT('Ctrl Pts',(-8.57224006554592,-1.22306556372403,
22.9682025746981));
#15977=CARTESIAN_POINT('Ctrl Pts',(-8.88610136060078,-1.16276985666979,
22.9561993879088));
#15978=CARTESIAN_POINT('Ctrl Pts',(-9.13808834820213,-1.00235817476274,
22.9441962011194));
#15979=CARTESIAN_POINT('Ctrl Pts',(-9.39007533580348,-0.841946492855682,
22.9321930143301));
#15980=CARTESIAN_POINT('Ctrl Pts',(-9.57754329642207,-0.583102430601619,
22.9201898275408));
#15981=CARTESIAN_POINT('Ctrl Pts',(-9.65136659729226,-0.293655596344823,
22.9081866407515));
#15982=CARTESIAN_POINT('Ctrl Pts',(-9.67581103310564,-0.197813707971187,
22.904212135066));
#15983=CARTESIAN_POINT('Ctrl Pts',(-9.6882250000001,-0.0989100500911656,
22.9002376293806));
#15984=CARTESIAN_POINT('Ctrl Pts',(-9.688225,1.12065912105663E-12,22.8962631236951));
#15985=CARTESIAN_POINT('Ctrl Pts',(-9.688225,-5.96633853433559E-13,22.8537368763049));
#15986=CARTESIAN_POINT('Ctrl Pts',(-9.68822499999985,-0.298712821306679,
22.8657400630942));
#15987=CARTESIAN_POINT('Ctrl Pts',(-9.57054245632557,-0.595858078272044,
22.8777432498835));
#15988=CARTESIAN_POINT('Ctrl Pts',(-9.36601586214896,-0.813569405233129,
22.8897464366728));
#15989=CARTESIAN_POINT('Ctrl Pts',(-9.16148926797235,-1.03128073219422,
22.9017496234621));
#15990=CARTESIAN_POINT('Ctrl Pts',(-8.87226522412793,-1.16727314847152,
22.9137528102515));
#15991=CARTESIAN_POINT('Ctrl Pts',(-8.57413435701398,-1.18591009260193,
22.9257559970408));
#15992=CARTESIAN_POINT('Ctrl Pts',(-8.27600348990002,-1.20454703673234,
22.9377591838301));
#15993=CARTESIAN_POINT('Ctrl Pts',(-7.97209482032048,-1.10563290540087,
22.9497623706194));
#15994=CARTESIAN_POINT('Ctrl Pts',(-7.74204705372025,-0.915087963996274,
22.9617655574087));
#15995=CARTESIAN_POINT('Ctrl Pts',(-7.51199928712001,-0.724543022591673,
22.973768744198));
#15996=CARTESIAN_POINT('Ctrl Pts',(-7.35822688079618,-0.444367128061042,
22.9857719309874));
#15997=CARTESIAN_POINT('Ctrl Pts',(-7.32102560975812,-0.147979855989868,
22.9977751177767));
#15998=CARTESIAN_POINT('Ctrl Pts',(-7.28382433872006,0.148407416081306,
23.009778304566));
#15999=CARTESIAN_POINT('Ctrl Pts',(-7.36358464744652,0.457895344722344,
23.0217814913553));
#16000=CARTESIAN_POINT('Ctrl Pts',(-7.53940549437905,0.699383189958014,
23.0337846781446));
#16001=CARTESIAN_POINT('Ctrl Pts',(-7.71522634131158,0.940871035193684,
23.0457878649339));
#16002=CARTESIAN_POINT('Ctrl Pts',(-7.98526240565818,1.11182427083098,23.0577910517233));
#16003=CARTESIAN_POINT('Ctrl Pts',(-8.27875123560152,1.16744491727753,23.0697942385126));
#16004=CARTESIAN_POINT('Ctrl Pts',(-8.57224006554485,1.22306556372409,23.0817974253019));
#16005=CARTESIAN_POINT('Ctrl Pts',(-8.88610136059973,1.16276985667013,23.0938006120912));
#16006=CARTESIAN_POINT('Ctrl Pts',(-9.13808834820121,1.00235817476332,23.1058037988805));
#16007=CARTESIAN_POINT('Ctrl Pts',(-9.39007533580268,0.84194649285651,23.1178069856698));
#16008=CARTESIAN_POINT('Ctrl Pts',(-9.57754329642151,0.583102430602647,
23.1298101724592));
#16009=CARTESIAN_POINT('Ctrl Pts',(-9.65136659729198,0.293655596345944,
23.1418133592485));
#16010=CARTESIAN_POINT('Ctrl Pts',(-9.67581103310549,0.19781370797218,23.1457878649339));
#16011=CARTESIAN_POINT('Ctrl Pts',(-9.68822500000003,0.098910050092008,
23.1497623706194));
#16012=CARTESIAN_POINT('Ctrl Pts',(-9.688225,-4.35929070619068E-13,23.1537368763049));
#16013=CARTESIAN_POINT('Origin',(-8.5,0.,1.8));
#16014=CARTESIAN_POINT('',(-9.688225,1.17184040249185E-12,23.4962631236951));
#16015=CARTESIAN_POINT('',(-9.688225,-5.45341549695877E-13,23.4537368763049));
#16016=CARTESIAN_POINT('',(-9.688225,-1.45515594291686E-16,1.8));
#16017=CARTESIAN_POINT('Ctrl Pts',(-9.688225,1.23945298469152E-12,23.4962631236951));
#16018=CARTESIAN_POINT('Ctrl Pts',(-9.68822499999969,0.298712821307322,
23.4842599369058));
#16019=CARTESIAN_POINT('Ctrl Pts',(-9.57054245632525,0.595858078272623,
23.4722567501165));
#16020=CARTESIAN_POINT('Ctrl Pts',(-9.36601586214852,0.813569405233598,
23.4602535633272));
#16021=CARTESIAN_POINT('Ctrl Pts',(-9.1614892679718,1.03128073219457,23.4482503765379));
#16022=CARTESIAN_POINT('Ctrl Pts',(-8.8722652241273,1.16727314847172,23.4362471897485));
#16023=CARTESIAN_POINT('Ctrl Pts',(-8.57413435701333,1.18591009260197,23.4242440029592));
#16024=CARTESIAN_POINT('Ctrl Pts',(-8.27600348989937,1.20454703673222,23.4122408161699));
#16025=CARTESIAN_POINT('Ctrl Pts',(-7.97209482031989,1.10563290540059,23.4002376293806));
#16026=CARTESIAN_POINT('Ctrl Pts',(-7.74204705371975,0.915087963995864,
23.3882344425913));
#16027=CARTESIAN_POINT('Ctrl Pts',(-7.51199928711962,0.724543022591139,
23.376231255802));
#16028=CARTESIAN_POINT('Ctrl Pts',(-7.35822688079594,0.444367128060424,
23.3642280690126));
#16029=CARTESIAN_POINT('Ctrl Pts',(-7.32102560975804,0.14797985598923,23.3522248822233));
#16030=CARTESIAN_POINT('Ctrl Pts',(-7.28382433872014,-0.148407416081964,
23.340221695434));
#16031=CARTESIAN_POINT('Ctrl Pts',(-7.36358464744677,-0.457895344722959,
23.3282185086447));
#16032=CARTESIAN_POINT('Ctrl Pts',(-7.53940549437943,-0.699383189958534,
23.3162153218554));
#16033=CARTESIAN_POINT('Ctrl Pts',(-7.71522634131209,-0.940871035194109,
23.304212135066));
#16034=CARTESIAN_POINT('Ctrl Pts',(-7.98526240565878,-1.11182427083126,
23.2922089482767));
#16035=CARTESIAN_POINT('Ctrl Pts',(-8.27875123560215,-1.16744491727765,
23.2802057614874));
#16036=CARTESIAN_POINT('Ctrl Pts',(-8.57224006554551,-1.22306556372405,
23.2682025746981));
#16037=CARTESIAN_POINT('Ctrl Pts',(-8.88610136060036,-1.16276985666992,
23.2561993879088));
#16038=CARTESIAN_POINT('Ctrl Pts',(-9.13808834820175,-1.00235817476298,
23.2441962011195));
#16039=CARTESIAN_POINT('Ctrl Pts',(-9.39007533580314,-0.841946492856029,
23.2321930143301));
#16040=CARTESIAN_POINT('Ctrl Pts',(-9.57754329642182,-0.583102430602064,
23.2201898275408));
#16041=CARTESIAN_POINT('Ctrl Pts',(-9.65136659729214,-0.293655596345322,
23.2081866407515));
#16042=CARTESIAN_POINT('Ctrl Pts',(-9.6758110331056,-0.1978137079715,23.2042121350661));
#16043=CARTESIAN_POINT('Ctrl Pts',(-9.6882250000001,-0.098910050091275,
23.2002376293806));
#16044=CARTESIAN_POINT('Ctrl Pts',(-9.688225,1.21391785512515E-12,23.1962631236951));
#16045=CARTESIAN_POINT('Ctrl Pts',(-9.688225,-4.35929070619068E-13,23.1537368763049));
#16046=CARTESIAN_POINT('Ctrl Pts',(-9.68822499999989,-0.298712821306496,
23.1657400630942));
#16047=CARTESIAN_POINT('Ctrl Pts',(-9.57054245632567,-0.595858078271855,
23.1777432498835));
#16048=CARTESIAN_POINT('Ctrl Pts',(-9.36601586214912,-0.813569405232963,
23.1897464366728));
#16049=CARTESIAN_POINT('Ctrl Pts',(-9.16148926797257,-1.03128073219407,
23.2017496234621));
#16050=CARTESIAN_POINT('Ctrl Pts',(-8.8722652241282,-1.16727314847143,23.2137528102514));
#16051=CARTESIAN_POINT('Ctrl Pts',(-8.57413435701427,-1.18591009260191,
23.2257559970408));
#16052=CARTESIAN_POINT('Ctrl Pts',(-8.27600348990034,-1.2045470367324,23.2377591838301));
#16053=CARTESIAN_POINT('Ctrl Pts',(-7.97209482032081,-1.10563290540102,
23.2497623706194));
#16054=CARTESIAN_POINT('Ctrl Pts',(-7.74204705372053,-0.915087963996506,
23.2617655574087));
#16055=CARTESIAN_POINT('Ctrl Pts',(-7.51199928712025,-0.72454302259199,
23.273768744198));
#16056=CARTESIAN_POINT('Ctrl Pts',(-7.35822688079634,-0.444367128061434,
23.2857719309873));
#16057=CARTESIAN_POINT('Ctrl Pts',(-7.32102560975817,-0.147979855990296,
23.2977751177767));
#16058=CARTESIAN_POINT('Ctrl Pts',(-7.28382433872001,0.148407416080842,
23.309778304566));
#16059=CARTESIAN_POINT('Ctrl Pts',(-7.36358464744634,0.457895344721885,
23.3217814913553));
#16060=CARTESIAN_POINT('Ctrl Pts',(-7.53940549437876,0.699383189957611,
23.3337846781446));
#16061=CARTESIAN_POINT('Ctrl Pts',(-7.71522634131117,0.940871035193337,
23.3457878649339));
#16062=CARTESIAN_POINT('Ctrl Pts',(-7.98526240565768,1.11182427083074,23.3577910517232));
#16063=CARTESIAN_POINT('Ctrl Pts',(-8.27875123560096,1.16744491727743,23.3697942385126));
#16064=CARTESIAN_POINT('Ctrl Pts',(-8.57224006554425,1.22306556372412,23.3817974253019));
#16065=CARTESIAN_POINT('Ctrl Pts',(-8.88610136059913,1.16276985667033,23.3938006120912));
#16066=CARTESIAN_POINT('Ctrl Pts',(-9.13808834820067,1.00235817476366,23.4058037988805));
#16067=CARTESIAN_POINT('Ctrl Pts',(-9.39007533580222,0.841946492856997,
23.4178069856698));
#16068=CARTESIAN_POINT('Ctrl Pts',(-9.57754329642117,0.583102430603261,
23.4298101724591));
#16069=CARTESIAN_POINT('Ctrl Pts',(-9.6513665972918,0.293655596346624,23.4418133592485));
#16070=CARTESIAN_POINT('Ctrl Pts',(-9.67581103310543,0.197813707972634,
23.4457878649339));
#16071=CARTESIAN_POINT('Ctrl Pts',(-9.68822500000004,0.0989100500922138,
23.4497623706194));
#16072=CARTESIAN_POINT('Ctrl Pts',(-9.688225,-4.77784478647436E-13,23.4537368763049));
#16073=CARTESIAN_POINT('Origin',(-8.5,0.,1.8));
#16074=CARTESIAN_POINT('',(-9.688225,1.19748655436069E-12,23.7962631236951));
#16075=CARTESIAN_POINT('',(-9.688225,-5.19806420129498E-13,23.7537368763049));
#16076=CARTESIAN_POINT('',(-9.688225,-1.45515594291686E-16,1.8));
#16077=CARTESIAN_POINT('Ctrl Pts',(-9.688225,1.33260069645758E-12,23.7962631236951));
#16078=CARTESIAN_POINT('Ctrl Pts',(-9.68822499999967,0.298712821307437,
23.7842599369058));
#16079=CARTESIAN_POINT('Ctrl Pts',(-9.57054245632518,0.595858078272752,
23.7722567501165));
#16080=CARTESIAN_POINT('Ctrl Pts',(-9.36601586214841,0.813569405233715,
23.7602535633272));
#16081=CARTESIAN_POINT('Ctrl Pts',(-9.16148926797164,1.03128073219468,23.7482503765379));
#16082=CARTESIAN_POINT('Ctrl Pts',(-8.8722652241271,1.16727314847179,23.7362471897485));
#16083=CARTESIAN_POINT('Ctrl Pts',(-8.57413435701311,1.18591009260199,23.7242440029592));
#16084=CARTESIAN_POINT('Ctrl Pts',(-8.27600348989911,1.20454703673218,23.7122408161699));
#16085=CARTESIAN_POINT('Ctrl Pts',(-7.97209482031963,1.10563290540047,23.7002376293806));
#16086=CARTESIAN_POINT('Ctrl Pts',(-7.74204705371953,0.915087963995675,
23.6882344425913));
#16087=CARTESIAN_POINT('Ctrl Pts',(-7.51199928711942,0.724543022590878,
23.6762312558019));
#16088=CARTESIAN_POINT('Ctrl Pts',(-7.35822688079581,0.444367128060098,
23.6642280690126));
#16089=CARTESIAN_POINT('Ctrl Pts',(-7.32102560975799,0.14797985598887,23.6522248822233));
#16090=CARTESIAN_POINT('Ctrl Pts',(-7.28382433872018,-0.148407416082358,
23.640221695434));
#16091=CARTESIAN_POINT('Ctrl Pts',(-7.36358464744692,-0.457895344723353,
23.6282185086447));
#16092=CARTESIAN_POINT('Ctrl Pts',(-7.53940549437968,-0.699383189958882,
23.6162153218553));
#16093=CARTESIAN_POINT('Ctrl Pts',(-7.71522634131245,-0.940871035194412,
23.604212135066));
#16094=CARTESIAN_POINT('Ctrl Pts',(-7.98526240565923,-1.11182427083147,
23.5922089482767));
#16095=CARTESIAN_POINT('Ctrl Pts',(-8.27875123560264,-1.16744491727775,
23.5802057614874));
#16096=CARTESIAN_POINT('Ctrl Pts',(-8.57224006554605,-1.22306556372402,
23.5682025746981));
#16097=CARTESIAN_POINT('Ctrl Pts',(-8.88610136060089,-1.16276985666975,
23.5561993879088));
#16098=CARTESIAN_POINT('Ctrl Pts',(-9.13808834820223,-1.00235817476267,
23.5441962011194));
#16099=CARTESIAN_POINT('Ctrl Pts',(-9.39007533580356,-0.841946492855593,
23.5321930143301));
#16100=CARTESIAN_POINT('Ctrl Pts',(-9.57754329642213,-0.583102430601512,
23.5201898275408));
#16101=CARTESIAN_POINT('Ctrl Pts',(-9.65136659729229,-0.293655596344708,
23.5081866407515));
#16102=CARTESIAN_POINT('Ctrl Pts',(-9.67581103310566,-0.19781370797107,
23.504212135066));
#16103=CARTESIAN_POINT('Ctrl Pts',(-9.6882250000001,-0.0989100500910468,
23.5002376293806));
#16104=CARTESIAN_POINT('Ctrl Pts',(-9.688225,1.23945298469152E-12,23.4962631236951));
#16105=CARTESIAN_POINT('Ctrl Pts',(-9.688225,-4.77784478647436E-13,23.4537368763049));
#16106=CARTESIAN_POINT('Ctrl Pts',(-9.68822499999988,-0.298712821306605,
23.4657400630942));
#16107=CARTESIAN_POINT('Ctrl Pts',(-9.57054245632559,-0.595858078272026,
23.4777432498835));
#16108=CARTESIAN_POINT('Ctrl Pts',(-9.36601586214895,-0.813569405233141,
23.4897464366728));
#16109=CARTESIAN_POINT('Ctrl Pts',(-9.16148926797231,-1.03128073219426,
23.5017496234621));
#16110=CARTESIAN_POINT('Ctrl Pts',(-8.87226522412783,-1.16727314847157,
23.5137528102515));
#16111=CARTESIAN_POINT('Ctrl Pts',(-8.57413435701383,-1.18591009260194,
23.5257559970408));
#16112=CARTESIAN_POINT('Ctrl Pts',(-8.27600348989982,-1.20454703673232,
23.5377591838301));
#16113=CARTESIAN_POINT('Ctrl Pts',(-7.97209482032025,-1.10563290540078,
23.5497623706194));
#16114=CARTESIAN_POINT('Ctrl Pts',(-7.74204705372003,-0.915087963996091,
23.5617655574087));
#16115=CARTESIAN_POINT('Ctrl Pts',(-7.5119992871198,-0.724543022591406,
23.5737687441981));
#16116=CARTESIAN_POINT('Ctrl Pts',(-7.35822688079603,-0.444367128060682,
23.5857719309874));
#16117=CARTESIAN_POINT('Ctrl Pts',(-7.32102560975807,-0.14797985598945,
23.5977751177767));
#16118=CARTESIAN_POINT('Ctrl Pts',(-7.2838243387201,0.148407416081782,23.609778304566));
#16119=CARTESIAN_POINT('Ctrl Pts',(-7.36358464744671,0.45789534472284,23.6217814913553));
#16120=CARTESIAN_POINT('Ctrl Pts',(-7.53940549437938,0.699383189958464,
23.6337846781447));
#16121=CARTESIAN_POINT('Ctrl Pts',(-7.71522634131205,0.940871035194088,
23.645787864934));
#16122=CARTESIAN_POINT('Ctrl Pts',(-7.98526240565879,1.11182427083127,23.6577910517233));
#16123=CARTESIAN_POINT('Ctrl Pts',(-8.2787512356022,1.16744491727766,23.6697942385126));
#16124=CARTESIAN_POINT('Ctrl Pts',(-8.57224006554561,1.22306556372405,23.6817974253019));
#16125=CARTESIAN_POINT('Ctrl Pts',(-8.8861013606005,1.16276985666989,23.6938006120912));
#16126=CARTESIAN_POINT('Ctrl Pts',(-9.1380883482019,1.00235817476288,23.7058037988806));
#16127=CARTESIAN_POINT('Ctrl Pts',(-9.39007533580331,0.841946492855867,
23.7178069856699));
#16128=CARTESIAN_POINT('Ctrl Pts',(-9.57754329642197,0.583102430601818,
23.7298101724592));
#16129=CARTESIAN_POINT('Ctrl Pts',(-9.65136659729222,0.293655596345012,
23.7418133592485));
#16130=CARTESIAN_POINT('Ctrl Pts',(-9.67581103310558,0.19781370797149,23.745787864934));
#16131=CARTESIAN_POINT('Ctrl Pts',(-9.68822500000005,0.0989100500915865,
23.7497623706194));
#16132=CARTESIAN_POINT('Ctrl Pts',(-9.688225,-5.87252468875477E-13,23.7537368763049));
#16133=CARTESIAN_POINT('Origin',(-8.5,0.,1.8));
#16134=CARTESIAN_POINT('',(-9.688225,1.223243728532E-12,24.0962631236951));
#16135=CARTESIAN_POINT('',(-9.688225,-4.94104757109426E-13,24.0537368763049));
#16136=CARTESIAN_POINT('',(-9.688225,-1.45515594291686E-16,1.8));
#16137=CARTESIAN_POINT('Ctrl Pts',(-9.688225,1.223243728532E-12,24.0962631236951));
#16138=CARTESIAN_POINT('Ctrl Pts',(-9.68822499999969,0.298712821307283,
24.0842599369058));
#16139=CARTESIAN_POINT('Ctrl Pts',(-9.57054245632528,0.595858078272564,
24.0722567501165));
#16140=CARTESIAN_POINT('Ctrl Pts',(-9.36601586214858,0.813569405233537,
24.0602535633272));
#16141=CARTESIAN_POINT('Ctrl Pts',(-9.16148926797189,1.03128073219451,24.0482503765379));
#16142=CARTESIAN_POINT('Ctrl Pts',(-8.87226522412743,1.16727314847168,24.0362471897486));
#16143=CARTESIAN_POINT('Ctrl Pts',(-8.57413435701348,1.18591009260196,24.0242440029592));
#16144=CARTESIAN_POINT('Ctrl Pts',(-8.27600348989954,1.20454703673225,24.0122408161699));
#16145=CARTESIAN_POINT('Ctrl Pts',(-7.97209482032007,1.10563290540067,24.0002376293806));
#16146=CARTESIAN_POINT('Ctrl Pts',(-7.74204705371992,0.915087963996004,
23.9882344425913));
#16147=CARTESIAN_POINT('Ctrl Pts',(-7.51199928711977,0.724543022591335,
23.976231255802));
#16148=CARTESIAN_POINT('Ctrl Pts',(-7.35822688079604,0.444367128060677,
23.9642280690127));
#16149=CARTESIAN_POINT('Ctrl Pts',(-7.32102560975807,0.147979855989515,
23.9522248822233));
#16150=CARTESIAN_POINT('Ctrl Pts',(-7.2838243387201,-0.148407416081648,
23.940221695434));
#16151=CARTESIAN_POINT('Ctrl Pts',(-7.36358464744665,-0.457895344722638,
23.9282185086447));
#16152=CARTESIAN_POINT('Ctrl Pts',(-7.53940549437922,-0.699383189958248,
23.9162153218554));
#16153=CARTESIAN_POINT('Ctrl Pts',(-7.7152263413118,-0.940871035193857,
23.9042121350661));
#16154=CARTESIAN_POINT('Ctrl Pts',(-7.98526240565841,-1.11182427083108,
23.8922089482768));
#16155=CARTESIAN_POINT('Ctrl Pts',(-8.27875123560173,-1.16744491727757,
23.8802057614874));
#16156=CARTESIAN_POINT('Ctrl Pts',(-8.57224006554505,-1.22306556372407,
23.8682025746981));
#16157=CARTESIAN_POINT('Ctrl Pts',(-8.8861013605999,-1.16276985667007,23.8561993879088));
#16158=CARTESIAN_POINT('Ctrl Pts',(-9.13808834820134,-1.00235817476324,
23.8441962011195));
#16159=CARTESIAN_POINT('Ctrl Pts',(-9.39007533580278,-0.841946492856407,
23.8321930143302));
#16160=CARTESIAN_POINT('Ctrl Pts',(-9.57754329642155,-0.583102430602547,
23.8201898275409));
#16161=CARTESIAN_POINT('Ctrl Pts',(-9.651366597292,-0.293655596345861,23.8081866407515));
#16162=CARTESIAN_POINT('Ctrl Pts',(-9.67581103310557,-0.197813707971833,
23.8042121350661));
#16163=CARTESIAN_POINT('Ctrl Pts',(-9.68822500000011,-0.0989100500913815,
23.8002376293806));
#16164=CARTESIAN_POINT('Ctrl Pts',(-9.688225,1.33260069645758E-12,23.7962631236951));
#16165=CARTESIAN_POINT('Ctrl Pts',(-9.688225,-5.87252468875477E-13,23.7537368763049));
#16166=CARTESIAN_POINT('Ctrl Pts',(-9.68822499999985,-0.298712821306647,
23.7657400630942));
#16167=CARTESIAN_POINT('Ctrl Pts',(-9.57054245632559,-0.595858078271991,
23.7777432498835));
#16168=CARTESIAN_POINT('Ctrl Pts',(-9.36601586214902,-0.813569405233074,
23.7897464366728));
#16169=CARTESIAN_POINT('Ctrl Pts',(-9.16148926797244,-1.03128073219416,
23.8017496234621));
#16170=CARTESIAN_POINT('Ctrl Pts',(-8.87226522412805,-1.16727314847148,
23.8137528102514));
#16171=CARTESIAN_POINT('Ctrl Pts',(-8.57413435701412,-1.18591009260192,
23.8257559970408));
#16172=CARTESIAN_POINT('Ctrl Pts',(-8.27600348990019,-1.20454703673237,
23.8377591838301));
#16173=CARTESIAN_POINT('Ctrl Pts',(-7.97209482032066,-1.10563290540095,
23.8497623706194));
#16174=CARTESIAN_POINT('Ctrl Pts',(-7.74204705372041,-0.915087963996409,
23.8617655574087));
#16175=CARTESIAN_POINT('Ctrl Pts',(-7.51199928712016,-0.724543022591864,
23.873768744198));
#16176=CARTESIAN_POINT('Ctrl Pts',(-7.35822688079628,-0.444367128061288,
23.8857719309873));
#16177=CARTESIAN_POINT('Ctrl Pts',(-7.32102560975815,-0.147979855990145,
23.8977751177767));
#16178=CARTESIAN_POINT('Ctrl Pts',(-7.28382433872002,0.148407416080997,
23.909778304566));
#16179=CARTESIAN_POINT('Ctrl Pts',(-7.3635846474464,0.45789534472203,23.9217814913553));
#16180=CARTESIAN_POINT('Ctrl Pts',(-7.53940549437885,0.699383189957734,
23.9337846781446));
#16181=CARTESIAN_POINT('Ctrl Pts',(-7.7152263413113,0.940871035193437,23.9457878649339));
#16182=CARTESIAN_POINT('Ctrl Pts',(-7.98526240565782,1.1118242708308,23.9577910517232));
#16183=CARTESIAN_POINT('Ctrl Pts',(-8.27875123560111,1.16744491727746,23.9697942385126));
#16184=CARTESIAN_POINT('Ctrl Pts',(-8.5722400655444,1.22306556372411,23.9817974253019));
#16185=CARTESIAN_POINT('Ctrl Pts',(-8.88610136059927,1.16276985667028,23.9938006120912));
#16186=CARTESIAN_POINT('Ctrl Pts',(-9.1380883482008,1.00235817476358,24.0058037988805));
#16187=CARTESIAN_POINT('Ctrl Pts',(-9.39007533580232,0.841946492856883,
24.0178069856698));
#16188=CARTESIAN_POINT('Ctrl Pts',(-9.57754329642124,0.583102430603124,
24.0298101724591));
#16189=CARTESIAN_POINT('Ctrl Pts',(-9.65136659729184,0.293655596346477,
24.0418133592485));
#16190=CARTESIAN_POINT('Ctrl Pts',(-9.67581103310544,0.197813707972528,
24.0457878649339));
#16191=CARTESIAN_POINT('Ctrl Pts',(-9.68822500000004,0.0989100500921524,
24.0497623706194));
#16192=CARTESIAN_POINT('Ctrl Pts',(-9.688225,-4.94104757109426E-13,24.0537368763049));
#16193=CARTESIAN_POINT('Origin',(-8.5,0.,1.8));
#16194=CARTESIAN_POINT('',(-9.688225,1.24877885809838E-12,24.3962631236951));
#16195=CARTESIAN_POINT('',(-9.688225,-4.68514116391816E-13,24.3537368763049));
#16196=CARTESIAN_POINT('',(-9.688225,-1.45515594291686E-16,1.8));
#16197=CARTESIAN_POINT('Ctrl Pts',(-9.688225,1.1811662758987E-12,24.3962631236951));
#16198=CARTESIAN_POINT('Ctrl Pts',(-9.6882249999997,0.298712821307263,24.3842599369058));
#16199=CARTESIAN_POINT('Ctrl Pts',(-9.57054245632528,0.595858078272571,
24.3722567501165));
#16200=CARTESIAN_POINT('Ctrl Pts',(-9.36601586214856,0.813569405233556,
24.3602535633272));
#16201=CARTESIAN_POINT('Ctrl Pts',(-9.16148926797185,1.03128073219454,24.3482503765379));
#16202=CARTESIAN_POINT('Ctrl Pts',(-8.87226522412736,1.16727314847171,24.3362471897485));
#16203=CARTESIAN_POINT('Ctrl Pts',(-8.57413435701339,1.18591009260197,24.3242440029592));
#16204=CARTESIAN_POINT('Ctrl Pts',(-8.27600348989943,1.20454703673223,24.3122408161699));
#16205=CARTESIAN_POINT('Ctrl Pts',(-7.97209482031994,1.10563290540062,24.3002376293806));
#16206=CARTESIAN_POINT('Ctrl Pts',(-7.7420470537198,0.915087963995901,24.2882344425913));
#16207=CARTESIAN_POINT('Ctrl Pts',(-7.51199928711966,0.724543022591188,
24.276231255802));
#16208=CARTESIAN_POINT('Ctrl Pts',(-7.35822688079596,0.44436712806048,24.2642280690126));
#16209=CARTESIAN_POINT('Ctrl Pts',(-7.32102560975804,0.147979855989288,
24.2522248822233));
#16210=CARTESIAN_POINT('Ctrl Pts',(-7.28382433872013,-0.148407416081904,
24.240221695434));
#16211=CARTESIAN_POINT('Ctrl Pts',(-7.36358464744675,-0.457895344722903,
24.2282185086447));
#16212=CARTESIAN_POINT('Ctrl Pts',(-7.5394054943794,-0.699383189958487,
24.2162153218554));
#16213=CARTESIAN_POINT('Ctrl Pts',(-7.71522634131205,-0.940871035194071,
24.2042121350661));
#16214=CARTESIAN_POINT('Ctrl Pts',(-7.98526240565873,-1.11182427083123,
24.1922089482767));
#16215=CARTESIAN_POINT('Ctrl Pts',(-8.27875123560209,-1.16744491727764,
24.1802057614874));
#16216=CARTESIAN_POINT('Ctrl Pts',(-8.57224006554545,-1.22306556372405,
24.1682025746981));
#16217=CARTESIAN_POINT('Ctrl Pts',(-8.8861013606003,-1.16276985666994,24.1561993879088));
#16218=CARTESIAN_POINT('Ctrl Pts',(-9.1380883482017,-1.00235817476301,24.1441962011195));
#16219=CARTESIAN_POINT('Ctrl Pts',(-9.3900753358031,-0.841946492856072,
24.1321930143301));
#16220=CARTESIAN_POINT('Ctrl Pts',(-9.57754329642179,-0.583102430602117,
24.1201898275408));
#16221=CARTESIAN_POINT('Ctrl Pts',(-9.65136659729212,-0.293655596345378,
24.1081866407515));
#16222=CARTESIAN_POINT('Ctrl Pts',(-9.6758110331056,-0.197813707971536,
24.1042121350661));
#16223=CARTESIAN_POINT('Ctrl Pts',(-9.6882250000001,-0.0989100500912883,
24.1002376293806));
#16224=CARTESIAN_POINT('Ctrl Pts',(-9.688225,1.223243728532E-12,24.0962631236951));
#16225=CARTESIAN_POINT('Ctrl Pts',(-9.688225,-4.94104757109426E-13,24.0537368763049));
#16226=CARTESIAN_POINT('Ctrl Pts',(-9.68822499999987,-0.298712821306554,
24.0657400630942));
#16227=CARTESIAN_POINT('Ctrl Pts',(-9.57054245632564,-0.595858078271907,
24.0777432498835));
#16228=CARTESIAN_POINT('Ctrl Pts',(-9.36601586214908,-0.813569405233006,
24.0897464366728));
#16229=CARTESIAN_POINT('Ctrl Pts',(-9.16148926797252,-1.0312807321941,24.1017496234621));
#16230=CARTESIAN_POINT('Ctrl Pts',(-8.87226522412814,-1.16727314847145,
24.1137528102514));
#16231=CARTESIAN_POINT('Ctrl Pts',(-8.57413435701421,-1.18591009260192,
24.1257559970408));
#16232=CARTESIAN_POINT('Ctrl Pts',(-8.27600348990028,-1.20454703673239,
24.1377591838301));
#16233=CARTESIAN_POINT('Ctrl Pts',(-7.97209482032075,-1.105632905401,24.1497623706194));
#16234=CARTESIAN_POINT('Ctrl Pts',(-7.74204705372048,-0.915087963996469,
24.1617655574087));
#16235=CARTESIAN_POINT('Ctrl Pts',(-7.51199928712022,-0.724543022591941,
24.173768744198));
#16236=CARTESIAN_POINT('Ctrl Pts',(-7.35822688079632,-0.444367128061378,
24.1857719309873));
#16237=CARTESIAN_POINT('Ctrl Pts',(-7.32102560975816,-0.147979855990238,
24.1977751177767));
#16238=CARTESIAN_POINT('Ctrl Pts',(-7.28382433872001,0.148407416080902,
24.209778304566));
#16239=CARTESIAN_POINT('Ctrl Pts',(-7.36358464744637,0.457895344721941,
24.2217814913553));
#16240=CARTESIAN_POINT('Ctrl Pts',(-7.53940549437879,0.699383189957658,
24.2337846781446));
#16241=CARTESIAN_POINT('Ctrl Pts',(-7.71522634131122,0.940871035193376,
24.2457878649339));
#16242=CARTESIAN_POINT('Ctrl Pts',(-7.98526240565773,1.11182427083076,24.2577910517232));
#16243=CARTESIAN_POINT('Ctrl Pts',(-8.27875123560102,1.16744491727744,24.2697942385126));
#16244=CARTESIAN_POINT('Ctrl Pts',(-8.5722400655443,1.22306556372411,24.2817974253019));
#16245=CARTESIAN_POINT('Ctrl Pts',(-8.88610136059918,1.16276985667031,24.2938006120912));
#16246=CARTESIAN_POINT('Ctrl Pts',(-9.13808834820072,1.00235817476363,24.3058037988805));
#16247=CARTESIAN_POINT('Ctrl Pts',(-9.39007533580226,0.841946492856953,
24.3178069856698));
#16248=CARTESIAN_POINT('Ctrl Pts',(-9.5775432964212,0.583102430603208,24.3298101724591));
#16249=CARTESIAN_POINT('Ctrl Pts',(-9.65136659729182,0.293655596346567,
24.3418133592485));
#16250=CARTESIAN_POINT('Ctrl Pts',(-9.67581103310543,0.197813707972598,
24.3457878649339));
#16251=CARTESIAN_POINT('Ctrl Pts',(-9.68822500000004,0.0989100500922005,
24.3497623706194));
#16252=CARTESIAN_POINT('Ctrl Pts',(-9.688225,-4.68514116391816E-13,24.3537368763049));
#16253=CARTESIAN_POINT('Origin',(-8.5,0.,1.8));
#16254=CARTESIAN_POINT('',(-9.688225,1.27431398766475E-12,24.6962631236951));
#16255=CARTESIAN_POINT('',(-9.688225,-4.42923475674206E-13,24.6537368763049));
#16256=CARTESIAN_POINT('',(-9.688225,-1.45515594291686E-16,1.8));
#16257=CARTESIAN_POINT('Ctrl Pts',(-9.688225,1.27431398766475E-12,24.6962631236951));
#16258=CARTESIAN_POINT('Ctrl Pts',(-9.68822499999968,0.298712821307379,
24.6842599369058));
#16259=CARTESIAN_POINT('Ctrl Pts',(-9.57054245632521,0.595858078272699,
24.6722567501165));
#16260=CARTESIAN_POINT('Ctrl Pts',(-9.36601586214845,0.813569405233673,
24.6602535633272));
#16261=CARTESIAN_POINT('Ctrl Pts',(-9.16148926797169,1.03128073219465,24.6482503765379));
#16262=CARTESIAN_POINT('Ctrl Pts',(-8.87226522412716,1.16727314847178,24.6362471897485));
#16263=CARTESIAN_POINT('Ctrl Pts',(-8.57413435701316,1.18591009260198,24.6242440029592));
#16264=CARTESIAN_POINT('Ctrl Pts',(-8.27600348989917,1.20454703673219,24.6122408161699));
#16265=CARTESIAN_POINT('Ctrl Pts',(-7.97209482031968,1.1056329054005,24.6002376293806));
#16266=CARTESIAN_POINT('Ctrl Pts',(-7.74204705371957,0.915087963995712,
24.5882344425913));
#16267=CARTESIAN_POINT('Ctrl Pts',(-7.51199928711946,0.724543022590927,
24.5762312558019));
#16268=CARTESIAN_POINT('Ctrl Pts',(-7.35822688079583,0.444367128060154,
24.5642280690126));
#16269=CARTESIAN_POINT('Ctrl Pts',(-7.321025609758,0.147979855988928,24.5522248822233));
#16270=CARTESIAN_POINT('Ctrl Pts',(-7.28382433872017,-0.148407416082298,
24.540221695434));
#16271=CARTESIAN_POINT('Ctrl Pts',(-7.3635846474469,-0.457895344723297,
24.5282185086447));
#16272=CARTESIAN_POINT('Ctrl Pts',(-7.53940549437965,-0.699383189958835,
24.5162153218554));
#16273=CARTESIAN_POINT('Ctrl Pts',(-7.7152263413124,-0.940871035194374,
24.504212135066));
#16274=CARTESIAN_POINT('Ctrl Pts',(-7.98526240565917,-1.11182427083144,
24.4922089482767));
#16275=CARTESIAN_POINT('Ctrl Pts',(-8.27875123560258,-1.16744491727773,
24.4802057614874));
#16276=CARTESIAN_POINT('Ctrl Pts',(-8.57224006554599,-1.22306556372402,
24.4682025746981));
#16277=CARTESIAN_POINT('Ctrl Pts',(-8.88610136060084,-1.16276985666977,
24.4561993879088));
#16278=CARTESIAN_POINT('Ctrl Pts',(-9.13808834820218,-1.0023581747627,24.4441962011194));
#16279=CARTESIAN_POINT('Ctrl Pts',(-9.39007533580352,-0.841946492855636,
24.4321930143301));
#16280=CARTESIAN_POINT('Ctrl Pts',(-9.5775432964221,-0.583102430601564,
24.4201898275408));
#16281=CARTESIAN_POINT('Ctrl Pts',(-9.65136659729228,-0.293655596344764,
24.4081866407515));
#16282=CARTESIAN_POINT('Ctrl Pts',(-9.67581103310565,-0.197813707971127,
24.404212135066));
#16283=CARTESIAN_POINT('Ctrl Pts',(-9.6882250000001,-0.0989100500911051,
24.4002376293806));
#16284=CARTESIAN_POINT('Ctrl Pts',(-9.688225,1.1811662758987E-12,24.3962631236951));
#16285=CARTESIAN_POINT('Ctrl Pts',(-9.688225,-4.68514116391816E-13,24.3537368763049));
#16286=CARTESIAN_POINT('Ctrl Pts',(-9.68822499999988,-0.298712821306551,
24.3657400630942));
#16287=CARTESIAN_POINT('Ctrl Pts',(-9.57054245632564,-0.595858078271928,
24.3777432498835));
#16288=CARTESIAN_POINT('Ctrl Pts',(-9.36601586214905,-0.813569405233036,
24.3897464366728));
#16289=CARTESIAN_POINT('Ctrl Pts',(-9.16148926797247,-1.03128073219414,
24.4017496234621));
#16290=CARTESIAN_POINT('Ctrl Pts',(-8.87226522412806,-1.16727314847148,
24.4137528102514));
#16291=CARTESIAN_POINT('Ctrl Pts',(-8.5741343570141,-1.18591009260192,24.4257559970408));
#16292=CARTESIAN_POINT('Ctrl Pts',(-8.27600348990015,-1.20454703673237,
24.4377591838301));
#16293=CARTESIAN_POINT('Ctrl Pts',(-7.97209482032061,-1.10563290540093,
24.4497623706194));
#16294=CARTESIAN_POINT('Ctrl Pts',(-7.74204705372035,-0.915087963996356,
24.4617655574087));
#16295=CARTESIAN_POINT('Ctrl Pts',(-7.51199928712009,-0.72454302259178,
24.473768744198));
#16296=CARTESIAN_POINT('Ctrl Pts',(-7.35822688079623,-0.444367128061165,
24.4857719309874));
#16297=CARTESIAN_POINT('Ctrl Pts',(-7.32102560975813,-0.147979855989995,
24.4977751177767));
#16298=CARTESIAN_POINT('Ctrl Pts',(-7.28382433872004,0.148407416081174,
24.509778304566));
#16299=CARTESIAN_POINT('Ctrl Pts',(-7.36358464744647,0.457895344722221,
24.5217814913553));
#16300=CARTESIAN_POINT('Ctrl Pts',(-7.53940549437898,0.699383189957911,
24.5337846781446));
#16301=CARTESIAN_POINT('Ctrl Pts',(-7.71522634131148,0.9408710351936,24.5457878649339));
#16302=CARTESIAN_POINT('Ctrl Pts',(-7.98526240565806,1.11182427083092,24.5577910517233));
#16303=CARTESIAN_POINT('Ctrl Pts',(-8.27875123560139,1.16744491727751,24.5697942385126));
#16304=CARTESIAN_POINT('Ctrl Pts',(-8.57224006554472,1.22306556372409,24.5817974253019));
#16305=CARTESIAN_POINT('Ctrl Pts',(-8.8861013605996,1.16276985667017,24.5938006120912));
#16306=CARTESIAN_POINT('Ctrl Pts',(-9.1380883482011,1.00235817476339,24.6058037988805));
#16307=CARTESIAN_POINT('Ctrl Pts',(-9.39007533580259,0.841946492856606,
24.6178069856698));
#16308=CARTESIAN_POINT('Ctrl Pts',(-9.57754329642144,0.583102430602763,
24.6298101724592));
#16309=CARTESIAN_POINT('Ctrl Pts',(-9.65136659729195,0.293655596346069,
24.6418133592485));
#16310=CARTESIAN_POINT('Ctrl Pts',(-9.67581103310547,0.197813707972285,
24.6457878649339));
#16311=CARTESIAN_POINT('Ctrl Pts',(-9.68822500000003,0.0989100500920911,
24.6497623706194));
#16312=CARTESIAN_POINT('Ctrl Pts',(-9.688225,-3.75310893474534E-13,24.6537368763049));
#16313=CARTESIAN_POINT('Origin',(-8.5,0.,1.8));
#16314=CARTESIAN_POINT('',(-9.68868882774917,0.000480291784193624,24.9962631236951));
#16315=CARTESIAN_POINT('',(-9.688225,-4.17277323805365E-13,24.9537368763049));
#16316=CARTESIAN_POINT('',(-9.688225,-1.45515594291686E-16,1.8));
#16317=CARTESIAN_POINT('Ctrl Pts',(-9.688225,1.2999601395336E-12,24.9962631236951));
#16318=CARTESIAN_POINT('Ctrl Pts',(-9.68822499999967,0.298712821307405,
24.9842599369058));
#16319=CARTESIAN_POINT('Ctrl Pts',(-9.5705424563252,0.595858078272722,24.9722567501165));
#16320=CARTESIAN_POINT('Ctrl Pts',(-9.36601586214844,0.813569405233692,
24.9602535633272));
#16321=CARTESIAN_POINT('Ctrl Pts',(-9.16148926797167,1.03128073219466,24.9482503765379));
#16322=CARTESIAN_POINT('Ctrl Pts',(-8.87226522412713,1.16727314847178,24.9362471897485));
#16323=CARTESIAN_POINT('Ctrl Pts',(-8.57413435701314,1.18591009260199,24.9242440029592));
#16324=CARTESIAN_POINT('Ctrl Pts',(-8.27600348989915,1.20454703673219,24.9122408161699));
#16325=CARTESIAN_POINT('Ctrl Pts',(-7.97209482031966,1.10563290540049,24.9002376293806));
#16326=CARTESIAN_POINT('Ctrl Pts',(-7.74204705371955,0.915087963995696,
24.8882344425913));
#16327=CARTESIAN_POINT('Ctrl Pts',(-7.51199928711944,0.724543022590906,
24.8762312558019));
#16328=CARTESIAN_POINT('Ctrl Pts',(-7.35822688079582,0.444367128060129,
24.8642280690126));
#16329=CARTESIAN_POINT('Ctrl Pts',(-7.321025609758,0.147979855988902,24.8522248822233));
#16330=CARTESIAN_POINT('Ctrl Pts',(-7.28382433872017,-0.148407416082324,
24.840221695434));
#16331=CARTESIAN_POINT('Ctrl Pts',(-7.36358464744691,-0.457895344723321,
24.8282185086447));
#16332=CARTESIAN_POINT('Ctrl Pts',(-7.53940549437966,-0.699383189958856,
24.8162153218554));
#16333=CARTESIAN_POINT('Ctrl Pts',(-7.71522634131242,-0.940871035194391,
24.804212135066));
#16334=CARTESIAN_POINT('Ctrl Pts',(-7.9852624056592,-1.11182427083146,24.7922089482767));
#16335=CARTESIAN_POINT('Ctrl Pts',(-8.27875123560261,-1.16744491727774,
24.7802057614874));
#16336=CARTESIAN_POINT('Ctrl Pts',(-8.57224006554601,-1.22306556372402,
24.7682025746981));
#16337=CARTESIAN_POINT('Ctrl Pts',(-8.88610136060086,-1.16276985666976,
24.7561993879088));
#16338=CARTESIAN_POINT('Ctrl Pts',(-9.1380883482022,-1.00235817476269,24.7441962011194));
#16339=CARTESIAN_POINT('Ctrl Pts',(-9.39007533580354,-0.841946492855617,
24.7321930143301));
#16340=CARTESIAN_POINT('Ctrl Pts',(-9.57754329642211,-0.583102430601541,
24.7201898275408));
#16341=CARTESIAN_POINT('Ctrl Pts',(-9.65136659729229,-0.293655596344739,
24.7081866407515));
#16342=CARTESIAN_POINT('Ctrl Pts',(-9.67581103310566,-0.19781370797108,
24.704212135066));
#16343=CARTESIAN_POINT('Ctrl Pts',(-9.68822500000011,-0.0989100500910345,
24.7002376293806));
#16344=CARTESIAN_POINT('Ctrl Pts',(-9.688225,1.27431398766475E-12,24.6962631236951));
#16345=CARTESIAN_POINT('Ctrl Pts',(-9.688225,-3.75310893474534E-13,24.6537368763049));
#16346=CARTESIAN_POINT('Ctrl Pts',(-9.68822499999991,-0.298712821306457,
24.6657400630942));
#16347=CARTESIAN_POINT('Ctrl Pts',(-9.57054245632568,-0.595858078271845,
24.6777432498835));
#16348=CARTESIAN_POINT('Ctrl Pts',(-9.36601586214912,-0.813569405232968,
24.6897464366728));
#16349=CARTESIAN_POINT('Ctrl Pts',(-9.16148926797255,-1.03128073219409,
24.7017496234621));
#16350=CARTESIAN_POINT('Ctrl Pts',(-8.87226522412815,-1.16727314847145,
24.7137528102514));
#16351=CARTESIAN_POINT('Ctrl Pts',(-8.5741343570142,-1.18591009260192,24.7257559970408));
#16352=CARTESIAN_POINT('Ctrl Pts',(-8.27600348990024,-1.20454703673238,
24.7377591838301));
#16353=CARTESIAN_POINT('Ctrl Pts',(-7.97209482032069,-1.10563290540097,
24.7497623706194));
#16354=CARTESIAN_POINT('Ctrl Pts',(-7.74204705372042,-0.915087963996415,
24.7617655574087));
#16355=CARTESIAN_POINT('Ctrl Pts',(-7.51199928712015,-0.724543022591857,
24.773768744198));
#16356=CARTESIAN_POINT('Ctrl Pts',(-7.35822688079626,-0.444367128061255,
24.7857719309873));
#16357=CARTESIAN_POINT('Ctrl Pts',(-7.32102560975814,-0.147979855990088,
24.7977751177767));
#16358=CARTESIAN_POINT('Ctrl Pts',(-7.28382433872003,0.148407416081079,
24.809778304566));
#16359=CARTESIAN_POINT('Ctrl Pts',(-7.36358464744644,0.457895344722132,
24.8217814913553));
#16360=CARTESIAN_POINT('Ctrl Pts',(-7.53940549437892,0.699383189957835,
24.8337846781446));
#16361=CARTESIAN_POINT('Ctrl Pts',(-7.71522634131141,0.940871035193538,
24.8457878649339));
#16362=CARTESIAN_POINT('Ctrl Pts',(-7.98526240565798,1.11182427083088,24.8577910517233));
#16363=CARTESIAN_POINT('Ctrl Pts',(-8.2787512356013,1.16744491727749,24.8697942385126));
#16364=CARTESIAN_POINT('Ctrl Pts',(-8.57224006554462,1.2230655637241,24.8817974253019));
#16365=CARTESIAN_POINT('Ctrl Pts',(-8.88610136059951,1.1627698566702,24.8938006120912));
#16366=CARTESIAN_POINT('Ctrl Pts',(-9.13808834820102,1.00235817476344,24.9058037988805));
#16367=CARTESIAN_POINT('Ctrl Pts',(-9.39007533580253,0.841946492856676,
24.9178069856698));
#16368=CARTESIAN_POINT('Ctrl Pts',(-9.5775432964214,0.583102430602848,24.9298101724592));
#16369=CARTESIAN_POINT('Ctrl Pts',(-9.65136659729192,0.293655596346159,
24.9418133592485));
#16370=CARTESIAN_POINT('Ctrl Pts',(-9.67581103310546,0.197813707972355,
24.9457878649339));
#16371=CARTESIAN_POINT('Ctrl Pts',(-9.68822500000003,0.0989100500921392,
24.9497623706194));
#16372=CARTESIAN_POINT('Ctrl Pts',(-9.688225,-3.49664741605693E-13,24.9537368763049));
#16373=CARTESIAN_POINT('Origin',(-8.5,0.,1.8));
#16374=CARTESIAN_POINT('',(-9.6871905929363,0.000217402971942964,25.2962631236951));
#16375=CARTESIAN_POINT('',(-9.688225,-3.91631171936524E-13,25.2537368763049));
#16376=CARTESIAN_POINT('',(-9.688225,-1.45515594291686E-16,1.8));
#16377=CARTESIAN_POINT('Ctrl Pts',(-9.68646993064437,0.000368865704102106,
25.2962631236951));
#16378=CARTESIAN_POINT('Ctrl Pts',(-9.68708439251358,0.173016958435834,
25.2893486417863));
#16379=CARTESIAN_POINT('Ctrl Pts',(-9.65191323401855,0.345465200581628,
25.2824341598775));
#16380=CARTESIAN_POINT('Ctrl Pts',(-9.5797823988822,0.500859996551334,25.2755196779686));
#16381=CARTESIAN_POINT('Ctrl Pts',(-9.41383940890919,0.858358658818528,
25.259612336817));
#16382=CARTESIAN_POINT('Ctrl Pts',(-9.05228055867788,1.12559883272073,25.2437049956654));
#16383=CARTESIAN_POINT('Ctrl Pts',(-8.66213915242611,1.17921575971508,25.2277976545138));
#16384=CARTESIAN_POINT('Ctrl Pts',(-8.2719977461744,1.23283268670942,25.2118903133621));
#16385=CARTESIAN_POINT('Ctrl Pts',(-7.85327378390223,1.07282636679594,25.1959829722105));
#16386=CARTESIAN_POINT('Ctrl Pts',(-7.59622570194734,0.773747699679508,
25.1800756310589));
#16387=CARTESIAN_POINT('Ctrl Pts',(-7.46770166096987,0.624208366121258,
25.1721219604831));
#16388=CARTESIAN_POINT('Ctrl Pts',(-7.37959659007174,0.439900945762252,
25.1641682899073));
#16389=CARTESIAN_POINT('Ctrl Pts',(-7.3385132018884,0.245648673673906,25.1562146193315));
#16390=CARTESIAN_POINT('Ctrl Pts',(-7.29742981370506,0.0513964015856042,
25.1482609487557));
#16391=CARTESIAN_POINT('Ctrl Pts',(-7.3033681082365,-0.152800722232033,
25.1403072781799));
#16392=CARTESIAN_POINT('Ctrl Pts',(-7.36034118769235,-0.34157177299863,
25.1323536076041));
#16393=CARTESIAN_POINT('Ctrl Pts',(-7.47428734660405,-0.719113874531823,
25.1164462664524));
#16394=CARTESIAN_POINT('Ctrl Pts',(-7.7923726452134,-1.03495168386085,25.1005389253008));
#16395=CARTESIAN_POINT('Ctrl Pts',(-8.1708146320899,-1.1438863170192,25.0846315841492));
#16396=CARTESIAN_POINT('Ctrl Pts',(-8.54925661896646,-1.25282095017757,
25.0687242429976));
#16397=CARTESIAN_POINT('Ctrl Pts',(-8.98805529411019,-1.1548524071652,25.052816901846));
#16398=CARTESIAN_POINT('Ctrl Pts',(-9.28453253432374,-0.895153320760619,
25.0369095606943));
#16399=CARTESIAN_POINT('Ctrl Pts',(-9.53705207548348,-0.673958958281899,
25.0233607483613));
#16400=CARTESIAN_POINT('Ctrl Pts',(-9.68632458412737,-0.335437232707008,
25.0098119360282));
#16401=CARTESIAN_POINT('Ctrl Pts',(-9.68908827253991,0.000893915270617441,
24.9962631236951));
#16402=CARTESIAN_POINT('Ctrl Pts',(-9.688225,-3.49664741605693E-13,24.9537368763049));
#16403=CARTESIAN_POINT('Ctrl Pts',(-9.68822499999991,-0.298712821306432,
24.9657400630942));
#16404=CARTESIAN_POINT('Ctrl Pts',(-9.57054245632569,-0.595858078271821,
24.9777432498835));
#16405=CARTESIAN_POINT('Ctrl Pts',(-9.36601586214913,-0.81356940523295,
24.9897464366728));
#16406=CARTESIAN_POINT('Ctrl Pts',(-9.16148926797257,-1.03128073219408,
25.0017496234621));
#16407=CARTESIAN_POINT('Ctrl Pts',(-8.87226522412817,-1.16727314847144,
25.0137528102514));
#16408=CARTESIAN_POINT('Ctrl Pts',(-8.57413435701422,-1.18591009260192,
25.0257559970408));
#16409=CARTESIAN_POINT('Ctrl Pts',(-8.27600348990027,-1.20454703673239,
25.0377591838301));
#16410=CARTESIAN_POINT('Ctrl Pts',(-7.97209482032071,-1.10563290540098,
25.0497623706194));
#16411=CARTESIAN_POINT('Ctrl Pts',(-7.74204705372044,-0.915087963996431,
25.0617655574087));
#16412=CARTESIAN_POINT('Ctrl Pts',(-7.51199928712016,-0.724543022591879,
25.073768744198));
#16413=CARTESIAN_POINT('Ctrl Pts',(-7.35822688079627,-0.444367128061279,
25.0857719309873));
#16414=CARTESIAN_POINT('Ctrl Pts',(-7.32102560975815,-0.147979855990113,
25.0977751177767));
#16415=CARTESIAN_POINT('Ctrl Pts',(-7.28382433872002,0.148407416081053,
25.109778304566));
#16416=CARTESIAN_POINT('Ctrl Pts',(-7.36358464744643,0.457895344722108,
25.1217814913553));
#16417=CARTESIAN_POINT('Ctrl Pts',(-7.53940549437891,0.699383189957815,
25.1337846781446));
#16418=CARTESIAN_POINT('Ctrl Pts',(-7.71522634131139,0.940871035193521,
25.1457878649339));
#16419=CARTESIAN_POINT('Ctrl Pts',(-7.98526240565795,1.11182427083087,25.1577910517233));
#16420=CARTESIAN_POINT('Ctrl Pts',(-8.27875123560127,1.16744491727749,25.1697942385126));
#16421=CARTESIAN_POINT('Ctrl Pts',(-8.57224006554459,1.2230655637241,25.1817974253019));
#16422=CARTESIAN_POINT('Ctrl Pts',(-8.88610136059949,1.16276985667021,25.1938006120912));
#16423=CARTESIAN_POINT('Ctrl Pts',(-9.138088348201,1.00235817476345,25.2058037988805));
#16424=CARTESIAN_POINT('Ctrl Pts',(-9.39007533580251,0.841946492856695,
25.2178069856698));
#16425=CARTESIAN_POINT('Ctrl Pts',(-9.57754329642138,0.583102430602871,
25.2298101724592));
#16426=CARTESIAN_POINT('Ctrl Pts',(-9.65136659729192,0.293655596346184,
25.2418133592485));
#16427=CARTESIAN_POINT('Ctrl Pts',(-9.67581103310546,0.197813707972359,
25.2457878649339));
#16428=CARTESIAN_POINT('Ctrl Pts',(-9.68822500000003,0.0989100500921199,
25.2497623706194));
#16429=CARTESIAN_POINT('Ctrl Pts',(-9.688225,-3.91631171936524E-13,25.2537368763049));
#16430=CARTESIAN_POINT('Origin',(-8.5,0.,1.8));
#16431=CARTESIAN_POINT('',(-9.688225,1.35125244327128E-12,25.5962631236951));
#16432=CARTESIAN_POINT('',(-9.688225,-3.66040531218914E-13,25.5537368763049));
#16433=CARTESIAN_POINT('',(-9.688225,-1.45515594291686E-16,1.8));
#16434=CARTESIAN_POINT('Ctrl Pts',(-9.688225,1.41875400316849E-12,25.5962631236951));
#16435=CARTESIAN_POINT('Ctrl Pts',(-9.68822499999964,0.298712821307546,
25.5842599369058));
#16436=CARTESIAN_POINT('Ctrl Pts',(-9.57054245632512,0.595858078272874,
25.5722567501165));
#16437=CARTESIAN_POINT('Ctrl Pts',(-9.36601586214831,0.813569405233827,
25.5602535633272));
#16438=CARTESIAN_POINT('Ctrl Pts',(-9.16148926797149,1.03128073219478,25.5482503765378));
#16439=CARTESIAN_POINT('Ctrl Pts',(-8.8722652241269,1.16727314847186,25.5362471897485));
#16440=CARTESIAN_POINT('Ctrl Pts',(-8.57413435701289,1.185910092602,25.5242440029592));
#16441=CARTESIAN_POINT('Ctrl Pts',(-8.27600348989887,1.20454703673214,25.5122408161699));
#16442=CARTESIAN_POINT('Ctrl Pts',(-7.97209482031938,1.10563290540036,25.5002376293806));
#16443=CARTESIAN_POINT('Ctrl Pts',(-7.7420470537193,0.915087963995491,25.4882344425912));
#16444=CARTESIAN_POINT('Ctrl Pts',(-7.51199928711923,0.724543022590624,
25.4762312558019));
#16445=CARTESIAN_POINT('Ctrl Pts',(-7.35822688079568,0.444367128059778,
25.4642280690126));
#16446=CARTESIAN_POINT('Ctrl Pts',(-7.32102560975795,0.147979855988516,
25.4522248822233));
#16447=CARTESIAN_POINT('Ctrl Pts',(-7.28382433872022,-0.148407416082745,
25.440221695434));
#16448=CARTESIAN_POINT('Ctrl Pts',(-7.36358464744707,-0.45789534472374,
25.4282185086447));
#16449=CARTESIAN_POINT('Ctrl Pts',(-7.53940549437993,-0.699383189959225,
25.4162153218553));
#16450=CARTESIAN_POINT('Ctrl Pts',(-7.7152263413128,-0.94087103519471,25.404212135066));
#16451=CARTESIAN_POINT('Ctrl Pts',(-7.98526240565967,-1.11182427083168,
25.3922089482767));
#16452=CARTESIAN_POINT('Ctrl Pts',(-8.27875123560312,-1.16744491727784,
25.3802057614874));
#16453=CARTESIAN_POINT('Ctrl Pts',(-8.57224006554658,-1.223065563724,25.3682025746981));
#16454=CARTESIAN_POINT('Ctrl Pts',(-8.88610136060142,-1.16276985666958,
25.3561993879087));
#16455=CARTESIAN_POINT('Ctrl Pts',(-9.1380883482027,-1.00235817476237,25.3441962011194));
#16456=CARTESIAN_POINT('Ctrl Pts',(-9.39007533580398,-0.841946492855162,
25.3321930143301));
#16457=CARTESIAN_POINT('Ctrl Pts',(-9.57754329642243,-0.583102430600965,
25.3201898275408));
#16458=CARTESIAN_POINT('Ctrl Pts',(-9.65136659729245,-0.293655596344101,
25.3081866407515));
#16459=CARTESIAN_POINT('Ctrl Pts',(-9.67581103310572,-0.197813707970602,
25.304212135066));
#16460=CARTESIAN_POINT('Ctrl Pts',(-9.68822500000012,-0.0989100500907355,
25.3002376293806));
#16461=CARTESIAN_POINT('Ctrl Pts',(-9.688225,1.39321887360211E-12,25.2962631236951));
#16462=CARTESIAN_POINT('Ctrl Pts',(-9.688225,-3.91631171936524E-13,25.2537368763049));
#16463=CARTESIAN_POINT('Ctrl Pts',(-9.6882249999999,-0.298712821306451,
25.2657400630942));
#16464=CARTESIAN_POINT('Ctrl Pts',(-9.57054245632569,-0.595858078271815,
25.2777432498835));
#16465=CARTESIAN_POINT('Ctrl Pts',(-9.36601586214915,-0.813569405232931,
25.2897464366728));
#16466=CARTESIAN_POINT('Ctrl Pts',(-9.16148926797261,-1.03128073219405,
25.3017496234621));
#16467=CARTESIAN_POINT('Ctrl Pts',(-8.87226522412824,-1.16727314847142,
25.3137528102514));
#16468=CARTESIAN_POINT('Ctrl Pts',(-8.57413435701432,-1.18591009260191,
25.3257559970408));
#16469=CARTESIAN_POINT('Ctrl Pts',(-8.27600348990039,-1.20454703673241,
25.3377591838301));
#16470=CARTESIAN_POINT('Ctrl Pts',(-7.97209482032085,-1.10563290540104,
25.3497623706194));
#16471=CARTESIAN_POINT('Ctrl Pts',(-7.74204705372056,-0.915087963996534,
25.3617655574087));
#16472=CARTESIAN_POINT('Ctrl Pts',(-7.51199928712028,-0.724543022592027,
25.373768744198));
#16473=CARTESIAN_POINT('Ctrl Pts',(-7.35822688079636,-0.444367128061476,
25.3857719309873));
#16474=CARTESIAN_POINT('Ctrl Pts',(-7.32102560975818,-0.14797985599034,
25.3977751177767));
#16475=CARTESIAN_POINT('Ctrl Pts',(-7.28382433872,0.148407416080797,25.409778304566));
#16476=CARTESIAN_POINT('Ctrl Pts',(-7.36358464744633,0.457895344721843,
25.4217814913553));
#16477=CARTESIAN_POINT('Ctrl Pts',(-7.53940549437873,0.699383189957575,
25.4337846781446));
#16478=CARTESIAN_POINT('Ctrl Pts',(-7.71522634131114,0.940871035193308,
25.4457878649339));
#16479=CARTESIAN_POINT('Ctrl Pts',(-7.98526240565763,1.11182427083072,25.4577910517232));
#16480=CARTESIAN_POINT('Ctrl Pts',(-8.27875123560092,1.16744491727742,25.4697942385126));
#16481=CARTESIAN_POINT('Ctrl Pts',(-8.5722400655442,1.22306556372412,25.4817974253019));
#16482=CARTESIAN_POINT('Ctrl Pts',(-8.88610136059908,1.16276985667034,25.4938006120912));
#16483=CARTESIAN_POINT('Ctrl Pts',(-9.13808834820063,1.00235817476368,25.5058037988805));
#16484=CARTESIAN_POINT('Ctrl Pts',(-9.39007533580219,0.84194649285703,25.5178069856698));
#16485=CARTESIAN_POINT('Ctrl Pts',(-9.57754329642115,0.583102430603301,
25.5298101724591));
#16486=CARTESIAN_POINT('Ctrl Pts',(-9.65136659729179,0.293655596346667,
25.5418133592485));
#16487=CARTESIAN_POINT('Ctrl Pts',(-9.67581103310542,0.197813707972699,
25.5457878649339));
#16488=CARTESIAN_POINT('Ctrl Pts',(-9.68822500000003,0.0989100500923029,
25.5497623706194));
#16489=CARTESIAN_POINT('Ctrl Pts',(-9.688225,-3.66040531218914E-13,25.5537368763049));
#16490=CARTESIAN_POINT('Origin',(-8.5,0.,1.8));
#16491=CARTESIAN_POINT('',(-9.688225,1.37678757283766E-12,25.8962631236951));
#16492=CARTESIAN_POINT('',(-9.688225,-3.40394379350073E-13,25.8537368763049));
#16493=CARTESIAN_POINT('',(-9.688225,-1.45515594291686E-16,1.8));
#16494=CARTESIAN_POINT('Ctrl Pts',(-9.688225,1.37678757283766E-12,25.8962631236951));
#16495=CARTESIAN_POINT('Ctrl Pts',(-9.68822499999965,0.298712821307437,
25.8842599369058));
#16496=CARTESIAN_POINT('Ctrl Pts',(-9.5705424563252,0.595858078272703,25.8722567501165));
#16497=CARTESIAN_POINT('Ctrl Pts',(-9.36601586214848,0.813569405233649,
25.8602535633272));
#16498=CARTESIAN_POINT('Ctrl Pts',(-9.16148926797175,1.0312807321946,25.8482503765379));
#16499=CARTESIAN_POINT('Ctrl Pts',(-8.87226522412728,1.16727314847173,25.8362471897485));
#16500=CARTESIAN_POINT('Ctrl Pts',(-8.57413435701333,1.18591009260197,25.8242440029592));
#16501=CARTESIAN_POINT('Ctrl Pts',(-8.27600348989939,1.20454703673222,25.8122408161699));
#16502=CARTESIAN_POINT('Ctrl Pts',(-7.97209482031993,1.1056329054006,25.8002376293806));
#16503=CARTESIAN_POINT('Ctrl Pts',(-7.7420470537198,0.915087963995906,25.7882344425913));
#16504=CARTESIAN_POINT('Ctrl Pts',(-7.51199928711968,0.724543022591208,
25.776231255802));
#16505=CARTESIAN_POINT('Ctrl Pts',(-7.35822688079599,0.44436712806053,25.7642280690126));
#16506=CARTESIAN_POINT('Ctrl Pts',(-7.32102560975805,0.147979855989362,
25.7522248822233));
#16507=CARTESIAN_POINT('Ctrl Pts',(-7.28382433872012,-0.148407416081805,
25.740221695434));
#16508=CARTESIAN_POINT('Ctrl Pts',(-7.36358464744671,-0.457895344722785,
25.7282185086447));
#16509=CARTESIAN_POINT('Ctrl Pts',(-7.53940549437931,-0.699383189958372,
25.7162153218554));
#16510=CARTESIAN_POINT('Ctrl Pts',(-7.71522634131192,-0.940871035193959,
25.7042121350661));
#16511=CARTESIAN_POINT('Ctrl Pts',(-7.98526240565856,-1.11182427083115,
25.6922089482767));
#16512=CARTESIAN_POINT('Ctrl Pts',(-8.27875123560188,-1.1674449172776,25.6802057614874));
#16513=CARTESIAN_POINT('Ctrl Pts',(-8.57224006554521,-1.22306556372406,
25.6682025746981));
#16514=CARTESIAN_POINT('Ctrl Pts',(-8.88610136060005,-1.16276985667002,
25.6561993879088));
#16515=CARTESIAN_POINT('Ctrl Pts',(-9.13808834820147,-1.00235817476316,
25.6441962011195));
#16516=CARTESIAN_POINT('Ctrl Pts',(-9.39007533580288,-0.841946492856292,
25.6321930143302));
#16517=CARTESIAN_POINT('Ctrl Pts',(-9.57754329642163,-0.583102430602408,
25.6201898275408));
#16518=CARTESIAN_POINT('Ctrl Pts',(-9.65136659729204,-0.293655596345712,
25.6081866407515));
#16519=CARTESIAN_POINT('Ctrl Pts',(-9.67581103310559,-0.197813707971703,
25.6042121350661));
#16520=CARTESIAN_POINT('Ctrl Pts',(-9.68822500000012,-0.0989100500912729,
25.6002376293806));
#16521=CARTESIAN_POINT('Ctrl Pts',(-9.688225,1.41875400316849E-12,25.5962631236951));
#16522=CARTESIAN_POINT('Ctrl Pts',(-9.688225,-3.66040531218914E-13,25.5537368763049));
#16523=CARTESIAN_POINT('Ctrl Pts',(-9.68822499999991,-0.298712821306471,
25.5657400630942));
#16524=CARTESIAN_POINT('Ctrl Pts',(-9.57054245632567,-0.595858078271881,
25.5777432498835));
#16525=CARTESIAN_POINT('Ctrl Pts',(-9.36601586214907,-0.813569405233011,
25.5897464366728));
#16526=CARTESIAN_POINT('Ctrl Pts',(-9.16148926797248,-1.03128073219414,
25.6017496234621));
#16527=CARTESIAN_POINT('Ctrl Pts',(-8.87226522412805,-1.16727314847149,
25.6137528102514));
#16528=CARTESIAN_POINT('Ctrl Pts',(-8.57413435701407,-1.18591009260193,
25.6257559970408));
#16529=CARTESIAN_POINT('Ctrl Pts',(-8.27600348990009,-1.20454703673236,
25.6377591838301));
#16530=CARTESIAN_POINT('Ctrl Pts',(-7.97209482032053,-1.1056329054009,25.6497623706194));
#16531=CARTESIAN_POINT('Ctrl Pts',(-7.74204705372027,-0.915087963996292,
25.6617655574087));
#16532=CARTESIAN_POINT('Ctrl Pts',(-7.51199928712001,-0.724543022591682,
25.673768744198));
#16533=CARTESIAN_POINT('Ctrl Pts',(-7.35822688079617,-0.444367128061026,
25.6857719309874));
#16534=CARTESIAN_POINT('Ctrl Pts',(-7.32102560975811,-0.147979855989829,
25.6977751177767));
#16535=CARTESIAN_POINT('Ctrl Pts',(-7.28382433872006,0.148407416081368,
25.709778304566));
#16536=CARTESIAN_POINT('Ctrl Pts',(-7.36358464744655,0.457895344722428,
25.7217814913553));
#16537=CARTESIAN_POINT('Ctrl Pts',(-7.53940549437912,0.699383189958101,
25.7337846781446));
#16538=CARTESIAN_POINT('Ctrl Pts',(-7.71522634131168,0.940871035193773,
25.7457878649339));
#16539=CARTESIAN_POINT('Ctrl Pts',(-7.98526240565833,1.11182427083105,25.7577910517233));
#16540=CARTESIAN_POINT('Ctrl Pts',(-8.27875123560169,1.16744491727756,25.7697942385126));
#16541=CARTESIAN_POINT('Ctrl Pts',(-8.57224006554505,1.22306556372408,25.7817974253019));
#16542=CARTESIAN_POINT('Ctrl Pts',(-8.88610136059995,1.16276985667006,25.7938006120912));
#16543=CARTESIAN_POINT('Ctrl Pts',(-9.13808834820141,1.00235817476319,25.8058037988805));
#16544=CARTESIAN_POINT('Ctrl Pts',(-9.39007533580287,0.841946492856317,
25.8178069856699));
#16545=CARTESIAN_POINT('Ctrl Pts',(-9.57754329642165,0.583102430602388,
25.8298101724592));
#16546=CARTESIAN_POINT('Ctrl Pts',(-9.65136659729205,0.293655596345644,
25.8418133592485));
#16547=CARTESIAN_POINT('Ctrl Pts',(-9.6758110331055,0.197813707972026,25.8457878649339));
#16548=CARTESIAN_POINT('Ctrl Pts',(-9.68822500000002,0.0989100500920135,
25.8497623706194));
#16549=CARTESIAN_POINT('Ctrl Pts',(-9.688225,-2.72781797150401E-13,25.8537368763049));
#16550=CARTESIAN_POINT('Origin',(-8.5,0.,1.8));
#16551=CARTESIAN_POINT('',(-9.688225,1.40254474700896E-12,26.1962631236951));
#16552=CARTESIAN_POINT('',(-9.688225,-3.14803738632463E-13,26.1537368763049));
#16553=CARTESIAN_POINT('',(-9.688225,-1.45515594291686E-16,1.8));
#16554=CARTESIAN_POINT('Ctrl Pts',(-9.688225,1.40254474700896E-12,26.1962631236951));
#16555=CARTESIAN_POINT('Ctrl Pts',(-9.68822499999965,0.298712821307485,
26.1842599369058));
#16556=CARTESIAN_POINT('Ctrl Pts',(-9.57054245632517,0.59585807827277,26.1722567501165));
#16557=CARTESIAN_POINT('Ctrl Pts',(-9.36601586214841,0.813569405233717,
26.1602535633272));
#16558=CARTESIAN_POINT('Ctrl Pts',(-9.16148926797166,1.03128073219466,26.1482503765379));
#16559=CARTESIAN_POINT('Ctrl Pts',(-8.87226522412714,1.16727314847177,26.1362471897485));
#16560=CARTESIAN_POINT('Ctrl Pts',(-8.57413435701317,1.18591009260198,26.1242440029592));
#16561=CARTESIAN_POINT('Ctrl Pts',(-8.2760034898992,1.20454703673219,26.1122408161699));
#16562=CARTESIAN_POINT('Ctrl Pts',(-7.97209482031974,1.10563290540052,26.1002376293806));
#16563=CARTESIAN_POINT('Ctrl Pts',(-7.74204705371963,0.91508796399576,26.0882344425913));
#16564=CARTESIAN_POINT('Ctrl Pts',(-7.51199928711952,0.724543022591003,
26.076231255802));
#16565=CARTESIAN_POINT('Ctrl Pts',(-7.35822688079588,0.444367128060268,
26.0642280690126));
#16566=CARTESIAN_POINT('Ctrl Pts',(-7.32102560975802,0.147979855989069,
26.0522248822233));
#16567=CARTESIAN_POINT('Ctrl Pts',(-7.28382433872016,-0.14840741608213,
26.040221695434));
#16568=CARTESIAN_POINT('Ctrl Pts',(-7.36358464744683,-0.457895344723115,
26.0282185086447));
#16569=CARTESIAN_POINT('Ctrl Pts',(-7.53940549437953,-0.699383189958666,
26.0162153218554));
#16570=CARTESIAN_POINT('Ctrl Pts',(-7.71522634131222,-0.940871035194217,
26.004212135066));
#16571=CARTESIAN_POINT('Ctrl Pts',(-7.98526240565894,-1.11182427083133,
25.9922089482767));
#16572=CARTESIAN_POINT('Ctrl Pts',(-8.27875123560231,-1.16744491727768,
25.9802057614874));
#16573=CARTESIAN_POINT('Ctrl Pts',(-8.57224006554568,-1.22306556372404,
25.9682025746981));
#16574=CARTESIAN_POINT('Ctrl Pts',(-8.88610136060052,-1.16276985666987,
25.9561993879088));
#16575=CARTESIAN_POINT('Ctrl Pts',(-9.13808834820189,-1.00235817476289,
25.9441962011195));
#16576=CARTESIAN_POINT('Ctrl Pts',(-9.39007533580326,-0.841946492855907,
25.9321930143301));
#16577=CARTESIAN_POINT('Ctrl Pts',(-9.5775432964219,-0.583102430601916,
25.9201898275408));
#16578=CARTESIAN_POINT('Ctrl Pts',(-9.65136659729218,-0.293655596345164,
25.9081866407515));
#16579=CARTESIAN_POINT('Ctrl Pts',(-9.67581103310563,-0.197813707971339,
25.904212135066));
#16580=CARTESIAN_POINT('Ctrl Pts',(-9.68822500000012,-0.0989100500911121,
25.9002376293806));
#16581=CARTESIAN_POINT('Ctrl Pts',(-9.688225,1.37678757283766E-12,25.8962631236951));
#16582=CARTESIAN_POINT('Ctrl Pts',(-9.688225,-2.72781797150401E-13,25.8537368763049));
#16583=CARTESIAN_POINT('Ctrl Pts',(-9.68822499999993,-0.2987128213064,25.8657400630942));
#16584=CARTESIAN_POINT('Ctrl Pts',(-9.5705424563257,-0.595858078271841,
25.8777432498835));
#16585=CARTESIAN_POINT('Ctrl Pts',(-9.36601586214909,-0.813569405232992,
25.8897464366728));
#16586=CARTESIAN_POINT('Ctrl Pts',(-9.16148926797249,-1.03128073219414,
25.9017496234621));
#16587=CARTESIAN_POINT('Ctrl Pts',(-8.87226522412803,-1.1672731484715,25.9137528102514));
#16588=CARTESIAN_POINT('Ctrl Pts',(-8.57413435701403,-1.18591009260193,
25.9257559970408));
#16589=CARTESIAN_POINT('Ctrl Pts',(-8.27600348990003,-1.20454703673236,
25.9377591838301));
#16590=CARTESIAN_POINT('Ctrl Pts',(-7.97209482032044,-1.10563290540087,
25.9497623706194));
#16591=CARTESIAN_POINT('Ctrl Pts',(-7.74204705372019,-0.915087963996222,
25.9617655574087));
#16592=CARTESIAN_POINT('Ctrl Pts',(-7.51199928711993,-0.724543022591577,
25.973768744198));
#16593=CARTESIAN_POINT('Ctrl Pts',(-7.3582268807961,-0.444367128060879,
25.9857719309874));
#16594=CARTESIAN_POINT('Ctrl Pts',(-7.32102560975809,-0.147979855989653,
25.9977751177767));
#16595=CARTESIAN_POINT('Ctrl Pts',(-7.28382433872008,0.148407416081572,
26.009778304566));
#16596=CARTESIAN_POINT('Ctrl Pts',(-7.36358464744663,0.457895344722644,
26.0217814913553));
#16597=CARTESIAN_POINT('Ctrl Pts',(-7.53940549437926,0.699383189958299,
26.0337846781446));
#16598=CARTESIAN_POINT('Ctrl Pts',(-7.71522634131189,0.940871035193953,
26.045787864934));
#16599=CARTESIAN_POINT('Ctrl Pts',(-7.98526240565859,1.11182427083118,26.0577910517233));
#16600=CARTESIAN_POINT('Ctrl Pts',(-8.27875123560199,1.16744491727762,26.0697942385126));
#16601=CARTESIAN_POINT('Ctrl Pts',(-8.5722400655454,1.22306556372406,26.0817974253019));
#16602=CARTESIAN_POINT('Ctrl Pts',(-8.8861013606003,1.16276985666995,26.0938006120912));
#16603=CARTESIAN_POINT('Ctrl Pts',(-9.13808834820173,1.00235817476299,26.1058037988806));
#16604=CARTESIAN_POINT('Ctrl Pts',(-9.39007533580316,0.84194649285602,26.1178069856699));
#16605=CARTESIAN_POINT('Ctrl Pts',(-9.57754329642187,0.583102430602004,
26.1298101724592));
#16606=CARTESIAN_POINT('Ctrl Pts',(-9.65136659729217,0.293655596345211,
26.1418133592485));
#16607=CARTESIAN_POINT('Ctrl Pts',(-9.67581103310554,0.197813707971715,
26.145787864934));
#16608=CARTESIAN_POINT('Ctrl Pts',(-9.68822500000003,0.0989100500918363,
26.1497623706194));
#16609=CARTESIAN_POINT('Ctrl Pts',(-9.688225,-3.14803738632463E-13,26.1537368763049));
#16610=CARTESIAN_POINT('Origin',(-8.5,0.,1.8));
#16611=CARTESIAN_POINT('',(-9.688225,1.42807987657534E-12,26.4962631236951));
#16612=CARTESIAN_POINT('',(-9.68738609224838,-0.000346572711688259,26.4537368763049));
#16613=CARTESIAN_POINT('',(-9.688225,-1.45515594291686E-16,1.8));
#16614=CARTESIAN_POINT('Ctrl Pts',(-9.688225,1.56308299636976E-12,26.4962631236951));
#16615=CARTESIAN_POINT('Ctrl Pts',(-9.68822499999961,0.2987128213076,26.4842599369058));
#16616=CARTESIAN_POINT('Ctrl Pts',(-9.57054245632512,0.595858078272826,
26.4722567501165));
#16617=CARTESIAN_POINT('Ctrl Pts',(-9.36601586214839,0.813569405233736,
26.4602535633272));
#16618=CARTESIAN_POINT('Ctrl Pts',(-9.16148926797167,1.03128073219465,26.4482503765379));
#16619=CARTESIAN_POINT('Ctrl Pts',(-8.8722652241272,1.16727314847174,26.4362471897485));
#16620=CARTESIAN_POINT('Ctrl Pts',(-8.57413435701328,1.18591009260198,26.4242440029592));
#16621=CARTESIAN_POINT('Ctrl Pts',(-8.27600348989936,1.20454703673221,26.4122408161699));
#16622=CARTESIAN_POINT('Ctrl Pts',(-7.97209482031993,1.1056329054006,26.4002376293806));
#16623=CARTESIAN_POINT('Ctrl Pts',(-7.74204705371982,0.915087963995916,
26.3882344425913));
#16624=CARTESIAN_POINT('Ctrl Pts',(-7.51199928711971,0.724543022591235,
26.376231255802));
#16625=CARTESIAN_POINT('Ctrl Pts',(-7.35822688079601,0.444367128060588,
26.3642280690126));
#16626=CARTESIAN_POINT('Ctrl Pts',(-7.32102560975806,0.147979855989445,
26.3522248822233));
#16627=CARTESIAN_POINT('Ctrl Pts',(-7.28382433872011,-0.148407416081697,
26.340221695434));
#16628=CARTESIAN_POINT('Ctrl Pts',(-7.36358464744666,-0.457895344722659,
26.3282185086447));
#16629=CARTESIAN_POINT('Ctrl Pts',(-7.53940549437922,-0.69938318995825,
26.3162153218554));
#16630=CARTESIAN_POINT('Ctrl Pts',(-7.71522634131179,-0.940871035193841,
26.3042121350661));
#16631=CARTESIAN_POINT('Ctrl Pts',(-7.98526240565837,-1.11182427083106,
26.2922089482768));
#16632=CARTESIAN_POINT('Ctrl Pts',(-8.27875123560167,-1.16744491727756,
26.2802057614874));
#16633=CARTESIAN_POINT('Ctrl Pts',(-8.57224006554497,-1.22306556372407,
26.2682025746981));
#16634=CARTESIAN_POINT('Ctrl Pts',(-8.88610136059979,-1.1627698566701,26.2561993879088));
#16635=CARTESIAN_POINT('Ctrl Pts',(-9.13808834820122,-1.00235817476331,
26.2441962011195));
#16636=CARTESIAN_POINT('Ctrl Pts',(-9.39007533580266,-0.841946492856519,
26.2321930143302));
#16637=CARTESIAN_POINT('Ctrl Pts',(-9.57754329642146,-0.583102430602707,
26.2201898275409));
#16638=CARTESIAN_POINT('Ctrl Pts',(-9.65136659729195,-0.293655596346055,
26.2081866407515));
#16639=CARTESIAN_POINT('Ctrl Pts',(-9.67581103310556,-0.197813707971944,
26.2042121350661));
#16640=CARTESIAN_POINT('Ctrl Pts',(-9.68822500000012,-0.0989100500914016,
26.2002376293806));
#16641=CARTESIAN_POINT('Ctrl Pts',(-9.688225,1.40254474700896E-12,26.1962631236951));
#16642=CARTESIAN_POINT('Ctrl Pts',(-9.688225,-3.14803738632463E-13,26.1537368763049));
#16643=CARTESIAN_POINT('Ctrl Pts',(-9.68822499999992,-0.298712821306329,
26.1657400630942));
#16644=CARTESIAN_POINT('Ctrl Pts',(-9.57054245632577,-0.595858078271657,
26.1777432498835));
#16645=CARTESIAN_POINT('Ctrl Pts',(-9.3660158621493,-0.813569405232776,
26.1897464366728));
#16646=CARTESIAN_POINT('Ctrl Pts',(-9.16148926797282,-1.0312807321939,26.2017496234621));
#16647=CARTESIAN_POINT('Ctrl Pts',(-8.87226522412854,-1.16727314847131,
26.2137528102514));
#16648=CARTESIAN_POINT('Ctrl Pts',(-8.57413435701466,-1.18591009260189,
26.2257559970407));
#16649=CARTESIAN_POINT('Ctrl Pts',(-8.27600348990081,-1.20454703673247,
26.2377591838301));
#16650=CARTESIAN_POINT('Ctrl Pts',(-7.97209482032131,-1.10563290540124,
26.2497623706194));
#16651=CARTESIAN_POINT('Ctrl Pts',(-7.74204705372099,-0.915087963996884,
26.2617655574087));
#16652=CARTESIAN_POINT('Ctrl Pts',(-7.51199928712063,-0.724543022592498,
26.273768744198));
#16653=CARTESIAN_POINT('Ctrl Pts',(-7.35822688079658,-0.444367128062047,
26.2857719309873));
#16654=CARTESIAN_POINT('Ctrl Pts',(-7.32102560975825,-0.147979855990952,
26.2977751177766));
#16655=CARTESIAN_POINT('Ctrl Pts',(-7.28382433871992,0.148407416080143,
26.3097783045659));
#16656=CARTESIAN_POINT('Ctrl Pts',(-7.36358464744607,0.457895344721206,
26.3217814913553));
#16657=CARTESIAN_POINT('Ctrl Pts',(-7.53940549437833,0.699383189957022,
26.3337846781446));
#16658=CARTESIAN_POINT('Ctrl Pts',(-7.71522634131058,0.940871035192837,
26.3457878649339));
#16659=CARTESIAN_POINT('Ctrl Pts',(-7.98526240565695,1.1118242708304,26.3577910517232));
#16660=CARTESIAN_POINT('Ctrl Pts',(-8.27875123560018,1.16744491727728,26.3697942385125));
#16661=CARTESIAN_POINT('Ctrl Pts',(-8.5722400655434,1.22306556372416,26.3817974253018));
#16662=CARTESIAN_POINT('Ctrl Pts',(-8.8861013605983,1.16276985667059,26.3938006120912));
#16663=CARTESIAN_POINT('Ctrl Pts',(-9.13808834819994,1.00235817476413,26.4058037988805));
#16664=CARTESIAN_POINT('Ctrl Pts',(-9.39007533580159,0.841946492857656,
26.4178069856698));
#16665=CARTESIAN_POINT('Ctrl Pts',(-9.57754329642071,0.583102430604084,
26.4298101724591));
#16666=CARTESIAN_POINT('Ctrl Pts',(-9.65136659729157,0.293655596347526,
26.4418133592484));
#16667=CARTESIAN_POINT('Ctrl Pts',(-9.67581103310532,0.197813707973359,
26.4457878649339));
#16668=CARTESIAN_POINT('Ctrl Pts',(-9.68822500000001,0.0989100500927401,
26.4497623706194));
#16669=CARTESIAN_POINT('Ctrl Pts',(-9.688225,-1.54098955817972E-13,26.4537368763048));
#16670=CARTESIAN_POINT('Origin',(-8.5,0.,1.8));
#16671=CARTESIAN_POINT('',(-9.688225,1.45372602844418E-12,26.7962631236951));
#16672=CARTESIAN_POINT('',(-9.68877351310573,-0.000284106499024444,26.7537368763048));
#16673=CARTESIAN_POINT('',(-9.688225,-1.45515594291686E-16,1.8));
#16674=CARTESIAN_POINT('Ctrl Pts',(-9.688225,1.45372602844418E-12,26.7962631236951));
#16675=CARTESIAN_POINT('Ctrl Pts',(-9.68822499999964,0.298712821307536,
26.7842599369058));
#16676=CARTESIAN_POINT('Ctrl Pts',(-9.57054245632514,0.595858078272816,
26.7722567501165));
#16677=CARTESIAN_POINT('Ctrl Pts',(-9.36601586214838,0.813569405233754,
26.7602535633272));
#16678=CARTESIAN_POINT('Ctrl Pts',(-9.16148926797161,1.03128073219469,26.7482503765379));
#16679=CARTESIAN_POINT('Ctrl Pts',(-8.87226522412709,1.16727314847179,26.7362471897485));
#16680=CARTESIAN_POINT('Ctrl Pts',(-8.57413435701312,1.18591009260199,26.7242440029592));
#16681=CARTESIAN_POINT('Ctrl Pts',(-8.27600348989915,1.20454703673218,26.7122408161699));
#16682=CARTESIAN_POINT('Ctrl Pts',(-7.97209482031969,1.10563290540049,26.7002376293806));
#16683=CARTESIAN_POINT('Ctrl Pts',(-7.74204705371959,0.915087963995727,
26.6882344425913));
#16684=CARTESIAN_POINT('Ctrl Pts',(-7.51199928711949,0.724543022590961,
26.6762312558019));
#16685=CARTESIAN_POINT('Ctrl Pts',(-7.35822688079586,0.444367128060219,
26.6642280690126));
#16686=CARTESIAN_POINT('Ctrl Pts',(-7.32102560975801,0.147979855989018,
26.6522248822233));
#16687=CARTESIAN_POINT('Ctrl Pts',(-7.28382433872016,-0.148407416082183,
26.640221695434));
#16688=CARTESIAN_POINT('Ctrl Pts',(-7.36358464744685,-0.457895344723164,
26.6282185086447));
#16689=CARTESIAN_POINT('Ctrl Pts',(-7.53940549437956,-0.699383189958707,
26.6162153218554));
#16690=CARTESIAN_POINT('Ctrl Pts',(-7.71522634131226,-0.940871035194251,
26.604212135066));
#16691=CARTESIAN_POINT('Ctrl Pts',(-7.98526240565899,-1.11182427083135,
26.5922089482767));
#16692=CARTESIAN_POINT('Ctrl Pts',(-8.27875123560236,-1.16744491727769,
26.5802057614874));
#16693=CARTESIAN_POINT('Ctrl Pts',(-8.57224006554573,-1.22306556372403,
26.5682025746981));
#16694=CARTESIAN_POINT('Ctrl Pts',(-8.88610136060057,-1.16276985666985,
26.5561993879088));
#16695=CARTESIAN_POINT('Ctrl Pts',(-9.13808834820193,-1.00235817476286,
26.5441962011195));
#16696=CARTESIAN_POINT('Ctrl Pts',(-9.39007533580329,-0.841946492855868,
26.5321930143301));
#16697=CARTESIAN_POINT('Ctrl Pts',(-9.57754329642193,-0.58310243060187,
26.5201898275408));
#16698=CARTESIAN_POINT('Ctrl Pts',(-9.65136659729219,-0.293655596345114,
26.5081866407515));
#16699=CARTESIAN_POINT('Ctrl Pts',(-9.67581103310565,-0.197813707971245,
26.504212135066));
#16700=CARTESIAN_POINT('Ctrl Pts',(-9.68822500000013,-0.0989100500909709,
26.5002376293806));
#16701=CARTESIAN_POINT('Ctrl Pts',(-9.688225,1.56308299636976E-12,26.4962631236951));
#16702=CARTESIAN_POINT('Ctrl Pts',(-9.68674334601053,-0.000612106443772073,
26.4537368763049));
#16703=CARTESIAN_POINT('Ctrl Pts',(-9.68760064018175,-0.15491495328169,
26.4599199595912));
#16704=CARTESIAN_POINT('Ctrl Pts',(-9.65970073938658,-0.308953253913664,
26.4661030428775));
#16705=CARTESIAN_POINT('Ctrl Pts',(-9.60165140328844,-0.450727135541932,
26.4722861261638));
#16706=CARTESIAN_POINT('Ctrl Pts',(-9.45230672359085,-0.815471616089674,
26.4881934673154));
#16707=CARTESIAN_POINT('Ctrl Pts',(-9.10340632447576,-1.09903928742264,
26.504100808467));
#16708=CARTESIAN_POINT('Ctrl Pts',(-8.71613991619992,-1.17052229766671,
26.5200081496187));
#16709=CARTESIAN_POINT('Ctrl Pts',(-8.32887350792413,-1.24200530791077,
26.5359154907703));
#16710=CARTESIAN_POINT('Ctrl Pts',(-7.90324109048761,-1.10140365706596,
26.5518228319219));
#16711=CARTESIAN_POINT('Ctrl Pts',(-7.63272502524997,-0.81444926346103,
26.5677301730735));
#16712=CARTESIAN_POINT('Ctrl Pts',(-7.49746699263114,-0.670972066658563,
26.5756838436493));
#16713=CARTESIAN_POINT('Ctrl Pts',(-7.40098804806204,-0.490906684166065,
26.5836375142251));
#16714=CARTESIAN_POINT('Ctrl Pts',(-7.35102428689118,-0.298746822161143,
26.591591184801));
#16715=CARTESIAN_POINT('Ctrl Pts',(-7.3010605257203,-0.106586960156177,
26.5995448553768));
#16716=CARTESIAN_POINT('Ctrl Pts',(-7.29761194794768,0.0976673813612168,
26.6074985259526));
#16717=CARTESIAN_POINT('Ctrl Pts',(-7.34585293277445,0.288856420725844,
26.6154521965284));
#16718=CARTESIAN_POINT('Ctrl Pts',(-7.44233490242797,0.671234499455056,
26.63135953768));
#16719=CARTESIAN_POINT('Ctrl Pts',(-7.74557512247899,1.00135136957321,26.6472668788316));
#16720=CARTESIAN_POINT('Ctrl Pts',(-8.11861322531683,1.1275562251199,26.6631742199833));
#16721=CARTESIAN_POINT('Ctrl Pts',(-8.49165132815463,1.25376108066657,26.6790815611349));
#16722=CARTESIAN_POINT('Ctrl Pts',(-8.93448731377924,1.17605392164181,26.6949889022865));
#16723=CARTESIAN_POINT('Ctrl Pts',(-9.24258185301928,0.930248868124899,
26.7108962434381));
#16724=CARTESIAN_POINT('Ctrl Pts',(-9.51916201639636,0.709586723225101,
26.7251764543937));
#16725=CARTESIAN_POINT('Ctrl Pts',(-9.68715582329318,0.353456699772103,
26.7394566653493));
#16726=CARTESIAN_POINT('Ctrl Pts',(-9.68953524092888,-0.000678649168437481,
26.7537368763049));
#16727=CARTESIAN_POINT('Origin',(-8.5,0.,1.8));
#16728=CARTESIAN_POINT('',(-9.688225,1.47926115801056E-12,27.0962631236951));
#16729=CARTESIAN_POINT('',(-9.688225,-2.37920794177171E-13,27.0537368763048));
#16730=CARTESIAN_POINT('',(-9.688225,-1.45515594291686E-16,1.8));
#16731=CARTESIAN_POINT('Ctrl Pts',(-9.688225,1.6144863224099E-12,27.0962631236951));
#16732=CARTESIAN_POINT('Ctrl Pts',(-9.6882249999996,0.298712821307742,27.0842599369058));
#16733=CARTESIAN_POINT('Ctrl Pts',(-9.57054245632502,0.59585807827305,27.0722567501165));
#16734=CARTESIAN_POINT('Ctrl Pts',(-9.36601586214817,0.81356940523397,27.0602535633272));
#16735=CARTESIAN_POINT('Ctrl Pts',(-9.16148926797132,1.03128073219489,27.0482503765378));
#16736=CARTESIAN_POINT('Ctrl Pts',(-8.87226522412671,1.16727314847192,27.0362471897485));
#16737=CARTESIAN_POINT('Ctrl Pts',(-8.57413435701269,1.18591009260201,27.0242440029592));
#16738=CARTESIAN_POINT('Ctrl Pts',(-8.27600348989867,1.2045470367321,27.0122408161699));
#16739=CARTESIAN_POINT('Ctrl Pts',(-7.9720948203192,1.10563290540027,27.0002376293806));
#16740=CARTESIAN_POINT('Ctrl Pts',(-7.74204705371915,0.915087963995366,
26.9882344425912));
#16741=CARTESIAN_POINT('Ctrl Pts',(-7.51199928711911,0.724543022590461,
26.9762312558019));
#16742=CARTESIAN_POINT('Ctrl Pts',(-7.3582268807956,0.44436712805959,26.9642280690126));
#16743=CARTESIAN_POINT('Ctrl Pts',(-7.32102560975792,0.147979855988322,
26.9522248822233));
#16744=CARTESIAN_POINT('Ctrl Pts',(-7.28382433872024,-0.148407416082945,
26.940221695434));
#16745=CARTESIAN_POINT('Ctrl Pts',(-7.36358464744715,-0.457895344723927,
26.9282185086446));
#16746=CARTESIAN_POINT('Ctrl Pts',(-7.53940549438005,-0.699383189959383,
26.9162153218553));
#16747=CARTESIAN_POINT('Ctrl Pts',(-7.71522634131295,-0.94087103519484,
26.904212135066));
#16748=CARTESIAN_POINT('Ctrl Pts',(-7.98526240565985,-1.11182427083176,
26.8922089482767));
#16749=CARTESIAN_POINT('Ctrl Pts',(-8.27875123560331,-1.16744491727787,
26.8802057614874));
#16750=CARTESIAN_POINT('Ctrl Pts',(-8.57224006554678,-1.22306556372398,
26.8682025746981));
#16751=CARTESIAN_POINT('Ctrl Pts',(-8.88610136060161,-1.16276985666952,
26.8561993879087));
#16752=CARTESIAN_POINT('Ctrl Pts',(-9.13808834820286,-1.00235817476227,
26.8441962011194));
#16753=CARTESIAN_POINT('Ctrl Pts',(-9.39007533580411,-0.841946492855016,
26.8321930143301));
#16754=CARTESIAN_POINT('Ctrl Pts',(-9.57754329642253,-0.583102430600788,
26.8201898275408));
#16755=CARTESIAN_POINT('Ctrl Pts',(-9.6513665972925,-0.293655596343911,
26.8081866407515));
#16756=CARTESIAN_POINT('Ctrl Pts',(-9.67581103310575,-0.197813707970453,
26.804212135066));
#16757=CARTESIAN_POINT('Ctrl Pts',(-9.68822500000012,-0.09891005009063,
26.8002376293806));
#16758=CARTESIAN_POINT('Ctrl Pts',(-9.688225,1.45372602844418E-12,26.7962631236951));
#16759=CARTESIAN_POINT('Ctrl Pts',(-9.688225,-1.28397292797899E-13,26.7537368763048));
#16760=CARTESIAN_POINT('Ctrl Pts',(-9.68822499999997,-0.298712821306256,
26.7657400630942));
#16761=CARTESIAN_POINT('Ctrl Pts',(-9.57054245632577,-0.595858078271711,
26.7777432498835));
#16762=CARTESIAN_POINT('Ctrl Pts',(-9.36601586214919,-0.813569405232887,
26.7897464366728));
#16763=CARTESIAN_POINT('Ctrl Pts',(-9.16148926797261,-1.03128073219406,
26.8017496234621));
#16764=CARTESIAN_POINT('Ctrl Pts',(-8.87226522412817,-1.16727314847146,
26.8137528102514));
#16765=CARTESIAN_POINT('Ctrl Pts',(-8.57413435701417,-1.18591009260192,
26.8257559970408));
#16766=CARTESIAN_POINT('Ctrl Pts',(-8.27600348990018,-1.20454703673238,
26.8377591838301));
#16767=CARTESIAN_POINT('Ctrl Pts',(-7.97209482032058,-1.10563290540093,
26.8497623706194));
#16768=CARTESIAN_POINT('Ctrl Pts',(-7.7420470537203,-0.915087963996314,
26.8617655574087));
#16769=CARTESIAN_POINT('Ctrl Pts',(-7.51199928712002,-0.724543022591697,
26.873768744198));
#16770=CARTESIAN_POINT('Ctrl Pts',(-7.35822688079616,-0.444367128061017,
26.8857719309874));
#16771=CARTESIAN_POINT('Ctrl Pts',(-7.32102560975811,-0.147979855989797,
26.8977751177767));
#16772=CARTESIAN_POINT('Ctrl Pts',(-7.28382433872006,0.148407416081424,
26.909778304566));
#16773=CARTESIAN_POINT('Ctrl Pts',(-7.36358464744657,0.457895344722506,
26.9217814913553));
#16774=CARTESIAN_POINT('Ctrl Pts',(-7.53940549437917,0.699383189958182,
26.9337846781446));
#16775=CARTESIAN_POINT('Ctrl Pts',(-7.71522634131177,0.940871035193858,
26.945787864934));
#16776=CARTESIAN_POINT('Ctrl Pts',(-7.98526240565846,1.11182427083112,26.9577910517233));
#16777=CARTESIAN_POINT('Ctrl Pts',(-8.27875123560185,1.1674449172776,26.9697942385126));
#16778=CARTESIAN_POINT('Ctrl Pts',(-8.57224006554525,1.22306556372407,26.9817974253019));
#16779=CARTESIAN_POINT('Ctrl Pts',(-8.88610136060016,1.16276985667,26.9938006120912));
#16780=CARTESIAN_POINT('Ctrl Pts',(-9.13808834820161,1.00235817476306,27.0058037988805));
#16781=CARTESIAN_POINT('Ctrl Pts',(-9.39007533580306,0.841946492856128,
27.0178069856699));
#16782=CARTESIAN_POINT('Ctrl Pts',(-9.5775432964218,0.583102430602135,27.0298101724592));
#16783=CARTESIAN_POINT('Ctrl Pts',(-9.65136659729213,0.293655596345351,
27.0418133592485));
#16784=CARTESIAN_POINT('Ctrl Pts',(-9.67581103310552,0.197813707971836,
27.045787864934));
#16785=CARTESIAN_POINT('Ctrl Pts',(-9.68822500000002,0.0989100500919358,
27.0497623706194));
#16786=CARTESIAN_POINT('Ctrl Pts',(-9.688225,-2.37920794177171E-13,27.0537368763048));
#16787=CARTESIAN_POINT('Origin',(-8.5,0.,1.8));
#16788=CARTESIAN_POINT('',(-9.688225,1.5049073098794E-12,27.3962631236951));
#16789=CARTESIAN_POINT('',(-9.688225,-2.12330153459561E-13,27.3537368763049));
#16790=CARTESIAN_POINT('',(-9.688225,-1.45515594291686E-16,1.8));
#16791=CARTESIAN_POINT('Ctrl Pts',(-9.688225,1.5049073098794E-12,27.3962631236951));
#16792=CARTESIAN_POINT('Ctrl Pts',(-9.68822499999962,0.298712821307587,
27.3842599369058));
#16793=CARTESIAN_POINT('Ctrl Pts',(-9.57054245632511,0.595858078272862,
27.3722567501165));
#16794=CARTESIAN_POINT('Ctrl Pts',(-9.36601586214834,0.813569405233792,
27.3602535633272));
#16795=CARTESIAN_POINT('Ctrl Pts',(-9.16148926797157,1.03128073219472,27.3482503765378));
#16796=CARTESIAN_POINT('Ctrl Pts',(-8.87226522412704,1.16727314847181,27.3362471897485));
#16797=CARTESIAN_POINT('Ctrl Pts',(-8.57413435701307,1.18591009260199,27.3242440029592));
#16798=CARTESIAN_POINT('Ctrl Pts',(-8.2760034898991,1.20454703673217,27.3122408161699));
#16799=CARTESIAN_POINT('Ctrl Pts',(-7.97209482031964,1.10563290540047,27.3002376293806));
#16800=CARTESIAN_POINT('Ctrl Pts',(-7.74204705371955,0.915087963995695,
27.2882344425913));
#16801=CARTESIAN_POINT('Ctrl Pts',(-7.51199928711946,0.724543022590918,
27.2762312558019));
#16802=CARTESIAN_POINT('Ctrl Pts',(-7.35822688079584,0.444367128060169,
27.2642280690126));
#16803=CARTESIAN_POINT('Ctrl Pts',(-7.321025609758,0.147979855988967,27.2522248822233));
#16804=CARTESIAN_POINT('Ctrl Pts',(-7.28382433872017,-0.148407416082235,
27.240221695434));
#16805=CARTESIAN_POINT('Ctrl Pts',(-7.36358464744687,-0.457895344723213,
27.2282185086447));
#16806=CARTESIAN_POINT('Ctrl Pts',(-7.53940549437959,-0.699383189958749,
27.2162153218554));
#16807=CARTESIAN_POINT('Ctrl Pts',(-7.7152263413123,-0.940871035194285,
27.204212135066));
#16808=CARTESIAN_POINT('Ctrl Pts',(-7.98526240565903,-1.11182427083137,
27.1922089482767));
#16809=CARTESIAN_POINT('Ctrl Pts',(-8.27875123560241,-1.1674449172777,27.1802057614874));
#16810=CARTESIAN_POINT('Ctrl Pts',(-8.57224006554578,-1.22306556372403,
27.1682025746981));
#16811=CARTESIAN_POINT('Ctrl Pts',(-8.88610136060062,-1.16276985666984,
27.1561993879088));
#16812=CARTESIAN_POINT('Ctrl Pts',(-9.13808834820197,-1.00235817476283,
27.1441962011195));
#16813=CARTESIAN_POINT('Ctrl Pts',(-9.39007533580333,-0.84194649285583,
27.1321930143301));
#16814=CARTESIAN_POINT('Ctrl Pts',(-9.57754329642195,-0.583102430601823,
27.1201898275408));
#16815=CARTESIAN_POINT('Ctrl Pts',(-9.6513665972922,-0.293655596345064,
27.1081866407515));
#16816=CARTESIAN_POINT('Ctrl Pts',(-9.67581103310566,-0.197813707971194,
27.104212135066));
#16817=CARTESIAN_POINT('Ctrl Pts',(-9.68822500000014,-0.0989100500909195,
27.1002376293806));
#16818=CARTESIAN_POINT('Ctrl Pts',(-9.688225,1.6144863224099E-12,27.0962631236951));
#16819=CARTESIAN_POINT('Ctrl Pts',(-9.688225,-2.37920794177171E-13,27.0537368763048));
#16820=CARTESIAN_POINT('Ctrl Pts',(-9.68822499999994,-0.29871282130632,
27.0657400630942));
#16821=CARTESIAN_POINT('Ctrl Pts',(-9.57054245632575,-0.595858078271721,
27.0777432498835));
#16822=CARTESIAN_POINT('Ctrl Pts',(-9.36601586214921,-0.813569405232868,
27.0897464366728));
#16823=CARTESIAN_POINT('Ctrl Pts',(-9.16148926797267,-1.03128073219402,
27.1017496234621));
#16824=CARTESIAN_POINT('Ctrl Pts',(-8.87226522412828,-1.16727314847141,
27.1137528102514));
#16825=CARTESIAN_POINT('Ctrl Pts',(-8.57413435701433,-1.18591009260191,
27.1257559970408));
#16826=CARTESIAN_POINT('Ctrl Pts',(-8.27600348990038,-1.20454703673241,
27.1377591838301));
#16827=CARTESIAN_POINT('Ctrl Pts',(-7.97209482032082,-1.10563290540103,
27.1497623706194));
#16828=CARTESIAN_POINT('Ctrl Pts',(-7.74204705372053,-0.915087963996503,
27.1617655574087));
#16829=CARTESIAN_POINT('Ctrl Pts',(-7.51199928712023,-0.724543022591972,
27.173768744198));
#16830=CARTESIAN_POINT('Ctrl Pts',(-7.35822688079631,-0.444367128061387,
27.1857719309873));
#16831=CARTESIAN_POINT('Ctrl Pts',(-7.32102560975816,-0.147979855990224,
27.1977751177767));
#16832=CARTESIAN_POINT('Ctrl Pts',(-7.28382433872001,0.148407416080939,
27.209778304566));
#16833=CARTESIAN_POINT('Ctrl Pts',(-7.36358464744638,0.457895344722001,
27.2217814913553));
#16834=CARTESIAN_POINT('Ctrl Pts',(-7.53940549437884,0.699383189957724,
27.2337846781446));
#16835=CARTESIAN_POINT('Ctrl Pts',(-7.7152263413113,0.940871035193448,27.2457878649339));
#16836=CARTESIAN_POINT('Ctrl Pts',(-7.98526240565785,1.11182427083082,27.2577910517232));
#16837=CARTESIAN_POINT('Ctrl Pts',(-8.27875123560116,1.16744491727747,27.2697942385126));
#16838=CARTESIAN_POINT('Ctrl Pts',(-8.57224006554448,1.22306556372411,27.2817974253019));
#16839=CARTESIAN_POINT('Ctrl Pts',(-8.88610136059938,1.16276985667025,27.2938006120912));
#16840=CARTESIAN_POINT('Ctrl Pts',(-9.1380883482009,1.00235817476351,27.3058037988805));
#16841=CARTESIAN_POINT('Ctrl Pts',(-9.39007533580243,0.841946492856779,
27.3178069856698));
#16842=CARTESIAN_POINT('Ctrl Pts',(-9.57754329642133,0.583102430602972,
27.3298101724592));
#16843=CARTESIAN_POINT('Ctrl Pts',(-9.65136659729189,0.293655596346292,
27.3418133592485));
#16844=CARTESIAN_POINT('Ctrl Pts',(-9.67581103310544,0.197813707972491,
27.3457878649339));
#16845=CARTESIAN_POINT('Ctrl Pts',(-9.68822500000002,0.0989100500922765,
27.3497623706194));
#16846=CARTESIAN_POINT('Ctrl Pts',(-9.688225,-2.12330153459561E-13,27.3537368763049));
#16847=CARTESIAN_POINT('Origin',(-8.5,0.,1.8));
#16848=CARTESIAN_POINT('',(-9.688225,1.53055346174824E-12,27.6962631236951));
#16849=CARTESIAN_POINT('',(-9.688225,-1.8668400159072E-13,27.6537368763048));
#16850=CARTESIAN_POINT('',(-9.688225,-1.45515594291686E-16,1.8));
#16851=CARTESIAN_POINT('Ctrl Pts',(-9.688225,1.53055346174824E-12,27.6962631236951));
#16852=CARTESIAN_POINT('Ctrl Pts',(-9.68822499999962,0.298712821307613,
27.6842599369058));
#16853=CARTESIAN_POINT('Ctrl Pts',(-9.5705424563251,0.595858078272886,27.6722567501165));
#16854=CARTESIAN_POINT('Ctrl Pts',(-9.36601586214832,0.81356940523381,27.6602535633272));
#16855=CARTESIAN_POINT('Ctrl Pts',(-9.16148926797154,1.03128073219474,27.6482503765378));
#16856=CARTESIAN_POINT('Ctrl Pts',(-8.87226522412701,1.16727314847182,27.6362471897485));
#16857=CARTESIAN_POINT('Ctrl Pts',(-8.57413435701304,1.18591009260199,27.6242440029592));
#16858=CARTESIAN_POINT('Ctrl Pts',(-8.27600348989907,1.20454703673217,27.6122408161699));
#16859=CARTESIAN_POINT('Ctrl Pts',(-7.97209482031962,1.10563290540046,27.6002376293806));
#16860=CARTESIAN_POINT('Ctrl Pts',(-7.74204705371953,0.915087963995678,
27.5882344425913));
#16861=CARTESIAN_POINT('Ctrl Pts',(-7.51199928711944,0.724543022590897,
27.5762312558019));
#16862=CARTESIAN_POINT('Ctrl Pts',(-7.35822688079583,0.444367128060145,
27.5642280690126));
#16863=CARTESIAN_POINT('Ctrl Pts',(-7.321025609758,0.147979855988942,27.5522248822233));
#16864=CARTESIAN_POINT('Ctrl Pts',(-7.28382433872017,-0.148407416082262,
27.540221695434));
#16865=CARTESIAN_POINT('Ctrl Pts',(-7.36358464744688,-0.457895344723237,
27.5282185086447));
#16866=CARTESIAN_POINT('Ctrl Pts',(-7.5394054943796,-0.699383189958769,
27.5162153218554));
#16867=CARTESIAN_POINT('Ctrl Pts',(-7.71522634131232,-0.940871035194301,
27.504212135066));
#16868=CARTESIAN_POINT('Ctrl Pts',(-7.98526240565906,-1.11182427083138,
27.4922089482767));
#16869=CARTESIAN_POINT('Ctrl Pts',(-8.27875123560243,-1.16744491727771,
27.4802057614874));
#16870=CARTESIAN_POINT('Ctrl Pts',(-8.57224006554581,-1.22306556372403,
27.4682025746981));
#16871=CARTESIAN_POINT('Ctrl Pts',(-8.88610136060064,-1.16276985666983,
27.4561993879088));
#16872=CARTESIAN_POINT('Ctrl Pts',(-9.138088348202,-1.00235817476282,27.4441962011195));
#16873=CARTESIAN_POINT('Ctrl Pts',(-9.39007533580335,-0.841946492855811,
27.4321930143301));
#16874=CARTESIAN_POINT('Ctrl Pts',(-9.57754329642196,-0.5831024306018,27.4201898275408));
#16875=CARTESIAN_POINT('Ctrl Pts',(-9.65136659729221,-0.293655596345039,
27.4081866407515));
#16876=CARTESIAN_POINT('Ctrl Pts',(-9.67581103310565,-0.197813707971212,
27.404212135066));
#16877=CARTESIAN_POINT('Ctrl Pts',(-9.68822500000013,-0.098910050090984,
27.4002376293806));
#16878=CARTESIAN_POINT('Ctrl Pts',(-9.688225,1.5049073098794E-12,27.3962631236951));
#16879=CARTESIAN_POINT('Ctrl Pts',(-9.688225,-2.12330153459561E-13,27.3537368763049));
#16880=CARTESIAN_POINT('Ctrl Pts',(-9.68822499999995,-0.298712821306295,
27.3657400630942));
#16881=CARTESIAN_POINT('Ctrl Pts',(-9.57054245632576,-0.595858078271698,
27.3777432498835));
#16882=CARTESIAN_POINT('Ctrl Pts',(-9.36601586214923,-0.813569405232849,
27.3897464366728));
#16883=CARTESIAN_POINT('Ctrl Pts',(-9.16148926797269,-1.031280732194,27.4017496234621));
#16884=CARTESIAN_POINT('Ctrl Pts',(-8.87226522412831,-1.1672731484714,27.4137528102514));
#16885=CARTESIAN_POINT('Ctrl Pts',(-8.57413435701436,-1.18591009260191,
27.4257559970408));
#16886=CARTESIAN_POINT('Ctrl Pts',(-8.27600348990041,-1.20454703673242,
27.4377591838301));
#16887=CARTESIAN_POINT('Ctrl Pts',(-7.97209482032084,-1.10563290540105,
27.4497623706194));
#16888=CARTESIAN_POINT('Ctrl Pts',(-7.74204705372055,-0.915087963996519,
27.4617655574087));
#16889=CARTESIAN_POINT('Ctrl Pts',(-7.51199928712025,-0.724543022591993,
27.473768744198));
#16890=CARTESIAN_POINT('Ctrl Pts',(-7.35822688079632,-0.444367128061411,
27.4857719309873));
#16891=CARTESIAN_POINT('Ctrl Pts',(-7.32102560975817,-0.14797985599025,
27.4977751177767));
#16892=CARTESIAN_POINT('Ctrl Pts',(-7.28382433872001,0.148407416080912,
27.509778304566));
#16893=CARTESIAN_POINT('Ctrl Pts',(-7.36358464744637,0.457895344721976,
27.5217814913553));
#16894=CARTESIAN_POINT('Ctrl Pts',(-7.53940549437883,0.699383189957703,
27.5337846781446));
#16895=CARTESIAN_POINT('Ctrl Pts',(-7.71522634131128,0.940871035193431,
27.5457878649339));
#16896=CARTESIAN_POINT('Ctrl Pts',(-7.98526240565782,1.11182427083081,27.5577910517232));
#16897=CARTESIAN_POINT('Ctrl Pts',(-8.27875123560114,1.16744491727746,27.5697942385126));
#16898=CARTESIAN_POINT('Ctrl Pts',(-8.57224006554445,1.22306556372411,27.5817974253019));
#16899=CARTESIAN_POINT('Ctrl Pts',(-8.88610136059935,1.16276985667026,27.5938006120912));
#16900=CARTESIAN_POINT('Ctrl Pts',(-9.13808834820088,1.00235817476353,27.6058037988805));
#16901=CARTESIAN_POINT('Ctrl Pts',(-9.39007533580241,0.841946492856798,
27.6178069856698));
#16902=CARTESIAN_POINT('Ctrl Pts',(-9.57754329642132,0.583102430602995,
27.6298101724592));
#16903=CARTESIAN_POINT('Ctrl Pts',(-9.65136659729188,0.293655596346317,
27.6418133592485));
#16904=CARTESIAN_POINT('Ctrl Pts',(-9.67581103310542,0.19781370797256,27.6457878649339));
#16905=CARTESIAN_POINT('Ctrl Pts',(-9.688225,0.0989100500923923,27.6497623706194));
#16906=CARTESIAN_POINT('Ctrl Pts',(-9.688225,-5.15698594938385E-14,27.6537368763048));
#16907=CARTESIAN_POINT('Origin',(-8.5,0.,1.8));
#16908=CARTESIAN_POINT('',(-9.688225,1.55619961361708E-12,27.9962631236951));
#16909=CARTESIAN_POINT('',(-9.688225,-1.61037849721879E-13,27.9537368763048));
#16910=CARTESIAN_POINT('',(-9.688225,-1.45515594291686E-16,1.8));
#16911=CARTESIAN_POINT('Ctrl Pts',(-9.688225,1.55619961361708E-12,27.9962631236951));
#16912=CARTESIAN_POINT('Ctrl Pts',(-9.68822499999961,0.298712821307638,
27.9842599369058));
#16913=CARTESIAN_POINT('Ctrl Pts',(-9.57054245632509,0.595858078272909,
27.9722567501165));
#16914=CARTESIAN_POINT('Ctrl Pts',(-9.36601586214831,0.813569405233829,
27.9602535633272));
#16915=CARTESIAN_POINT('Ctrl Pts',(-9.16148926797152,1.03128073219475,27.9482503765378));
#16916=CARTESIAN_POINT('Ctrl Pts',(-8.87226522412699,1.16727314847182,27.9362471897485));
#16917=CARTESIAN_POINT('Ctrl Pts',(-8.57413435701302,1.18591009260199,27.9242440029592));
#16918=CARTESIAN_POINT('Ctrl Pts',(-8.27600348989905,1.20454703673216,27.9122408161699));
#16919=CARTESIAN_POINT('Ctrl Pts',(-7.97209482031959,1.10563290540045,27.9002376293806));
#16920=CARTESIAN_POINT('Ctrl Pts',(-7.74204705371951,0.915087963995662,
27.8882344425913));
#16921=CARTESIAN_POINT('Ctrl Pts',(-7.51199928711943,0.724543022590876,
27.8762312558019));
#16922=CARTESIAN_POINT('Ctrl Pts',(-7.35822688079582,0.44436712806012,27.8642280690126));
#16923=CARTESIAN_POINT('Ctrl Pts',(-7.321025609758,0.147979855988916,27.8522248822233));
#16924=CARTESIAN_POINT('Ctrl Pts',(-7.28382433872017,-0.148407416082288,
27.840221695434));
#16925=CARTESIAN_POINT('Ctrl Pts',(-7.36358464744689,-0.457895344723262,
27.8282185086447));
#16926=CARTESIAN_POINT('Ctrl Pts',(-7.53940549437962,-0.69938318995879,
27.8162153218554));
#16927=CARTESIAN_POINT('Ctrl Pts',(-7.71522634131234,-0.940871035194318,
27.804212135066));
#16928=CARTESIAN_POINT('Ctrl Pts',(-7.98526240565908,-1.1118242708314,27.7922089482767));
#16929=CARTESIAN_POINT('Ctrl Pts',(-8.27875123560246,-1.16744491727771,
27.7802057614874));
#16930=CARTESIAN_POINT('Ctrl Pts',(-8.57224006554584,-1.22306556372403,
27.7682025746981));
#16931=CARTESIAN_POINT('Ctrl Pts',(-8.88610136060067,-1.16276985666982,
27.7561993879088));
#16932=CARTESIAN_POINT('Ctrl Pts',(-9.13808834820202,-1.00235817476281,
27.7441962011195));
#16933=CARTESIAN_POINT('Ctrl Pts',(-9.39007533580337,-0.841946492855791,
27.7321930143301));
#16934=CARTESIAN_POINT('Ctrl Pts',(-9.57754329642198,-0.583102430601777,
27.7201898275408));
#16935=CARTESIAN_POINT('Ctrl Pts',(-9.65136659729222,-0.293655596345015,
27.7081866407515));
#16936=CARTESIAN_POINT('Ctrl Pts',(-9.67581103310565,-0.197813707971187,
27.704212135066));
#16937=CARTESIAN_POINT('Ctrl Pts',(-9.68822500000013,-0.0989100500909583,
27.7002376293806));
#16938=CARTESIAN_POINT('Ctrl Pts',(-9.688225,1.53055346174824E-12,27.6962631236951));
#16939=CARTESIAN_POINT('Ctrl Pts',(-9.688225,-5.15698594938385E-14,27.6537368763048));
#16940=CARTESIAN_POINT('Ctrl Pts',(-9.68822499999999,-0.298712821306134,
27.6657400630942));
#16941=CARTESIAN_POINT('Ctrl Pts',(-9.57054245632584,-0.595858078271553,
27.6777432498835));
#16942=CARTESIAN_POINT('Ctrl Pts',(-9.36601586214934,-0.813569405232732,
27.6897464366728));
#16943=CARTESIAN_POINT('Ctrl Pts',(-9.16148926797283,-1.03128073219391,
27.7017496234621));
#16944=CARTESIAN_POINT('Ctrl Pts',(-8.87226522412847,-1.16727314847135,
27.7137528102514));
#16945=CARTESIAN_POINT('Ctrl Pts',(-8.57413435701452,-1.1859100926019,27.7257559970407));
#16946=CARTESIAN_POINT('Ctrl Pts',(-8.27600348990057,-1.20454703673245,
27.7377591838301));
#16947=CARTESIAN_POINT('Ctrl Pts',(-7.97209482032099,-1.10563290540112,
27.7497623706194));
#16948=CARTESIAN_POINT('Ctrl Pts',(-7.74204705372067,-0.915087963996622,
27.7617655574087));
#16949=CARTESIAN_POINT('Ctrl Pts',(-7.51199928712035,-0.724543022592127,
27.773768744198));
#16950=CARTESIAN_POINT('Ctrl Pts',(-7.35822688079638,-0.444367128061566,
27.7857719309873));
#16951=CARTESIAN_POINT('Ctrl Pts',(-7.32102560975819,-0.147979855990409,
27.7977751177767));
#16952=CARTESIAN_POINT('Ctrl Pts',(-7.28382433871999,0.148407416080748,
27.809778304566));
#16953=CARTESIAN_POINT('Ctrl Pts',(-7.36358464744631,0.457895344721823,
27.8217814913553));
#16954=CARTESIAN_POINT('Ctrl Pts',(-7.53940549437873,0.699383189957574,
27.8337846781446));
#16955=CARTESIAN_POINT('Ctrl Pts',(-7.71522634131115,0.940871035193324,
27.8457878649339));
#16956=CARTESIAN_POINT('Ctrl Pts',(-7.98526240565767,1.11182427083074,27.8577910517232));
#16957=CARTESIAN_POINT('Ctrl Pts',(-8.27875123560098,1.16744491727743,27.8697942385126));
#16958=CARTESIAN_POINT('Ctrl Pts',(-8.57224006554429,1.22306556372412,27.8817974253019));
#16959=CARTESIAN_POINT('Ctrl Pts',(-8.88610136059919,1.16276985667031,27.8938006120912));
#16960=CARTESIAN_POINT('Ctrl Pts',(-9.13808834820075,1.00235817476361,27.9058037988805));
#16961=CARTESIAN_POINT('Ctrl Pts',(-9.3900753358023,0.841946492856918,27.9178069856698));
#16962=CARTESIAN_POINT('Ctrl Pts',(-9.57754329642124,0.583102430603141,
27.9298101724591));
#16963=CARTESIAN_POINT('Ctrl Pts',(-9.65136659729184,0.293655596346473,
27.9418133592485));
#16964=CARTESIAN_POINT('Ctrl Pts',(-9.67581103310542,0.197813707972632,
27.9457878649339));
#16965=CARTESIAN_POINT('Ctrl Pts',(-9.68822500000001,0.0989100500923729,
27.9497623706194));
#16966=CARTESIAN_POINT('Ctrl Pts',(-9.688225,-1.61037849721879E-13,27.9537368763048));
#16967=CARTESIAN_POINT('Origin',(-8.5,0.,1.8));
#16968=CARTESIAN_POINT('',(-9.688225,1.58184576548592E-12,28.2962631236951));
#16969=CARTESIAN_POINT('',(-9.688225,-1.35447209004269E-13,28.2537368763048));
#16970=CARTESIAN_POINT('',(-9.688225,-1.45515594291686E-16,1.8));
#16971=CARTESIAN_POINT('Ctrl Pts',(-9.688225,1.71684888528034E-12,28.2962631236951));
#16972=CARTESIAN_POINT('Ctrl Pts',(-9.68822499999957,0.298712821307844,
28.2842599369058));
#16973=CARTESIAN_POINT('Ctrl Pts',(-9.57054245632497,0.595858078273142,
28.2722567501165));
#16974=CARTESIAN_POINT('Ctrl Pts',(-9.3660158621481,0.813569405234045,28.2602535633272));
#16975=CARTESIAN_POINT('Ctrl Pts',(-9.16148926797123,1.03128073219495,28.2482503765378));
#16976=CARTESIAN_POINT('Ctrl Pts',(-8.87226522412661,1.16727314847196,28.2362471897485));
#16977=CARTESIAN_POINT('Ctrl Pts',(-8.57413435701259,1.18591009260202,28.2242440029592));
#16978=CARTESIAN_POINT('Ctrl Pts',(-8.27600348989856,1.20454703673208,28.2122408161699));
#16979=CARTESIAN_POINT('Ctrl Pts',(-7.9720948203191,1.10563290540023,28.2002376293806));
#16980=CARTESIAN_POINT('Ctrl Pts',(-7.74204705371907,0.915087963995301,
28.1882344425912));
#16981=CARTESIAN_POINT('Ctrl Pts',(-7.51199928711905,0.724543022590376,
28.1762312558019));
#16982=CARTESIAN_POINT('Ctrl Pts',(-7.35822688079556,0.444367128059491,
28.1642280690126));
#16983=CARTESIAN_POINT('Ctrl Pts',(-7.32102560975791,0.147979855988221,
28.1522248822233));
#16984=CARTESIAN_POINT('Ctrl Pts',(-7.28382433872026,-0.14840741608305,
28.140221695434));
#16985=CARTESIAN_POINT('Ctrl Pts',(-7.36358464744719,-0.457895344724025,
28.1282185086446));
#16986=CARTESIAN_POINT('Ctrl Pts',(-7.53940549438011,-0.699383189959466,
28.1162153218553));
#16987=CARTESIAN_POINT('Ctrl Pts',(-7.71522634131303,-0.940871035194907,
28.104212135066));
#16988=CARTESIAN_POINT('Ctrl Pts',(-7.98526240565995,-1.11182427083181,
28.0922089482767));
#16989=CARTESIAN_POINT('Ctrl Pts',(-8.27875123560341,-1.16744491727789,
28.0802057614874));
#16990=CARTESIAN_POINT('Ctrl Pts',(-8.57224006554688,-1.22306556372398,
28.068202574698));
#16991=CARTESIAN_POINT('Ctrl Pts',(-8.88610136060171,-1.16276985666948,
28.0561993879087));
#16992=CARTESIAN_POINT('Ctrl Pts',(-9.13808834820295,-1.00235817476221,
28.0441962011194));
#16993=CARTESIAN_POINT('Ctrl Pts',(-9.39007533580419,-0.841946492854939,
28.0321930143301));
#16994=CARTESIAN_POINT('Ctrl Pts',(-9.57754329642258,-0.583102430600695,
28.0201898275408));
#16995=CARTESIAN_POINT('Ctrl Pts',(-9.65136659729252,-0.293655596343812,
28.0081866407515));
#16996=CARTESIAN_POINT('Ctrl Pts',(-9.67581103310576,-0.197813707970351,
28.004212135066));
#16997=CARTESIAN_POINT('Ctrl Pts',(-9.68822500000013,-0.0989100500905275,
28.0002376293806));
#16998=CARTESIAN_POINT('Ctrl Pts',(-9.688225,1.55619961361708E-12,27.9962631236951));
#16999=CARTESIAN_POINT('Ctrl Pts',(-9.688225,-1.61037849721879E-13,27.9537368763048));
#17000=CARTESIAN_POINT('Ctrl Pts',(-9.68822499999996,-0.298712821306243,
27.9657400630942));
#17001=CARTESIAN_POINT('Ctrl Pts',(-9.57054245632579,-0.595858078271651,
27.9777432498835));
#17002=CARTESIAN_POINT('Ctrl Pts',(-9.36601586214926,-0.813569405232812,
27.9897464366728));
#17003=CARTESIAN_POINT('Ctrl Pts',(-9.16148926797273,-1.03128073219397,
28.0017496234621));
#17004=CARTESIAN_POINT('Ctrl Pts',(-8.87226522412836,-1.16727314847139,
28.0137528102514));
#17005=CARTESIAN_POINT('Ctrl Pts',(-8.57413435701441,-1.18591009260191,
28.0257559970408));
#17006=CARTESIAN_POINT('Ctrl Pts',(-8.27600348990046,-1.20454703673243,
28.0377591838301));
#17007=CARTESIAN_POINT('Ctrl Pts',(-7.97209482032089,-1.10563290540107,
28.0497623706194));
#17008=CARTESIAN_POINT('Ctrl Pts',(-7.74204705372058,-0.915087963996552,
28.0617655574087));
#17009=CARTESIAN_POINT('Ctrl Pts',(-7.51199928712028,-0.724543022592035,
28.073768744198));
#17010=CARTESIAN_POINT('Ctrl Pts',(-7.35822688079634,-0.444367128061461,
28.0857719309873));
#17011=CARTESIAN_POINT('Ctrl Pts',(-7.32102560975817,-0.1479798559903,28.0977751177767));
#17012=CARTESIAN_POINT('Ctrl Pts',(-7.28382433872,0.14840741608086,28.109778304566));
#17013=CARTESIAN_POINT('Ctrl Pts',(-7.36358464744635,0.457895344721927,
28.1217814913553));
#17014=CARTESIAN_POINT('Ctrl Pts',(-7.5394054943788,0.699383189957662,28.1337846781446));
#17015=CARTESIAN_POINT('Ctrl Pts',(-7.71522634131124,0.940871035193397,
28.1457878649339));
#17016=CARTESIAN_POINT('Ctrl Pts',(-7.98526240565778,1.11182427083079,28.1577910517232));
#17017=CARTESIAN_POINT('Ctrl Pts',(-8.27875123560109,1.16744491727745,28.1697942385126));
#17018=CARTESIAN_POINT('Ctrl Pts',(-8.5722400655444,1.22306556372411,28.1817974253019));
#17019=CARTESIAN_POINT('Ctrl Pts',(-8.8861013605993,1.16276985667027,28.1938006120912));
#17020=CARTESIAN_POINT('Ctrl Pts',(-9.13808834820084,1.00235817476355,28.2058037988805));
#17021=CARTESIAN_POINT('Ctrl Pts',(-9.39007533580238,0.841946492856836,
28.2178069856698));
#17022=CARTESIAN_POINT('Ctrl Pts',(-9.57754329642129,0.583102430603042,
28.2298101724591));
#17023=CARTESIAN_POINT('Ctrl Pts',(-9.65136659729187,0.293655596346366,
28.2418133592485));
#17024=CARTESIAN_POINT('Ctrl Pts',(-9.67581103310542,0.197813707972567,
28.2457878649339));
#17025=CARTESIAN_POINT('Ctrl Pts',(-9.68822500000001,0.0989100500923534,
28.2497623706194));
#17026=CARTESIAN_POINT('Ctrl Pts',(-9.688225,-1.35447209004269E-13,28.2537368763048));
#17027=CARTESIAN_POINT('Origin',(-8.5,0.,1.8));
#17028=CARTESIAN_POINT('',(-9.688225,1.6073808950523E-12,28.5962631236951));
#17029=CARTESIAN_POINT('',(-9.688225,-1.09801057135428E-13,28.5537368763048));
#17030=CARTESIAN_POINT('',(-9.688225,-1.45515594291686E-16,1.8));
#17031=CARTESIAN_POINT('Ctrl Pts',(-9.688225,1.74249503714918E-12,28.5962631236951));
#17032=CARTESIAN_POINT('Ctrl Pts',(-9.68822499999956,0.29871282130778,28.5842599369058));
#17033=CARTESIAN_POINT('Ctrl Pts',(-9.57054245632503,0.595858078272988,
28.5722567501165));
#17034=CARTESIAN_POINT('Ctrl Pts',(-9.36601586214827,0.813569405233866,
28.5602535633272));
#17035=CARTESIAN_POINT('Ctrl Pts',(-9.16148926797151,1.03128073219475,28.5482503765379));
#17036=CARTESIAN_POINT('Ctrl Pts',(-8.87226522412703,1.1672731484718,28.5362471897485));
#17037=CARTESIAN_POINT('Ctrl Pts',(-8.5741343570131,1.18591009260199,28.5242440029592));
#17038=CARTESIAN_POINT('Ctrl Pts',(-8.27600348989918,1.20454703673218,28.5122408161699));
#17039=CARTESIAN_POINT('Ctrl Pts',(-7.97209482031976,1.10563290540052,28.5002376293806));
#17040=CARTESIAN_POINT('Ctrl Pts',(-7.74204705371968,0.915087963995802,
28.4882344425913));
#17041=CARTESIAN_POINT('Ctrl Pts',(-7.5119992871196,0.724543022591086,28.476231255802));
#17042=CARTESIAN_POINT('Ctrl Pts',(-7.35822688079595,0.444367128060416,
28.4642280690126));
#17043=CARTESIAN_POINT('Ctrl Pts',(-7.32102560975804,0.147979855989267,
28.4522248822233));
#17044=CARTESIAN_POINT('Ctrl Pts',(-7.28382433872014,-0.148407416081881,
28.440221695434));
#17045=CARTESIAN_POINT('Ctrl Pts',(-7.36358464744673,-0.45789534472283,
28.4282185086447));
#17046=CARTESIAN_POINT('Ctrl Pts',(-7.53940549437933,-0.699383189958395,
28.4162153218554));
#17047=CARTESIAN_POINT('Ctrl Pts',(-7.71522634131193,-0.940871035193959,
28.4042121350661));
#17048=CARTESIAN_POINT('Ctrl Pts',(-7.98526240565854,-1.11182427083113,
28.3922089482767));
#17049=CARTESIAN_POINT('Ctrl Pts',(-8.27875123560185,-1.1674449172776,28.3802057614874));
#17050=CARTESIAN_POINT('Ctrl Pts',(-8.57224006554515,-1.22306556372406,
28.3682025746981));
#17051=CARTESIAN_POINT('Ctrl Pts',(-8.88610136059996,-1.16276985667004,
28.3561993879088));
#17052=CARTESIAN_POINT('Ctrl Pts',(-9.13808834820138,-1.00235817476321,
28.3441962011195));
#17053=CARTESIAN_POINT('Ctrl Pts',(-9.39007533580279,-0.841946492856384,
28.3321930143302));
#17054=CARTESIAN_POINT('Ctrl Pts',(-9.57754329642155,-0.583102430602544,
28.3201898275409));
#17055=CARTESIAN_POINT('Ctrl Pts',(-9.65136659729199,-0.293655596345881,
28.3081866407515));
#17056=CARTESIAN_POINT('Ctrl Pts',(-9.6758110331056,-0.197813707971723,
28.3042121350661));
#17057=CARTESIAN_POINT('Ctrl Pts',(-9.68822500000014,-0.0989100500911323,
28.3002376293806));
#17058=CARTESIAN_POINT('Ctrl Pts',(-9.688225,1.71684888528034E-12,28.2962631236951));
#17059=CARTESIAN_POINT('Ctrl Pts',(-9.688225,-1.35447209004269E-13,28.2537368763048));
#17060=CARTESIAN_POINT('Ctrl Pts',(-9.68822499999997,-0.298712821306263,
28.2657400630942));
#17061=CARTESIAN_POINT('Ctrl Pts',(-9.57054245632576,-0.595858078271717,
28.2777432498835));
#17062=CARTESIAN_POINT('Ctrl Pts',(-9.36601586214919,-0.813569405232892,
28.2897464366728));
#17063=CARTESIAN_POINT('Ctrl Pts',(-9.16148926797261,-1.03128073219407,
28.3017496234621));
#17064=CARTESIAN_POINT('Ctrl Pts',(-8.87226522412817,-1.16727314847146,
28.3137528102514));
#17065=CARTESIAN_POINT('Ctrl Pts',(-8.57413435701417,-1.18591009260192,
28.3257559970408));
#17066=CARTESIAN_POINT('Ctrl Pts',(-8.27600348990017,-1.20454703673238,
28.3377591838301));
#17067=CARTESIAN_POINT('Ctrl Pts',(-7.97209482032057,-1.10563290540093,
28.3497623706194));
#17068=CARTESIAN_POINT('Ctrl Pts',(-7.74204705372029,-0.91508796399631,
28.3617655574087));
#17069=CARTESIAN_POINT('Ctrl Pts',(-7.51199928712001,-0.724543022591691,
28.373768744198));
#17070=CARTESIAN_POINT('Ctrl Pts',(-7.35822688079616,-0.444367128061011,
28.3857719309874));
#17071=CARTESIAN_POINT('Ctrl Pts',(-7.32102560975811,-0.14797985598979,
28.3977751177767));
#17072=CARTESIAN_POINT('Ctrl Pts',(-7.28382433872006,0.148407416081431,
28.409778304566));
#17073=CARTESIAN_POINT('Ctrl Pts',(-7.36358464744658,0.457895344722512,
28.4217814913553));
#17074=CARTESIAN_POINT('Ctrl Pts',(-7.53940549437918,0.699383189958187,
28.4337846781446));
#17075=CARTESIAN_POINT('Ctrl Pts',(-7.71522634131178,0.940871035193862,
28.445787864934));
#17076=CARTESIAN_POINT('Ctrl Pts',(-7.98526240565847,1.11182427083112,28.4577910517233));
#17077=CARTESIAN_POINT('Ctrl Pts',(-8.27875123560186,1.1674449172776,28.4697942385126));
#17078=CARTESIAN_POINT('Ctrl Pts',(-8.57224006554525,1.22306556372407,28.4817974253019));
#17079=CARTESIAN_POINT('Ctrl Pts',(-8.88610136060016,1.16276985667,28.4938006120912));
#17080=CARTESIAN_POINT('Ctrl Pts',(-9.13808834820161,1.00235817476306,28.5058037988805));
#17081=CARTESIAN_POINT('Ctrl Pts',(-9.39007533580306,0.841946492856123,
28.5178069856699));
#17082=CARTESIAN_POINT('Ctrl Pts',(-9.5775432964218,0.583102430602129,28.5298101724592));
#17083=CARTESIAN_POINT('Ctrl Pts',(-9.65136659729213,0.293655596345344,
28.5418133592485));
#17084=CARTESIAN_POINT('Ctrl Pts',(-9.67581103310551,0.197813707971872,
28.545787864934));
#17085=CARTESIAN_POINT('Ctrl Pts',(-9.68822500000001,0.0989100500920189,
28.5497623706194));
#17086=CARTESIAN_POINT('Ctrl Pts',(-9.688225,-1.09801057135428E-13,28.5537368763048));
#17087=CARTESIAN_POINT('Origin',(-8.5,0.,1.8));
#17088=CARTESIAN_POINT('',(-9.688225,1.63313806922361E-12,28.8962631236951));
#17089=CARTESIAN_POINT('',(-9.688225,-8.42104164178181E-14,28.8537368763048));
#17090=CARTESIAN_POINT('',(-9.688225,-1.45515594291686E-16,1.8));
#17091=CARTESIAN_POINT('Ctrl Pts',(-9.688225,1.63313806922361E-12,28.8962631236951));
#17092=CARTESIAN_POINT('Ctrl Pts',(-9.68822499999959,0.29871282130767,28.8842599369058));
#17093=CARTESIAN_POINT('Ctrl Pts',(-9.57054245632509,0.595858078272889,
28.8722567501165));
#17094=CARTESIAN_POINT('Ctrl Pts',(-9.36601586214835,0.813569405233787,
28.8602535633272));
#17095=CARTESIAN_POINT('Ctrl Pts',(-9.16148926797161,1.03128073219468,28.8482503765379));
#17096=CARTESIAN_POINT('Ctrl Pts',(-8.87226522412713,1.16727314847177,28.8362471897485));
#17097=CARTESIAN_POINT('Ctrl Pts',(-8.57413435701321,1.18591009260198,28.8242440029592));
#17098=CARTESIAN_POINT('Ctrl Pts',(-8.27600348989929,1.2045470367322,28.8122408161699));
#17099=CARTESIAN_POINT('Ctrl Pts',(-7.97209482031986,1.10563290540057,28.8002376293806));
#17100=CARTESIAN_POINT('Ctrl Pts',(-7.74204705371976,0.915087963995872,
28.7882344425913));
#17101=CARTESIAN_POINT('Ctrl Pts',(-7.51199928711966,0.724543022591177,
28.776231255802));
#17102=CARTESIAN_POINT('Ctrl Pts',(-7.35822688079599,0.444367128060521,
28.7642280690126));
#17103=CARTESIAN_POINT('Ctrl Pts',(-7.32102560975806,0.147979855989376,
28.7522248822233));
#17104=CARTESIAN_POINT('Ctrl Pts',(-7.28382433872012,-0.148407416081769,
28.740221695434));
#17105=CARTESIAN_POINT('Ctrl Pts',(-7.36358464744669,-0.457895344722725,
28.7282185086447));
#17106=CARTESIAN_POINT('Ctrl Pts',(-7.53940549437926,-0.699383189958306,
28.7162153218554));
#17107=CARTESIAN_POINT('Ctrl Pts',(-7.71522634131184,-0.940871035193887,
28.7042121350661));
#17108=CARTESIAN_POINT('Ctrl Pts',(-7.98526240565844,-1.11182427083109,
28.6922089482768));
#17109=CARTESIAN_POINT('Ctrl Pts',(-8.27875123560174,-1.16744491727757,
28.6802057614874));
#17110=CARTESIAN_POINT('Ctrl Pts',(-8.57224006554504,-1.22306556372406,
28.6682025746981));
#17111=CARTESIAN_POINT('Ctrl Pts',(-8.88610136059985,-1.16276985667008,
28.6561993879088));
#17112=CARTESIAN_POINT('Ctrl Pts',(-9.13808834820128,-1.00235817476327,
28.6441962011195));
#17113=CARTESIAN_POINT('Ctrl Pts',(-9.39007533580271,-0.841946492856467,
28.6321930143302));
#17114=CARTESIAN_POINT('Ctrl Pts',(-9.5775432964215,-0.583102430602644,
28.6201898275409));
#17115=CARTESIAN_POINT('Ctrl Pts',(-9.65136659729197,-0.293655596345987,
28.6081866407515));
#17116=CARTESIAN_POINT('Ctrl Pts',(-9.67581103310559,-0.197813707971787,
28.6042121350661));
#17117=CARTESIAN_POINT('Ctrl Pts',(-9.68822500000015,-0.0989100500911517,
28.6002376293806));
#17118=CARTESIAN_POINT('Ctrl Pts',(-9.688225,1.74249503714918E-12,28.5962631236951));
#17119=CARTESIAN_POINT('Ctrl Pts',(-9.688225,-1.09801057135428E-13,28.5537368763048));
#17120=CARTESIAN_POINT('Ctrl Pts',(-9.68822499999997,-0.298712821306192,
28.5657400630942));
#17121=CARTESIAN_POINT('Ctrl Pts',(-9.57054245632581,-0.595858078271605,
28.5777432498835));
#17122=CARTESIAN_POINT('Ctrl Pts',(-9.3660158621493,-0.813569405232775,
28.5897464366728));
#17123=CARTESIAN_POINT('Ctrl Pts',(-9.16148926797278,-1.03128073219394,
28.6017496234621));
#17124=CARTESIAN_POINT('Ctrl Pts',(-8.87226522412841,-1.16727314847137,
28.6137528102514));
#17125=CARTESIAN_POINT('Ctrl Pts',(-8.57413435701446,-1.1859100926019,28.6257559970408));
#17126=CARTESIAN_POINT('Ctrl Pts',(-8.27600348990051,-1.20454703673244,
28.6377591838301));
#17127=CARTESIAN_POINT('Ctrl Pts',(-7.97209482032094,-1.10563290540109,
28.6497623706194));
#17128=CARTESIAN_POINT('Ctrl Pts',(-7.74204705372062,-0.915087963996584,
28.6617655574087));
#17129=CARTESIAN_POINT('Ctrl Pts',(-7.51199928712031,-0.724543022592078,
28.673768744198));
#17130=CARTESIAN_POINT('Ctrl Pts',(-7.35822688079636,-0.44436712806151,
28.6857719309873));
#17131=CARTESIAN_POINT('Ctrl Pts',(-7.32102560975818,-0.147979855990351,
28.6977751177767));
#17132=CARTESIAN_POINT('Ctrl Pts',(-7.28382433872,0.148407416080807,28.709778304566));
#17133=CARTESIAN_POINT('Ctrl Pts',(-7.36358464744633,0.457895344721878,
28.7217814913553));
#17134=CARTESIAN_POINT('Ctrl Pts',(-7.53940549437877,0.699383189957621,
28.7337846781446));
#17135=CARTESIAN_POINT('Ctrl Pts',(-7.7152263413112,0.940871035193363,28.7457878649339));
#17136=CARTESIAN_POINT('Ctrl Pts',(-7.98526240565773,1.11182427083077,28.7577910517232));
#17137=CARTESIAN_POINT('Ctrl Pts',(-8.27875123560104,1.16744491727744,28.7697942385126));
#17138=CARTESIAN_POINT('Ctrl Pts',(-8.57224006554435,1.22306556372412,28.7817974253019));
#17139=CARTESIAN_POINT('Ctrl Pts',(-8.88610136059925,1.16276985667029,28.7938006120912));
#17140=CARTESIAN_POINT('Ctrl Pts',(-9.1380883482008,1.00235817476358,28.8058037988805));
#17141=CARTESIAN_POINT('Ctrl Pts',(-9.39007533580234,0.841946492856875,
28.8178069856698));
#17142=CARTESIAN_POINT('Ctrl Pts',(-9.57754329642127,0.583102430603088,
28.8298101724591));
#17143=CARTESIAN_POINT('Ctrl Pts',(-9.65136659729186,0.293655596346416,
28.8418133592485));
#17144=CARTESIAN_POINT('Ctrl Pts',(-9.67581103310541,0.197813707972618,
28.8457878649339));
#17145=CARTESIAN_POINT('Ctrl Pts',(-9.68822500000001,0.0989100500924047,
28.8497623706194));
#17146=CARTESIAN_POINT('Ctrl Pts',(-9.688225,-8.42104164178181E-14,28.8537368763048));
#17147=CARTESIAN_POINT('Origin',(-8.5,0.,1.8));
#17148=CARTESIAN_POINT('',(-9.688225,1.65867319878998E-12,29.1962631236951));
#17149=CARTESIAN_POINT('',(-9.688225,-5.8564264548977E-14,29.1537368763048));
#17150=CARTESIAN_POINT('',(-9.688225,-1.45515594291686E-16,1.8));
#17151=CARTESIAN_POINT('Ctrl Pts',(-9.688225,1.65867319878998E-12,29.1962631236951));
#17152=CARTESIAN_POINT('Ctrl Pts',(-9.68822499999958,0.298712821307696,
29.1842599369058));
#17153=CARTESIAN_POINT('Ctrl Pts',(-9.57054245632508,0.595858078272912,
29.1722567501165));
#17154=CARTESIAN_POINT('Ctrl Pts',(-9.36601586214833,0.813569405233805,
29.1602535633272));
#17155=CARTESIAN_POINT('Ctrl Pts',(-9.16148926797158,1.0312807321947,29.1482503765379));
#17156=CARTESIAN_POINT('Ctrl Pts',(-8.87226522412711,1.16727314847177,29.1362471897485));
#17157=CARTESIAN_POINT('Ctrl Pts',(-8.57413435701319,1.18591009260198,29.1242440029592));
#17158=CARTESIAN_POINT('Ctrl Pts',(-8.27600348989926,1.20454703673219,29.1122408161699));
#17159=CARTESIAN_POINT('Ctrl Pts',(-7.97209482031984,1.10563290540055,29.1002376293806));
#17160=CARTESIAN_POINT('Ctrl Pts',(-7.74204705371974,0.915087963995855,
29.0882344425913));
#17161=CARTESIAN_POINT('Ctrl Pts',(-7.51199928711965,0.724543022591156,
29.076231255802));
#17162=CARTESIAN_POINT('Ctrl Pts',(-7.35822688079598,0.444367128060496,
29.0642280690126));
#17163=CARTESIAN_POINT('Ctrl Pts',(-7.32102560975805,0.147979855989351,
29.0522248822233));
#17164=CARTESIAN_POINT('Ctrl Pts',(-7.28382433872013,-0.148407416081795,
29.040221695434));
#17165=CARTESIAN_POINT('Ctrl Pts',(-7.3635846474467,-0.45789534472275,29.0282185086447));
#17166=CARTESIAN_POINT('Ctrl Pts',(-7.53940549437928,-0.699383189958327,
29.0162153218554));
#17167=CARTESIAN_POINT('Ctrl Pts',(-7.71522634131186,-0.940871035193904,
29.0042121350661));
#17168=CARTESIAN_POINT('Ctrl Pts',(-7.98526240565846,-1.1118242708311,28.9922089482767));
#17169=CARTESIAN_POINT('Ctrl Pts',(-8.27875123560176,-1.16744491727758,
28.9802057614874));
#17170=CARTESIAN_POINT('Ctrl Pts',(-8.57224006554507,-1.22306556372406,
28.9682025746981));
#17171=CARTESIAN_POINT('Ctrl Pts',(-8.88610136059988,-1.16276985667007,
28.9561993879088));
#17172=CARTESIAN_POINT('Ctrl Pts',(-9.1380883482013,-1.00235817476326,28.9441962011195));
#17173=CARTESIAN_POINT('Ctrl Pts',(-9.39007533580273,-0.841946492856447,
28.9321930143302));
#17174=CARTESIAN_POINT('Ctrl Pts',(-9.57754329642151,-0.58310243060262,
28.9201898275409));
#17175=CARTESIAN_POINT('Ctrl Pts',(-9.65136659729197,-0.293655596345962,
28.9081866407515));
#17176=CARTESIAN_POINT('Ctrl Pts',(-9.67581103310558,-0.197813707971806,
28.9042121350661));
#17177=CARTESIAN_POINT('Ctrl Pts',(-9.68822500000014,-0.098910050091216,
28.9002376293806));
#17178=CARTESIAN_POINT('Ctrl Pts',(-9.688225,1.63313806922361E-12,28.8962631236951));
#17179=CARTESIAN_POINT('Ctrl Pts',(-9.688225,-8.42104164178181E-14,28.8537368763048));
#17180=CARTESIAN_POINT('Ctrl Pts',(-9.68822499999998,-0.298712821306166,
28.8657400630942));
#17181=CARTESIAN_POINT('Ctrl Pts',(-9.57054245632583,-0.595858078271582,
28.8777432498835));
#17182=CARTESIAN_POINT('Ctrl Pts',(-9.36601586214931,-0.813569405232756,
28.8897464366728));
#17183=CARTESIAN_POINT('Ctrl Pts',(-9.1614892679728,-1.03128073219393,28.9017496234621));
#17184=CARTESIAN_POINT('Ctrl Pts',(-8.87226522412844,-1.16727314847136,
28.9137528102514));
#17185=CARTESIAN_POINT('Ctrl Pts',(-8.57413435701449,-1.1859100926019,28.9257559970407));
#17186=CARTESIAN_POINT('Ctrl Pts',(-8.27600348990054,-1.20454703673244,
28.9377591838301));
#17187=CARTESIAN_POINT('Ctrl Pts',(-7.97209482032096,-1.1056329054011,28.9497623706194));
#17188=CARTESIAN_POINT('Ctrl Pts',(-7.74204705372064,-0.915087963996601,
28.9617655574087));
#17189=CARTESIAN_POINT('Ctrl Pts',(-7.51199928712033,-0.724543022592099,
28.973768744198));
#17190=CARTESIAN_POINT('Ctrl Pts',(-7.35822688079637,-0.444367128061534,
28.9857719309873));
#17191=CARTESIAN_POINT('Ctrl Pts',(-7.32102560975818,-0.147979855990377,
28.9977751177767));
#17192=CARTESIAN_POINT('Ctrl Pts',(-7.28382433871999,0.148407416080781,
29.009778304566));
#17193=CARTESIAN_POINT('Ctrl Pts',(-7.36358464744632,0.457895344721854,
29.0217814913553));
#17194=CARTESIAN_POINT('Ctrl Pts',(-7.53940549437875,0.6993831899576,29.0337846781446));
#17195=CARTESIAN_POINT('Ctrl Pts',(-7.71522634131118,0.940871035193346,
29.0457878649339));
#17196=CARTESIAN_POINT('Ctrl Pts',(-7.9852624056577,1.11182427083076,29.0577910517232));
#17197=CARTESIAN_POINT('Ctrl Pts',(-8.27875123560101,1.16744491727744,29.0697942385126));
#17198=CARTESIAN_POINT('Ctrl Pts',(-8.57224006554432,1.22306556372412,29.0817974253019));
#17199=CARTESIAN_POINT('Ctrl Pts',(-8.88610136059923,1.1627698566703,29.0938006120912));
#17200=CARTESIAN_POINT('Ctrl Pts',(-9.13808834820077,1.0023581747636,29.1058037988805));
#17201=CARTESIAN_POINT('Ctrl Pts',(-9.39007533580232,0.841946492856894,
29.1178069856698));
#17202=CARTESIAN_POINT('Ctrl Pts',(-9.57754329642125,0.583102430603112,
29.1298101724591));
#17203=CARTESIAN_POINT('Ctrl Pts',(-9.65136659729185,0.293655596346441,
29.1418133592485));
#17204=CARTESIAN_POINT('Ctrl Pts',(-9.67581103310541,0.197813707972643,
29.1457878649339));
#17205=CARTESIAN_POINT('Ctrl Pts',(-9.688225,0.0989100500924303,29.1497623706194));
#17206=CARTESIAN_POINT('Ctrl Pts',(-9.688225,-5.8564264548977E-14,29.1537368763048));
#17207=CARTESIAN_POINT('Origin',(-8.5,0.,1.8));
#17208=CARTESIAN_POINT('',(-9.688225,1.68431935065882E-12,29.4962631236951));
#17209=CARTESIAN_POINT('',(-9.68727888030919,8.85048131729375E-5,29.4537368763048));
#17210=CARTESIAN_POINT('',(-9.688225,-1.45515594291686E-16,1.8));
#17211=CARTESIAN_POINT('Ctrl Pts',(-9.688225,1.68431935065882E-12,29.4962631236951));
#17212=CARTESIAN_POINT('Ctrl Pts',(-9.68822499999958,0.298712821307722,
29.4842599369058));
#17213=CARTESIAN_POINT('Ctrl Pts',(-9.57054245632506,0.595858078272935,
29.4722567501165));
#17214=CARTESIAN_POINT('Ctrl Pts',(-9.36601586214831,0.813569405233824,
29.4602535633272));
#17215=CARTESIAN_POINT('Ctrl Pts',(-9.16148926797156,1.03128073219471,29.4482503765379));
#17216=CARTESIAN_POINT('Ctrl Pts',(-8.87226522412708,1.16727314847178,29.4362471897485));
#17217=CARTESIAN_POINT('Ctrl Pts',(-8.57413435701316,1.18591009260198,29.4242440029592));
#17218=CARTESIAN_POINT('Ctrl Pts',(-8.27600348989924,1.20454703673219,29.4122408161699));
#17219=CARTESIAN_POINT('Ctrl Pts',(-7.97209482031981,1.10563290540054,29.4002376293806));
#17220=CARTESIAN_POINT('Ctrl Pts',(-7.74204705371972,0.915087963995839,
29.3882344425913));
#17221=CARTESIAN_POINT('Ctrl Pts',(-7.51199928711963,0.724543022591135,
29.376231255802));
#17222=CARTESIAN_POINT('Ctrl Pts',(-7.35822688079597,0.444367128060472,
29.3642280690126));
#17223=CARTESIAN_POINT('Ctrl Pts',(-7.32102560975805,0.147979855989325,
29.3522248822233));
#17224=CARTESIAN_POINT('Ctrl Pts',(-7.28382433872013,-0.148407416081821,
29.340221695434));
#17225=CARTESIAN_POINT('Ctrl Pts',(-7.36358464744671,-0.457895344722775,
29.3282185086447));
#17226=CARTESIAN_POINT('Ctrl Pts',(-7.5394054943793,-0.699383189958348,
29.3162153218554));
#17227=CARTESIAN_POINT('Ctrl Pts',(-7.71522634131188,-0.940871035193921,
29.3042121350661));
#17228=CARTESIAN_POINT('Ctrl Pts',(-7.98526240565849,-1.11182427083111,
29.2922089482767));
#17229=CARTESIAN_POINT('Ctrl Pts',(-8.27875123560179,-1.16744491727758,
29.2802057614874));
#17230=CARTESIAN_POINT('Ctrl Pts',(-8.57224006554509,-1.22306556372406,
29.2682025746981));
#17231=CARTESIAN_POINT('Ctrl Pts',(-8.88610136059991,-1.16276985667006,
29.2561993879088));
#17232=CARTESIAN_POINT('Ctrl Pts',(-9.13808834820133,-1.00235817476324,
29.2441962011195));
#17233=CARTESIAN_POINT('Ctrl Pts',(-9.39007533580275,-0.841946492856428,
29.2321930143302));
#17234=CARTESIAN_POINT('Ctrl Pts',(-9.57754329642152,-0.583102430602597,
29.2201898275409));
#17235=CARTESIAN_POINT('Ctrl Pts',(-9.65136659729198,-0.293655596345938,
29.2081866407515));
#17236=CARTESIAN_POINT('Ctrl Pts',(-9.67581103310559,-0.19781370797178,
29.2042121350661));
#17237=CARTESIAN_POINT('Ctrl Pts',(-9.68822500000014,-0.0989100500911904,
29.2002376293806));
#17238=CARTESIAN_POINT('Ctrl Pts',(-9.688225,1.65867319878998E-12,29.1962631236951));
#17239=CARTESIAN_POINT('Ctrl Pts',(-9.688225,-5.8564264548977E-14,29.1537368763048));
#17240=CARTESIAN_POINT('Ctrl Pts',(-9.68822499999998,-0.298712821306141,
29.1657400630942));
#17241=CARTESIAN_POINT('Ctrl Pts',(-9.57054245632584,-0.595858078271559,
29.1777432498835));
#17242=CARTESIAN_POINT('Ctrl Pts',(-9.36601586214933,-0.813569405232737,
29.1897464366728));
#17243=CARTESIAN_POINT('Ctrl Pts',(-9.16148926797282,-1.03128073219392,
29.2017496234621));
#17244=CARTESIAN_POINT('Ctrl Pts',(-8.87226522412846,-1.16727314847135,
29.2137528102514));
#17245=CARTESIAN_POINT('Ctrl Pts',(-8.57413435701451,-1.1859100926019,29.2257559970407));
#17246=CARTESIAN_POINT('Ctrl Pts',(-8.27600348990057,-1.20454703673244,
29.2377591838301));
#17247=CARTESIAN_POINT('Ctrl Pts',(-7.97209482032099,-1.10563290540111,
29.2497623706194));
#17248=CARTESIAN_POINT('Ctrl Pts',(-7.74204705372066,-0.915087963996617,
29.2617655574087));
#17249=CARTESIAN_POINT('Ctrl Pts',(-7.51199928712034,-0.724543022592121,
29.273768744198));
#17250=CARTESIAN_POINT('Ctrl Pts',(-7.35822688079638,-0.444367128061559,
29.2857719309873));
#17251=CARTESIAN_POINT('Ctrl Pts',(-7.32102560975818,-0.147979855990402,
29.2977751177767));
#17252=CARTESIAN_POINT('Ctrl Pts',(-7.28382433871999,0.148407416080755,
29.309778304566));
#17253=CARTESIAN_POINT('Ctrl Pts',(-7.36358464744631,0.457895344721829,
29.3217814913553));
#17254=CARTESIAN_POINT('Ctrl Pts',(-7.53940549437874,0.699383189957579,
29.3337846781446));
#17255=CARTESIAN_POINT('Ctrl Pts',(-7.71522634131116,0.940871035193329,
29.3457878649339));
#17256=CARTESIAN_POINT('Ctrl Pts',(-7.98526240565768,1.11182427083075,29.3577910517232));
#17257=CARTESIAN_POINT('Ctrl Pts',(-8.27875123560099,1.16744491727743,29.3697942385126));
#17258=CARTESIAN_POINT('Ctrl Pts',(-8.5722400655443,1.22306556372412,29.3817974253019));
#17259=CARTESIAN_POINT('Ctrl Pts',(-8.8861013605992,1.16276985667031,29.3938006120912));
#17260=CARTESIAN_POINT('Ctrl Pts',(-9.13808834820075,1.00235817476361,29.4058037988805));
#17261=CARTESIAN_POINT('Ctrl Pts',(-9.3900753358023,0.841946492856913,29.4178069856698));
#17262=CARTESIAN_POINT('Ctrl Pts',(-9.57754329642124,0.583102430603135,
29.4298101724591));
#17263=CARTESIAN_POINT('Ctrl Pts',(-9.65136659729185,0.293655596346466,
29.4418133592485));
#17264=CARTESIAN_POINT('Ctrl Pts',(-9.67581103310541,0.197813707972669,
29.4457878649339));
#17265=CARTESIAN_POINT('Ctrl Pts',(-9.688225,0.0989100500924559,29.4497623706194));
#17266=CARTESIAN_POINT('Ctrl Pts',(-9.688225,-3.29736238313671E-14,29.4537368763048));
#17267=CARTESIAN_POINT('Origin',(-8.5,0.,1.8));
#17268=CARTESIAN_POINT('',(-9.688225,1.70996550252767E-12,29.7962631236951));
#17269=CARTESIAN_POINT('',(-9.68829027239597,-0.000978575593966811,29.7537368763048));
#17270=CARTESIAN_POINT('',(-9.688225,-1.45515594291686E-16,1.8));
#17271=CARTESIAN_POINT('Ctrl Pts',(-9.688225,1.70996550252767E-12,29.7962631236951));
#17272=CARTESIAN_POINT('Ctrl Pts',(-9.68822499999957,0.298712821307747,
29.7842599369058));
#17273=CARTESIAN_POINT('Ctrl Pts',(-9.57054245632505,0.595858078272958,
29.7722567501165));
#17274=CARTESIAN_POINT('Ctrl Pts',(-9.36601586214829,0.813569405233843,
29.7602535633272));
#17275=CARTESIAN_POINT('Ctrl Pts',(-9.16148926797154,1.03128073219473,29.7482503765379));
#17276=CARTESIAN_POINT('Ctrl Pts',(-8.87226522412706,1.16727314847179,29.7362471897485));
#17277=CARTESIAN_POINT('Ctrl Pts',(-8.57413435701313,1.18591009260199,29.7242440029592));
#17278=CARTESIAN_POINT('Ctrl Pts',(-8.27600348989921,1.20454703673218,29.7122408161699));
#17279=CARTESIAN_POINT('Ctrl Pts',(-7.97209482031979,1.10563290540053,29.7002376293806));
#17280=CARTESIAN_POINT('Ctrl Pts',(-7.7420470537197,0.915087963995822,29.6882344425913));
#17281=CARTESIAN_POINT('Ctrl Pts',(-7.51199928711962,0.724543022591113,
29.676231255802));
#17282=CARTESIAN_POINT('Ctrl Pts',(-7.35822688079596,0.444367128060447,
29.6642280690126));
#17283=CARTESIAN_POINT('Ctrl Pts',(-7.32102560975805,0.1479798559893,29.6522248822233));
#17284=CARTESIAN_POINT('Ctrl Pts',(-7.28382433872013,-0.148407416081847,
29.640221695434));
#17285=CARTESIAN_POINT('Ctrl Pts',(-7.36358464744672,-0.457895344722799,
29.6282185086447));
#17286=CARTESIAN_POINT('Ctrl Pts',(-7.53940549437931,-0.699383189958368,
29.6162153218554));
#17287=CARTESIAN_POINT('Ctrl Pts',(-7.7152263413119,-0.940871035193937,
29.6042121350661));
#17288=CARTESIAN_POINT('Ctrl Pts',(-7.98526240565851,-1.11182427083112,
29.5922089482767));
#17289=CARTESIAN_POINT('Ctrl Pts',(-8.27875123560181,-1.16744491727759,
29.5802057614874));
#17290=CARTESIAN_POINT('Ctrl Pts',(-8.57224006554512,-1.22306556372406,
29.5682025746981));
#17291=CARTESIAN_POINT('Ctrl Pts',(-8.88610136059993,-1.16276985667005,
29.5561993879088));
#17292=CARTESIAN_POINT('Ctrl Pts',(-9.13808834820135,-1.00235817476323,
29.5441962011195));
#17293=CARTESIAN_POINT('Ctrl Pts',(-9.39007533580277,-0.841946492856409,
29.5321930143302));
#17294=CARTESIAN_POINT('Ctrl Pts',(-9.57754329642153,-0.583102430602574,
29.5201898275409));
#17295=CARTESIAN_POINT('Ctrl Pts',(-9.65136659729199,-0.293655596345913,
29.5081866407515));
#17296=CARTESIAN_POINT('Ctrl Pts',(-9.67581103310559,-0.197813707971755,
29.5042121350661));
#17297=CARTESIAN_POINT('Ctrl Pts',(-9.68822500000014,-0.0989100500911648,
29.5002376293806));
#17298=CARTESIAN_POINT('Ctrl Pts',(-9.688225,1.68431935065882E-12,29.4962631236951));
#17299=CARTESIAN_POINT('Ctrl Pts',(-9.68630702871204,0.000179416718910312,
29.4537368763049));
#17300=CARTESIAN_POINT('Ctrl Pts',(-9.68614803161525,-0.208258635069709,
29.4620824521433));
#17301=CARTESIAN_POINT('Ctrl Pts',(-9.63399075937292,-0.416818054777034,
29.4704280279817));
#17302=CARTESIAN_POINT('Ctrl Pts',(-9.53044187393016,-0.595799011918308,
29.4787736038201));
#17303=CARTESIAN_POINT('Ctrl Pts',(-9.33306934044666,-0.936951162472383,
29.4946809449717));
#17304=CARTESIAN_POINT('Ctrl Pts',(-8.94898369186194,-1.17064050846203,
29.5105882861234));
#17305=CARTESIAN_POINT('Ctrl Pts',(-8.55559785580855,-1.18900976154421,
29.526495627275));
#17306=CARTESIAN_POINT('Ctrl Pts',(-8.16221201975512,-1.2073790146264,29.5424029684266));
#17307=CARTESIAN_POINT('Ctrl Pts',(-7.75952599623297,-1.01042817480108,
29.5583103095782));
#17308=CARTESIAN_POINT('Ctrl Pts',(-7.53039248685666,-0.689467174220619,
29.5742176507298));
#17309=CARTESIAN_POINT('Ctrl Pts',(-7.41582573216856,-0.528986673930462,
29.5821713213056));
#17310=CARTESIAN_POINT('Ctrl Pts',(-7.34464710601685,-0.33750363345153,
29.5901249918815));
#17311=CARTESIAN_POINT('Ctrl Pts',(-7.32116324979802,-0.140351109640275,
29.5980786624573));
#17312=CARTESIAN_POINT('Ctrl Pts',(-7.29767939357918,0.0568014141710692,
29.6060323330331));
#17313=CARTESIAN_POINT('Ctrl Pts',(-7.32189030729322,0.259623421314646,
29.6139860036089));
#17314=CARTESIAN_POINT('Ctrl Pts',(-7.39558129849426,0.442514540719367,
29.6219396741847));
#17315=CARTESIAN_POINT('Ctrl Pts',(-7.54296328089633,0.808296779528768,
29.6378470153363));
#17316=CARTESIAN_POINT('Ctrl Pts',(-7.88826557324638,1.09435546738231,29.6537543564879));
#17317=CARTESIAN_POINT('Ctrl Pts',(-8.27492430307999,1.16885146040352,29.6696616976396));
#17318=CARTESIAN_POINT('Ctrl Pts',(-8.66158303291351,1.2433474534247,29.6855690387912));
#17319=CARTESIAN_POINT('Ctrl Pts',(-9.08959820023061,1.10628075161366,29.7014763799428));
#17320=CARTESIAN_POINT('Ctrl Pts',(-9.36164000612452,0.821043330033523,
29.7173837210944));
#17321=CARTESIAN_POINT('Ctrl Pts',(-9.56887300417075,0.603758321816504,
29.7295014394979));
#17322=CARTESIAN_POINT('Ctrl Pts',(-9.68559592122482,0.300491042494952,
29.7416191579014));
#17323=CARTESIAN_POINT('Ctrl Pts',(-9.68829027239597,-0.000978575593966811,
29.7537368763048));
#17324=CARTESIAN_POINT('Origin',(-8.5,0.,1.24542303242842));
#17325=CARTESIAN_POINT('',(-9.516475,1.77136955610542E-12,29.8954230324284));
#17326=CARTESIAN_POINT('',(-9.516475,1.79831334285591E-12,29.9545769675714));
#17327=CARTESIAN_POINT('',(-9.516475,1.78524650477582E-12,1.24542303242842));
#17328=CARTESIAN_POINT('',(-7.90984029786094,-0.827606761449023,30.));
#17329=CARTESIAN_POINT('Ctrl Pts',(-9.516475,1.8869293844785E-12,29.8954230324284));
#17330=CARTESIAN_POINT('Ctrl Pts',(-9.51647500000049,-0.265706620582062,
29.9079039656766));
#17331=CARTESIAN_POINT('Ctrl Pts',(-9.40727465387295,-0.529786878175418,
29.9203848989248));
#17332=CARTESIAN_POINT('Ctrl Pts',(-9.21961691907893,-0.717894780173495,
29.932865832173));
#17333=CARTESIAN_POINT('Ctrl Pts',(-9.0319591842849,-0.906002682171572,
29.9453467654212));
#17334=CARTESIAN_POINT('Ctrl Pts',(-8.7681413283455,-1.01583545019863,29.9578276986694));
#17335=CARTESIAN_POINT('Ctrl Pts',(-8.50243547044677,-1.01647208230659,
29.9703086319176));
#17336=CARTESIAN_POINT('Ctrl Pts',(-8.29173620430335,-1.0169769184401,29.9802057546117));
#17337=CARTESIAN_POINT('Ctrl Pts',(-8.0813906437366,-0.94993792854409,29.9901028773059));
#17338=CARTESIAN_POINT('Ctrl Pts',(-7.90984029786094,-0.827606761449023,
30.));
#17339=CARTESIAN_POINT('',(-9.09015970213943,-0.827606761448756,30.));
#17340=CARTESIAN_POINT('Origin',(-8.5,0.,30.));
#17341=CARTESIAN_POINT('Ctrl Pts',(-9.51769523843386,0.000138611918728023,
29.9545769675714));
#17342=CARTESIAN_POINT('Ctrl Pts',(-9.51757347611664,-0.152713583871541,
29.9617643078051));
#17343=CARTESIAN_POINT('Ctrl Pts',(-9.44060368458966,-0.475706479329954,
29.9769053186147));
#17344=CARTESIAN_POINT('Ctrl Pts',(-9.22802350159151,-0.72929719873085,
29.9920463294242));
#17345=CARTESIAN_POINT('Ctrl Pts',(-9.09015970213924,-0.82760676144889,
30.));
#17346=CARTESIAN_POINT('Origin',(-8.5,0.,1.24542303242842));
#17347=CARTESIAN_POINT('',(-9.516475,1.74945312371443E-12,29.5954230324284));
#17348=CARTESIAN_POINT('',(-9.516475,1.776396937294E-12,29.6545769675714));
#17349=CARTESIAN_POINT('',(-9.516475,1.78524650477582E-12,1.24542303242842));
#17350=CARTESIAN_POINT('Ctrl Pts',(-9.516475,1.74945312371443E-12,29.5954230324284));
#17351=CARTESIAN_POINT('Ctrl Pts',(-9.51647500000046,-0.2657066205822,29.6079039656766));
#17352=CARTESIAN_POINT('Ctrl Pts',(-9.40727465387288,-0.529786878175541,
29.6203848989248));
#17353=CARTESIAN_POINT('Ctrl Pts',(-9.21961691907883,-0.717894780173593,
29.632865832173));
#17354=CARTESIAN_POINT('Ctrl Pts',(-9.03195918428478,-0.906002682171644,
29.6453467654212));
#17355=CARTESIAN_POINT('Ctrl Pts',(-8.76814132834537,-1.01583545019867,
29.6578276986694));
#17356=CARTESIAN_POINT('Ctrl Pts',(-8.50243547044663,-1.01647208230659,
29.6703086319176));
#17357=CARTESIAN_POINT('Ctrl Pts',(-8.2367296125479,-1.01710871441452,29.6827895651657));
#17358=CARTESIAN_POINT('Ctrl Pts',(-7.9723884693348,-0.908541417083597,
29.6952704984139));
#17359=CARTESIAN_POINT('Ctrl Pts',(-7.78383148002456,-0.72133492679974,
29.7077514316621));
#17360=CARTESIAN_POINT('Ctrl Pts',(-7.59527449071432,-0.534128436515884,
29.7202323649103));
#17361=CARTESIAN_POINT('Ctrl Pts',(-7.48480993131748,-0.270574496757414,
29.7327132981585));
#17362=CARTESIAN_POINT('Ctrl Pts',(-7.48353667075687,-0.00487092690994738,
29.7451942314067));
#17363=CARTESIAN_POINT('Ctrl Pts',(-7.48226341019625,0.260832642937519,
29.7576751646549));
#17364=CARTESIAN_POINT('Ctrl Pts',(-7.59019703546662,0.525433154238881,
29.7701560979031));
#17365=CARTESIAN_POINT('Ctrl Pts',(-7.77695120652395,0.71443814839203,29.7826370311513));
#17366=CARTESIAN_POINT('Ctrl Pts',(-7.96370537758128,0.903443142545179,
29.7951179643995));
#17367=CARTESIAN_POINT('Ctrl Pts',(-8.2269938881465,1.01453885915611,29.8075988976476));
#17368=CARTESIAN_POINT('Ctrl Pts',(-8.49269364458979,1.01644874085987,29.8200798308958));
#17369=CARTESIAN_POINT('Ctrl Pts',(-8.75839340103307,1.01835862256364,29.832560764144));
#17370=CARTESIAN_POINT('Ctrl Pts',(-9.02325176140223,0.911059288979924,
29.8450416973922));
#17371=CARTESIAN_POINT('Ctrl Pts',(-9.21270367535709,0.724758509268773,
29.8575226306404));
#17372=CARTESIAN_POINT('Ctrl Pts',(-9.40215558931195,0.538457729557621,
29.8700035638886));
#17373=CARTESIAN_POINT('Ctrl Pts',(-9.51388182535791,0.275436159674178,
29.8824844971368));
#17374=CARTESIAN_POINT('Ctrl Pts',(-9.51642831724056,0.00974174196610049,
29.894965430385));
#17375=CARTESIAN_POINT('Ctrl Pts',(-9.51645943884196,0.00649459406839334,
29.8951179643995));
#17376=CARTESIAN_POINT('Ctrl Pts',(-9.51647499999999,0.00324729703536851,
29.8952704984139));
#17377=CARTESIAN_POINT('Ctrl Pts',(-9.516475,1.8869293844785E-12,29.8954230324284));
#17378=CARTESIAN_POINT('Ctrl Pts',(-9.516475,1.776396937294E-12,29.6545769675714));
#17379=CARTESIAN_POINT('Ctrl Pts',(-9.51647500000046,-0.265706620582173,
29.6670579008196));
#17380=CARTESIAN_POINT('Ctrl Pts',(-9.4072746538729,-0.529786878175517,
29.6795388340678));
#17381=CARTESIAN_POINT('Ctrl Pts',(-9.21961691907885,-0.717894780173574,
29.692019767316));
#17382=CARTESIAN_POINT('Ctrl Pts',(-9.0319591842848,-0.90600268217163,29.7045007005642));
#17383=CARTESIAN_POINT('Ctrl Pts',(-8.76814132834539,-1.01583545019866,
29.7169816338124));
#17384=CARTESIAN_POINT('Ctrl Pts',(-8.50243547044666,-1.01647208230659,
29.7294625670606));
#17385=CARTESIAN_POINT('Ctrl Pts',(-8.23672961254792,-1.01710871441453,
29.7419435003088));
#17386=CARTESIAN_POINT('Ctrl Pts',(-7.97238846933483,-0.908541417083611,
29.754424433557));
#17387=CARTESIAN_POINT('Ctrl Pts',(-7.78383148002458,-0.721334926799759,
29.7669053668051));
#17388=CARTESIAN_POINT('Ctrl Pts',(-7.59527449071433,-0.534128436515908,
29.7793863000533));
#17389=CARTESIAN_POINT('Ctrl Pts',(-7.48480993131749,-0.270574496757441,
29.7918672333015));
#17390=CARTESIAN_POINT('Ctrl Pts',(-7.48353667075687,-0.00487092690997433,
29.8043481665497));
#17391=CARTESIAN_POINT('Ctrl Pts',(-7.48226341019624,0.260832642937492,
29.8168290997979));
#17392=CARTESIAN_POINT('Ctrl Pts',(-7.59019703546661,0.525433154238857,
29.8293100330461));
#17393=CARTESIAN_POINT('Ctrl Pts',(-7.77695120652393,0.714438148392011,
29.8417909662943));
#17394=CARTESIAN_POINT('Ctrl Pts',(-7.96370537758126,0.903443142545165,
29.8542718995425));
#17395=CARTESIAN_POINT('Ctrl Pts',(-8.22699388814648,1.0145388591561,29.8667528327907));
#17396=CARTESIAN_POINT('Ctrl Pts',(-8.49269364458976,1.01644874085987,29.8792337660389));
#17397=CARTESIAN_POINT('Ctrl Pts',(-8.75839340103304,1.01835862256364,29.891714699287));
#17398=CARTESIAN_POINT('Ctrl Pts',(-9.02325176140221,0.911059288979938,
29.9041956325352));
#17399=CARTESIAN_POINT('Ctrl Pts',(-9.21270367535707,0.724758509268792,
29.9166765657834));
#17400=CARTESIAN_POINT('Ctrl Pts',(-9.40215558931194,0.538457729557645,
29.9291574990316));
#17401=CARTESIAN_POINT('Ctrl Pts',(-9.5138818253579,0.275436159674205,29.9416384322798));
#17402=CARTESIAN_POINT('Ctrl Pts',(-9.51642831724056,0.00974174196612743,
29.954119365528));
#17403=CARTESIAN_POINT('Ctrl Pts',(-9.51645943884196,0.00649459406838176,
29.9542718995425));
#17404=CARTESIAN_POINT('Ctrl Pts',(-9.51647499999999,0.00324729703531833,
29.954424433557));
#17405=CARTESIAN_POINT('Ctrl Pts',(-9.516475,1.79831336968498E-12,29.9545769675714));
#17406=CARTESIAN_POINT('Origin',(-8.5,0.,1.24542303242842));
#17407=CARTESIAN_POINT('',(-9.516475,1.72753669132345E-12,29.2954230324284));
#17408=CARTESIAN_POINT('',(-9.51618362200288,2.72569712245247E-5,29.3545769675714));
#17409=CARTESIAN_POINT('',(-9.516475,1.78524650477582E-12,1.24542303242842));
#17410=CARTESIAN_POINT('Ctrl Pts',(-9.516475,1.72753669132345E-12,29.2954230324284));
#17411=CARTESIAN_POINT('Ctrl Pts',(-9.51647500000045,-0.265706620582183,
29.3079039656766));
#17412=CARTESIAN_POINT('Ctrl Pts',(-9.4072746538729,-0.529786878175485,
29.3203848989248));
#17413=CARTESIAN_POINT('Ctrl Pts',(-9.2196169190789,-0.717894780173526,
29.332865832173));
#17414=CARTESIAN_POINT('Ctrl Pts',(-9.03195918428489,-0.906002682171568,
29.3453467654212));
#17415=CARTESIAN_POINT('Ctrl Pts',(-8.76814132834554,-1.01583545019861,
29.3578276986694));
#17416=CARTESIAN_POINT('Ctrl Pts',(-8.50243547044684,-1.01647208230659,
29.3703086319175));
#17417=CARTESIAN_POINT('Ctrl Pts',(-8.23672961254815,-1.01710871441458,
29.3827895651657));
#17418=CARTESIAN_POINT('Ctrl Pts',(-7.97238846933507,-0.908541417083738,
29.3952704984139));
#17419=CARTESIAN_POINT('Ctrl Pts',(-7.78383148002479,-0.721334926799969,
29.4077514316621));
#17420=CARTESIAN_POINT('Ctrl Pts',(-7.59527449071451,-0.5341284365162,29.4202323649103));
#17421=CARTESIAN_POINT('Ctrl Pts',(-7.4848099313176,-0.270574496757815,
29.4327132981585));
#17422=CARTESIAN_POINT('Ctrl Pts',(-7.48353667075687,-0.0048709269103877,
29.4451942314067));
#17423=CARTESIAN_POINT('Ctrl Pts',(-7.48226341019614,0.26083264293704,29.4576751646549));
#17424=CARTESIAN_POINT('Ctrl Pts',(-7.59019703546636,0.525433154238411,
29.4701560979031));
#17425=CARTESIAN_POINT('Ctrl Pts',(-7.77695120652356,0.714438148391635,
29.4826370311512));
#17426=CARTESIAN_POINT('Ctrl Pts',(-7.96370537758076,0.903443142544859,
29.4951179643994));
#17427=CARTESIAN_POINT('Ctrl Pts',(-8.22699388814587,1.01453885915593,29.5075988976476));
#17428=CARTESIAN_POINT('Ctrl Pts',(-8.49269364458912,1.01644874085987,29.5200798308958));
#17429=CARTESIAN_POINT('Ctrl Pts',(-8.75839340103236,1.01835862256381,29.532560764144));
#17430=CARTESIAN_POINT('Ctrl Pts',(-9.02325176140155,0.911059288980303,
29.5450416973922));
#17431=CARTESIAN_POINT('Ctrl Pts',(-9.21270367535653,0.724758509269325,
29.5575226306404));
#17432=CARTESIAN_POINT('Ctrl Pts',(-9.40215558931151,0.538457729558346,
29.5700035638886));
#17433=CARTESIAN_POINT('Ctrl Pts',(-9.51388182535766,0.27543615967504,29.5824844971367));
#17434=CARTESIAN_POINT('Ctrl Pts',(-9.51642831724055,0.00974174196700301,
29.5949654303849));
#17435=CARTESIAN_POINT('Ctrl Pts',(-9.51645943884196,0.00649459406894922,
29.5951179643994));
#17436=CARTESIAN_POINT('Ctrl Pts',(-9.51647499999999,0.00324729703557761,
29.5952704984139));
#17437=CARTESIAN_POINT('Ctrl Pts',(-9.516475,1.74945312371443E-12,29.5954230324284));
#17438=CARTESIAN_POINT('Ctrl Pts',(-9.51483425867161,0.000153483230988238,
29.3545769675714));
#17439=CARTESIAN_POINT('Ctrl Pts',(-9.51469824354527,-0.178156238154032,
29.3629225434099));
#17440=CARTESIAN_POINT('Ctrl Pts',(-9.47007995719168,-0.356569784534552,
29.3712681192483));
#17441=CARTESIAN_POINT('Ctrl Pts',(-9.38149837261734,-0.509680237866999,
29.3796136950868));
#17442=CARTESIAN_POINT('Ctrl Pts',(-9.21265472265832,-0.801521120052119,
29.3955210362384));
#17443=CARTESIAN_POINT('Ctrl Pts',(-8.8840860932784,-1.00143222945046,29.41142837739));
#17444=CARTESIAN_POINT('Ctrl Pts',(-8.54756155650945,-1.01714632949621,
29.4273357185417));
#17445=CARTESIAN_POINT('Ctrl Pts',(-8.21103701974038,-1.03286042954196,
29.4432430596933));
#17446=CARTESIAN_POINT('Ctrl Pts',(-7.86655657558232,-0.864377520234989,
29.4591504008449));
#17447=CARTESIAN_POINT('Ctrl Pts',(-7.67054278699563,-0.589809291940723,
29.4750577419965));
#17448=CARTESIAN_POINT('Ctrl Pts',(-7.57253589270232,-0.452525177793652,
29.4830114125723));
#17449=CARTESIAN_POINT('Ctrl Pts',(-7.51164566230181,-0.288719733899682,
29.4909650831482));
#17450=CARTESIAN_POINT('Ctrl Pts',(-7.49155624089586,-0.12006429268186,
29.498918753724));
#17451=CARTESIAN_POINT('Ctrl Pts',(-7.4714668194899,0.0485911485360002,
29.5068724242998));
#17452=CARTESIAN_POINT('Ctrl Pts',(-7.49217820707847,0.222096587077811,
29.5148260948756));
#17453=CARTESIAN_POINT('Ctrl Pts',(-7.55521765691417,0.378552014793018,
29.5227797654514));
#17454=CARTESIAN_POINT('Ctrl Pts',(-7.68129655658559,0.691462870223505,
29.538687106603));
#17455=CARTESIAN_POINT('Ctrl Pts',(-7.97668770524555,0.936173682347486,
29.5545944477546));
#17456=CARTESIAN_POINT('Ctrl Pts',(-8.30745749413879,0.999901776358546,
29.5705017889063));
#17457=CARTESIAN_POINT('Ctrl Pts',(-8.63822728303192,1.06362987036958,29.5864091300579));
#17458=CARTESIAN_POINT('Ctrl Pts',(-9.00437571215826,0.94637524626783,29.6023164712095));
#17459=CARTESIAN_POINT('Ctrl Pts',(-9.23709568913741,0.702366991854193,
29.6182238123611));
#17460=CARTESIAN_POINT('Ctrl Pts',(-9.41437453926143,0.516489082597208,
29.6303415307646));
#17461=CARTESIAN_POINT('Ctrl Pts',(-9.51422593702913,0.25705706614624,29.642459249168));
#17462=CARTESIAN_POINT('Ctrl Pts',(-9.51653083770639,-0.000837129015673788,
29.6545769675714));
#17463=CARTESIAN_POINT('Origin',(-8.5,0.,1.24542303242842));
#17464=CARTESIAN_POINT('',(-9.516475,1.70562025893246E-12,28.9954230324284));
#17465=CARTESIAN_POINT('',(-9.516475,1.73256407251203E-12,29.0545769675714));
#17466=CARTESIAN_POINT('',(-9.516475,1.78524650477582E-12,1.24542303242842));
#17467=CARTESIAN_POINT('Ctrl Pts',(-9.516475,1.70562025893246E-12,28.9954230324284));
#17468=CARTESIAN_POINT('Ctrl Pts',(-9.51647500000045,-0.265706620582321,
29.0079039656766));
#17469=CARTESIAN_POINT('Ctrl Pts',(-9.40727465387279,-0.529786878175732,
29.0203848989248));
#17470=CARTESIAN_POINT('Ctrl Pts',(-9.21961691907864,-0.717894780173787,
29.032865832173));
#17471=CARTESIAN_POINT('Ctrl Pts',(-9.03195918428448,-0.906002682171843,
29.0453467654212));
#17472=CARTESIAN_POINT('Ctrl Pts',(-8.76814132834494,-1.0158354501988,29.0578276986694));
#17473=CARTESIAN_POINT('Ctrl Pts',(-8.50243547044612,-1.0164720823066,29.0703086319176));
#17474=CARTESIAN_POINT('Ctrl Pts',(-8.23672961254731,-1.01710871441439,
29.0827895651658));
#17475=CARTESIAN_POINT('Ctrl Pts',(-7.9723884693342,-0.908541417083268,
29.095270498414));
#17476=CARTESIAN_POINT('Ctrl Pts',(-7.78383148002404,-0.721334926799221,
29.1077514316622));
#17477=CARTESIAN_POINT('Ctrl Pts',(-7.59527449071387,-0.534128436515173,
29.1202323649104));
#17478=CARTESIAN_POINT('Ctrl Pts',(-7.48480993131723,-0.270574496756524,
29.1327132981585));
#17479=CARTESIAN_POINT('Ctrl Pts',(-7.48353667075686,-0.00487092690897908,
29.1451942314067));
#17480=CARTESIAN_POINT('Ctrl Pts',(-7.4822634101965,0.260832642938566,29.1576751646549));
#17481=CARTESIAN_POINT('Ctrl Pts',(-7.59019703546719,0.5254331542399,29.1701560979031));
#17482=CARTESIAN_POINT('Ctrl Pts',(-7.7769512065248,0.714438148392883,29.1826370311513));
#17483=CARTESIAN_POINT('Ctrl Pts',(-7.9637053775824,0.903443142545867,29.1951179643995));
#17484=CARTESIAN_POINT('Ctrl Pts',(-8.22699388814785,1.01453885915649,29.2075988976477));
#17485=CARTESIAN_POINT('Ctrl Pts',(-8.49269364459122,1.01644874085988,29.2200798308959));
#17486=CARTESIAN_POINT('Ctrl Pts',(-8.75839340103458,1.01835862256327,29.2325607641441));
#17487=CARTESIAN_POINT('Ctrl Pts',(-9.02325176140366,0.911059288979123,
29.2450416973923));
#17488=CARTESIAN_POINT('Ctrl Pts',(-9.21270367535828,0.724758509267608,
29.2575226306405));
#17489=CARTESIAN_POINT('Ctrl Pts',(-9.40215558931289,0.538457729556092,
29.2700035638887));
#17490=CARTESIAN_POINT('Ctrl Pts',(-9.51388182535842,0.275436159672367,
29.2824844971369));
#17491=CARTESIAN_POINT('Ctrl Pts',(-9.51642831724057,0.00974174196420779,
29.2949654303851));
#17492=CARTESIAN_POINT('Ctrl Pts',(-9.51645943884196,0.00649459406707835,
29.2951179643995));
#17493=CARTESIAN_POINT('Ctrl Pts',(-9.51647499999999,0.00324729703463126,
29.295270498414));
#17494=CARTESIAN_POINT('Ctrl Pts',(-9.516475,1.72753669132345E-12,29.2954230324284));
#17495=CARTESIAN_POINT('Ctrl Pts',(-9.516475,1.73256407251203E-12,29.0545769675714));
#17496=CARTESIAN_POINT('Ctrl Pts',(-9.51647500000045,-0.265706620582294,
29.0670579008196));
#17497=CARTESIAN_POINT('Ctrl Pts',(-9.40727465387281,-0.529786878175708,
29.0795388340678));
#17498=CARTESIAN_POINT('Ctrl Pts',(-9.21961691907866,-0.717894780173768,
29.092019767316));
#17499=CARTESIAN_POINT('Ctrl Pts',(-9.0319591842845,-0.906002682171829,
29.1045007005642));
#17500=CARTESIAN_POINT('Ctrl Pts',(-8.76814132834496,-1.01583545019879,
29.1169816338124));
#17501=CARTESIAN_POINT('Ctrl Pts',(-8.50243547044615,-1.0164720823066,29.1294625670606));
#17502=CARTESIAN_POINT('Ctrl Pts',(-8.23672961254734,-1.0171087144144,29.1419435003088));
#17503=CARTESIAN_POINT('Ctrl Pts',(-7.97238846933422,-0.908541417083282,
29.154424433557));
#17504=CARTESIAN_POINT('Ctrl Pts',(-7.78383148002406,-0.72133492679924,
29.1669053668052));
#17505=CARTESIAN_POINT('Ctrl Pts',(-7.59527449071389,-0.534128436515197,
29.1793863000534));
#17506=CARTESIAN_POINT('Ctrl Pts',(-7.48480993131723,-0.270574496756551,
29.1918672333016));
#17507=CARTESIAN_POINT('Ctrl Pts',(-7.48353667075686,-0.00487092690900603,
29.2043481665498));
#17508=CARTESIAN_POINT('Ctrl Pts',(-7.48226341019649,0.260832642938539,
29.216829099798));
#17509=CARTESIAN_POINT('Ctrl Pts',(-7.59019703546717,0.525433154239876,
29.2293100330462));
#17510=CARTESIAN_POINT('Ctrl Pts',(-7.77695120652478,0.714438148392864,
29.2417909662943));
#17511=CARTESIAN_POINT('Ctrl Pts',(-7.96370537758238,0.903443142545853,
29.2542718995425));
#17512=CARTESIAN_POINT('Ctrl Pts',(-8.22699388814783,1.01453885915649,29.2667528327907));
#17513=CARTESIAN_POINT('Ctrl Pts',(-8.49269364459119,1.01644874085988,29.2792337660389));
#17514=CARTESIAN_POINT('Ctrl Pts',(-8.75839340103456,1.01835862256328,29.2917146992871));
#17515=CARTESIAN_POINT('Ctrl Pts',(-9.02325176140364,0.911059288979137,
29.3041956325353));
#17516=CARTESIAN_POINT('Ctrl Pts',(-9.21270367535826,0.724758509267627,
29.3166765657835));
#17517=CARTESIAN_POINT('Ctrl Pts',(-9.40215558931287,0.538457729556116,
29.3291574990317));
#17518=CARTESIAN_POINT('Ctrl Pts',(-9.51388182535841,0.275436159672394,
29.3416384322799));
#17519=CARTESIAN_POINT('Ctrl Pts',(-9.51642831724057,0.00974174196423473,
29.3541193655281));
#17520=CARTESIAN_POINT('Ctrl Pts',(-9.51645943884196,0.00649459406714381,
29.3542718995425));
#17521=CARTESIAN_POINT('Ctrl Pts',(-9.51647499999999,0.00324729703473532,
29.354424433557));
#17522=CARTESIAN_POINT('Ctrl Pts',(-9.516475,1.87004033327609E-12,29.3545769675714));
#17523=CARTESIAN_POINT('Origin',(-8.5,0.,1.24542303242842));
#17524=CARTESIAN_POINT('',(-9.516475,1.68370382654148E-12,28.6954230324284));
#17525=CARTESIAN_POINT('',(-9.51677113484703,-0.000181121393472947,28.7545769675714));
#17526=CARTESIAN_POINT('',(-9.516475,1.78524650477582E-12,1.24542303242842));
#17527=CARTESIAN_POINT('Ctrl Pts',(-9.516475,1.79926365491456E-12,28.6954230324284));
#17528=CARTESIAN_POINT('Ctrl Pts',(-9.51647500000047,-0.26570662058215,
28.7079039656766));
#17529=CARTESIAN_POINT('Ctrl Pts',(-9.40727465387291,-0.529786878175496,
28.7203848989248));
#17530=CARTESIAN_POINT('Ctrl Pts',(-9.21961691907887,-0.717894780173557,
28.732865832173));
#17531=CARTESIAN_POINT('Ctrl Pts',(-9.03195918428482,-0.906002682171618,
28.7453467654212));
#17532=CARTESIAN_POINT('Ctrl Pts',(-8.76814132834541,-1.01583545019865,
28.7578276986694));
#17533=CARTESIAN_POINT('Ctrl Pts',(-8.50243547044668,-1.01647208230659,
28.7703086319176));
#17534=CARTESIAN_POINT('Ctrl Pts',(-8.23672961254795,-1.01710871441454,
28.7827895651657));
#17535=CARTESIAN_POINT('Ctrl Pts',(-7.97238846933485,-0.908541417083623,
28.7952704984139));
#17536=CARTESIAN_POINT('Ctrl Pts',(-7.78383148002459,-0.721334926799775,
28.8077514316621));
#17537=CARTESIAN_POINT('Ctrl Pts',(-7.59527449071434,-0.534128436515928,
28.8202323649103));
#17538=CARTESIAN_POINT('Ctrl Pts',(-7.4848099313175,-0.270574496757464,
28.8327132981585));
#17539=CARTESIAN_POINT('Ctrl Pts',(-7.48353667075687,-0.00487092690999719,
28.8451942314067));
#17540=CARTESIAN_POINT('Ctrl Pts',(-7.48226341019623,0.260832642937469,
28.8576751646549));
#17541=CARTESIAN_POINT('Ctrl Pts',(-7.5901970354666,0.525433154238836,28.8701560979031));
#17542=CARTESIAN_POINT('Ctrl Pts',(-7.77695120652392,0.714438148391995,
28.8826370311513));
#17543=CARTESIAN_POINT('Ctrl Pts',(-7.96370537758124,0.903443142545153,
28.8951179643995));
#17544=CARTESIAN_POINT('Ctrl Pts',(-8.22699388814645,1.0145388591561,28.9075988976476));
#17545=CARTESIAN_POINT('Ctrl Pts',(-8.49269364458974,1.01644874085987,28.9200798308958));
#17546=CARTESIAN_POINT('Ctrl Pts',(-8.75839340103302,1.01835862256365,28.932560764144));
#17547=CARTESIAN_POINT('Ctrl Pts',(-9.02325176140219,0.91105928897995,28.9450416973922));
#17548=CARTESIAN_POINT('Ctrl Pts',(-9.21270367535706,0.724758509268808,
28.9575226306404));
#17549=CARTESIAN_POINT('Ctrl Pts',(-9.40215558931192,0.538457729557665,
28.9700035638886));
#17550=CARTESIAN_POINT('Ctrl Pts',(-9.51388182535789,0.275436159674228,
28.9824844971368));
#17551=CARTESIAN_POINT('Ctrl Pts',(-9.51642831724055,0.0097417419661503,
28.994965430385));
#17552=CARTESIAN_POINT('Ctrl Pts',(-9.51645943884196,0.00649459406836611,
28.9951179643995));
#17553=CARTESIAN_POINT('Ctrl Pts',(-9.51647499999999,0.00324729703526424,
28.9952704984139));
#17554=CARTESIAN_POINT('Ctrl Pts',(-9.516475,1.70562025893246E-12,28.9954230324284));
#17555=CARTESIAN_POINT('Ctrl Pts',(-9.516475,1.71064764012104E-12,28.7545769675714));
#17556=CARTESIAN_POINT('Ctrl Pts',(-9.51647500000045,-0.265706620582239,
28.7670579008196));
#17557=CARTESIAN_POINT('Ctrl Pts',(-9.40727465387286,-0.529786878175576,
28.7795388340678));
#17558=CARTESIAN_POINT('Ctrl Pts',(-9.2196169190788,-0.71789478017362,28.792019767316));
#17559=CARTESIAN_POINT('Ctrl Pts',(-9.03195918428474,-0.906002682171665,
28.8045007005642));
#17560=CARTESIAN_POINT('Ctrl Pts',(-8.76814132834533,-1.01583545019868,
28.8169816338124));
#17561=CARTESIAN_POINT('Ctrl Pts',(-8.50243547044659,-1.01647208230659,
28.8294625670606));
#17562=CARTESIAN_POINT('Ctrl Pts',(-8.23672961254786,-1.01710871441451,
28.8419435003088));
#17563=CARTESIAN_POINT('Ctrl Pts',(-7.97238846933477,-0.908541417083576,
28.854424433557));
#17564=CARTESIAN_POINT('Ctrl Pts',(-7.78383148002453,-0.721334926799713,
28.8669053668052));
#17565=CARTESIAN_POINT('Ctrl Pts',(-7.5952744907143,-0.534128436515849,
28.8793863000533));
#17566=CARTESIAN_POINT('Ctrl Pts',(-7.48480993131747,-0.270574496757375,
28.8918672333015));
#17567=CARTESIAN_POINT('Ctrl Pts',(-7.48353667075687,-0.00487092690990858,
28.9043481665497));
#17568=CARTESIAN_POINT('Ctrl Pts',(-7.48226341019626,0.260832642937558,
28.9168290997979));
#17569=CARTESIAN_POINT('Ctrl Pts',(-7.59019703546664,0.525433154238916,
28.9293100330461));
#17570=CARTESIAN_POINT('Ctrl Pts',(-7.77695120652398,0.714438148392058,
28.9417909662943));
#17571=CARTESIAN_POINT('Ctrl Pts',(-7.96370537758132,0.9034431425452,28.9542718995425));
#17572=CARTESIAN_POINT('Ctrl Pts',(-8.22699388814654,1.01453885915612,28.9667528327907));
#17573=CARTESIAN_POINT('Ctrl Pts',(-8.49269364458983,1.01644874085987,28.9792337660389));
#17574=CARTESIAN_POINT('Ctrl Pts',(-8.75839340103311,1.01835862256363,28.991714699287));
#17575=CARTESIAN_POINT('Ctrl Pts',(-9.02325176140227,0.911059288979904,
29.0041956325352));
#17576=CARTESIAN_POINT('Ctrl Pts',(-9.21270367535712,0.724758509268745,
29.0166765657834));
#17577=CARTESIAN_POINT('Ctrl Pts',(-9.40215558931197,0.538457729557587,
29.0291574990316));
#17578=CARTESIAN_POINT('Ctrl Pts',(-9.51388182535792,0.275436159674139,
29.0416384322798));
#17579=CARTESIAN_POINT('Ctrl Pts',(-9.51642831724056,0.00974174196606169,
29.054119365528));
#17580=CARTESIAN_POINT('Ctrl Pts',(-9.51645943884196,0.00649459406831602,
29.0542718995425));
#17581=CARTESIAN_POINT('Ctrl Pts',(-9.51647499999999,0.00324729703525258,
29.054424433557));
#17582=CARTESIAN_POINT('Ctrl Pts',(-9.516475,1.73256407251203E-12,29.0545769675714));
#17583=CARTESIAN_POINT('Origin',(-8.5,0.,1.24542303242842));
#17584=CARTESIAN_POINT('',(-9.516475,1.66178739415049E-12,28.3954230324284));
#17585=CARTESIAN_POINT('',(-9.51596463663996,-0.000112154843913254,28.4545769675714));
#17586=CARTESIAN_POINT('',(-9.516475,1.78524650477582E-12,1.24542303242842));
#17587=CARTESIAN_POINT('Ctrl Pts',(-9.516475,1.77734722252357E-12,28.3954230324284));
#17588=CARTESIAN_POINT('Ctrl Pts',(-9.51647500000047,-0.265706620582211,
28.4079039656766));
#17589=CARTESIAN_POINT('Ctrl Pts',(-9.40727465387286,-0.529786878175592,
28.4203848989248));
#17590=CARTESIAN_POINT('Ctrl Pts',(-9.21961691907877,-0.717894780173655,
28.432865832173));
#17591=CARTESIAN_POINT('Ctrl Pts',(-9.03195918428468,-0.906002682171718,
28.4453467654212));
#17592=CARTESIAN_POINT('Ctrl Pts',(-8.7681413283452,-1.01583545019872,28.4578276986694));
#17593=CARTESIAN_POINT('Ctrl Pts',(-8.50243547044643,-1.01647208230659,
28.4703086319176));
#17594=CARTESIAN_POINT('Ctrl Pts',(-8.23672961254766,-1.01710871441447,
28.4827895651658));
#17595=CARTESIAN_POINT('Ctrl Pts',(-7.97238846933455,-0.908541417083458,
28.4952704984139));
#17596=CARTESIAN_POINT('Ctrl Pts',(-7.78383148002433,-0.721334926799516,
28.5077514316621));
#17597=CARTESIAN_POINT('Ctrl Pts',(-7.59527449071412,-0.534128436515573,
28.5202323649103));
#17598=CARTESIAN_POINT('Ctrl Pts',(-7.48480993131737,-0.270574496757019,
28.5327132981585));
#17599=CARTESIAN_POINT('Ctrl Pts',(-7.48353667075686,-0.00487092690951304,
28.5451942314067));
#17600=CARTESIAN_POINT('Ctrl Pts',(-7.48226341019636,0.260832642937993,
28.5576751646549));
#17601=CARTESIAN_POINT('Ctrl Pts',(-7.59019703546688,0.525433154239346,
28.5701560979031));
#17602=CARTESIAN_POINT('Ctrl Pts',(-7.77695120652434,0.714438148392421,
28.5826370311513));
#17603=CARTESIAN_POINT('Ctrl Pts',(-7.9637053775818,0.903443142545497,28.5951179643995));
#17604=CARTESIAN_POINT('Ctrl Pts',(-8.22699388814713,1.01453885915629,28.6075988976477));
#17605=CARTESIAN_POINT('Ctrl Pts',(-8.49269364459045,1.01644874085988,28.6200798308959));
#17606=CARTESIAN_POINT('Ctrl Pts',(-8.75839340103378,1.01835862256347,28.6325607641441));
#17607=CARTESIAN_POINT('Ctrl Pts',(-9.0232517614029,0.911059288979549,28.6450416973922));
#17608=CARTESIAN_POINT('Ctrl Pts',(-9.21270367535765,0.724758509268225,
28.6575226306404));
#17609=CARTESIAN_POINT('Ctrl Pts',(-9.40215558931239,0.538457729556901,
28.6700035638886));
#17610=CARTESIAN_POINT('Ctrl Pts',(-9.51388182535815,0.275436159673322,
28.6824844971368));
#17611=CARTESIAN_POINT('Ctrl Pts',(-9.51642831724056,0.00974174196520395,
28.694965430385));
#17612=CARTESIAN_POINT('Ctrl Pts',(-9.51645943884196,0.0064945940677664,
28.6951179643995));
#17613=CARTESIAN_POINT('Ctrl Pts',(-9.51647499999999,0.00324729703501113,
28.6952704984139));
#17614=CARTESIAN_POINT('Ctrl Pts',(-9.516475,1.79926365491456E-12,28.6954230324284));
#17615=CARTESIAN_POINT('Ctrl Pts',(-9.51470232196842,-0.000389554669110295,
28.4545769675714));
#17616=CARTESIAN_POINT('Ctrl Pts',(-9.51530181937862,-0.130740653459931,
28.4606830615291));
#17617=CARTESIAN_POINT('Ctrl Pts',(-9.4616334089974,-0.430481838946053,
28.4747428260626));
#17618=CARTESIAN_POINT('Ctrl Pts',(-9.17050079378615,-0.816721293551335,
28.4967562611719));
#17619=CARTESIAN_POINT('Ctrl Pts',(-8.5410371348917,-1.12070821481403,28.5285709434751));
#17620=CARTESIAN_POINT('Ctrl Pts',(-7.62806957928328,-0.828287897936413,
28.5683392963542));
#17621=CARTESIAN_POINT('Ctrl Pts',(-7.33220907315438,0.286981604349355,
28.616061319809));
#17622=CARTESIAN_POINT('Ctrl Pts',(-8.10971802963793,1.13653082253137,28.6637833432638));
#17623=CARTESIAN_POINT('Ctrl Pts',(-9.20823837075766,0.950128537031716,
28.7099552258513));
#17624=CARTESIAN_POINT('Ctrl Pts',(-9.51583879936752,0.303640361218014,
28.7402197672872));
#17625=CARTESIAN_POINT('Ctrl Pts',(-9.5178552445993,-0.000844182403807882,
28.7545769675715));
#17626=CARTESIAN_POINT('Origin',(-8.5,0.,1.24542303242842));
#17627=CARTESIAN_POINT('',(-9.5167407851321,1.32517023624598E-5,28.0954230324284));
#17628=CARTESIAN_POINT('',(-9.516475,1.66681477533907E-12,28.1545769675714));
#17629=CARTESIAN_POINT('',(-9.516475,1.78524650477582E-12,1.24542303242842));
#17630=CARTESIAN_POINT('Ctrl Pts',(-9.51800967957185,7.65171274508918E-5,
28.0954230324284));
#17631=CARTESIAN_POINT('Ctrl Pts',(-9.51765220615975,-0.332868200880708,
28.1111343373136));
#17632=CARTESIAN_POINT('Ctrl Pts',(-9.15838448307071,-1.00358273601128,
28.1427529833504));
#17633=CARTESIAN_POINT('Ctrl Pts',(-8.01331019109225,-1.09975294067858,
28.1902789705388));
#17634=CARTESIAN_POINT('Ctrl Pts',(-7.43080495083982,-0.338367989046775,
28.2300473234179));
#17635=CARTESIAN_POINT('Ctrl Pts',(-7.50531901190296,0.356671722620504,
28.2618620057211));
#17636=CARTESIAN_POINT('Ctrl Pts',(-7.88944826933002,0.940689924117418,
28.2936766880244));
#17637=CARTESIAN_POINT('Ctrl Pts',(-8.8230477467519,1.15843154909714,28.3334450409034));
#17638=CARTESIAN_POINT('Ctrl Pts',(-9.45630261489437,0.541449066543569,
28.3700117125634));
#17639=CARTESIAN_POINT('Ctrl Pts',(-9.51678407727377,0.102067591494495,
28.3906710430717));
#17640=CARTESIAN_POINT('Ctrl Pts',(-9.51592367502213,0.000791130475659388,
28.3954230324284));
#17641=CARTESIAN_POINT('Ctrl Pts',(-9.516475,1.78237460371215E-12,28.1545769675714));
#17642=CARTESIAN_POINT('Ctrl Pts',(-9.51647500000047,-0.265706620582167,
28.1670579008196));
#17643=CARTESIAN_POINT('Ctrl Pts',(-9.4072746538729,-0.529786878175512,
28.1795388340678));
#17644=CARTESIAN_POINT('Ctrl Pts',(-9.21961691907885,-0.717894780173569,
28.192019767316));
#17645=CARTESIAN_POINT('Ctrl Pts',(-9.03195918428481,-0.906002682171627,
28.2045007005642));
#17646=CARTESIAN_POINT('Ctrl Pts',(-8.7681413283454,-1.01583545019866,28.2169816338124));
#17647=CARTESIAN_POINT('Ctrl Pts',(-8.50243547044666,-1.01647208230659,
28.2294625670606));
#17648=CARTESIAN_POINT('Ctrl Pts',(-8.23672961254793,-1.01710871441453,
28.2419435003088));
#17649=CARTESIAN_POINT('Ctrl Pts',(-7.97238846933483,-0.908541417083614,
28.254424433557));
#17650=CARTESIAN_POINT('Ctrl Pts',(-7.78383148002458,-0.721334926799763,
28.2669053668051));
#17651=CARTESIAN_POINT('Ctrl Pts',(-7.59527449071433,-0.534128436515913,
28.2793863000533));
#17652=CARTESIAN_POINT('Ctrl Pts',(-7.48480993131749,-0.270574496757447,
28.2918672333015));
#17653=CARTESIAN_POINT('Ctrl Pts',(-7.48353667075687,-0.00487092690998031,
28.3043481665497));
#17654=CARTESIAN_POINT('Ctrl Pts',(-7.48226341019624,0.260832642937486,
28.3168290997979));
#17655=CARTESIAN_POINT('Ctrl Pts',(-7.5901970354666,0.525433154238852,28.3293100330461));
#17656=CARTESIAN_POINT('Ctrl Pts',(-7.77695120652393,0.714438148392007,
28.3417909662943));
#17657=CARTESIAN_POINT('Ctrl Pts',(-7.96370537758126,0.903443142545162,
28.3542718995425));
#17658=CARTESIAN_POINT('Ctrl Pts',(-8.22699388814647,1.0145388591561,28.3667528327907));
#17659=CARTESIAN_POINT('Ctrl Pts',(-8.49269364458975,1.01644874085987,28.3792337660389));
#17660=CARTESIAN_POINT('Ctrl Pts',(-8.75839340103304,1.01835862256364,28.391714699287));
#17661=CARTESIAN_POINT('Ctrl Pts',(-9.0232517614022,0.911059288979941,28.4041956325352));
#17662=CARTESIAN_POINT('Ctrl Pts',(-9.21270367535707,0.724758509268796,
28.4166765657834));
#17663=CARTESIAN_POINT('Ctrl Pts',(-9.40215558931193,0.53845772955765,28.4291574990316));
#17664=CARTESIAN_POINT('Ctrl Pts',(-9.5138818253579,0.275436159674211,28.4416384322798));
#17665=CARTESIAN_POINT('Ctrl Pts',(-9.51642831724055,0.00974174196613341,
28.454119365528));
#17666=CARTESIAN_POINT('Ctrl Pts',(-9.51645943884196,0.00649459406834922,
28.4542718995425));
#17667=CARTESIAN_POINT('Ctrl Pts',(-9.51647499999999,0.00324729703524735,
28.454424433557));
#17668=CARTESIAN_POINT('Ctrl Pts',(-9.516475,1.68873120773006E-12,28.4545769675714));
#17669=CARTESIAN_POINT('Origin',(-8.5,0.,1.24542303242842));
#17670=CARTESIAN_POINT('',(-9.516475,1.61795452936852E-12,27.7954230324284));
#17671=CARTESIAN_POINT('',(-9.51669945074544,6.82738928919885E-5,27.8545769675714));
#17672=CARTESIAN_POINT('',(-9.516475,1.78524650477582E-12,1.24542303242842));
#17673=CARTESIAN_POINT('Ctrl Pts',(-9.516475,1.7335143577416E-12,27.7954230324284));
#17674=CARTESIAN_POINT('Ctrl Pts',(-9.51647500000045,-0.265706620582254,
27.8079039656766));
#17675=CARTESIAN_POINT('Ctrl Pts',(-9.40727465387284,-0.529786878175631,
27.8203848989248));
#17676=CARTESIAN_POINT('Ctrl Pts',(-9.21961691907874,-0.717894780173686,
27.832865832173));
#17677=CARTESIAN_POINT('Ctrl Pts',(-9.03195918428464,-0.906002682171741,
27.8453467654212));
#17678=CARTESIAN_POINT('Ctrl Pts',(-8.76814132834516,-1.01583545019873,
27.8578276986694));
#17679=CARTESIAN_POINT('Ctrl Pts',(-8.50243547044638,-1.01647208230659,
27.8703086319176));
#17680=CARTESIAN_POINT('Ctrl Pts',(-8.23672961254761,-1.01710871441446,
27.8827895651658));
#17681=CARTESIAN_POINT('Ctrl Pts',(-7.97238846933451,-0.908541417083436,
27.895270498414));
#17682=CARTESIAN_POINT('Ctrl Pts',(-7.7838314800243,-0.721334926799485,
27.9077514316621));
#17683=CARTESIAN_POINT('Ctrl Pts',(-7.5952744907141,-0.534128436515534,
27.9202323649103));
#17684=CARTESIAN_POINT('Ctrl Pts',(-7.48480993131736,-0.270574496756975,
27.9327132981585));
#17685=CARTESIAN_POINT('Ctrl Pts',(-7.48353667075686,-0.00487092690946921,
27.9451942314067));
#17686=CARTESIAN_POINT('Ctrl Pts',(-7.48226341019637,0.260832642938037,
27.9576751646549));
#17687=CARTESIAN_POINT('Ctrl Pts',(-7.5901970354669,0.525433154239385,27.9701560979031));
#17688=CARTESIAN_POINT('Ctrl Pts',(-7.77695120652437,0.714438148392453,
27.9826370311513));
#17689=CARTESIAN_POINT('Ctrl Pts',(-7.96370537758184,0.90344314254552,27.9951179643995));
#17690=CARTESIAN_POINT('Ctrl Pts',(-8.22699388814717,1.0145388591563,28.0075988976477));
#17691=CARTESIAN_POINT('Ctrl Pts',(-8.4926936445905,1.01644874085988,28.0200798308959));
#17692=CARTESIAN_POINT('Ctrl Pts',(-8.75839340103382,1.01835862256346,28.0325607641441));
#17693=CARTESIAN_POINT('Ctrl Pts',(-9.02325176140294,0.911059288979527,
28.0450416973922));
#17694=CARTESIAN_POINT('Ctrl Pts',(-9.21270367535768,0.724758509268194,
28.0575226306404));
#17695=CARTESIAN_POINT('Ctrl Pts',(-9.40215558931241,0.538457729556862,
28.0700035638886));
#17696=CARTESIAN_POINT('Ctrl Pts',(-9.51388182535816,0.275436159673279,
28.0824844971368));
#17697=CARTESIAN_POINT('Ctrl Pts',(-9.51642831724056,0.00974174196516012,
28.094965430385));
#17698=CARTESIAN_POINT('Ctrl Pts',(-9.51645943884196,0.00649459406768405,
28.0951179643995));
#17699=CARTESIAN_POINT('Ctrl Pts',(-9.51647499999999,0.00324729703489034,
28.095270498414));
#17700=CARTESIAN_POINT('Ctrl Pts',(-9.516475,1.63987096175951E-12,28.0954230324284));
#17701=CARTESIAN_POINT('Ctrl Pts',(-9.51761484906871,0.000346721644969969,
27.8545769675714));
#17702=CARTESIAN_POINT('Ctrl Pts',(-9.51603164570953,-0.322453934885924,
27.8697949677096));
#17703=CARTESIAN_POINT('Ctrl Pts',(-9.17770066316481,-0.98391483713693,
27.9009203089995));
#17704=CARTESIAN_POINT('Ctrl Pts',(-8.04802974380756,-1.1143684208142,27.9479529914409));
#17705=CARTESIAN_POINT('Ctrl Pts',(-7.31915026362204,-0.222747002236805,
27.9956750148958));
#17706=CARTESIAN_POINT('Ctrl Pts',(-7.67312128813442,0.873135548270785,
28.0433970383507));
#17707=CARTESIAN_POINT('Ctrl Pts',(-8.78880236016895,1.16744023289704,28.0911190618055));
#17708=CARTESIAN_POINT('Ctrl Pts',(-9.44635199105584,0.562681634430224,
28.1281790382124));
#17709=CARTESIAN_POINT('Ctrl Pts',(-9.51666892397189,0.112429099594727,
28.1493316734677));
#17710=CARTESIAN_POINT('Ctrl Pts',(-9.5160973699535,0.000575295411255838,
28.1545769675714));
#17711=CARTESIAN_POINT('Origin',(-8.5,0.,1.24542303242842));
#17712=CARTESIAN_POINT('',(-9.516475,1.59603809697754E-12,27.4954230324284));
#17713=CARTESIAN_POINT('',(-9.516475,1.6229819105571E-12,27.5545769675714));
#17714=CARTESIAN_POINT('',(-9.516475,1.78524650477582E-12,1.24542303242842));
#17715=CARTESIAN_POINT('Ctrl Pts',(-9.516475,1.59603809697754E-12,27.4954230324284));
#17716=CARTESIAN_POINT('Ctrl Pts',(-9.51647500000042,-0.26570662058243,
27.5079039656766));
#17717=CARTESIAN_POINT('Ctrl Pts',(-9.40727465387273,-0.52978687817583,
27.5203848989248));
#17718=CARTESIAN_POINT('Ctrl Pts',(-9.21961691907856,-0.717894780173865,
27.532865832173));
#17719=CARTESIAN_POINT('Ctrl Pts',(-9.03195918428438,-0.9060026821719,27.5453467654212));
#17720=CARTESIAN_POINT('Ctrl Pts',(-8.76814132834483,-1.01583545019883,
27.5578276986694));
#17721=CARTESIAN_POINT('Ctrl Pts',(-8.50243547044602,-1.0164720823066,27.5703086319176));
#17722=CARTESIAN_POINT('Ctrl Pts',(-8.23672961254721,-1.01710871441436,
27.5827895651658));
#17723=CARTESIAN_POINT('Ctrl Pts',(-7.9723884693341,-0.908541417083211,
27.595270498414));
#17724=CARTESIAN_POINT('Ctrl Pts',(-7.78383148002396,-0.721334926799144,
27.6077514316622));
#17725=CARTESIAN_POINT('Ctrl Pts',(-7.59527449071382,-0.534128436515076,
27.6202323649104));
#17726=CARTESIAN_POINT('Ctrl Pts',(-7.4848099313172,-0.270574496756415,
27.6327132981586));
#17727=CARTESIAN_POINT('Ctrl Pts',(-7.48353667075686,-0.0048709269088695,
27.6451942314067));
#17728=CARTESIAN_POINT('Ctrl Pts',(-7.48226341019652,0.260832642938676,
27.6576751646549));
#17729=CARTESIAN_POINT('Ctrl Pts',(-7.59019703546725,0.525433154239998,
27.6701560979031));
#17730=CARTESIAN_POINT('Ctrl Pts',(-7.77695120652487,0.714438148392961,
27.6826370311513));
#17731=CARTESIAN_POINT('Ctrl Pts',(-7.9637053775825,0.903443142545925,27.6951179643995));
#17732=CARTESIAN_POINT('Ctrl Pts',(-8.22699388814796,1.01453885915652,27.7075988976477));
#17733=CARTESIAN_POINT('Ctrl Pts',(-8.49269364459133,1.01644874085988,27.7200798308959));
#17734=CARTESIAN_POINT('Ctrl Pts',(-8.75839340103469,1.01835862256324,27.7325607641441));
#17735=CARTESIAN_POINT('Ctrl Pts',(-9.02325176140376,0.911059288979067,
27.7450416973923));
#17736=CARTESIAN_POINT('Ctrl Pts',(-9.21270367535835,0.724758509267531,
27.7575226306405));
#17737=CARTESIAN_POINT('Ctrl Pts',(-9.40215558931294,0.538457729555995,
27.7700035638887));
#17738=CARTESIAN_POINT('Ctrl Pts',(-9.51388182535845,0.275436159672258,
27.7824844971369));
#17739=CARTESIAN_POINT('Ctrl Pts',(-9.51642831724057,0.00974174196409821,
27.7949654303851));
#17740=CARTESIAN_POINT('Ctrl Pts',(-9.51645943884197,0.00649459406700729,
27.7951179643995));
#17741=CARTESIAN_POINT('Ctrl Pts',(-9.51647499999999,0.0032472970345988,
27.795270498414));
#17742=CARTESIAN_POINT('Ctrl Pts',(-9.516475,1.7335143577416E-12,27.7954230324284));
#17743=CARTESIAN_POINT('Ctrl Pts',(-9.516475,1.6229819105571E-12,27.5545769675714));
#17744=CARTESIAN_POINT('Ctrl Pts',(-9.51647500000042,-0.265706620582365,
27.5670579008196));
#17745=CARTESIAN_POINT('Ctrl Pts',(-9.40727465387278,-0.52978687817573,
27.5795388340678));
#17746=CARTESIAN_POINT('Ctrl Pts',(-9.21961691907866,-0.717894780173764,
27.592019767316));
#17747=CARTESIAN_POINT('Ctrl Pts',(-9.03195918428454,-0.906002682171798,
27.6045007005642));
#17748=CARTESIAN_POINT('Ctrl Pts',(-8.76814132834505,-1.01583545019876,
27.6169816338124));
#17749=CARTESIAN_POINT('Ctrl Pts',(-8.50243547044627,-1.01647208230659,
27.6294625670606));
#17750=CARTESIAN_POINT('Ctrl Pts',(-8.2367296125475,-1.01710871441443,27.6419435003088));
#17751=CARTESIAN_POINT('Ctrl Pts',(-7.97238846933441,-0.908541417083378,
27.654424433557));
#17752=CARTESIAN_POINT('Ctrl Pts',(-7.78383148002422,-0.721334926799407,
27.6669053668052));
#17753=CARTESIAN_POINT('Ctrl Pts',(-7.59527449071404,-0.534128436515436,
27.6793863000534));
#17754=CARTESIAN_POINT('Ctrl Pts',(-7.48480993131733,-0.270574496756865,
27.6918672333016));
#17755=CARTESIAN_POINT('Ctrl Pts',(-7.48353667075686,-0.00487092690935868,
27.7043481665497));
#17756=CARTESIAN_POINT('Ctrl Pts',(-7.4822634101964,0.260832642938147,27.7168290997979));
#17757=CARTESIAN_POINT('Ctrl Pts',(-7.59019703546696,0.525433154239484,
27.7293100330461));
#17758=CARTESIAN_POINT('Ctrl Pts',(-7.77695120652445,0.714438148392531,
27.7417909662943));
#17759=CARTESIAN_POINT('Ctrl Pts',(-7.96370537758194,0.903443142545578,
27.7542718995425));
#17760=CARTESIAN_POINT('Ctrl Pts',(-8.22699388814728,1.01453885915633,27.7667528327907));
#17761=CARTESIAN_POINT('Ctrl Pts',(-8.49269364459061,1.01644874085988,27.7792337660389));
#17762=CARTESIAN_POINT('Ctrl Pts',(-8.75839340103393,1.01835862256343,27.7917146992871));
#17763=CARTESIAN_POINT('Ctrl Pts',(-9.02325176140304,0.91105928897947,27.8041956325353));
#17764=CARTESIAN_POINT('Ctrl Pts',(-9.21270367535776,0.724758509268117,
27.8166765657835));
#17765=CARTESIAN_POINT('Ctrl Pts',(-9.40215558931247,0.538457729556764,
27.8291574990317));
#17766=CARTESIAN_POINT('Ctrl Pts',(-9.51388182535819,0.275436159673168,
27.8416384322799));
#17767=CARTESIAN_POINT('Ctrl Pts',(-9.51642831724056,0.00974174196504959,
27.854119365528));
#17768=CARTESIAN_POINT('Ctrl Pts',(-9.51645943884196,0.00649459406765055,
27.8542718995425));
#17769=CARTESIAN_POINT('Ctrl Pts',(-9.51647499999999,0.00324729703493389,
27.854424433557));
#17770=CARTESIAN_POINT('Ctrl Pts',(-9.516475,1.76045817132117E-12,27.8545769675714));
#17771=CARTESIAN_POINT('Origin',(-8.5,0.,1.24542303242842));
#17772=CARTESIAN_POINT('',(-9.516475,1.57412166458655E-12,27.1954230324284));
#17773=CARTESIAN_POINT('',(-9.516475,1.60106547816612E-12,27.2545769675714));
#17774=CARTESIAN_POINT('',(-9.516475,1.78524650477582E-12,1.24542303242842));
#17775=CARTESIAN_POINT('Ctrl Pts',(-9.516475,1.57412166458655E-12,27.1954230324284));
#17776=CARTESIAN_POINT('Ctrl Pts',(-9.51647500000041,-0.265706620582452,
27.2079039656766));
#17777=CARTESIAN_POINT('Ctrl Pts',(-9.40727465387272,-0.529786878175849,
27.2203848989248));
#17778=CARTESIAN_POINT('Ctrl Pts',(-9.21961691907854,-0.71789478017388,
27.232865832173));
#17779=CARTESIAN_POINT('Ctrl Pts',(-9.03195918428436,-0.906002682171912,
27.2453467654212));
#17780=CARTESIAN_POINT('Ctrl Pts',(-8.7681413283448,-1.01583545019883,27.2578276986694));
#17781=CARTESIAN_POINT('Ctrl Pts',(-8.50243547044599,-1.0164720823066,27.2703086319176));
#17782=CARTESIAN_POINT('Ctrl Pts',(-8.23672961254718,-1.01710871441436,
27.2827895651658));
#17783=CARTESIAN_POINT('Ctrl Pts',(-7.97238846933408,-0.9085414170832,27.295270498414));
#17784=CARTESIAN_POINT('Ctrl Pts',(-7.78383148002394,-0.721334926799128,
27.3077514316622));
#17785=CARTESIAN_POINT('Ctrl Pts',(-7.59527449071381,-0.534128436515056,
27.3202323649104));
#17786=CARTESIAN_POINT('Ctrl Pts',(-7.48480993131719,-0.270574496756393,
27.3327132981586));
#17787=CARTESIAN_POINT('Ctrl Pts',(-7.48353667075686,-0.00487092690884759,
27.3451942314067));
#17788=CARTESIAN_POINT('Ctrl Pts',(-7.48226341019653,0.260832642938698,
27.3576751646549));
#17789=CARTESIAN_POINT('Ctrl Pts',(-7.59019703546726,0.525433154240017,
27.3701560979031));
#17790=CARTESIAN_POINT('Ctrl Pts',(-7.77695120652489,0.714438148392977,
27.3826370311513));
#17791=CARTESIAN_POINT('Ctrl Pts',(-7.96370537758252,0.903443142545937,
27.3951179643995));
#17792=CARTESIAN_POINT('Ctrl Pts',(-8.22699388814799,1.01453885915653,27.4075988976477));
#17793=CARTESIAN_POINT('Ctrl Pts',(-8.49269364459135,1.01644874085988,27.4200798308959));
#17794=CARTESIAN_POINT('Ctrl Pts',(-8.75839340103471,1.01835862256324,27.4325607641441));
#17795=CARTESIAN_POINT('Ctrl Pts',(-9.02325176140378,0.911059288979055,
27.4450416973923));
#17796=CARTESIAN_POINT('Ctrl Pts',(-9.21270367535837,0.724758509267516,
27.4575226306405));
#17797=CARTESIAN_POINT('Ctrl Pts',(-9.40215558931296,0.538457729555976,
27.4700035638887));
#17798=CARTESIAN_POINT('Ctrl Pts',(-9.51388182535846,0.275436159672236,
27.4824844971369));
#17799=CARTESIAN_POINT('Ctrl Pts',(-9.51642831724057,0.00974174196407629,
27.4949654303851));
#17800=CARTESIAN_POINT('Ctrl Pts',(-9.51645943884197,0.00649459406694685,
27.4951179643995));
#17801=CARTESIAN_POINT('Ctrl Pts',(-9.51647499999999,0.00324729703449976,
27.495270498414));
#17802=CARTESIAN_POINT('Ctrl Pts',(-9.516475,1.59603809697754E-12,27.4954230324284));
#17803=CARTESIAN_POINT('Ctrl Pts',(-9.516475,1.60106547816612E-12,27.2545769675714));
#17804=CARTESIAN_POINT('Ctrl Pts',(-9.51647500000042,-0.265706620582425,
27.2670579008196));
#17805=CARTESIAN_POINT('Ctrl Pts',(-9.40727465387274,-0.529786878175825,
27.2795388340678));
#17806=CARTESIAN_POINT('Ctrl Pts',(-9.21961691907856,-0.717894780173861,
27.292019767316));
#17807=CARTESIAN_POINT('Ctrl Pts',(-9.03195918428439,-0.906002682171897,
27.3045007005642));
#17808=CARTESIAN_POINT('Ctrl Pts',(-8.76814132834483,-1.01583545019883,
27.3169816338124));
#17809=CARTESIAN_POINT('Ctrl Pts',(-8.50243547044602,-1.0164720823066,27.3294625670606));
#17810=CARTESIAN_POINT('Ctrl Pts',(-8.23672961254721,-1.01710871441436,
27.3419435003088));
#17811=CARTESIAN_POINT('Ctrl Pts',(-7.97238846933411,-0.908541417083214,
27.354424433557));
#17812=CARTESIAN_POINT('Ctrl Pts',(-7.78383148002396,-0.721334926799147,
27.3669053668052));
#17813=CARTESIAN_POINT('Ctrl Pts',(-7.59527449071382,-0.53412843651508,
27.3793863000534));
#17814=CARTESIAN_POINT('Ctrl Pts',(-7.4848099313172,-0.27057449675642,27.3918672333016));
#17815=CARTESIAN_POINT('Ctrl Pts',(-7.48353667075686,-0.00487092690887453,
27.4043481665498));
#17816=CARTESIAN_POINT('Ctrl Pts',(-7.48226341019652,0.260832642938671,
27.416829099798));
#17817=CARTESIAN_POINT('Ctrl Pts',(-7.59019703546724,0.525433154239993,
27.4293100330462));
#17818=CARTESIAN_POINT('Ctrl Pts',(-7.77695120652487,0.714438148392958,
27.4417909662943));
#17819=CARTESIAN_POINT('Ctrl Pts',(-7.9637053775825,0.903443142545922,27.4542718995425));
#17820=CARTESIAN_POINT('Ctrl Pts',(-8.22699388814796,1.01453885915652,27.4667528327907));
#17821=CARTESIAN_POINT('Ctrl Pts',(-8.49269364459132,1.01644874085988,27.4792337660389));
#17822=CARTESIAN_POINT('Ctrl Pts',(-8.75839340103469,1.01835862256325,27.4917146992871));
#17823=CARTESIAN_POINT('Ctrl Pts',(-9.02325176140376,0.911059288979069,
27.5041956325353));
#17824=CARTESIAN_POINT('Ctrl Pts',(-9.21270367535835,0.724758509267534,
27.5166765657835));
#17825=CARTESIAN_POINT('Ctrl Pts',(-9.40215558931294,0.538457729555999,
27.5291574990317));
#17826=CARTESIAN_POINT('Ctrl Pts',(-9.51388182535845,0.275436159672263,
27.5416384322799));
#17827=CARTESIAN_POINT('Ctrl Pts',(-9.51642831724057,0.00974174196410324,
27.5541193655281));
#17828=CARTESIAN_POINT('Ctrl Pts',(-9.51645943884197,0.0064945940669738,
27.5542718995425));
#17829=CARTESIAN_POINT('Ctrl Pts',(-9.51647499999999,0.0032472970345267,
27.554424433557));
#17830=CARTESIAN_POINT('Ctrl Pts',(-9.516475,1.6229819105571E-12,27.5545769675714));
#17831=CARTESIAN_POINT('Origin',(-8.5,0.,1.24542303242842));
#17832=CARTESIAN_POINT('',(-9.516475,1.55220523219556E-12,26.8954230324284));
#17833=CARTESIAN_POINT('',(-9.516475,1.57914904577513E-12,26.9545769675715));
#17834=CARTESIAN_POINT('',(-9.516475,1.78524650477582E-12,1.24542303242842));
#17835=CARTESIAN_POINT('Ctrl Pts',(-9.516475,1.55220523219556E-12,26.8954230324284));
#17836=CARTESIAN_POINT('Ctrl Pts',(-9.5164750000004,-0.26570662058232,26.9079039656766));
#17837=CARTESIAN_POINT('Ctrl Pts',(-9.40727465387284,-0.529786878175565,
26.9203848989248));
#17838=CARTESIAN_POINT('Ctrl Pts',(-9.21961691907885,-0.717894780173569,
26.932865832173));
#17839=CARTESIAN_POINT('Ctrl Pts',(-9.03195918428486,-0.906002682171572,
26.9453467654212));
#17840=CARTESIAN_POINT('Ctrl Pts',(-8.76814132834555,-1.0158354501986,26.9578276986694));
#17841=CARTESIAN_POINT('Ctrl Pts',(-8.5024354704469,-1.01647208230659,26.9703086319175));
#17842=CARTESIAN_POINT('Ctrl Pts',(-8.23672961254824,-1.01710871441459,
26.9827895651657));
#17843=CARTESIAN_POINT('Ctrl Pts',(-7.97238846933519,-0.9085414170838,26.9952704984139));
#17844=CARTESIAN_POINT('Ctrl Pts',(-7.78383148002491,-0.72133492680009,
27.0077514316621));
#17845=CARTESIAN_POINT('Ctrl Pts',(-7.59527449071463,-0.53412843651638,
27.0202323649103));
#17846=CARTESIAN_POINT('Ctrl Pts',(-7.48480993131768,-0.270574496758063,
27.0327132981585));
#17847=CARTESIAN_POINT('Ctrl Pts',(-7.48353667075687,-0.00487092691067461,
27.0451942314067));
#17848=CARTESIAN_POINT('Ctrl Pts',(-7.48226341019606,0.260832642936714,
27.0576751646548));
#17849=CARTESIAN_POINT('Ctrl Pts',(-7.59019703546618,0.525433154238078,
27.070156097903));
#17850=CARTESIAN_POINT('Ctrl Pts',(-7.77695120652328,0.714438148391349,
27.0826370311512));
#17851=CARTESIAN_POINT('Ctrl Pts',(-7.96370537758038,0.903443142544619,
27.0951179643994));
#17852=CARTESIAN_POINT('Ctrl Pts',(-8.22699388814539,1.01453885915579,27.1075988976476));
#17853=CARTESIAN_POINT('Ctrl Pts',(-8.4926936445886,1.01644874085986,27.1200798308958));
#17854=CARTESIAN_POINT('Ctrl Pts',(-8.7583934010318,1.01835862256394,27.132560764144));
#17855=CARTESIAN_POINT('Ctrl Pts',(-9.02325176140101,0.911059288980602,
27.1450416973921));
#17856=CARTESIAN_POINT('Ctrl Pts',(-9.21270367535608,0.724758509269769,
27.1575226306403));
#17857=CARTESIAN_POINT('Ctrl Pts',(-9.40215558931114,0.538457729558936,
27.1700035638885));
#17858=CARTESIAN_POINT('Ctrl Pts',(-9.51388182535746,0.275436159675749,
27.1824844971367));
#17859=CARTESIAN_POINT('Ctrl Pts',(-9.51642831724054,0.00974174196775212,
27.1949654303849));
#17860=CARTESIAN_POINT('Ctrl Pts',(-9.51645943884195,0.00649459406939021,
27.1951179643994));
#17861=CARTESIAN_POINT('Ctrl Pts',(-9.51647499999999,0.00324729703571043,
27.1952704984139));
#17862=CARTESIAN_POINT('Ctrl Pts',(-9.516475,1.57412166458655E-12,27.1954230324284));
#17863=CARTESIAN_POINT('Ctrl Pts',(-9.516475,1.57914904577513E-12,26.9545769675715));
#17864=CARTESIAN_POINT('Ctrl Pts',(-9.51647500000041,-0.265706620582332,
26.9670579008196));
#17865=CARTESIAN_POINT('Ctrl Pts',(-9.40727465387283,-0.529786878175617,
26.9795388340678));
#17866=CARTESIAN_POINT('Ctrl Pts',(-9.21961691907879,-0.717894780173631,
26.992019767316));
#17867=CARTESIAN_POINT('Ctrl Pts',(-9.03195918428476,-0.906002682171646,
27.0045007005642));
#17868=CARTESIAN_POINT('Ctrl Pts',(-8.76814132834539,-1.01583545019865,
27.0169816338124));
#17869=CARTESIAN_POINT('Ctrl Pts',(-8.50243547044669,-1.01647208230659,
27.0294625670606));
#17870=CARTESIAN_POINT('Ctrl Pts',(-8.236729612548,-1.01710871441454,27.0419435003088));
#17871=CARTESIAN_POINT('Ctrl Pts',(-7.97238846933493,-0.908541417083661,
27.054424433557));
#17872=CARTESIAN_POINT('Ctrl Pts',(-7.78383148002468,-0.721334926799864,
27.0669053668051));
#17873=CARTESIAN_POINT('Ctrl Pts',(-7.59527449071444,-0.534128436516068,
27.0793863000533));
#17874=CARTESIAN_POINT('Ctrl Pts',(-7.48480993131756,-0.270574496757667,
27.0918672333015));
#17875=CARTESIAN_POINT('Ctrl Pts',(-7.48353667075687,-0.00487092691023932,
27.1043481665497));
#17876=CARTESIAN_POINT('Ctrl Pts',(-7.48226341019617,0.260832642937188,
27.1168290997979));
#17877=CARTESIAN_POINT('Ctrl Pts',(-7.59019703546644,0.525433154238544,
27.1293100330461));
#17878=CARTESIAN_POINT('Ctrl Pts',(-7.77695120652367,0.71443814839174,27.1417909662943));
#17879=CARTESIAN_POINT('Ctrl Pts',(-7.9637053775809,0.903443142544937,27.1542718995425));
#17880=CARTESIAN_POINT('Ctrl Pts',(-8.22699388814602,1.01453885915597,27.1667528327906));
#17881=CARTESIAN_POINT('Ctrl Pts',(-8.49269364458926,1.01644874085987,27.1792337660388));
#17882=CARTESIAN_POINT('Ctrl Pts',(-8.75839340103251,1.01835862256377,27.191714699287));
#17883=CARTESIAN_POINT('Ctrl Pts',(-9.02325176140169,0.911059288980226,
27.2041956325352));
#17884=CARTESIAN_POINT('Ctrl Pts',(-9.21270367535664,0.72475850926922,27.2166765657834));
#17885=CARTESIAN_POINT('Ctrl Pts',(-9.40215558931158,0.538457729558215,
27.2291574990316));
#17886=CARTESIAN_POINT('Ctrl Pts',(-9.5138818253577,0.275436159674892,27.2416384322798));
#17887=CARTESIAN_POINT('Ctrl Pts',(-9.51642831724055,0.00974174196685463,
27.254119365528));
#17888=CARTESIAN_POINT('Ctrl Pts',(-9.51645943884196,0.00649459406880084,
27.2542718995425));
#17889=CARTESIAN_POINT('Ctrl Pts',(-9.51647499999999,0.00324729703542923,
27.254424433557));
#17890=CARTESIAN_POINT('Ctrl Pts',(-9.516475,1.60106547816612E-12,27.2545769675714));
#17891=CARTESIAN_POINT('Origin',(-8.5,0.,1.24542303242842));
#17892=CARTESIAN_POINT('',(-9.516475,1.53028879980458E-12,26.5954230324284));
#17893=CARTESIAN_POINT('',(-9.51655216780646,-3.99696456298066E-5,26.6545769675714));
#17894=CARTESIAN_POINT('',(-9.516475,1.78524650477582E-12,1.24542303242842));
#17895=CARTESIAN_POINT('Ctrl Pts',(-9.516475,1.64584862817766E-12,26.5954230324284));
#17896=CARTESIAN_POINT('Ctrl Pts',(-9.51647500000043,-0.265706620582265,
26.6079039656766));
#17897=CARTESIAN_POINT('Ctrl Pts',(-9.40727465387286,-0.529786878175558,
26.6203848989248));
#17898=CARTESIAN_POINT('Ctrl Pts',(-9.21961691907884,-0.717894780173584,
26.632865832173));
#17899=CARTESIAN_POINT('Ctrl Pts',(-9.03195918428482,-0.906002682171611,
26.6453467654212));
#17900=CARTESIAN_POINT('Ctrl Pts',(-8.76814132834545,-1.01583545019863,
26.6578276986694));
#17901=CARTESIAN_POINT('Ctrl Pts',(-8.50243547044676,-1.01647208230659,
26.6703086319175));
#17902=CARTESIAN_POINT('Ctrl Pts',(-8.23672961254806,-1.01710871441456,
26.6827895651657));
#17903=CARTESIAN_POINT('Ctrl Pts',(-7.97238846933499,-0.908541417083696,
26.6952704984139));
#17904=CARTESIAN_POINT('Ctrl Pts',(-7.78383148002473,-0.721334926799912,
26.7077514316621));
#17905=CARTESIAN_POINT('Ctrl Pts',(-7.59527449071447,-0.534128436516127,
26.7202323649103));
#17906=CARTESIAN_POINT('Ctrl Pts',(-7.48480993131758,-0.270574496757734,
26.7327132981585));
#17907=CARTESIAN_POINT('Ctrl Pts',(-7.48353667075687,-0.00487092691030601,
26.7451942314067));
#17908=CARTESIAN_POINT('Ctrl Pts',(-7.48226341019616,0.260832642937122,
26.7576751646549));
#17909=CARTESIAN_POINT('Ctrl Pts',(-7.5901970354664,0.525433154238484,26.7701560979031));
#17910=CARTESIAN_POINT('Ctrl Pts',(-7.77695120652362,0.714438148391693,
26.7826370311512));
#17911=CARTESIAN_POINT('Ctrl Pts',(-7.96370537758084,0.903443142544902,
26.7951179643994));
#17912=CARTESIAN_POINT('Ctrl Pts',(-8.22699388814596,1.01453885915595,26.8075988976476));
#17913=CARTESIAN_POINT('Ctrl Pts',(-8.4926936445892,1.01644874085987,26.8200798308958));
#17914=CARTESIAN_POINT('Ctrl Pts',(-8.75839340103244,1.01835862256379,26.832560764144));
#17915=CARTESIAN_POINT('Ctrl Pts',(-9.02325176140163,0.911059288980261,
26.8450416973922));
#17916=CARTESIAN_POINT('Ctrl Pts',(-9.21270367535659,0.724758509269267,
26.8575226306404));
#17917=CARTESIAN_POINT('Ctrl Pts',(-9.40215558931155,0.538457729558274,
26.8700035638886));
#17918=CARTESIAN_POINT('Ctrl Pts',(-9.51388182535769,0.275436159674958,
26.8824844971367));
#17919=CARTESIAN_POINT('Ctrl Pts',(-9.51642831724055,0.00974174196692133,
26.8949654303849));
#17920=CARTESIAN_POINT('Ctrl Pts',(-9.51645943884196,0.00649459406882902,
26.8951179643994));
#17921=CARTESIAN_POINT('Ctrl Pts',(-9.51647499999999,0.00324729703541897,
26.8952704984139));
#17922=CARTESIAN_POINT('Ctrl Pts',(-9.516475,1.55220523219556E-12,26.8954230324284));
#17923=CARTESIAN_POINT('Ctrl Pts',(-9.516475,1.55723261338415E-12,26.6545769675715));
#17924=CARTESIAN_POINT('Ctrl Pts',(-9.51647500000041,-0.265706620582431,
26.6670579008196));
#17925=CARTESIAN_POINT('Ctrl Pts',(-9.40727465387275,-0.529786878175788,
26.6795388340678));
#17926=CARTESIAN_POINT('Ctrl Pts',(-9.21961691907861,-0.71789478017381,
26.692019767316));
#17927=CARTESIAN_POINT('Ctrl Pts',(-9.03195918428448,-0.906002682171833,
26.7045007005642));
#17928=CARTESIAN_POINT('Ctrl Pts',(-8.76814132834498,-1.01583545019878,
26.7169816338124));
#17929=CARTESIAN_POINT('Ctrl Pts',(-8.50243547044621,-1.0164720823066,26.7294625670606));
#17930=CARTESIAN_POINT('Ctrl Pts',(-8.23672961254744,-1.01710871441441,
26.7419435003088));
#17931=CARTESIAN_POINT('Ctrl Pts',(-7.97238846933435,-0.908541417083344,
26.754424433557));
#17932=CARTESIAN_POINT('Ctrl Pts',(-7.78383148002418,-0.721334926799361,
26.7669053668052));
#17933=CARTESIAN_POINT('Ctrl Pts',(-7.59527449071401,-0.534128436515377,
26.7793863000534));
#17934=CARTESIAN_POINT('Ctrl Pts',(-7.48480993131731,-0.270574496756799,
26.7918672333016));
#17935=CARTESIAN_POINT('Ctrl Pts',(-7.48353667075686,-0.00487092690929293,
26.8043481665497));
#17936=CARTESIAN_POINT('Ctrl Pts',(-7.48226341019642,0.260832642938213,
26.8168290997979));
#17937=CARTESIAN_POINT('Ctrl Pts',(-7.59019703546699,0.525433154239543,
26.8293100330461));
#17938=CARTESIAN_POINT('Ctrl Pts',(-7.77695120652449,0.714438148392578,
26.8417909662943));
#17939=CARTESIAN_POINT('Ctrl Pts',(-7.963705377582,0.903443142545613,26.8542718995425));
#17940=CARTESIAN_POINT('Ctrl Pts',(-8.22699388814735,1.01453885915635,26.8667528327907));
#17941=CARTESIAN_POINT('Ctrl Pts',(-8.49269364459067,1.01644874085988,26.8792337660389));
#17942=CARTESIAN_POINT('Ctrl Pts',(-8.758393401034,1.01835862256341,26.8917146992871));
#17943=CARTESIAN_POINT('Ctrl Pts',(-9.0232517614031,0.911059288979436,26.9041956325353));
#17944=CARTESIAN_POINT('Ctrl Pts',(-9.2127036753578,0.724758509268071,26.9166765657835));
#17945=CARTESIAN_POINT('Ctrl Pts',(-9.40215558931251,0.538457729556705,
26.9291574990317));
#17946=CARTESIAN_POINT('Ctrl Pts',(-9.51388182535821,0.275436159673103,
26.9416384322799));
#17947=CARTESIAN_POINT('Ctrl Pts',(-9.51642831724057,0.00974174196498384,
26.954119365528));
#17948=CARTESIAN_POINT('Ctrl Pts',(-9.51645943884196,0.00649459406754628,
26.9542718995425));
#17949=CARTESIAN_POINT('Ctrl Pts',(-9.51647499999999,0.00324729703479102,
26.954424433557));
#17950=CARTESIAN_POINT('Ctrl Pts',(-9.516475,1.57914904577513E-12,26.9545769675715));
#17951=CARTESIAN_POINT('Origin',(-8.5,0.,1.24542303242842));
#17952=CARTESIAN_POINT('',(-9.516475,1.50837236741359E-12,26.2954230324284));
#17953=CARTESIAN_POINT('',(-9.51621740714814,-0.000106417722281503,26.3545769675715));
#17954=CARTESIAN_POINT('',(-9.516475,1.78524650477582E-12,1.24542303242842));
#17955=CARTESIAN_POINT('Ctrl Pts',(-9.516475,1.50837236741359E-12,26.2954230324284));
#17956=CARTESIAN_POINT('Ctrl Pts',(-9.51647500000039,-0.26570662058248,
26.3079039656766));
#17957=CARTESIAN_POINT('Ctrl Pts',(-9.40727465387272,-0.529786878175832,
26.3203848989248));
#17958=CARTESIAN_POINT('Ctrl Pts',(-9.21961691907858,-0.717894780173845,
26.332865832173));
#17959=CARTESIAN_POINT('Ctrl Pts',(-9.03195918428444,-0.906002682171858,
26.3453467654212));
#17960=CARTESIAN_POINT('Ctrl Pts',(-8.76814132834493,-1.01583545019879,
26.3578276986694));
#17961=CARTESIAN_POINT('Ctrl Pts',(-8.50243547044616,-1.0164720823066,26.3703086319176));
#17962=CARTESIAN_POINT('Ctrl Pts',(-8.23672961254739,-1.0171087144144,26.3827895651658));
#17963=CARTESIAN_POINT('Ctrl Pts',(-7.9723884693343,-0.908541417083319,
26.395270498414));
#17964=CARTESIAN_POINT('Ctrl Pts',(-7.78383148002414,-0.721334926799326,
26.4077514316622));
#17965=CARTESIAN_POINT('Ctrl Pts',(-7.59527449071398,-0.534128436515333,
26.4202323649103));
#17966=CARTESIAN_POINT('Ctrl Pts',(-7.4848099313173,-0.27057449675675,26.4327132981585));
#17967=CARTESIAN_POINT('Ctrl Pts',(-7.48353667075686,-0.00487092690924407,
26.4451942314067));
#17968=CARTESIAN_POINT('Ctrl Pts',(-7.48226341019643,0.260832642938262,
26.4576751646549));
#17969=CARTESIAN_POINT('Ctrl Pts',(-7.59019703546702,0.525433154239586,
26.4701560979031));
#17970=CARTESIAN_POINT('Ctrl Pts',(-7.77695120652453,0.714438148392613,
26.4826370311513));
#17971=CARTESIAN_POINT('Ctrl Pts',(-7.96370537758204,0.903443142545639,
26.4951179643995));
#17972=CARTESIAN_POINT('Ctrl Pts',(-8.2269938881474,1.01453885915636,26.5075988976477));
#17973=CARTESIAN_POINT('Ctrl Pts',(-8.49269364459072,1.01644874085988,26.5200798308959));
#17974=CARTESIAN_POINT('Ctrl Pts',(-8.75839340103405,1.0183586225634,26.5325607641441));
#17975=CARTESIAN_POINT('Ctrl Pts',(-9.02325176140315,0.911059288979411,
26.5450416973923));
#17976=CARTESIAN_POINT('Ctrl Pts',(-9.21270367535784,0.724758509268037,
26.5575226306404));
#17977=CARTESIAN_POINT('Ctrl Pts',(-9.40215558931254,0.538457729556662,
26.5700035638886));
#17978=CARTESIAN_POINT('Ctrl Pts',(-9.51388182535822,0.275436159673054,
26.5824844971368));
#17979=CARTESIAN_POINT('Ctrl Pts',(-9.51642831724057,0.00974174196493498,
26.594965430385));
#17980=CARTESIAN_POINT('Ctrl Pts',(-9.51645943884196,0.00649459406753594,
26.5951179643995));
#17981=CARTESIAN_POINT('Ctrl Pts',(-9.51647499999999,0.00324729703481928,
26.595270498414));
#17982=CARTESIAN_POINT('Ctrl Pts',(-9.516475,1.64584862817766E-12,26.5954230324284));
#17983=CARTESIAN_POINT('Ctrl Pts',(-9.5152075092142,-0.000523630537313469,
26.3545769675714));
#17984=CARTESIAN_POINT('Ctrl Pts',(-9.51594088723012,-0.132523029843183,
26.3607600508578));
#17985=CARTESIAN_POINT('Ctrl Pts',(-9.43067022437642,-0.60331137049921,
26.3828504752957));
#17986=CARTESIAN_POINT('Ctrl Pts',(-8.71771879103822,-1.18276034286521,
26.4208482408854));
#17987=CARTESIAN_POINT('Ctrl Pts',(-7.80744356640935,-0.882063793301015,
26.4606165937644));
#17988=CARTESIAN_POINT('Ctrl Pts',(-7.47730934038002,-0.265911264380824,
26.4924312760676));
#17989=CARTESIAN_POINT('Ctrl Pts',(-7.4655089049693,0.433011689752842,26.5242459583709));
#17990=CARTESIAN_POINT('Ctrl Pts',(-8.11403107601491,1.13901338462003,26.5640143112499));
#17991=CARTESIAN_POINT('Ctrl Pts',(-9.21176260908216,0.946387668608936,
26.6101092045087));
#17992=CARTESIAN_POINT('Ctrl Pts',(-9.51556036565569,0.302366890868681,
26.6402967566159));
#17993=CARTESIAN_POINT('Ctrl Pts',(-9.51759585434001,-0.000580554954882254,
26.6545769675714));
#17994=CARTESIAN_POINT('Origin',(-8.5,0.,1.24542303242842));
#17995=CARTESIAN_POINT('',(-9.516475,1.48645593502261E-12,25.9954230324284));
#17996=CARTESIAN_POINT('',(-9.516475,1.51339974860218E-12,26.0545769675715));
#17997=CARTESIAN_POINT('',(-9.516475,1.78524650477582E-12,1.24542303242842));
#17998=CARTESIAN_POINT('Ctrl Pts',(-9.516475,1.48645593502261E-12,25.9954230324284));
#17999=CARTESIAN_POINT('Ctrl Pts',(-9.51647500000039,-0.265706620582424,
26.0079039656766));
#18000=CARTESIAN_POINT('Ctrl Pts',(-9.40727465387278,-0.5297868781757,26.0203848989248));
#18001=CARTESIAN_POINT('Ctrl Pts',(-9.21961691907873,-0.717894780173697,
26.032865832173));
#18002=CARTESIAN_POINT('Ctrl Pts',(-9.03195918428468,-0.906002682171694,
26.0453467654212));
#18003=CARTESIAN_POINT('Ctrl Pts',(-8.76814132834529,-1.01583545019867,
26.0578276986694));
#18004=CARTESIAN_POINT('Ctrl Pts',(-8.5024354704466,-1.01647208230659,26.0703086319176));
#18005=CARTESIAN_POINT('Ctrl Pts',(-8.2367296125479,-1.01710871441451,26.0827895651657));
#18006=CARTESIAN_POINT('Ctrl Pts',(-7.97238846933485,-0.908541417083613,
26.0952704984139));
#18007=CARTESIAN_POINT('Ctrl Pts',(-7.78383148002462,-0.721334926799799,
26.1077514316621));
#18008=CARTESIAN_POINT('Ctrl Pts',(-7.59527449071439,-0.534128436515985,
26.1202323649103));
#18009=CARTESIAN_POINT('Ctrl Pts',(-7.48480993131754,-0.270574496757575,
26.1327132981585));
#18010=CARTESIAN_POINT('Ctrl Pts',(-7.48353667075687,-0.00487092691014662,
26.1451942314067));
#18011=CARTESIAN_POINT('Ctrl Pts',(-7.4822634101962,0.260832642937281,26.1576751646549));
#18012=CARTESIAN_POINT('Ctrl Pts',(-7.59019703546649,0.525433154238627,
26.1701560979031));
#18013=CARTESIAN_POINT('Ctrl Pts',(-7.77695120652373,0.714438148391806,
26.1826370311512));
#18014=CARTESIAN_POINT('Ctrl Pts',(-7.96370537758098,0.903443142544986,
26.1951179643994));
#18015=CARTESIAN_POINT('Ctrl Pts',(-8.22699388814611,1.01453885915599,26.2075988976476));
#18016=CARTESIAN_POINT('Ctrl Pts',(-8.49269364458936,1.01644874085987,26.2200798308958));
#18017=CARTESIAN_POINT('Ctrl Pts',(-8.7583934010326,1.01835862256374,26.232560764144));
#18018=CARTESIAN_POINT('Ctrl Pts',(-9.02325176140177,0.911059288980179,
26.2450416973922));
#18019=CARTESIAN_POINT('Ctrl Pts',(-9.2127036753567,0.724758509269156,26.2575226306404));
#18020=CARTESIAN_POINT('Ctrl Pts',(-9.40215558931163,0.538457729558133,
26.2700035638886));
#18021=CARTESIAN_POINT('Ctrl Pts',(-9.51388182535773,0.275436159674799,
26.2824844971367));
#18022=CARTESIAN_POINT('Ctrl Pts',(-9.51642831724055,0.00974174196676194,
26.2949654303849));
#18023=CARTESIAN_POINT('Ctrl Pts',(-9.51645943884196,0.00649459406870815,
26.2951179643994));
#18024=CARTESIAN_POINT('Ctrl Pts',(-9.51647499999999,0.00324729703533653,
26.2952704984139));
#18025=CARTESIAN_POINT('Ctrl Pts',(-9.516475,1.50837236741359E-12,26.2954230324284));
#18026=CARTESIAN_POINT('Ctrl Pts',(-9.516475,1.62895957697526E-12,26.0545769675714));
#18027=CARTESIAN_POINT('Ctrl Pts',(-9.51647500000043,-0.265706620582359,
26.0670579008196));
#18028=CARTESIAN_POINT('Ctrl Pts',(-9.40727465387279,-0.529786878175724,
26.0795388340678));
#18029=CARTESIAN_POINT('Ctrl Pts',(-9.21961691907866,-0.71789478017376,
26.092019767316));
#18030=CARTESIAN_POINT('Ctrl Pts',(-9.03195918428454,-0.906002682171795,
26.1045007005642));
#18031=CARTESIAN_POINT('Ctrl Pts',(-8.76814132834505,-1.01583545019876,
26.1169816338124));
#18032=CARTESIAN_POINT('Ctrl Pts',(-8.50243547044628,-1.01647208230659,
26.1294625670606));
#18033=CARTESIAN_POINT('Ctrl Pts',(-8.23672961254751,-1.01710871441443,
26.1419435003088));
#18034=CARTESIAN_POINT('Ctrl Pts',(-7.97238846933441,-0.908541417083381,
26.154424433557));
#18035=CARTESIAN_POINT('Ctrl Pts',(-7.78383148002423,-0.721334926799411,
26.1669053668052));
#18036=CARTESIAN_POINT('Ctrl Pts',(-7.59527449071404,-0.534128436515441,
26.1793863000534));
#18037=CARTESIAN_POINT('Ctrl Pts',(-7.48480993131733,-0.270574496756871,
26.1918672333016));
#18038=CARTESIAN_POINT('Ctrl Pts',(-7.48353667075686,-0.00487092690936466,
26.2043481665497));
#18039=CARTESIAN_POINT('Ctrl Pts',(-7.4822634101964,0.260832642938141,26.2168290997979));
#18040=CARTESIAN_POINT('Ctrl Pts',(-7.59019703546696,0.525433154239479,
26.2293100330461));
#18041=CARTESIAN_POINT('Ctrl Pts',(-7.77695120652444,0.714438148392527,
26.2417909662943));
#18042=CARTESIAN_POINT('Ctrl Pts',(-7.96370537758193,0.903443142545575,
26.2542718995425));
#18043=CARTESIAN_POINT('Ctrl Pts',(-8.22699388814728,1.01453885915633,26.2667528327907));
#18044=CARTESIAN_POINT('Ctrl Pts',(-8.4926936445906,1.01644874085988,26.2792337660389));
#18045=CARTESIAN_POINT('Ctrl Pts',(-8.75839340103393,1.01835862256343,26.2917146992871));
#18046=CARTESIAN_POINT('Ctrl Pts',(-9.02325176140303,0.911059288979473,
26.3041956325353));
#18047=CARTESIAN_POINT('Ctrl Pts',(-9.21270367535775,0.724758509268121,
26.3166765657835));
#18048=CARTESIAN_POINT('Ctrl Pts',(-9.40215558931247,0.538457729556769,
26.3291574990317));
#18049=CARTESIAN_POINT('Ctrl Pts',(-9.51388182535819,0.275436159673174,
26.3416384322799));
#18050=CARTESIAN_POINT('Ctrl Pts',(-9.51642831724056,0.00974174196505557,
26.354119365528));
#18051=CARTESIAN_POINT('Ctrl Pts',(-9.51645943884196,0.00649459406757949,
26.3542718995425));
#18052=CARTESIAN_POINT('Ctrl Pts',(-9.51647499999999,0.00324729703478578,
26.354424433557));
#18053=CARTESIAN_POINT('Ctrl Pts',(-9.516475,1.53531618099316E-12,26.3545769675715));
#18054=CARTESIAN_POINT('Origin',(-8.5,0.,1.24542303242842));
#18055=CARTESIAN_POINT('',(-9.516475,1.46453950263162E-12,25.6954230324284));
#18056=CARTESIAN_POINT('',(-9.516475,1.49148331621119E-12,25.7545769675715));
#18057=CARTESIAN_POINT('',(-9.516475,1.78524650477582E-12,1.24542303242842));
#18058=CARTESIAN_POINT('Ctrl Pts',(-9.516475,1.46453950263162E-12,25.6954230324284));
#18059=CARTESIAN_POINT('Ctrl Pts',(-9.51647500000038,-0.265706620582523,
25.7079039656766));
#18060=CARTESIAN_POINT('Ctrl Pts',(-9.4072746538727,-0.529786878175871,
25.7203848989248));
#18061=CARTESIAN_POINT('Ctrl Pts',(-9.21961691907855,-0.717894780173876,
25.732865832173));
#18062=CARTESIAN_POINT('Ctrl Pts',(-9.0319591842844,-0.906002682171881,
25.7453467654212));
#18063=CARTESIAN_POINT('Ctrl Pts',(-8.76814132834489,-1.0158354501988,25.7578276986694));
#18064=CARTESIAN_POINT('Ctrl Pts',(-8.50243547044612,-1.0164720823066,25.7703086319176));
#18065=CARTESIAN_POINT('Ctrl Pts',(-8.23672961254734,-1.01710871441439,
25.7827895651658));
#18066=CARTESIAN_POINT('Ctrl Pts',(-7.97238846933427,-0.908541417083296,
25.795270498414));
#18067=CARTESIAN_POINT('Ctrl Pts',(-7.78383148002411,-0.721334926799295,
25.8077514316622));
#18068=CARTESIAN_POINT('Ctrl Pts',(-7.59527449071396,-0.534128436515294,
25.8202323649103));
#18069=CARTESIAN_POINT('Ctrl Pts',(-7.48480993131728,-0.270574496756706,
25.8327132981585));
#18070=CARTESIAN_POINT('Ctrl Pts',(-7.48353667075686,-0.00487092690920024,
25.8451942314067));
#18071=CARTESIAN_POINT('Ctrl Pts',(-7.48226341019644,0.260832642938306,
25.8576751646549));
#18072=CARTESIAN_POINT('Ctrl Pts',(-7.59019703546704,0.525433154239626,
25.8701560979031));
#18073=CARTESIAN_POINT('Ctrl Pts',(-7.77695120652456,0.714438148392644,
25.8826370311513));
#18074=CARTESIAN_POINT('Ctrl Pts',(-7.96370537758208,0.903443142545662,
25.8951179643995));
#18075=CARTESIAN_POINT('Ctrl Pts',(-8.22699388814744,1.01453885915637,25.9075988976477));
#18076=CARTESIAN_POINT('Ctrl Pts',(-8.49269364459077,1.01644874085988,25.9200798308959));
#18077=CARTESIAN_POINT('Ctrl Pts',(-8.75839340103409,1.01835862256339,25.9325607641441));
#18078=CARTESIAN_POINT('Ctrl Pts',(-9.02325176140318,0.911059288979388,
25.9450416973923));
#18079=CARTESIAN_POINT('Ctrl Pts',(-9.21270367535787,0.724758509268006,
25.9575226306405));
#18080=CARTESIAN_POINT('Ctrl Pts',(-9.40215558931256,0.538457729556623,
25.9700035638886));
#18081=CARTESIAN_POINT('Ctrl Pts',(-9.51388182535823,0.27543615967301,25.9824844971368));
#18082=CARTESIAN_POINT('Ctrl Pts',(-9.51642831724057,0.00974174196489115,
25.994965430385));
#18083=CARTESIAN_POINT('Ctrl Pts',(-9.51645943884196,0.00649459406745359,
25.9951179643995));
#18084=CARTESIAN_POINT('Ctrl Pts',(-9.51647499999999,0.00324729703469832,
25.995270498414));
#18085=CARTESIAN_POINT('Ctrl Pts',(-9.516475,1.48645593502261E-12,25.9954230324284));
#18086=CARTESIAN_POINT('Ctrl Pts',(-9.516475,1.49148331621119E-12,25.7545769675715));
#18087=CARTESIAN_POINT('Ctrl Pts',(-9.51647500000039,-0.265706620582535,
25.7670579008196));
#18088=CARTESIAN_POINT('Ctrl Pts',(-9.40727465387268,-0.529786878175923,
25.7795388340678));
#18089=CARTESIAN_POINT('Ctrl Pts',(-9.21961691907848,-0.717894780173939,
25.792019767316));
#18090=CARTESIAN_POINT('Ctrl Pts',(-9.03195918428429,-0.906002682171955,
25.8045007005642));
#18091=CARTESIAN_POINT('Ctrl Pts',(-8.76814132834472,-1.01583545019886,
25.8169816338124));
#18092=CARTESIAN_POINT('Ctrl Pts',(-8.50243547044591,-1.0164720823066,25.8294625670606));
#18093=CARTESIAN_POINT('Ctrl Pts',(-8.2367296125471,-1.01710871441434,25.8419435003088));
#18094=CARTESIAN_POINT('Ctrl Pts',(-7.97238846933401,-0.908541417083157,
25.854424433557));
#18095=CARTESIAN_POINT('Ctrl Pts',(-7.78383148002388,-0.72133492679907,
25.8669053668052));
#18096=CARTESIAN_POINT('Ctrl Pts',(-7.59527449071376,-0.534128436514983,
25.8793863000534));
#18097=CARTESIAN_POINT('Ctrl Pts',(-7.48480993131717,-0.27057449675631,
25.8918672333016));
#18098=CARTESIAN_POINT('Ctrl Pts',(-7.48353667075686,-0.00487092690876495,
25.9043481665498));
#18099=CARTESIAN_POINT('Ctrl Pts',(-7.48226341019655,0.26083264293878,25.916829099798));
#18100=CARTESIAN_POINT('Ctrl Pts',(-7.5901970354673,0.525433154240091,25.9293100330462));
#18101=CARTESIAN_POINT('Ctrl Pts',(-7.77695120652495,0.714438148393036,
25.9417909662944));
#18102=CARTESIAN_POINT('Ctrl Pts',(-7.96370537758259,0.90344314254598,25.9542718995425));
#18103=CARTESIAN_POINT('Ctrl Pts',(-8.22699388814807,1.01453885915655,25.9667528327907));
#18104=CARTESIAN_POINT('Ctrl Pts',(-8.49269364459143,1.01644874085988,25.9792337660389));
#18105=CARTESIAN_POINT('Ctrl Pts',(-8.7583934010348,1.01835862256322,25.9917146992871));
#18106=CARTESIAN_POINT('Ctrl Pts',(-9.02325176140386,0.911059288979013,
26.0041956325353));
#18107=CARTESIAN_POINT('Ctrl Pts',(-9.21270367535843,0.724758509267457,
26.0166765657835));
#18108=CARTESIAN_POINT('Ctrl Pts',(-9.402155589313,0.538457729555902,26.0291574990317));
#18109=CARTESIAN_POINT('Ctrl Pts',(-9.51388182535848,0.275436159672154,
26.0416384322799));
#18110=CARTESIAN_POINT('Ctrl Pts',(-9.51642831724057,0.00974174196399366,
26.0541193655281));
#18111=CARTESIAN_POINT('Ctrl Pts',(-9.51645943884197,0.00649459406690274,
26.0542718995425));
#18112=CARTESIAN_POINT('Ctrl Pts',(-9.51647499999999,0.00324729703449424,
26.054424433557));
#18113=CARTESIAN_POINT('Ctrl Pts',(-9.516475,1.62895957697526E-12,26.0545769675714));
#18114=CARTESIAN_POINT('Origin',(-8.5,0.,1.24542303242842));
#18115=CARTESIAN_POINT('',(-9.51609769462188,7.92988697302073E-5,25.3954230324284));
#18116=CARTESIAN_POINT('',(-9.516475,1.46956688382021E-12,25.4545769675715));
#18117=CARTESIAN_POINT('',(-9.516475,1.78524650477582E-12,1.24542303242842));
#18118=CARTESIAN_POINT('Ctrl Pts',(-9.516475,1.50040298442718E-12,25.3954230324284));
#18119=CARTESIAN_POINT('Ctrl Pts',(-9.51647500000039,-0.265706620582449,
25.4079039656766));
#18120=CARTESIAN_POINT('Ctrl Pts',(-9.40727465387275,-0.529786878175763,
25.4203848989248));
#18121=CARTESIAN_POINT('Ctrl Pts',(-9.21961691907866,-0.717894780173769,
25.432865832173));
#18122=CARTESIAN_POINT('Ctrl Pts',(-9.03195918428456,-0.906002682171775,
25.4453467654212));
#18123=CARTESIAN_POINT('Ctrl Pts',(-8.76814132834512,-1.01583545019873,
25.4578276986694));
#18124=CARTESIAN_POINT('Ctrl Pts',(-8.50243547044638,-1.01647208230659,
25.4703086319176));
#18125=CARTESIAN_POINT('Ctrl Pts',(-8.23672961254765,-1.01710871441446,
25.4827895651658));
#18126=CARTESIAN_POINT('Ctrl Pts',(-7.97238846933458,-0.908541417083467,
25.4952704984139));
#18127=CARTESIAN_POINT('Ctrl Pts',(-7.78383148002438,-0.721334926799565,
25.5077514316621));
#18128=CARTESIAN_POINT('Ctrl Pts',(-7.59527449071418,-0.534128436515662,
25.5202323649103));
#18129=CARTESIAN_POINT('Ctrl Pts',(-7.48480993131742,-0.270574496757165,
25.5327132981585));
#18130=CARTESIAN_POINT('Ctrl Pts',(-7.48353667075686,-0.00487092690969834,
25.5451942314067));
#18131=CARTESIAN_POINT('Ctrl Pts',(-7.48226341019631,0.260832642937769,
25.5576751646549));
#18132=CARTESIAN_POINT('Ctrl Pts',(-7.59019703546675,0.525433154239104,
25.5701560979031));
#18133=CARTESIAN_POINT('Ctrl Pts',(-7.77695120652413,0.714438148392207,
25.5826370311513));
#18134=CARTESIAN_POINT('Ctrl Pts',(-7.96370537758151,0.903443142545311,
25.5951179643995));
#18135=CARTESIAN_POINT('Ctrl Pts',(-8.22699388814675,1.01453885915618,25.6075988976477));
#18136=CARTESIAN_POINT('Ctrl Pts',(-8.49269364459004,1.01644874085987,25.6200798308958));
#18137=CARTESIAN_POINT('Ctrl Pts',(-8.75839340103332,1.01835862256357,25.632560764144));
#18138=CARTESIAN_POINT('Ctrl Pts',(-9.02325176140245,0.911059288979796,
25.6450416973922));
#18139=CARTESIAN_POINT('Ctrl Pts',(-9.21270367535727,0.724758509268598,
25.6575226306404));
#18140=CARTESIAN_POINT('Ctrl Pts',(-9.40215558931207,0.538457729557414,
25.6700035638886));
#18141=CARTESIAN_POINT('Ctrl Pts',(-9.51388182535796,0.275436159673968,
25.6824844971368));
#18142=CARTESIAN_POINT('Ctrl Pts',(-9.51642831724056,0.00974174196590923,
25.694965430385));
#18143=CARTESIAN_POINT('Ctrl Pts',(-9.51645943884196,0.00649459406812504,
25.6951179643995));
#18144=CARTESIAN_POINT('Ctrl Pts',(-9.51647499999999,0.00324729703502315,
25.6952704984139));
#18145=CARTESIAN_POINT('Ctrl Pts',(-9.516475,1.46453950263162E-12,25.6954230324284));
#18146=CARTESIAN_POINT('Ctrl Pts',(-9.516475,1.46956688382021E-12,25.4545769675715));
#18147=CARTESIAN_POINT('Ctrl Pts',(-9.51647500000038,-0.265706620582518,
25.4670579008196));
#18148=CARTESIAN_POINT('Ctrl Pts',(-9.4072746538727,-0.529786878175867,
25.4795388340678));
#18149=CARTESIAN_POINT('Ctrl Pts',(-9.21961691907855,-0.717894780173873,
25.492019767316));
#18150=CARTESIAN_POINT('Ctrl Pts',(-9.0319591842844,-0.906002682171879,
25.5045007005642));
#18151=CARTESIAN_POINT('Ctrl Pts',(-8.76814132834489,-1.0158354501988,25.5169816338124));
#18152=CARTESIAN_POINT('Ctrl Pts',(-8.50243547044612,-1.0164720823066,25.5294625670606));
#18153=CARTESIAN_POINT('Ctrl Pts',(-8.23672961254735,-1.01710871441439,
25.5419435003088));
#18154=CARTESIAN_POINT('Ctrl Pts',(-7.97238846933427,-0.908541417083299,
25.554424433557));
#18155=CARTESIAN_POINT('Ctrl Pts',(-7.78383148002411,-0.721334926799299,
25.5669053668052));
#18156=CARTESIAN_POINT('Ctrl Pts',(-7.59527449071396,-0.534128436515299,
25.5793863000534));
#18157=CARTESIAN_POINT('Ctrl Pts',(-7.48480993131728,-0.270574496756711,
25.5918672333016));
#18158=CARTESIAN_POINT('Ctrl Pts',(-7.48353667075686,-0.00487092690920527,
25.6043481665498));
#18159=CARTESIAN_POINT('Ctrl Pts',(-7.48226341019644,0.260832642938301,
25.6168290997979));
#18160=CARTESIAN_POINT('Ctrl Pts',(-7.59019703546704,0.525433154239621,
25.6293100330461));
#18161=CARTESIAN_POINT('Ctrl Pts',(-7.77695120652456,0.71443814839264,25.6417909662943));
#18162=CARTESIAN_POINT('Ctrl Pts',(-7.96370537758207,0.903443142545659,
25.6542718995425));
#18163=CARTESIAN_POINT('Ctrl Pts',(-8.22699388814744,1.01453885915637,25.6667528327907));
#18164=CARTESIAN_POINT('Ctrl Pts',(-8.49269364459076,1.01644874085988,25.6792337660389));
#18165=CARTESIAN_POINT('Ctrl Pts',(-8.75839340103408,1.01835862256339,25.6917146992871));
#18166=CARTESIAN_POINT('Ctrl Pts',(-9.02325176140318,0.911059288979391,
25.7041956325353));
#18167=CARTESIAN_POINT('Ctrl Pts',(-9.21270367535787,0.724758509268009,
25.7166765657835));
#18168=CARTESIAN_POINT('Ctrl Pts',(-9.40215558931255,0.538457729556628,
25.7291574990317));
#18169=CARTESIAN_POINT('Ctrl Pts',(-9.51388182535823,0.275436159673015,
25.7416384322799));
#18170=CARTESIAN_POINT('Ctrl Pts',(-9.51642831724057,0.00974174196489618,
25.754119365528));
#18171=CARTESIAN_POINT('Ctrl Pts',(-9.51645943884196,0.00649459406745862,
25.7542718995425));
#18172=CARTESIAN_POINT('Ctrl Pts',(-9.51647499999999,0.00324729703470335,
25.754424433557));
#18173=CARTESIAN_POINT('Ctrl Pts',(-9.516475,1.49148331621119E-12,25.7545769675715));
#18174=CARTESIAN_POINT('Origin',(-8.5,0.,1.24542303242842));
#18175=CARTESIAN_POINT('',(-9.51649580167683,2.1540054757358E-5,25.0954230324284));
#18176=CARTESIAN_POINT('',(-9.516475,1.44765045142922E-12,25.1545769675715));
#18177=CARTESIAN_POINT('',(-9.516475,1.78524650477582E-12,1.24542303242842));
#18178=CARTESIAN_POINT('Ctrl Pts',(-9.51721349225105,0.000764705779924109,
25.0954230324284));
#18179=CARTESIAN_POINT('Ctrl Pts',(-9.51484927656888,-0.286952017602154,
25.1089718447615));
#18180=CARTESIAN_POINT('Ctrl Pts',(-9.23722805908837,-0.916544261020621,
25.1384279982462));
#18181=CARTESIAN_POINT('Ctrl Pts',(-8.16676365035883,-1.15554187977053,
25.1837914928825));
#18182=CARTESIAN_POINT('Ctrl Pts',(-7.48649317569277,-0.480077979335733,
25.2235598457615));
#18183=CARTESIAN_POINT('Ctrl Pts',(-7.4661733610654,0.218649185746783,25.2553745280648));
#18184=CARTESIAN_POINT('Ctrl Pts',(-7.76765364280032,0.849317232991748,
25.287189210368));
#18185=CARTESIAN_POINT('Ctrl Pts',(-8.6631541573295,1.19151341644644,25.3269575632471));
#18186=CARTESIAN_POINT('Ctrl Pts',(-9.41619328487241,0.634917146514559,
25.3656867274592));
#18187=CARTESIAN_POINT('Ctrl Pts',(-9.51549925971945,0.148008510868454,
25.3885085505196));
#18188=CARTESIAN_POINT('Ctrl Pts',(-9.51497361421595,0.000315548626982715,
25.3954230324284));
#18189=CARTESIAN_POINT('Ctrl Pts',(-9.516475,1.50543036561576E-12,25.1545769675715));
#18190=CARTESIAN_POINT('Ctrl Pts',(-9.51647500000039,-0.265706620582463,
25.1670579008196));
#18191=CARTESIAN_POINT('Ctrl Pts',(-9.40727465387274,-0.529786878175797,
25.1795388340678));
#18192=CARTESIAN_POINT('Ctrl Pts',(-9.21961691907862,-0.717894780173806,
25.192019767316));
#18193=CARTESIAN_POINT('Ctrl Pts',(-9.0319591842845,-0.906002682171816,
25.2045007005642));
#18194=CARTESIAN_POINT('Ctrl Pts',(-8.76814132834503,-1.01583545019876,
25.2169816338124));
#18195=CARTESIAN_POINT('Ctrl Pts',(-8.50243547044627,-1.01647208230659,
25.2294625670606));
#18196=CARTESIAN_POINT('Ctrl Pts',(-8.23672961254752,-1.01710871441443,
25.2419435003088));
#18197=CARTESIAN_POINT('Ctrl Pts',(-7.97238846933444,-0.908541417083394,
25.254424433557));
#18198=CARTESIAN_POINT('Ctrl Pts',(-7.78383148002426,-0.721334926799446,
25.2669053668052));
#18199=CARTESIAN_POINT('Ctrl Pts',(-7.59527449071408,-0.534128436515499,
25.2793863000534));
#18200=CARTESIAN_POINT('Ctrl Pts',(-7.48480993131736,-0.270574496756959,
25.2918672333015));
#18201=CARTESIAN_POINT('Ctrl Pts',(-7.48353667075686,-0.00487092690947225,
25.3043481665497));
#18202=CARTESIAN_POINT('Ctrl Pts',(-7.48226341019637,0.260832642938014,
25.3168290997979));
#18203=CARTESIAN_POINT('Ctrl Pts',(-7.59019703546688,0.525433154239344,
25.3293100330461));
#18204=CARTESIAN_POINT('Ctrl Pts',(-7.77695120652433,0.714438148392409,
25.3417909662943));
#18205=CARTESIAN_POINT('Ctrl Pts',(-7.96370537758177,0.903443142545474,
25.3542718995425));
#18206=CARTESIAN_POINT('Ctrl Pts',(-8.22699388814707,1.01453885915627,25.3667528327907));
#18207=CARTESIAN_POINT('Ctrl Pts',(-8.49269364459038,1.01644874085988,25.3792337660389));
#18208=CARTESIAN_POINT('Ctrl Pts',(-8.75839340103368,1.01835862256349,25.3917146992871));
#18209=CARTESIAN_POINT('Ctrl Pts',(-9.0232517614028,0.911059288979604,25.4041956325353));
#18210=CARTESIAN_POINT('Ctrl Pts',(-9.21270367535755,0.724758509268318,
25.4166765657835));
#18211=CARTESIAN_POINT('Ctrl Pts',(-9.40215558931231,0.538457729557032,
25.4291574990316));
#18212=CARTESIAN_POINT('Ctrl Pts',(-9.5138818253581,0.275436159673493,25.4416384322798));
#18213=CARTESIAN_POINT('Ctrl Pts',(-9.51642831724056,0.00974174196539426,
25.454119365528));
#18214=CARTESIAN_POINT('Ctrl Pts',(-9.51645943884196,0.00649459406778338,
25.4542718995425));
#18215=CARTESIAN_POINT('Ctrl Pts',(-9.51647499999999,0.00324729703485473,
25.454424433557));
#18216=CARTESIAN_POINT('Ctrl Pts',(-9.516475,1.46956688382021E-12,25.4545769675715));
#18217=CARTESIAN_POINT('Origin',(-8.5,0.,1.24542303242842));
#18218=CARTESIAN_POINT('',(-9.516475,1.39879020545867E-12,24.7954230324284));
#18219=CARTESIAN_POINT('',(-9.516475,1.42573401903824E-12,24.8545769675715));
#18220=CARTESIAN_POINT('',(-9.516475,1.78524650477582E-12,1.24542303242842));
#18221=CARTESIAN_POINT('Ctrl Pts',(-9.516475,1.45657011964521E-12,24.7954230324284));
#18222=CARTESIAN_POINT('Ctrl Pts',(-9.51647500000038,-0.265706620582531,
24.8079039656766));
#18223=CARTESIAN_POINT('Ctrl Pts',(-9.4072746538727,-0.529786878175878,
24.8203848989248));
#18224=CARTESIAN_POINT('Ctrl Pts',(-9.21961691907854,-0.717894780173882,
24.832865832173));
#18225=CARTESIAN_POINT('Ctrl Pts',(-9.03195918428439,-0.906002682171885,
24.8453467654212));
#18226=CARTESIAN_POINT('Ctrl Pts',(-8.76814132834488,-1.0158354501988,24.8578276986694));
#18227=CARTESIAN_POINT('Ctrl Pts',(-8.50243547044611,-1.0164720823066,24.8703086319176));
#18228=CARTESIAN_POINT('Ctrl Pts',(-8.23672961254733,-1.01710871441439,
24.8827895651658));
#18229=CARTESIAN_POINT('Ctrl Pts',(-7.97238846933426,-0.908541417083292,
24.895270498414));
#18230=CARTESIAN_POINT('Ctrl Pts',(-7.78383148002411,-0.72133492679929,
24.9077514316622));
#18231=CARTESIAN_POINT('Ctrl Pts',(-7.59527449071395,-0.534128436515287,
24.9202323649103));
#18232=CARTESIAN_POINT('Ctrl Pts',(-7.48480993131728,-0.270574496756698,
24.9327132981585));
#18233=CARTESIAN_POINT('Ctrl Pts',(-7.48353667075686,-0.00487092690919227,
24.9451942314067));
#18234=CARTESIAN_POINT('Ctrl Pts',(-7.48226341019644,0.260832642938314,
24.9576751646549));
#18235=CARTESIAN_POINT('Ctrl Pts',(-7.59019703546705,0.525433154239633,
24.9701560979031));
#18236=CARTESIAN_POINT('Ctrl Pts',(-7.77695120652456,0.71443814839265,24.9826370311513));
#18237=CARTESIAN_POINT('Ctrl Pts',(-7.96370537758208,0.903443142545666,
24.9951179643995));
#18238=CARTESIAN_POINT('Ctrl Pts',(-8.22699388814745,1.01453885915637,25.0075988976477));
#18239=CARTESIAN_POINT('Ctrl Pts',(-8.49269364459077,1.01644874085988,25.0200798308959));
#18240=CARTESIAN_POINT('Ctrl Pts',(-8.7583934010341,1.01835862256338,25.0325607641441));
#18241=CARTESIAN_POINT('Ctrl Pts',(-9.02325176140319,0.911059288979384,
25.0450416973923));
#18242=CARTESIAN_POINT('Ctrl Pts',(-9.21270367535788,0.724758509268,25.0575226306405));
#18243=CARTESIAN_POINT('Ctrl Pts',(-9.40215558931256,0.538457729556616,
25.0700035638886));
#18244=CARTESIAN_POINT('Ctrl Pts',(-9.51388182535824,0.275436159673003,
25.0824844971368));
#18245=CARTESIAN_POINT('Ctrl Pts',(-9.51642831724057,0.00974174196488318,
25.094965430385));
#18246=CARTESIAN_POINT('Ctrl Pts',(-9.51645943884196,0.00649459406742636,
25.0951179643995));
#18247=CARTESIAN_POINT('Ctrl Pts',(-9.51647499999999,0.00324729703465179,
25.095270498414));
#18248=CARTESIAN_POINT('Ctrl Pts',(-9.516475,1.42070663784965E-12,25.0954230324284));
#18249=CARTESIAN_POINT('Ctrl Pts',(-9.516475,1.48351393322478E-12,24.8545769675715));
#18250=CARTESIAN_POINT('Ctrl Pts',(-9.51647500000039,-0.265706620582466,
24.8670579008196));
#18251=CARTESIAN_POINT('Ctrl Pts',(-9.40727465387274,-0.529786878175778,
24.8795388340678));
#18252=CARTESIAN_POINT('Ctrl Pts',(-9.21961691907864,-0.717894780173781,
24.892019767316));
#18253=CARTESIAN_POINT('Ctrl Pts',(-9.03195918428454,-0.906002682171783,
24.9045007005642));
#18254=CARTESIAN_POINT('Ctrl Pts',(-8.7681413283451,-1.01583545019874,24.9169816338124));
#18255=CARTESIAN_POINT('Ctrl Pts',(-8.50243547044636,-1.01647208230659,
24.9294625670606));
#18256=CARTESIAN_POINT('Ctrl Pts',(-8.23672961254763,-1.01710871441445,
24.9419435003088));
#18257=CARTESIAN_POINT('Ctrl Pts',(-7.97238846933456,-0.908541417083459,
24.954424433557));
#18258=CARTESIAN_POINT('Ctrl Pts',(-7.78383148002437,-0.721334926799553,
24.9669053668052));
#18259=CARTESIAN_POINT('Ctrl Pts',(-7.59527449071418,-0.534128436515647,
24.9793863000533));
#18260=CARTESIAN_POINT('Ctrl Pts',(-7.48480993131741,-0.270574496757148,
24.9918672333015));
#18261=CARTESIAN_POINT('Ctrl Pts',(-7.48353667075686,-0.00487092690968145,
25.0043481665497));
#18262=CARTESIAN_POINT('Ctrl Pts',(-7.48226341019632,0.260832642937786,
25.0168290997979));
#18263=CARTESIAN_POINT('Ctrl Pts',(-7.59019703546676,0.525433154239119,
25.0293100330461));
#18264=CARTESIAN_POINT('Ctrl Pts',(-7.77695120652414,0.714438148392219,
25.0417909662943));
#18265=CARTESIAN_POINT('Ctrl Pts',(-7.96370537758152,0.90344314254532,25.0542718995425));
#18266=CARTESIAN_POINT('Ctrl Pts',(-8.22699388814677,1.01453885915618,25.0667528327907));
#18267=CARTESIAN_POINT('Ctrl Pts',(-8.49269364459005,1.01644874085987,25.0792337660389));
#18268=CARTESIAN_POINT('Ctrl Pts',(-8.75839340103334,1.01835862256357,25.0917146992871));
#18269=CARTESIAN_POINT('Ctrl Pts',(-9.02325176140247,0.911059288979787,
25.1041956325352));
#18270=CARTESIAN_POINT('Ctrl Pts',(-9.21270367535728,0.724758509268586,
25.1166765657834));
#18271=CARTESIAN_POINT('Ctrl Pts',(-9.40215558931209,0.538457729557385,
25.1291574990316));
#18272=CARTESIAN_POINT('Ctrl Pts',(-9.51388182535798,0.275436159673913,
25.1416384322798));
#18273=CARTESIAN_POINT('Ctrl Pts',(-9.51642831724056,0.00974174196583456,
25.154119365528));
#18274=CARTESIAN_POINT('Ctrl Pts',(-9.51645943884196,0.00649459406808889,
25.1542718995425));
#18275=CARTESIAN_POINT('Ctrl Pts',(-9.51647499999999,0.00324729703502544,
25.154424433557));
#18276=CARTESIAN_POINT('Ctrl Pts',(-9.516475,1.50543036561576E-12,25.1545769675715));
#18277=CARTESIAN_POINT('Origin',(-8.5,0.,1.24542303242842));
#18278=CARTESIAN_POINT('',(-9.516475,1.37687377306768E-12,24.4954230324284));
#18279=CARTESIAN_POINT('',(-9.516475,1.40381758664725E-12,24.5545769675715));
#18280=CARTESIAN_POINT('',(-9.516475,1.78524650477582E-12,1.24542303242842));
#18281=CARTESIAN_POINT('Ctrl Pts',(-9.516475,1.31909385888114E-12,24.4954230324284));
#18282=CARTESIAN_POINT('Ctrl Pts',(-9.51647500000034,-0.26570662058263,
24.5079039656766));
#18283=CARTESIAN_POINT('Ctrl Pts',(-9.40727465387266,-0.529786878175925,
24.5203848989248));
#18284=CARTESIAN_POINT('Ctrl Pts',(-9.21961691907853,-0.717894780173897,
24.532865832173));
#18285=CARTESIAN_POINT('Ctrl Pts',(-9.0319591842844,-0.90600268217187,24.5453467654212));
#18286=CARTESIAN_POINT('Ctrl Pts',(-8.76814132834494,-1.01583545019878,
24.5578276986694));
#18287=CARTESIAN_POINT('Ctrl Pts',(-8.5024354704462,-1.0164720823066,24.5703086319176));
#18288=CARTESIAN_POINT('Ctrl Pts',(-8.23672961254747,-1.01710871441441,
24.5827895651658));
#18289=CARTESIAN_POINT('Ctrl Pts',(-7.97238846933442,-0.908541417083373,
24.595270498414));
#18290=CARTESIAN_POINT('Ctrl Pts',(-7.78383148002425,-0.721334926799437,
24.6077514316621));
#18291=CARTESIAN_POINT('Ctrl Pts',(-7.59527449071409,-0.534128436515501,
24.6202323649103));
#18292=CARTESIAN_POINT('Ctrl Pts',(-7.48480993131737,-0.270574496756984,
24.6327132981585));
#18293=CARTESIAN_POINT('Ctrl Pts',(-7.48353667075686,-0.00487092690951703,
24.6451942314067));
#18294=CARTESIAN_POINT('Ctrl Pts',(-7.48226341019636,0.26083264293795,24.6576751646549));
#18295=CARTESIAN_POINT('Ctrl Pts',(-7.59019703546684,0.525433154239266,
24.6701560979031));
#18296=CARTESIAN_POINT('Ctrl Pts',(-7.77695120652426,0.714438148392336,
24.6826370311513));
#18297=CARTESIAN_POINT('Ctrl Pts',(-7.96370537758167,0.903443142545406,
24.6951179643995));
#18298=CARTESIAN_POINT('Ctrl Pts',(-8.22699388814693,1.01453885915622,24.7075988976477));
#18299=CARTESIAN_POINT('Ctrl Pts',(-8.49269364459022,1.01644874085988,24.7200798308959));
#18300=CARTESIAN_POINT('Ctrl Pts',(-8.7583934010335,1.01835862256353,24.732560764144));
#18301=CARTESIAN_POINT('Ctrl Pts',(-9.02325176140262,0.911059288979703,
24.7450416973922));
#18302=CARTESIAN_POINT('Ctrl Pts',(-9.2127036753574,0.724758509268471,24.7575226306404));
#18303=CARTESIAN_POINT('Ctrl Pts',(-9.40215558931218,0.538457729557239,
24.7700035638886));
#18304=CARTESIAN_POINT('Ctrl Pts',(-9.51388182535803,0.275436159673749,
24.7824844971368));
#18305=CARTESIAN_POINT('Ctrl Pts',(-9.51642831724056,0.00974174196567015,
24.794965430385));
#18306=CARTESIAN_POINT('Ctrl Pts',(-9.51645943884196,0.00649459406796299,
24.7951179643995));
#18307=CARTESIAN_POINT('Ctrl Pts',(-9.51647499999999,0.00324729703493815,
24.7952704984139));
#18308=CARTESIAN_POINT('Ctrl Pts',(-9.516475,1.45657011964521E-12,24.7954230324284));
#18309=CARTESIAN_POINT('Ctrl Pts',(-9.516475,1.40381758664725E-12,24.5545769675715));
#18310=CARTESIAN_POINT('Ctrl Pts',(-9.51647500000037,-0.265706620582546,
24.5670579008196));
#18311=CARTESIAN_POINT('Ctrl Pts',(-9.4072746538727,-0.529786878175849,
24.5795388340678));
#18312=CARTESIAN_POINT('Ctrl Pts',(-9.21961691907859,-0.717894780173837,
24.592019767316));
#18313=CARTESIAN_POINT('Ctrl Pts',(-9.03195918428447,-0.906002682171825,
24.6045007005642));
#18314=CARTESIAN_POINT('Ctrl Pts',(-8.76814132834502,-1.01583545019876,
24.6169816338124));
#18315=CARTESIAN_POINT('Ctrl Pts',(-8.50243547044629,-1.01647208230659,
24.6294625670606));
#18316=CARTESIAN_POINT('Ctrl Pts',(-8.23672961254755,-1.01710871441443,
24.6419435003088));
#18317=CARTESIAN_POINT('Ctrl Pts',(-7.97238846933449,-0.908541417083417,
24.654424433557));
#18318=CARTESIAN_POINT('Ctrl Pts',(-7.78383148002431,-0.721334926799497,
24.6669053668052));
#18319=CARTESIAN_POINT('Ctrl Pts',(-7.59527449071413,-0.534128436515576,
24.6793863000534));
#18320=CARTESIAN_POINT('Ctrl Pts',(-7.48480993131739,-0.270574496757069,
24.6918672333015));
#18321=CARTESIAN_POINT('Ctrl Pts',(-7.48353667075686,-0.00487092690960175,
24.7043481665497));
#18322=CARTESIAN_POINT('Ctrl Pts',(-7.48226341019634,0.260832642937865,
24.7168290997979));
#18323=CARTESIAN_POINT('Ctrl Pts',(-7.5901970354668,0.52543315423919,24.7293100330461));
#18324=CARTESIAN_POINT('Ctrl Pts',(-7.7769512065242,0.714438148392276,24.7417909662943));
#18325=CARTESIAN_POINT('Ctrl Pts',(-7.96370537758159,0.903443142545362,
24.7542718995425));
#18326=CARTESIAN_POINT('Ctrl Pts',(-8.22699388814685,1.0145388591562,24.7667528327907));
#18327=CARTESIAN_POINT('Ctrl Pts',(-8.49269364459013,1.01644874085987,24.7792337660389));
#18328=CARTESIAN_POINT('Ctrl Pts',(-8.75839340103342,1.01835862256355,24.7917146992871));
#18329=CARTESIAN_POINT('Ctrl Pts',(-9.02325176140254,0.911059288979746,
24.8041956325353));
#18330=CARTESIAN_POINT('Ctrl Pts',(-9.21270367535734,0.72475850926853,24.8166765657834));
#18331=CARTESIAN_POINT('Ctrl Pts',(-9.40215558931213,0.538457729557314,
24.8291574990316));
#18332=CARTESIAN_POINT('Ctrl Pts',(-9.513881825358,0.275436159673833,24.8416384322798));
#18333=CARTESIAN_POINT('Ctrl Pts',(-9.51642831724056,0.00974174196575487,
24.854119365528));
#18334=CARTESIAN_POINT('Ctrl Pts',(-9.51645943884196,0.00649459406802845,
24.8542718995425));
#18335=CARTESIAN_POINT('Ctrl Pts',(-9.51647499999999,0.00324729703498431,
24.854424433557));
#18336=CARTESIAN_POINT('Ctrl Pts',(-9.516475,1.48351393322478E-12,24.8545769675715));
#18337=CARTESIAN_POINT('Origin',(-8.5,0.,1.24542303242842));
#18338=CARTESIAN_POINT('',(-9.516475,1.3549573406767E-12,24.1954230324284));
#18339=CARTESIAN_POINT('',(-9.516475,1.38190115425627E-12,24.2545769675715));
#18340=CARTESIAN_POINT('',(-9.516475,1.78524650477582E-12,1.24542303242842));
#18341=CARTESIAN_POINT('Ctrl Pts',(-9.516475,1.3549573406767E-12,24.1954230324284));
#18342=CARTESIAN_POINT('Ctrl Pts',(-9.51647500000035,-0.265706620582594,
24.2079039656766));
#18343=CARTESIAN_POINT('Ctrl Pts',(-9.40727465387268,-0.529786878175893,
24.2203848989248));
#18344=CARTESIAN_POINT('Ctrl Pts',(-9.21961691907855,-0.717894780173872,
24.232865832173));
#18345=CARTESIAN_POINT('Ctrl Pts',(-9.03195918428443,-0.906002682171851,
24.2453467654212));
#18346=CARTESIAN_POINT('Ctrl Pts',(-8.76814132834497,-1.01583545019877,
24.2578276986694));
#18347=CARTESIAN_POINT('Ctrl Pts',(-8.50243547044624,-1.0164720823066,24.2703086319176));
#18348=CARTESIAN_POINT('Ctrl Pts',(-8.2367296125475,-1.01710871441442,24.2827895651658));
#18349=CARTESIAN_POINT('Ctrl Pts',(-7.97238846933445,-0.908541417083392,
24.295270498414));
#18350=CARTESIAN_POINT('Ctrl Pts',(-7.78383148002428,-0.721334926799462,
24.3077514316621));
#18351=CARTESIAN_POINT('Ctrl Pts',(-7.59527449071411,-0.534128436515533,
24.3202323649103));
#18352=CARTESIAN_POINT('Ctrl Pts',(-7.48480993131738,-0.27057449675702,
24.3327132981585));
#18353=CARTESIAN_POINT('Ctrl Pts',(-7.48353667075686,-0.00487092690955289,
24.3451942314067));
#18354=CARTESIAN_POINT('Ctrl Pts',(-7.48226341019635,0.260832642937914,
24.3576751646549));
#18355=CARTESIAN_POINT('Ctrl Pts',(-7.59019703546683,0.525433154239234,
24.3701560979031));
#18356=CARTESIAN_POINT('Ctrl Pts',(-7.77695120652423,0.714438148392311,
24.3826370311513));
#18357=CARTESIAN_POINT('Ctrl Pts',(-7.96370537758163,0.903443142545388,
24.3951179643995));
#18358=CARTESIAN_POINT('Ctrl Pts',(-8.2269938881469,1.01453885915621,24.4075988976477));
#18359=CARTESIAN_POINT('Ctrl Pts',(-8.49269364459018,1.01644874085987,24.4200798308958));
#18360=CARTESIAN_POINT('Ctrl Pts',(-8.75839340103347,1.01835862256353,24.432560764144));
#18361=CARTESIAN_POINT('Ctrl Pts',(-9.02325176140259,0.911059288979721,
24.4450416973922));
#18362=CARTESIAN_POINT('Ctrl Pts',(-9.21270367535737,0.724758509268496,
24.4575226306404));
#18363=CARTESIAN_POINT('Ctrl Pts',(-9.40215558931216,0.538457729557271,
24.4700035638886));
#18364=CARTESIAN_POINT('Ctrl Pts',(-9.51388182535801,0.275436159673785,
24.4824844971368));
#18365=CARTESIAN_POINT('Ctrl Pts',(-9.51642831724056,0.00974174196570601,
24.494965430385));
#18366=CARTESIAN_POINT('Ctrl Pts',(-9.51645943884196,0.00649459406794107,
24.4951179643995));
#18367=CARTESIAN_POINT('Ctrl Pts',(-9.516475,0.00324729703485833,24.495270498414));
#18368=CARTESIAN_POINT('Ctrl Pts',(-9.516475,1.31909385888114E-12,24.4954230324284));
#18369=CARTESIAN_POINT('Ctrl Pts',(-9.516475,1.43968106844281E-12,24.2545769675715));
#18370=CARTESIAN_POINT('Ctrl Pts',(-9.51647500000038,-0.265706620582529,
24.2670579008196));
#18371=CARTESIAN_POINT('Ctrl Pts',(-9.4072746538727,-0.529786878175855,
24.2795388340678));
#18372=CARTESIAN_POINT('Ctrl Pts',(-9.21961691907857,-0.717894780173853,
24.292019767316));
#18373=CARTESIAN_POINT('Ctrl Pts',(-9.03195918428444,-0.90600268217185,
24.3045007005642));
#18374=CARTESIAN_POINT('Ctrl Pts',(-8.76814132834496,-1.01583545019878,
24.3169816338124));
#18375=CARTESIAN_POINT('Ctrl Pts',(-8.50243547044621,-1.0164720823066,24.3294625670606));
#18376=CARTESIAN_POINT('Ctrl Pts',(-8.23672961254745,-1.01710871441441,
24.3419435003088));
#18377=CARTESIAN_POINT('Ctrl Pts',(-7.97238846933439,-0.908541417083359,
24.354424433557));
#18378=CARTESIAN_POINT('Ctrl Pts',(-7.78383148002422,-0.7213349267994,24.3669053668052));
#18379=CARTESIAN_POINT('Ctrl Pts',(-7.59527449071405,-0.53412843651544,
24.3793863000534));
#18380=CARTESIAN_POINT('Ctrl Pts',(-7.48480993131734,-0.270574496756893,
24.3918672333016));
#18381=CARTESIAN_POINT('Ctrl Pts',(-7.48353667075686,-0.0048709269094065,
24.4043481665497));
#18382=CARTESIAN_POINT('Ctrl Pts',(-7.48226341019639,0.26083264293808,24.4168290997979));
#18383=CARTESIAN_POINT('Ctrl Pts',(-7.59019703546692,0.525433154239403,
24.4293100330461));
#18384=CARTESIAN_POINT('Ctrl Pts',(-7.77695120652437,0.714438148392456,
24.4417909662943));
#18385=CARTESIAN_POINT('Ctrl Pts',(-7.96370537758183,0.903443142545509,
24.4542718995425));
#18386=CARTESIAN_POINT('Ctrl Pts',(-8.22699388814714,1.01453885915628,24.4667528327907));
#18387=CARTESIAN_POINT('Ctrl Pts',(-8.49269364459044,1.01644874085988,24.4792337660389));
#18388=CARTESIAN_POINT('Ctrl Pts',(-8.75839340103375,1.01835862256347,24.4917146992871));
#18389=CARTESIAN_POINT('Ctrl Pts',(-9.02325176140286,0.91105928897957,24.5041956325353));
#18390=CARTESIAN_POINT('Ctrl Pts',(-9.2127036753576,0.724758509268272,24.5166765657835));
#18391=CARTESIAN_POINT('Ctrl Pts',(-9.40215558931234,0.538457729556974,
24.5291574990316));
#18392=CARTESIAN_POINT('Ctrl Pts',(-9.51388182535812,0.275436159673427,
24.5416384322798));
#18393=CARTESIAN_POINT('Ctrl Pts',(-9.51642831724056,0.00974174196532851,
24.554119365528));
#18394=CARTESIAN_POINT('Ctrl Pts',(-9.51645943884196,0.00649459406771764,
24.5542718995425));
#18395=CARTESIAN_POINT('Ctrl Pts',(-9.51647499999999,0.00324729703478898,
24.554424433557));
#18396=CARTESIAN_POINT('Ctrl Pts',(-9.516475,1.40381758664725E-12,24.5545769675715));
#18397=CARTESIAN_POINT('Origin',(-8.5,0.,1.24542303242842));
#18398=CARTESIAN_POINT('',(-9.516475,1.33304090828571E-12,23.8954230324284));
#18399=CARTESIAN_POINT('',(-9.51638018545619,9.50640762730683E-5,23.9545769675715));
#18400=CARTESIAN_POINT('',(-9.516475,1.78524650477582E-12,1.24542303242842));
#18401=CARTESIAN_POINT('Ctrl Pts',(-9.516475,1.33304090828571E-12,23.8954230324284));
#18402=CARTESIAN_POINT('Ctrl Pts',(-9.51647500000035,-0.265706620582636,
23.9079039656766));
#18403=CARTESIAN_POINT('Ctrl Pts',(-9.40727465387265,-0.52978687817595,
23.9203848989248));
#18404=CARTESIAN_POINT('Ctrl Pts',(-9.2196169190785,-0.717894780173928,
23.932865832173));
#18405=CARTESIAN_POINT('Ctrl Pts',(-9.03195918428434,-0.906002682171906,
23.9453467654212));
#18406=CARTESIAN_POINT('Ctrl Pts',(-8.76814132834485,-1.01583545019881,
23.9578276986694));
#18407=CARTESIAN_POINT('Ctrl Pts',(-8.5024354704461,-1.0164720823066,23.9703086319176));
#18408=CARTESIAN_POINT('Ctrl Pts',(-8.23672961254735,-1.01710871441438,
23.9827895651658));
#18409=CARTESIAN_POINT('Ctrl Pts',(-7.97238846933429,-0.908541417083304,
23.995270498414));
#18410=CARTESIAN_POINT('Ctrl Pts',(-7.78383148002414,-0.721334926799325,
24.0077514316622));
#18411=CARTESIAN_POINT('Ctrl Pts',(-7.59527449071399,-0.534128436515345,
24.0202323649103));
#18412=CARTESIAN_POINT('Ctrl Pts',(-7.48480993131731,-0.270574496756787,
24.0327132981585));
#18413=CARTESIAN_POINT('Ctrl Pts',(-7.48353667075686,-0.00487092690929986,
24.0451942314067));
#18414=CARTESIAN_POINT('Ctrl Pts',(-7.48226341019641,0.260832642938187,
24.0576751646549));
#18415=CARTESIAN_POINT('Ctrl Pts',(-7.59019703546697,0.525433154239499,
24.0701560979031));
#18416=CARTESIAN_POINT('Ctrl Pts',(-7.77695120652445,0.714438148392532,
24.0826370311513));
#18417=CARTESIAN_POINT('Ctrl Pts',(-7.96370537758192,0.903443142545565,
24.0951179643995));
#18418=CARTESIAN_POINT('Ctrl Pts',(-8.22699388814725,1.01453885915631,24.1075988976477));
#18419=CARTESIAN_POINT('Ctrl Pts',(-8.49269364459055,1.01644874085988,24.1200798308959));
#18420=CARTESIAN_POINT('Ctrl Pts',(-8.75839340103385,1.01835862256344,24.1325607641441));
#18421=CARTESIAN_POINT('Ctrl Pts',(-9.02325176140295,0.911059288979515,
24.1450416973922));
#18422=CARTESIAN_POINT('Ctrl Pts',(-9.21270367535768,0.724758509268197,
24.1575226306404));
#18423=CARTESIAN_POINT('Ctrl Pts',(-9.4021555893124,0.538457729556879,24.1700035638886));
#18424=CARTESIAN_POINT('Ctrl Pts',(-9.51388182535815,0.275436159673321,
24.1824844971368));
#18425=CARTESIAN_POINT('Ctrl Pts',(-9.51642831724056,0.00974174196522188,
24.194965430385));
#18426=CARTESIAN_POINT('Ctrl Pts',(-9.51645943884196,0.00649459406763026,
24.1951179643995));
#18427=CARTESIAN_POINT('Ctrl Pts',(-9.516475,0.0032472970347209,24.195270498414));
#18428=CARTESIAN_POINT('Ctrl Pts',(-9.516475,1.3549573406767E-12,24.1954230324284));
#18429=CARTESIAN_POINT('Ctrl Pts',(-9.516475,1.30220480767874E-12,23.9545769675715));
#18430=CARTESIAN_POINT('Ctrl Pts',(-9.51647500000034,-0.265706620582667,
23.9670579008197));
#18431=CARTESIAN_POINT('Ctrl Pts',(-9.40727465387263,-0.529786878175978,
23.9795388340678));
#18432=CARTESIAN_POINT('Ctrl Pts',(-9.21961691907847,-0.71789478017395,
23.992019767316));
#18433=CARTESIAN_POINT('Ctrl Pts',(-9.03195918428432,-0.906002682171922,
24.0045007005642));
#18434=CARTESIAN_POINT('Ctrl Pts',(-8.76814132834482,-1.01583545019881,
24.0169816338124));
#18435=CARTESIAN_POINT('Ctrl Pts',(-8.50243547044607,-1.0164720823066,24.0294625670606));
#18436=CARTESIAN_POINT('Ctrl Pts',(-8.23672961254731,-1.01710871441438,
24.0419435003088));
#18437=CARTESIAN_POINT('Ctrl Pts',(-7.97238846933426,-0.908541417083288,
24.054424433557));
#18438=CARTESIAN_POINT('Ctrl Pts',(-7.78383148002412,-0.721334926799303,
24.0669053668052));
#18439=CARTESIAN_POINT('Ctrl Pts',(-7.59527449071398,-0.534128436515318,
24.0793863000534));
#18440=CARTESIAN_POINT('Ctrl Pts',(-7.4848099313173,-0.270574496756756,
24.0918672333016));
#18441=CARTESIAN_POINT('Ctrl Pts',(-7.48353667075686,-0.00487092690926902,
24.1043481665497));
#18442=CARTESIAN_POINT('Ctrl Pts',(-7.48226341019642,0.260832642938218,
24.1168290997979));
#18443=CARTESIAN_POINT('Ctrl Pts',(-7.59019703546699,0.525433154239526,
24.1293100330461));
#18444=CARTESIAN_POINT('Ctrl Pts',(-7.77695120652447,0.714438148392554,
24.1417909662943));
#18445=CARTESIAN_POINT('Ctrl Pts',(-7.96370537758195,0.903443142545582,
24.1542718995425));
#18446=CARTESIAN_POINT('Ctrl Pts',(-8.22699388814728,1.01453885915632,24.1667528327907));
#18447=CARTESIAN_POINT('Ctrl Pts',(-8.49269364459058,1.01644874085988,24.1792337660389));
#18448=CARTESIAN_POINT('Ctrl Pts',(-8.75839340103389,1.01835862256343,24.1917146992871));
#18449=CARTESIAN_POINT('Ctrl Pts',(-9.02325176140298,0.9110592889795,24.2041956325353));
#18450=CARTESIAN_POINT('Ctrl Pts',(-9.2127036753577,0.724758509268176,24.2166765657835));
#18451=CARTESIAN_POINT('Ctrl Pts',(-9.40215558931242,0.538457729556852,
24.2291574990317));
#18452=CARTESIAN_POINT('Ctrl Pts',(-9.51388182535815,0.27543615967329,24.2416384322798));
#18453=CARTESIAN_POINT('Ctrl Pts',(-9.51642831724056,0.00974174196519104,
24.254119365528));
#18454=CARTESIAN_POINT('Ctrl Pts',(-9.51645943884196,0.00649459406763794,
24.2542718995425));
#18455=CARTESIAN_POINT('Ctrl Pts',(-9.51647499999999,0.00324729703476719,
24.254424433557));
#18456=CARTESIAN_POINT('Ctrl Pts',(-9.516475,1.43968106844281E-12,24.2545769675715));
#18457=CARTESIAN_POINT('Origin',(-8.5,0.,1.24542303242842));
#18458=CARTESIAN_POINT('',(-9.516475,1.31112447589473E-12,23.5954230324284));
#18459=CARTESIAN_POINT('',(-9.51682532410723,4.86896733354835E-5,23.6545769675715));
#18460=CARTESIAN_POINT('',(-9.516475,1.78524650477582E-12,1.24542303242842));
#18461=CARTESIAN_POINT('Ctrl Pts',(-9.516475,1.36890439008127E-12,23.5954230324284));
#18462=CARTESIAN_POINT('Ctrl Pts',(-9.51647500000036,-0.265706620582619,
23.6079039656766));
#18463=CARTESIAN_POINT('Ctrl Pts',(-9.40727465387265,-0.529786878175956,
23.6203848989248));
#18464=CARTESIAN_POINT('Ctrl Pts',(-9.21961691907848,-0.717894780173944,
23.632865832173));
#18465=CARTESIAN_POINT('Ctrl Pts',(-9.03195918428431,-0.906002682171931,
23.6453467654212));
#18466=CARTESIAN_POINT('Ctrl Pts',(-8.76814132834479,-1.01583545019883,
23.6578276986694));
#18467=CARTESIAN_POINT('Ctrl Pts',(-8.50243547044602,-1.0164720823066,23.6703086319176));
#18468=CARTESIAN_POINT('Ctrl Pts',(-8.23672961254725,-1.01710871441436,
23.6827895651658));
#18469=CARTESIAN_POINT('Ctrl Pts',(-7.97238846933418,-0.908541417083246,
23.695270498414));
#18470=CARTESIAN_POINT('Ctrl Pts',(-7.78383148002404,-0.721334926799228,
23.7077514316622));
#18471=CARTESIAN_POINT('Ctrl Pts',(-7.59527449071391,-0.534128436515209,
23.7202323649103));
#18472=CARTESIAN_POINT('Ctrl Pts',(-7.48480993131726,-0.270574496756611,
23.7327132981585));
#18473=CARTESIAN_POINT('Ctrl Pts',(-7.48353667075686,-0.00487092690910461,
23.7451942314067));
#18474=CARTESIAN_POINT('Ctrl Pts',(-7.48226341019646,0.260832642938402,
23.7576751646549));
#18475=CARTESIAN_POINT('Ctrl Pts',(-7.59019703546709,0.525433154239711,
23.7701560979031));
#18476=CARTESIAN_POINT('Ctrl Pts',(-7.77695120652463,0.714438148392712,
23.7826370311513));
#18477=CARTESIAN_POINT('Ctrl Pts',(-7.96370537758216,0.903443142545713,
23.7951179643995));
#18478=CARTESIAN_POINT('Ctrl Pts',(-8.22699388814754,1.0145388591564,23.8075988976477));
#18479=CARTESIAN_POINT('Ctrl Pts',(-8.49269364459086,1.01644874085988,23.8200798308959));
#18480=CARTESIAN_POINT('Ctrl Pts',(-8.75839340103419,1.01835862256336,23.8325607641441));
#18481=CARTESIAN_POINT('Ctrl Pts',(-9.02325176140327,0.911059288979339,
23.8450416973923));
#18482=CARTESIAN_POINT('Ctrl Pts',(-9.21270367535794,0.724758509267939,
23.8575226306405));
#18483=CARTESIAN_POINT('Ctrl Pts',(-9.40215558931261,0.538457729556538,
23.8700035638886));
#18484=CARTESIAN_POINT('Ctrl Pts',(-9.51388182535826,0.275436159672915,
23.8824844971368));
#18485=CARTESIAN_POINT('Ctrl Pts',(-9.51642831724057,0.00974174196479552,
23.894965430385));
#18486=CARTESIAN_POINT('Ctrl Pts',(-9.51645943884196,0.0064945940673387,
23.8951179643995));
#18487=CARTESIAN_POINT('Ctrl Pts',(-9.516475,0.00324729703456413,23.895270498414));
#18488=CARTESIAN_POINT('Ctrl Pts',(-9.516475,1.33304090828571E-12,23.8954230324284));
#18489=CARTESIAN_POINT('Ctrl Pts',(-9.51796493798108,0.000207078507120715,
23.6545769675715));
#18490=CARTESIAN_POINT('Ctrl Pts',(-9.51706691021463,-0.325585595105403,
23.669948946367));
#18491=CARTESIAN_POINT('Ctrl Pts',(-9.17147099560746,-0.99017940908471,
23.7012282663142));
#18492=CARTESIAN_POINT('Ctrl Pts',(-8.03686629447588,-1.10987867419518,
23.7484149274131));
#18493=CARTESIAN_POINT('Ctrl Pts',(-7.43826157375447,-0.361085119319684,
23.7881832802921));
#18494=CARTESIAN_POINT('Ctrl Pts',(-7.49794123728335,0.335385184319912,
23.8199979625954));
#18495=CARTESIAN_POINT('Ctrl Pts',(-7.86953258335037,0.927459856653405,
23.8518126448985));
#18496=CARTESIAN_POINT('Ctrl Pts',(-8.79827787305733,1.16505528240947,23.8915809977777));
#18497=CARTESIAN_POINT('Ctrl Pts',(-9.45053929968385,0.556114497354683,
23.9284869955272));
#18498=CARTESIAN_POINT('Ctrl Pts',(-9.51659141321842,0.1093069840508,23.9494856521251));
#18499=CARTESIAN_POINT('Ctrl Pts',(-9.51572863211466,0.000748332163859972,
23.9545769675715));
#18500=CARTESIAN_POINT('Origin',(-8.5,0.,1.24542303242842));
#18501=CARTESIAN_POINT('',(-9.516475,1.28920804350374E-12,23.2954230324284));
#18502=CARTESIAN_POINT('',(-9.516475,1.31615185708331E-12,23.3545769675715));
#18503=CARTESIAN_POINT('',(-9.516475,1.78524650477582E-12,1.24542303242842));
#18504=CARTESIAN_POINT('Ctrl Pts',(-9.516475,1.34698795769028E-12,23.2954230324284));
#18505=CARTESIAN_POINT('Ctrl Pts',(-9.51647500000035,-0.265706620582641,
23.3079039656766));
#18506=CARTESIAN_POINT('Ctrl Pts',(-9.40727465387264,-0.529786878175976,
23.3203848989248));
#18507=CARTESIAN_POINT('Ctrl Pts',(-9.21961691907847,-0.717894780173959,
23.332865832173));
#18508=CARTESIAN_POINT('Ctrl Pts',(-9.03195918428429,-0.906002682171943,
23.3453467654212));
#18509=CARTESIAN_POINT('Ctrl Pts',(-8.76814132834477,-1.01583545019883,
23.3578276986694));
#18510=CARTESIAN_POINT('Ctrl Pts',(-8.502435470446,-1.0164720823066,23.3703086319176));
#18511=CARTESIAN_POINT('Ctrl Pts',(-8.23672961254722,-1.01710871441436,
23.3827895651658));
#18512=CARTESIAN_POINT('Ctrl Pts',(-7.97238846933416,-0.908541417083235,
23.395270498414));
#18513=CARTESIAN_POINT('Ctrl Pts',(-7.78383148002403,-0.721334926799212,
23.4077514316622));
#18514=CARTESIAN_POINT('Ctrl Pts',(-7.5952744907139,-0.53412843651519,23.4202323649104));
#18515=CARTESIAN_POINT('Ctrl Pts',(-7.48480993131725,-0.270574496756589,
23.4327132981585));
#18516=CARTESIAN_POINT('Ctrl Pts',(-7.48353667075686,-0.00487092690908269,
23.4451942314067));
#18517=CARTESIAN_POINT('Ctrl Pts',(-7.48226341019647,0.260832642938424,
23.4576751646549));
#18518=CARTESIAN_POINT('Ctrl Pts',(-7.5901970354671,0.525433154239731,23.4701560979031));
#18519=CARTESIAN_POINT('Ctrl Pts',(-7.77695120652464,0.714438148392727,
23.4826370311513));
#18520=CARTESIAN_POINT('Ctrl Pts',(-7.96370537758218,0.903443142545724,
23.4951179643995));
#18521=CARTESIAN_POINT('Ctrl Pts',(-8.22699388814756,1.0145388591564,23.5075988976477));
#18522=CARTESIAN_POINT('Ctrl Pts',(-8.49269364459088,1.01644874085988,23.5200798308959));
#18523=CARTESIAN_POINT('Ctrl Pts',(-8.75839340103421,1.01835862256336,23.5325607641441));
#18524=CARTESIAN_POINT('Ctrl Pts',(-9.02325176140329,0.911059288979328,
23.5450416973923));
#18525=CARTESIAN_POINT('Ctrl Pts',(-9.21270367535795,0.724758509267924,
23.5575226306405));
#18526=CARTESIAN_POINT('Ctrl Pts',(-9.40215558931262,0.538457729556519,
23.5700035638886));
#18527=CARTESIAN_POINT('Ctrl Pts',(-9.51388182535827,0.275436159672893,
23.5824844971368));
#18528=CARTESIAN_POINT('Ctrl Pts',(-9.51642831724057,0.00974174196477361,
23.594965430385));
#18529=CARTESIAN_POINT('Ctrl Pts',(-9.51645943884196,0.00649459406733604,
23.5951179643995));
#18530=CARTESIAN_POINT('Ctrl Pts',(-9.516475,0.00324729703458077,23.595270498414));
#18531=CARTESIAN_POINT('Ctrl Pts',(-9.516475,1.36890439008127E-12,23.5954230324284));
#18532=CARTESIAN_POINT('Ctrl Pts',(-9.516475,1.43171168545639E-12,23.3545769675715));
#18533=CARTESIAN_POINT('Ctrl Pts',(-9.51647500000037,-0.265706620582537,
23.3670579008196));
#18534=CARTESIAN_POINT('Ctrl Pts',(-9.4072746538727,-0.529786878175862,
23.3795388340678));
#18535=CARTESIAN_POINT('Ctrl Pts',(-9.21961691907857,-0.717894780173858,
23.392019767316));
#18536=CARTESIAN_POINT('Ctrl Pts',(-9.03195918428443,-0.906002682171854,
23.4045007005642));
#18537=CARTESIAN_POINT('Ctrl Pts',(-8.76814132834495,-1.01583545019878,
23.4169816338124));
#18538=CARTESIAN_POINT('Ctrl Pts',(-8.5024354704462,-1.0164720823066,23.4294625670606));
#18539=CARTESIAN_POINT('Ctrl Pts',(-8.23672961254744,-1.01710871441441,
23.4419435003088));
#18540=CARTESIAN_POINT('Ctrl Pts',(-7.97238846933438,-0.908541417083355,
23.454424433557));
#18541=CARTESIAN_POINT('Ctrl Pts',(-7.78383148002421,-0.721334926799394,
23.4669053668052));
#18542=CARTESIAN_POINT('Ctrl Pts',(-7.59527449071404,-0.534128436515433,
23.4793863000534));
#18543=CARTESIAN_POINT('Ctrl Pts',(-7.48480993131734,-0.270574496756885,
23.4918672333016));
#18544=CARTESIAN_POINT('Ctrl Pts',(-7.48353667075686,-0.00487092690939853,
23.5043481665497));
#18545=CARTESIAN_POINT('Ctrl Pts',(-7.48226341019639,0.260832642938088,
23.5168290997979));
#18546=CARTESIAN_POINT('Ctrl Pts',(-7.59019703546692,0.52543315423941,23.5293100330461));
#18547=CARTESIAN_POINT('Ctrl Pts',(-7.77695120652438,0.714438148392462,
23.5417909662943));
#18548=CARTESIAN_POINT('Ctrl Pts',(-7.96370537758184,0.903443142545513,
23.5542718995425));
#18549=CARTESIAN_POINT('Ctrl Pts',(-8.22699388814715,1.01453885915629,23.5667528327907));
#18550=CARTESIAN_POINT('Ctrl Pts',(-8.49269364459045,1.01644874085988,23.5792337660389));
#18551=CARTESIAN_POINT('Ctrl Pts',(-8.75839340103376,1.01835862256347,23.5917146992871));
#18552=CARTESIAN_POINT('Ctrl Pts',(-9.02325176140286,0.911059288979566,
23.6041956325353));
#18553=CARTESIAN_POINT('Ctrl Pts',(-9.21270367535761,0.724758509268266,
23.6166765657835));
#18554=CARTESIAN_POINT('Ctrl Pts',(-9.40215558931235,0.538457729556966,
23.6291574990316));
#18555=CARTESIAN_POINT('Ctrl Pts',(-9.51388182535812,0.275436159673419,
23.6416384322798));
#18556=CARTESIAN_POINT('Ctrl Pts',(-9.51642831724056,0.00974174196532054,
23.654119365528));
#18557=CARTESIAN_POINT('Ctrl Pts',(-9.51645943884196,0.00649459406769041,
23.6542718995425));
#18558=CARTESIAN_POINT('Ctrl Pts',(-9.516475,0.00324729703474261,23.654424433557));
#18559=CARTESIAN_POINT('Ctrl Pts',(-9.516475,1.3380682894743E-12,23.6545769675715));
#18560=CARTESIAN_POINT('Origin',(-8.5,0.,1.24542303242842));
#18561=CARTESIAN_POINT('',(-9.516475,1.26729161111276E-12,22.9954230324284));
#18562=CARTESIAN_POINT('',(-9.516475,1.29423542469233E-12,23.0545769675715));
#18563=CARTESIAN_POINT('',(-9.516475,1.78524650477582E-12,1.24542303242842));
#18564=CARTESIAN_POINT('Ctrl Pts',(-9.516475,1.26729161111276E-12,22.9954230324284));
#18565=CARTESIAN_POINT('Ctrl Pts',(-9.51647500000033,-0.265706620582721,
23.0079039656766));
#18566=CARTESIAN_POINT('Ctrl Pts',(-9.4072746538726,-0.529786878176047,
23.0203848989248));
#18567=CARTESIAN_POINT('Ctrl Pts',(-9.21961691907841,-0.717894780174016,
23.032865832173));
#18568=CARTESIAN_POINT('Ctrl Pts',(-9.03195918428422,-0.906002682171985,
23.0453467654212));
#18569=CARTESIAN_POINT('Ctrl Pts',(-8.76814132834469,-1.01583545019885,
23.0578276986694));
#18570=CARTESIAN_POINT('Ctrl Pts',(-8.50243547044592,-1.0164720823066,23.0703086319176));
#18571=CARTESIAN_POINT('Ctrl Pts',(-8.23672961254715,-1.01710871441434,
23.0827895651658));
#18572=CARTESIAN_POINT('Ctrl Pts',(-7.97238846933409,-0.908541417083194,
23.095270498414));
#18573=CARTESIAN_POINT('Ctrl Pts',(-7.78383148002397,-0.721334926799156,
23.1077514316622));
#18574=CARTESIAN_POINT('Ctrl Pts',(-7.59527449071385,-0.534128436515119,
23.1202323649104));
#18575=CARTESIAN_POINT('Ctrl Pts',(-7.48480993131723,-0.270574496756509,
23.1327132981585));
#18576=CARTESIAN_POINT('Ctrl Pts',(-7.48353667075686,-0.00487092690900299,
23.1451942314067));
#18577=CARTESIAN_POINT('Ctrl Pts',(-7.48226341019649,0.260832642938503,
23.1576751646549));
#18578=CARTESIAN_POINT('Ctrl Pts',(-7.59019703546714,0.525433154239802,
23.1701560979031));
#18579=CARTESIAN_POINT('Ctrl Pts',(-7.7769512065247,0.714438148392784,23.1826370311513));
#18580=CARTESIAN_POINT('Ctrl Pts',(-7.96370537758225,0.903443142545766,
23.1951179643995));
#18581=CARTESIAN_POINT('Ctrl Pts',(-8.22699388814764,1.01453885915642,23.2075988976477));
#18582=CARTESIAN_POINT('Ctrl Pts',(-8.49269364459096,1.01644874085988,23.2200798308959));
#18583=CARTESIAN_POINT('Ctrl Pts',(-8.75839340103429,1.01835862256334,23.2325607641441));
#18584=CARTESIAN_POINT('Ctrl Pts',(-9.02325176140336,0.911059288979287,
23.2450416973923));
#18585=CARTESIAN_POINT('Ctrl Pts',(-9.21270367535801,0.724758509267868,
23.2575226306405));
#18586=CARTESIAN_POINT('Ctrl Pts',(-9.40215558931266,0.538457729556448,
23.2700035638887));
#18587=CARTESIAN_POINT('Ctrl Pts',(-9.51388182535829,0.275436159672814,
23.2824844971368));
#18588=CARTESIAN_POINT('Ctrl Pts',(-9.51642831724057,0.00974174196469391,
23.294965430385));
#18589=CARTESIAN_POINT('Ctrl Pts',(-9.51645943884196,0.00649459406727561,
23.2951179643995));
#18590=CARTESIAN_POINT('Ctrl Pts',(-9.516475,0.00324729703453964,23.295270498414));
#18591=CARTESIAN_POINT('Ctrl Pts',(-9.516475,1.34698795769028E-12,23.2954230324284));
#18592=CARTESIAN_POINT('Ctrl Pts',(-9.516475,1.35201533887887E-12,23.0545769675715));
#18593=CARTESIAN_POINT('Ctrl Pts',(-9.51647500000035,-0.265706620582617,
23.0670579008197));
#18594=CARTESIAN_POINT('Ctrl Pts',(-9.40727465387266,-0.529786878175934,
23.0795388340678));
#18595=CARTESIAN_POINT('Ctrl Pts',(-9.21961691907851,-0.717894780173915,
23.092019767316));
#18596=CARTESIAN_POINT('Ctrl Pts',(-9.03195918428436,-0.906002682171896,
23.1045007005642));
#18597=CARTESIAN_POINT('Ctrl Pts',(-8.76814132834487,-1.0158354501988,23.1169816338124));
#18598=CARTESIAN_POINT('Ctrl Pts',(-8.50243547044612,-1.0164720823066,23.1294625670606));
#18599=CARTESIAN_POINT('Ctrl Pts',(-8.23672961254736,-1.01710871441439,
23.1419435003088));
#18600=CARTESIAN_POINT('Ctrl Pts',(-7.97238846933431,-0.908541417083314,
23.154424433557));
#18601=CARTESIAN_POINT('Ctrl Pts',(-7.78383148002415,-0.721334926799338,
23.1669053668052));
#18602=CARTESIAN_POINT('Ctrl Pts',(-7.595274490714,-0.534128436515362,23.1793863000534));
#18603=CARTESIAN_POINT('Ctrl Pts',(-7.48480993131732,-0.270574496756806,
23.1918672333016));
#18604=CARTESIAN_POINT('Ctrl Pts',(-7.48353667075686,-0.00487092690931883,
23.2043481665497));
#18605=CARTESIAN_POINT('Ctrl Pts',(-7.48226341019641,0.260832642938168,
23.2168290997979));
#18606=CARTESIAN_POINT('Ctrl Pts',(-7.59019703546696,0.525433154239481,
23.2293100330461));
#18607=CARTESIAN_POINT('Ctrl Pts',(-7.77695120652444,0.714438148392518,
23.2417909662943));
#18608=CARTESIAN_POINT('Ctrl Pts',(-7.96370537758191,0.903443142545555,
23.2542718995425));
#18609=CARTESIAN_POINT('Ctrl Pts',(-8.22699388814723,1.01453885915631,23.2667528327907));
#18610=CARTESIAN_POINT('Ctrl Pts',(-8.49269364459053,1.01644874085988,23.2792337660389));
#18611=CARTESIAN_POINT('Ctrl Pts',(-8.75839340103384,1.01835862256345,23.2917146992871));
#18612=CARTESIAN_POINT('Ctrl Pts',(-9.02325176140294,0.911059288979525,
23.3041956325353));
#18613=CARTESIAN_POINT('Ctrl Pts',(-9.21270367535766,0.72475850926821,23.3166765657835));
#18614=CARTESIAN_POINT('Ctrl Pts',(-9.40215558931239,0.538457729556896,
23.3291574990317));
#18615=CARTESIAN_POINT('Ctrl Pts',(-9.51388182535814,0.27543615967334,23.3416384322798));
#18616=CARTESIAN_POINT('Ctrl Pts',(-9.51642831724056,0.00974174196524085,
23.354119365528));
#18617=CARTESIAN_POINT('Ctrl Pts',(-9.51645943884196,0.00649459406766849,
23.3542718995425));
#18618=CARTESIAN_POINT('Ctrl Pts',(-9.51647499999999,0.00324729703477843,
23.354424433557));
#18619=CARTESIAN_POINT('Ctrl Pts',(-9.516475,1.43171168545639E-12,23.3545769675715));
#18620=CARTESIAN_POINT('Origin',(-8.5,0.,1.24542303242842));
#18621=CARTESIAN_POINT('',(-9.516475,1.24537517872177E-12,22.6954230324284));
#18622=CARTESIAN_POINT('',(-9.516475,1.27231899230134E-12,22.7545769675715));
#18623=CARTESIAN_POINT('',(-9.516475,1.78524650477582E-12,1.24542303242842));
#18624=CARTESIAN_POINT('Ctrl Pts',(-9.516475,1.30315509290831E-12,22.6954230324284));
#18625=CARTESIAN_POINT('Ctrl Pts',(-9.51647500000034,-0.265706620582666,
22.7079039656766));
#18626=CARTESIAN_POINT('Ctrl Pts',(-9.40727465387263,-0.529786878175977,
22.7203848989248));
#18627=CARTESIAN_POINT('Ctrl Pts',(-9.21961691907848,-0.717894780173949,
22.732865832173));
#18628=CARTESIAN_POINT('Ctrl Pts',(-9.03195918428432,-0.906002682171922,
22.7453467654212));
#18629=CARTESIAN_POINT('Ctrl Pts',(-8.76814132834482,-1.01583545019881,
22.7578276986694));
#18630=CARTESIAN_POINT('Ctrl Pts',(-8.50243547044607,-1.0164720823066,22.7703086319176));
#18631=CARTESIAN_POINT('Ctrl Pts',(-8.23672961254732,-1.01710871441438,
22.7827895651658));
#18632=CARTESIAN_POINT('Ctrl Pts',(-7.97238846933426,-0.908541417083289,
22.795270498414));
#18633=CARTESIAN_POINT('Ctrl Pts',(-7.78383148002412,-0.721334926799304,
22.8077514316622));
#18634=CARTESIAN_POINT('Ctrl Pts',(-7.59527449071398,-0.534128436515318,
22.8202323649103));
#18635=CARTESIAN_POINT('Ctrl Pts',(-7.4848099313173,-0.270574496756757,
22.8327132981585));
#18636=CARTESIAN_POINT('Ctrl Pts',(-7.48353667075686,-0.00487092690926997,
22.8451942314067));
#18637=CARTESIAN_POINT('Ctrl Pts',(-7.48226341019642,0.260832642938217,
22.8576751646549));
#18638=CARTESIAN_POINT('Ctrl Pts',(-7.59019703546699,0.525433154239525,
22.8701560979031));
#18639=CARTESIAN_POINT('Ctrl Pts',(-7.77695120652447,0.714438148392553,
22.8826370311513));
#18640=CARTESIAN_POINT('Ctrl Pts',(-7.96370537758195,0.903443142545581,
22.8951179643995));
#18641=CARTESIAN_POINT('Ctrl Pts',(-8.22699388814728,1.01453885915632,22.9075988976477));
#18642=CARTESIAN_POINT('Ctrl Pts',(-8.49269364459058,1.01644874085988,22.9200798308959));
#18643=CARTESIAN_POINT('Ctrl Pts',(-8.75839340103389,1.01835862256343,22.9325607641441));
#18644=CARTESIAN_POINT('Ctrl Pts',(-9.02325176140298,0.9110592889795,22.9450416973922));
#18645=CARTESIAN_POINT('Ctrl Pts',(-9.2127036753577,0.724758509268176,22.9575226306404));
#18646=CARTESIAN_POINT('Ctrl Pts',(-9.40215558931242,0.538457729556853,
22.9700035638886));
#18647=CARTESIAN_POINT('Ctrl Pts',(-9.51388182535815,0.275436159673291,
22.9824844971368));
#18648=CARTESIAN_POINT('Ctrl Pts',(-9.51642831724056,0.00974174196519199,
22.994965430385));
#18649=CARTESIAN_POINT('Ctrl Pts',(-9.51645943884196,0.00649459406758111,
22.9951179643995));
#18650=CARTESIAN_POINT('Ctrl Pts',(-9.516475,0.00324729703465245,22.995270498414));
#18651=CARTESIAN_POINT('Ctrl Pts',(-9.516475,1.26729161111276E-12,22.9954230324284));
#18652=CARTESIAN_POINT('Ctrl Pts',(-9.516475,1.33009890648788E-12,22.7545769675715));
#18653=CARTESIAN_POINT('Ctrl Pts',(-9.51647500000035,-0.265706620582639,
22.7670579008197));
#18654=CARTESIAN_POINT('Ctrl Pts',(-9.40727465387265,-0.529786878175953,
22.7795388340678));
#18655=CARTESIAN_POINT('Ctrl Pts',(-9.21961691907849,-0.71789478017393,
22.792019767316));
#18656=CARTESIAN_POINT('Ctrl Pts',(-9.03195918428434,-0.906002682171908,
22.8045007005642));
#18657=CARTESIAN_POINT('Ctrl Pts',(-8.76814132834485,-1.01583545019881,
22.8169816338124));
#18658=CARTESIAN_POINT('Ctrl Pts',(-8.5024354704461,-1.0164720823066,22.8294625670606));
#18659=CARTESIAN_POINT('Ctrl Pts',(-8.23672961254734,-1.01710871441438,
22.8419435003088));
#18660=CARTESIAN_POINT('Ctrl Pts',(-7.97238846933429,-0.908541417083303,
22.854424433557));
#18661=CARTESIAN_POINT('Ctrl Pts',(-7.78383148002414,-0.721334926799323,
22.8669053668052));
#18662=CARTESIAN_POINT('Ctrl Pts',(-7.59527449071399,-0.534128436515342,
22.8793863000534));
#18663=CARTESIAN_POINT('Ctrl Pts',(-7.48480993131731,-0.270574496756784,
22.8918672333016));
#18664=CARTESIAN_POINT('Ctrl Pts',(-7.48353667075686,-0.00487092690929692,
22.9043481665497));
#18665=CARTESIAN_POINT('Ctrl Pts',(-7.48226341019642,0.26083264293819,22.9168290997979));
#18666=CARTESIAN_POINT('Ctrl Pts',(-7.59019703546697,0.525433154239501,
22.9293100330461));
#18667=CARTESIAN_POINT('Ctrl Pts',(-7.77695120652445,0.714438148392534,
22.9417909662943));
#18668=CARTESIAN_POINT('Ctrl Pts',(-7.96370537758193,0.903443142545567,
22.9542718995425));
#18669=CARTESIAN_POINT('Ctrl Pts',(-8.22699388814725,1.01453885915631,22.9667528327907));
#18670=CARTESIAN_POINT('Ctrl Pts',(-8.49269364459055,1.01644874085988,22.9792337660389));
#18671=CARTESIAN_POINT('Ctrl Pts',(-8.75839340103386,1.01835862256344,22.9917146992871));
#18672=CARTESIAN_POINT('Ctrl Pts',(-9.02325176140296,0.911059288979514,
23.0041956325353));
#18673=CARTESIAN_POINT('Ctrl Pts',(-9.21270367535768,0.724758509268195,
23.0166765657835));
#18674=CARTESIAN_POINT('Ctrl Pts',(-9.4021555893124,0.538457729556876,23.0291574990317));
#18675=CARTESIAN_POINT('Ctrl Pts',(-9.51388182535815,0.275436159673318,
23.0416384322798));
#18676=CARTESIAN_POINT('Ctrl Pts',(-9.51642831724056,0.00974174196521894,
23.054119365528));
#18677=CARTESIAN_POINT('Ctrl Pts',(-9.51645943884196,0.00649459406762731,
23.0542718995425));
#18678=CARTESIAN_POINT('Ctrl Pts',(-9.516475,0.00324729703471796,23.054424433557));
#18679=CARTESIAN_POINT('Ctrl Pts',(-9.516475,1.35201533887887E-12,23.0545769675715));
#18680=CARTESIAN_POINT('Origin',(-8.5,0.,1.24542303242842));
#18681=CARTESIAN_POINT('',(-9.5160605096938,-0.00010514095004287,22.3954230324284));
#18682=CARTESIAN_POINT('',(-9.516475,1.25040255991036E-12,22.4545769675715));
#18683=CARTESIAN_POINT('',(-9.516475,1.78524650477582E-12,1.24542303242842));
#18684=CARTESIAN_POINT('Ctrl Pts',(-9.516475,1.28123866051733E-12,22.3954230324284));
#18685=CARTESIAN_POINT('Ctrl Pts',(-9.51647500000034,-0.265706620582688,
22.4079039656766));
#18686=CARTESIAN_POINT('Ctrl Pts',(-9.40727465387262,-0.529786878175997,
22.4203848989248));
#18687=CARTESIAN_POINT('Ctrl Pts',(-9.21961691907846,-0.717894780173965,
22.432865832173));
#18688=CARTESIAN_POINT('Ctrl Pts',(-9.0319591842843,-0.906002682171933,
22.4453467654212));
#18689=CARTESIAN_POINT('Ctrl Pts',(-8.7681413283448,-1.01583545019882,22.4578276986694));
#18690=CARTESIAN_POINT('Ctrl Pts',(-8.50243547044605,-1.0164720823066,22.4703086319176));
#18691=CARTESIAN_POINT('Ctrl Pts',(-8.23672961254729,-1.01710871441437,
22.4827895651658));
#18692=CARTESIAN_POINT('Ctrl Pts',(-7.97238846933424,-0.908541417083277,
22.495270498414));
#18693=CARTESIAN_POINT('Ctrl Pts',(-7.7838314800241,-0.721334926799288,
22.5077514316622));
#18694=CARTESIAN_POINT('Ctrl Pts',(-7.59527449071397,-0.534128436515299,
22.5202323649103));
#18695=CARTESIAN_POINT('Ctrl Pts',(-7.4848099313173,-0.270574496756735,
22.5327132981585));
#18696=CARTESIAN_POINT('Ctrl Pts',(-7.48353667075686,-0.00487092690924806,
22.5451942314067));
#18697=CARTESIAN_POINT('Ctrl Pts',(-7.48226341019643,0.260832642938239,
22.5576751646549));
#18698=CARTESIAN_POINT('Ctrl Pts',(-7.590197035467,0.525433154239545,22.5701560979031));
#18699=CARTESIAN_POINT('Ctrl Pts',(-7.77695120652449,0.714438148392569,
22.5826370311513));
#18700=CARTESIAN_POINT('Ctrl Pts',(-7.96370537758197,0.903443142545593,
22.5951179643995));
#18701=CARTESIAN_POINT('Ctrl Pts',(-8.2269938881473,1.01453885915633,22.6075988976477));
#18702=CARTESIAN_POINT('Ctrl Pts',(-8.4926936445906,1.01644874085988,22.6200798308959));
#18703=CARTESIAN_POINT('Ctrl Pts',(-8.75839340103391,1.01835862256343,22.6325607641441));
#18704=CARTESIAN_POINT('Ctrl Pts',(-9.023251761403,0.911059288979489,22.6450416973922));
#18705=CARTESIAN_POINT('Ctrl Pts',(-9.21270367535771,0.724758509268161,
22.6575226306404));
#18706=CARTESIAN_POINT('Ctrl Pts',(-9.40215558931243,0.538457729556833,
22.6700035638886));
#18707=CARTESIAN_POINT('Ctrl Pts',(-9.51388182535816,0.275436159673269,
22.6824844971368));
#18708=CARTESIAN_POINT('Ctrl Pts',(-9.51642831724056,0.00974174196517008,
22.694965430385));
#18709=CARTESIAN_POINT('Ctrl Pts',(-9.51645943884196,0.00649459406757845,
22.6951179643995));
#18710=CARTESIAN_POINT('Ctrl Pts',(-9.516475,0.0032472970346691,22.695270498414));
#18711=CARTESIAN_POINT('Ctrl Pts',(-9.516475,1.30315509290831E-12,22.6954230324284));
#18712=CARTESIAN_POINT('Ctrl Pts',(-9.516475,1.25040255991036E-12,22.4545769675715));
#18713=CARTESIAN_POINT('Ctrl Pts',(-9.51647500000033,-0.265706620582718,
22.4670579008197));
#18714=CARTESIAN_POINT('Ctrl Pts',(-9.4072746538726,-0.529786878176024,
22.4795388340678));
#18715=CARTESIAN_POINT('Ctrl Pts',(-9.21961691907844,-0.717894780173987,
22.492019767316));
#18716=CARTESIAN_POINT('Ctrl Pts',(-9.03195918428427,-0.906002682171949,
22.5045007005642));
#18717=CARTESIAN_POINT('Ctrl Pts',(-8.76814132834477,-1.01583545019883,
22.5169816338124));
#18718=CARTESIAN_POINT('Ctrl Pts',(-8.50243547044602,-1.0164720823066,22.5294625670606));
#18719=CARTESIAN_POINT('Ctrl Pts',(-8.23672961254726,-1.01710871441436,
22.5419435003088));
#18720=CARTESIAN_POINT('Ctrl Pts',(-7.97238846933422,-0.908541417083261,
22.554424433557));
#18721=CARTESIAN_POINT('Ctrl Pts',(-7.78383148002408,-0.721334926799266,
22.5669053668052));
#18722=CARTESIAN_POINT('Ctrl Pts',(-7.59527449071395,-0.534128436515272,
22.5793863000534));
#18723=CARTESIAN_POINT('Ctrl Pts',(-7.48480993131729,-0.270574496756704,
22.5918672333016));
#18724=CARTESIAN_POINT('Ctrl Pts',(-7.48353667075686,-0.00487092690921722,
22.6043481665498));
#18725=CARTESIAN_POINT('Ctrl Pts',(-7.48226341019643,0.26083264293827,22.6168290997979));
#18726=CARTESIAN_POINT('Ctrl Pts',(-7.59019703546702,0.525433154239572,
22.6293100330461));
#18727=CARTESIAN_POINT('Ctrl Pts',(-7.77695120652451,0.714438148392591,
22.6417909662943));
#18728=CARTESIAN_POINT('Ctrl Pts',(-7.963705377582,0.903443142545609,22.6542718995425));
#18729=CARTESIAN_POINT('Ctrl Pts',(-8.22699388814733,1.01453885915634,22.6667528327907));
#18730=CARTESIAN_POINT('Ctrl Pts',(-8.49269364459063,1.01644874085988,22.6792337660389));
#18731=CARTESIAN_POINT('Ctrl Pts',(-8.75839340103394,1.01835862256342,22.6917146992871));
#18732=CARTESIAN_POINT('Ctrl Pts',(-9.02325176140303,0.911059288979473,
22.7041956325353));
#18733=CARTESIAN_POINT('Ctrl Pts',(-9.21270367535774,0.724758509268139,
22.7166765657835));
#18734=CARTESIAN_POINT('Ctrl Pts',(-9.40215558931244,0.538457729556806,
22.7291574990317));
#18735=CARTESIAN_POINT('Ctrl Pts',(-9.51388182535817,0.275436159673239,
22.7416384322798));
#18736=CARTESIAN_POINT('Ctrl Pts',(-9.51642831724056,0.00974174196513924,
22.754119365528));
#18737=CARTESIAN_POINT('Ctrl Pts',(-9.51645943884196,0.00649459406756688,
22.7542718995425));
#18738=CARTESIAN_POINT('Ctrl Pts',(-9.516475,0.00324729703467682,22.754424433557));
#18739=CARTESIAN_POINT('Ctrl Pts',(-9.516475,1.33009890648788E-12,22.7545769675715));
#18740=CARTESIAN_POINT('Origin',(-8.5,0.,1.24542303242842));
#18741=CARTESIAN_POINT('',(-9.51589627264183,0.00088909351918253,22.0954230324284));
#18742=CARTESIAN_POINT('',(-9.51647200958291,-1.63787847398016E-6,22.1545769675715));
#18743=CARTESIAN_POINT('',(-9.516475,1.78524650477582E-12,1.24542303242842));
#18744=CARTESIAN_POINT('Ctrl Pts',(-9.51589627264183,0.000889093519182621,
22.0954230324284));
#18745=CARTESIAN_POINT('Ctrl Pts',(-9.51392442065431,-0.241722873625218,
22.1068093522094));
#18746=CARTESIAN_POINT('Ctrl Pts',(-9.30556868281626,-0.826435388003987,
22.134103013142));
#18747=CARTESIAN_POINT('Ctrl Pts',(-8.3263597217982,-1.1900304846565,22.1773040152262));
#18748=CARTESIAN_POINT('Ctrl Pts',(-7.56086357421315,-0.61293859637056,
22.2170723681052));
#18749=CARTESIAN_POINT('Ctrl Pts',(-7.44608444309555,0.076596244772818,
22.2488870504085));
#18750=CARTESIAN_POINT('Ctrl Pts',(-7.65935850290658,0.742288907720554,
22.2807017327117));
#18751=CARTESIAN_POINT('Ctrl Pts',(-8.50025311474624,1.20263187907136,22.3204700855908));
#18752=CARTESIAN_POINT('Ctrl Pts',(-9.36761503946097,0.728072660225888,
22.3613617423549));
#18753=CARTESIAN_POINT('Ctrl Pts',(-9.51436567791787,0.193492055931185,
22.3863460579675));
#18754=CARTESIAN_POINT('Ctrl Pts',(-9.51493538331909,-0.000390544144346583,
22.3954230324284));
#18755=CARTESIAN_POINT('Ctrl Pts',(-9.51576916465609,-0.000386592347592606,
22.1545769675715));
#18756=CARTESIAN_POINT('Ctrl Pts',(-9.51620747696863,-0.135644650959571,
22.1609140295152));
#18757=CARTESIAN_POINT('Ctrl Pts',(-9.42610449104091,-0.60977881496797,
22.1831584326104));
#18758=CARTESIAN_POINT('Ctrl Pts',(-8.7081020895998,-1.18449019452673,22.2213101768575));
#18759=CARTESIAN_POINT('Ctrl Pts',(-7.61521781807871,-0.814404432911052,
22.2690322003123));
#18760=CARTESIAN_POINT('Ctrl Pts',(-7.33719548426661,0.30316329774476,22.3167542237672));
#18761=CARTESIAN_POINT('Ctrl Pts',(-8.12547601519426,1.14272738419793,22.364476247222));
#18762=CARTESIAN_POINT('Ctrl Pts',(-9.21759447524406,0.939966962847629,
22.4104171618235));
#18763=CARTESIAN_POINT('Ctrl Pts',(-9.51469503156432,0.299302442536928,
22.4404507352733));
#18764=CARTESIAN_POINT('Ctrl Pts',(-9.51711756914169,-0.000632200503468537,
22.4545769675715));
#18765=CARTESIAN_POINT('Origin',(-8.5,0.,1.24542303242842));
#18766=CARTESIAN_POINT('',(-9.51691317747902,3.08906250382967E-5,21.7954230324284));
#18767=CARTESIAN_POINT('',(-9.516475,1.20656969512839E-12,21.8545769675715));
#18768=CARTESIAN_POINT('',(-9.516475,1.78524650477582E-12,1.24542303242842));
#18769=CARTESIAN_POINT('Ctrl Pts',(-9.51824203506389,0.000124572390490018,
21.7954230324284));
#18770=CARTESIAN_POINT('Ctrl Pts',(-9.51824208893095,-0.000615822241855329,
21.7954579641481));
#18771=CARTESIAN_POINT('Ctrl Pts',(-9.5178614904951,-0.338520706650099,
21.8114002370193));
#18772=CARTESIAN_POINT('Ctrl Pts',(-9.14729583240704,-1.01357368058483,
21.8432498510421));
#18773=CARTESIAN_POINT('Ctrl Pts',(-8.19080776710961,-1.07799402237706,
21.8830182039212));
#18774=CARTESIAN_POINT('Ctrl Pts',(-7.65285755162984,-0.63162857595897,
21.9148328862244));
#18775=CARTESIAN_POINT('Ctrl Pts',(-7.37859808588644,0.0113444340040694,
21.9466475685277));
#18776=CARTESIAN_POINT('Ctrl Pts',(-7.71333472266603,0.909659959579857,
21.9864159214067));
#18777=CARTESIAN_POINT('Ctrl Pts',(-8.84120404649836,1.15311486350827,22.0341379448616));
#18778=CARTESIAN_POINT('Ctrl Pts',(-9.45970169651922,0.531555192179094,
22.0704736485355));
#18779=CARTESIAN_POINT('Ctrl Pts',(-9.5166792108648,0.0972199457469021,
22.0909020110578));
#18780=CARTESIAN_POINT('Ctrl Pts',(-9.51589627264183,0.000889093519182621,
22.0954230324284));
#18781=CARTESIAN_POINT('Ctrl Pts',(-9.516475,1.20656969512839E-12,21.8545769675715));
#18782=CARTESIAN_POINT('Ctrl Pts',(-9.51647500000032,-0.265706620582781,
21.8670579008197));
#18783=CARTESIAN_POINT('Ctrl Pts',(-9.40727465387257,-0.529786878176101,
21.8795388340679));
#18784=CARTESIAN_POINT('Ctrl Pts',(-9.21961691907837,-0.717894780174059,
21.892019767316));
#18785=CARTESIAN_POINT('Ctrl Pts',(-9.03195918428417,-0.906002682172016,
21.9045007005642));
#18786=CARTESIAN_POINT('Ctrl Pts',(-8.76814132834463,-1.01583545019887,
21.9169816338124));
#18787=CARTESIAN_POINT('Ctrl Pts',(-8.50243547044586,-1.0164720823066,21.9294625670606));
#18788=CARTESIAN_POINT('Ctrl Pts',(-8.23672961254708,-1.01710871441432,
21.9419435003088));
#18789=CARTESIAN_POINT('Ctrl Pts',(-7.97238846933404,-0.908541417083162,
21.954424433557));
#18790=CARTESIAN_POINT('Ctrl Pts',(-7.78383148002393,-0.721334926799113,
21.9669053668052));
#18791=CARTESIAN_POINT('Ctrl Pts',(-7.59527449071382,-0.534128436515065,
21.9793863000534));
#18792=CARTESIAN_POINT('Ctrl Pts',(-7.48480993131722,-0.270574496756449,
21.9918672333016));
#18793=CARTESIAN_POINT('Ctrl Pts',(-7.48353667075686,-0.00487092690894227,
22.0043481665498));
#18794=CARTESIAN_POINT('Ctrl Pts',(-7.48226341019651,0.260832642938564,
22.016829099798));
#18795=CARTESIAN_POINT('Ctrl Pts',(-7.59019703546717,0.525433154239857,
22.0293100330461));
#18796=CARTESIAN_POINT('Ctrl Pts',(-7.77695120652474,0.714438148392827,
22.0417909662943));
#18797=CARTESIAN_POINT('Ctrl Pts',(-7.96370537758231,0.903443142545798,
22.0542718995425));
#18798=CARTESIAN_POINT('Ctrl Pts',(-8.2269938881477,1.01453885915644,22.0667528327907));
#18799=CARTESIAN_POINT('Ctrl Pts',(-8.49269364459102,1.01644874085988,22.0792337660389));
#18800=CARTESIAN_POINT('Ctrl Pts',(-8.75839340103435,1.01835862256332,22.0917146992871));
#18801=CARTESIAN_POINT('Ctrl Pts',(-9.02325176140342,0.911059288979255,
22.1041956325353));
#18802=CARTESIAN_POINT('Ctrl Pts',(-9.21270367535806,0.724758509267825,
22.1166765657835));
#18803=CARTESIAN_POINT('Ctrl Pts',(-9.4021555893127,0.538457729556394,22.1291574990317));
#18804=CARTESIAN_POINT('Ctrl Pts',(-9.51388182535831,0.275436159672753,
22.1416384322799));
#18805=CARTESIAN_POINT('Ctrl Pts',(-9.51642831724057,0.00974174196463319,
22.1541193655281));
#18806=CARTESIAN_POINT('Ctrl Pts',(-9.51645943884197,0.00649459406721488,
22.1542718995425));
#18807=CARTESIAN_POINT('Ctrl Pts',(-9.516475,0.00324729703447892,22.154424433557));
#18808=CARTESIAN_POINT('Ctrl Pts',(-9.516475,1.28626604170591E-12,22.1545769675715));
#18809=CARTESIAN_POINT('Origin',(-8.5,0.,1.24542303242842));
#18810=CARTESIAN_POINT('',(-9.516475,1.15770944915783E-12,21.4954230324284));
#18811=CARTESIAN_POINT('',(-9.516475,1.1846532627374E-12,21.5545769675715));
#18812=CARTESIAN_POINT('',(-9.516475,1.78524650477582E-12,1.24542303242842));
#18813=CARTESIAN_POINT('Ctrl Pts',(-9.516475,1.21548936334437E-12,21.4954230324284));
#18814=CARTESIAN_POINT('Ctrl Pts',(-9.51647500000032,-0.265706620582753,
21.5079039656766));
#18815=CARTESIAN_POINT('Ctrl Pts',(-9.40727465387259,-0.529786878176055,
21.5203848989248));
#18816=CARTESIAN_POINT('Ctrl Pts',(-9.21961691907841,-0.717894780174012,
21.532865832173));
#18817=CARTESIAN_POINT('Ctrl Pts',(-9.03195918428424,-0.906002682171968,
21.5453467654212));
#18818=CARTESIAN_POINT('Ctrl Pts',(-8.76814132834473,-1.01583545019884,
21.5578276986694));
#18819=CARTESIAN_POINT('Ctrl Pts',(-8.50243547044598,-1.0164720823066,21.5703086319176));
#18820=CARTESIAN_POINT('Ctrl Pts',(-8.23672961254723,-1.01710871441435,
21.5827895651658));
#18821=CARTESIAN_POINT('Ctrl Pts',(-7.97238846933418,-0.908541417083243,
21.595270498414));
#18822=CARTESIAN_POINT('Ctrl Pts',(-7.78383148002406,-0.721334926799242,
21.6077514316622));
#18823=CARTESIAN_POINT('Ctrl Pts',(-7.59527449071393,-0.534128436515241,
21.6202323649103));
#18824=CARTESIAN_POINT('Ctrl Pts',(-7.48480993131728,-0.270574496756669,
21.6327132981585));
#18825=CARTESIAN_POINT('Ctrl Pts',(-7.48353667075686,-0.00487092690918231,
21.6451942314067));
#18826=CARTESIAN_POINT('Ctrl Pts',(-7.48226341019644,0.260832642938305,
21.6576751646549));
#18827=CARTESIAN_POINT('Ctrl Pts',(-7.59019703546703,0.525433154239604,
21.6701560979031));
#18828=CARTESIAN_POINT('Ctrl Pts',(-7.77695120652453,0.714438148392616,
21.6826370311513));
#18829=CARTESIAN_POINT('Ctrl Pts',(-7.96370537758203,0.903443142545627,
21.6951179643995));
#18830=CARTESIAN_POINT('Ctrl Pts',(-8.22699388814736,1.01453885915635,21.7075988976477));
#18831=CARTESIAN_POINT('Ctrl Pts',(-8.49269364459067,1.01644874085988,21.7200798308959));
#18832=CARTESIAN_POINT('Ctrl Pts',(-8.75839340103397,1.01835862256341,21.7325607641441));
#18833=CARTESIAN_POINT('Ctrl Pts',(-9.02325176140306,0.911059288979455,
21.7450416973922));
#18834=CARTESIAN_POINT('Ctrl Pts',(-9.21270367535776,0.724758509268115,
21.7575226306404));
#18835=CARTESIAN_POINT('Ctrl Pts',(-9.40215558931246,0.538457729556775,
21.7700035638886));
#18836=CARTESIAN_POINT('Ctrl Pts',(-9.51388182535818,0.275436159673204,
21.7824844971368));
#18837=CARTESIAN_POINT('Ctrl Pts',(-9.51642831724056,0.00974174196510433,
21.794965430385));
#18838=CARTESIAN_POINT('Ctrl Pts',(-9.51645943884196,0.00649459406749345,
21.7951179643995));
#18839=CARTESIAN_POINT('Ctrl Pts',(-9.516475,0.00324729703456478,21.795270498414));
#18840=CARTESIAN_POINT('Ctrl Pts',(-9.516475,1.17962588154882E-12,21.7954230324284));
#18841=CARTESIAN_POINT('Ctrl Pts',(-9.516475,1.24243317692394E-12,21.5545769675715));
#18842=CARTESIAN_POINT('Ctrl Pts',(-9.51647500000032,-0.265706620582746,
21.5670579008197));
#18843=CARTESIAN_POINT('Ctrl Pts',(-9.40727465387258,-0.529786878176069,
21.5795388340678));
#18844=CARTESIAN_POINT('Ctrl Pts',(-9.21961691907839,-0.717894780174033,
21.592019767316));
#18845=CARTESIAN_POINT('Ctrl Pts',(-9.0319591842842,-0.906002682171997,
21.6045007005642));
#18846=CARTESIAN_POINT('Ctrl Pts',(-8.76814132834467,-1.01583545019886,
21.6169816338124));
#18847=CARTESIAN_POINT('Ctrl Pts',(-8.50243547044589,-1.0164720823066,21.6294625670606));
#18848=CARTESIAN_POINT('Ctrl Pts',(-8.23672961254712,-1.01710871441433,
21.6419435003088));
#18849=CARTESIAN_POINT('Ctrl Pts',(-7.97238846933407,-0.908541417083181,
21.654424433557));
#18850=CARTESIAN_POINT('Ctrl Pts',(-7.78383148002395,-0.721334926799139,
21.6669053668052));
#18851=CARTESIAN_POINT('Ctrl Pts',(-7.59527449071384,-0.534128436515097,
21.6793863000534));
#18852=CARTESIAN_POINT('Ctrl Pts',(-7.48480993131722,-0.270574496756485,
21.6918672333016));
#18853=CARTESIAN_POINT('Ctrl Pts',(-7.48353667075686,-0.00487092690897814,
21.7043481665498));
#18854=CARTESIAN_POINT('Ctrl Pts',(-7.4822634101965,0.260832642938528,21.716829099798));
#18855=CARTESIAN_POINT('Ctrl Pts',(-7.59019703546716,0.525433154239825,
21.7293100330461));
#18856=CARTESIAN_POINT('Ctrl Pts',(-7.77695120652472,0.714438148392802,
21.7417909662943));
#18857=CARTESIAN_POINT('Ctrl Pts',(-7.96370537758228,0.903443142545779,
21.7542718995425));
#18858=CARTESIAN_POINT('Ctrl Pts',(-8.22699388814766,1.01453885915643,21.7667528327907));
#18859=CARTESIAN_POINT('Ctrl Pts',(-8.49269364459099,1.01644874085988,21.7792337660389));
#18860=CARTESIAN_POINT('Ctrl Pts',(-8.75839340103431,1.01835862256333,21.7917146992871));
#18861=CARTESIAN_POINT('Ctrl Pts',(-9.02325176140338,0.911059288979274,
21.8041956325353));
#18862=CARTESIAN_POINT('Ctrl Pts',(-9.21270367535803,0.72475850926785,21.8166765657835));
#18863=CARTESIAN_POINT('Ctrl Pts',(-9.40215558931268,0.538457729556426,
21.8291574990317));
#18864=CARTESIAN_POINT('Ctrl Pts',(-9.5138818253583,0.275436159672789,21.8416384322799));
#18865=CARTESIAN_POINT('Ctrl Pts',(-9.51642831724057,0.00974174196466906,
21.8541193655281));
#18866=CARTESIAN_POINT('Ctrl Pts',(-9.51645943884196,0.00649459406721223,
21.8542718995425));
#18867=CARTESIAN_POINT('Ctrl Pts',(-9.516475,0.00324729703443765,21.854424433557));
#18868=CARTESIAN_POINT('Ctrl Pts',(-9.516475,1.20656969512839E-12,21.8545769675715));
#18869=CARTESIAN_POINT('Origin',(-8.5,0.,1.24542303242842));
#18870=CARTESIAN_POINT('',(-9.51616151751664,0.000104592831971277,21.1954230324285));
#18871=CARTESIAN_POINT('',(-9.516475,1.16273683034641E-12,21.2545769675715));
#18872=CARTESIAN_POINT('',(-9.516475,1.78524650477582E-12,1.24542303242842));
#18873=CARTESIAN_POINT('Ctrl Pts',(-9.516475,1.13579301676685E-12,21.1954230324284));
#18874=CARTESIAN_POINT('Ctrl Pts',(-9.5164750000003,-0.265706620582814,
21.2079039656766));
#18875=CARTESIAN_POINT('Ctrl Pts',(-9.40727465387256,-0.529786878176089,
21.2203848989248));
#18876=CARTESIAN_POINT('Ctrl Pts',(-9.2196169190784,-0.717894780174027,
21.232865832173));
#18877=CARTESIAN_POINT('Ctrl Pts',(-9.03195918428423,-0.906002682171965,
21.2453467654212));
#18878=CARTESIAN_POINT('Ctrl Pts',(-8.76814132834475,-1.01583545019883,
21.2578276986694));
#18879=CARTESIAN_POINT('Ctrl Pts',(-8.50243547044602,-1.0164720823066,21.2703086319176));
#18880=CARTESIAN_POINT('Ctrl Pts',(-8.23672961254728,-1.01710871441436,
21.2827895651658));
#18881=CARTESIAN_POINT('Ctrl Pts',(-7.97238846933425,-0.908541417083278,
21.295270498414));
#18882=CARTESIAN_POINT('Ctrl Pts',(-7.78383148002412,-0.721334926799308,
21.3077514316622));
#18883=CARTESIAN_POINT('Ctrl Pts',(-7.59527449071399,-0.534128436515337,
21.3202323649103));
#18884=CARTESIAN_POINT('Ctrl Pts',(-7.48480993131732,-0.270574496756801,
21.3327132981585));
#18885=CARTESIAN_POINT('Ctrl Pts',(-7.48353667075686,-0.00487092690933373,
21.3451942314067));
#18886=CARTESIAN_POINT('Ctrl Pts',(-7.48226341019641,0.260832642938134,
21.3576751646549));
#18887=CARTESIAN_POINT('Ctrl Pts',(-7.59019703546694,0.52543315423943,21.3701560979031));
#18888=CARTESIAN_POINT('Ctrl Pts',(-7.77695120652438,0.714438148392467,
21.3826370311513));
#18889=CARTESIAN_POINT('Ctrl Pts',(-7.96370537758183,0.903443142545503,
21.3951179643995));
#18890=CARTESIAN_POINT('Ctrl Pts',(-8.22699388814712,1.01453885915627,21.4075988976477));
#18891=CARTESIAN_POINT('Ctrl Pts',(-8.4926936445904,1.01644874085988,21.4200798308959));
#18892=CARTESIAN_POINT('Ctrl Pts',(-8.75839340103369,1.01835862256348,21.432560764144));
#18893=CARTESIAN_POINT('Ctrl Pts',(-9.02325176140278,0.911059288979609,
21.4450416973922));
#18894=CARTESIAN_POINT('Ctrl Pts',(-9.21270367535753,0.724758509268343,
21.4575226306404));
#18895=CARTESIAN_POINT('Ctrl Pts',(-9.40215558931228,0.538457729557076,
21.4700035638886));
#18896=CARTESIAN_POINT('Ctrl Pts',(-9.51388182535807,0.275436159673566,
21.4824844971368));
#18897=CARTESIAN_POINT('Ctrl Pts',(-9.51642831724056,0.00974174196548686,
21.494965430385));
#18898=CARTESIAN_POINT('Ctrl Pts',(-9.51645943884196,0.00649459406776043,
21.4951179643995));
#18899=CARTESIAN_POINT('Ctrl Pts',(-9.516475,0.00324729703471629,21.495270498414));
#18900=CARTESIAN_POINT('Ctrl Pts',(-9.516475,1.21548936334437E-12,21.4954230324284));
#18901=CARTESIAN_POINT('Ctrl Pts',(-9.516475,1.16273683034641E-12,21.2545769675715));
#18902=CARTESIAN_POINT('Ctrl Pts',(-9.5164750000003,-0.265706620582787,
21.2670579008197));
#18903=CARTESIAN_POINT('Ctrl Pts',(-9.40727465387258,-0.529786878176065,
21.2795388340678));
#18904=CARTESIAN_POINT('Ctrl Pts',(-9.21961691907842,-0.717894780174008,
21.292019767316));
#18905=CARTESIAN_POINT('Ctrl Pts',(-9.03195918428426,-0.906002682171951,
21.3045007005642));
#18906=CARTESIAN_POINT('Ctrl Pts',(-8.76814132834478,-1.01583545019882,
21.3169816338124));
#18907=CARTESIAN_POINT('Ctrl Pts',(-8.50243547044604,-1.0164720823066,21.3294625670606));
#18908=CARTESIAN_POINT('Ctrl Pts',(-8.23672961254731,-1.01710871441437,
21.3419435003088));
#18909=CARTESIAN_POINT('Ctrl Pts',(-7.97238846933428,-0.908541417083292,
21.354424433557));
#18910=CARTESIAN_POINT('Ctrl Pts',(-7.78383148002414,-0.721334926799327,
21.3669053668052));
#18911=CARTESIAN_POINT('Ctrl Pts',(-7.59527449071401,-0.534128436515362,
21.3793863000534));
#18912=CARTESIAN_POINT('Ctrl Pts',(-7.48480993131733,-0.270574496756828,
21.3918672333016));
#18913=CARTESIAN_POINT('Ctrl Pts',(-7.48353667075686,-0.00487092690936068,
21.4043481665497));
#18914=CARTESIAN_POINT('Ctrl Pts',(-7.4822634101964,0.260832642938107,21.4168290997979));
#18915=CARTESIAN_POINT('Ctrl Pts',(-7.59019703546693,0.525433154239406,
21.4293100330461));
#18916=CARTESIAN_POINT('Ctrl Pts',(-7.77695120652437,0.714438148392448,
21.4417909662943));
#18917=CARTESIAN_POINT('Ctrl Pts',(-7.96370537758181,0.903443142545489,
21.4542718995425));
#18918=CARTESIAN_POINT('Ctrl Pts',(-8.22699388814709,1.01453885915627,21.4667528327907));
#18919=CARTESIAN_POINT('Ctrl Pts',(-8.49269364459037,1.01644874085988,21.4792337660389));
#18920=CARTESIAN_POINT('Ctrl Pts',(-8.75839340103366,1.01835862256349,21.4917146992871));
#18921=CARTESIAN_POINT('Ctrl Pts',(-9.02325176140276,0.911059288979622,
21.5041956325353));
#18922=CARTESIAN_POINT('Ctrl Pts',(-9.21270367535751,0.724758509268361,
21.5166765657834));
#18923=CARTESIAN_POINT('Ctrl Pts',(-9.40215558931226,0.5384577295571,21.5291574990316));
#18924=CARTESIAN_POINT('Ctrl Pts',(-9.51388182535807,0.275436159673593,
21.5416384322798));
#18925=CARTESIAN_POINT('Ctrl Pts',(-9.51642831724056,0.0097417419655138,
21.554119365528));
#18926=CARTESIAN_POINT('Ctrl Pts',(-9.51645943884196,0.00649459406778737,
21.5542718995425));
#18927=CARTESIAN_POINT('Ctrl Pts',(-9.516475,0.00324729703474323,21.554424433557));
#18928=CARTESIAN_POINT('Ctrl Pts',(-9.516475,1.24243317692394E-12,21.5545769675715));
#18929=CARTESIAN_POINT('Origin',(-8.5,0.,1.24542303242842));
#18930=CARTESIAN_POINT('',(-9.51651008988031,1.86612749551999E-5,20.8954230324284));
#18931=CARTESIAN_POINT('',(-9.51611841008406,4.72824068350965E-5,20.9545769675715));
#18932=CARTESIAN_POINT('',(-9.516475,1.78524650477582E-12,1.24542303242842));
#18933=CARTESIAN_POINT('Ctrl Pts',(-9.51739547620554,0.00048952171884608,
20.8954230324284));
#18934=CARTESIAN_POINT('Ctrl Pts',(-9.51672440796061,-0.121639760734766,
20.9011721528431));
#18935=CARTESIAN_POINT('Ctrl Pts',(-9.46120098978118,-0.413472798869971,
20.9148749438335));
#18936=CARTESIAN_POINT('Ctrl Pts',(-9.0945383169396,-0.950891759797607,
20.9444850759755));
#18937=CARTESIAN_POINT('Ctrl Pts',(-8.1573862740094,-1.15279631131811,20.9842534288547));
#18938=CARTESIAN_POINT('Ctrl Pts',(-7.34469566859739,-0.333715435113531,
21.0319754523094));
#18939=CARTESIAN_POINT('Ctrl Pts',(-7.59486638697568,0.790414745233752,
21.0796974757644));
#18940=CARTESIAN_POINT('Ctrl Pts',(-8.67505328733558,1.18972704280586,21.1274194992192));
#18941=CARTESIAN_POINT('Ctrl Pts',(-9.41959580507824,0.627975166168469,
21.1659946847739));
#18942=CARTESIAN_POINT('Ctrl Pts',(-9.51539910100029,0.144896470838527,
21.188662529177));
#18943=CARTESIAN_POINT('Ctrl Pts',(-9.51472347206447,0.000584393945904427,
21.1954230324284));
#18944=CARTESIAN_POINT('Ctrl Pts',(-9.516475,1.19860031214197E-12,20.9545769675715));
#18945=CARTESIAN_POINT('Ctrl Pts',(-9.51647500000031,-0.26570662058277,
20.9670579008197));
#18946=CARTESIAN_POINT('Ctrl Pts',(-9.40727465387258,-0.529786878176071,
20.9795388340678));
#18947=CARTESIAN_POINT('Ctrl Pts',(-9.2196169190784,-0.717894780174024,
20.992019767316));
#18948=CARTESIAN_POINT('Ctrl Pts',(-9.03195918428422,-0.906002682171976,
21.0045007005642));
#18949=CARTESIAN_POINT('Ctrl Pts',(-8.76814132834472,-1.01583545019884,
21.0169816338124));
#18950=CARTESIAN_POINT('Ctrl Pts',(-8.50243547044597,-1.0164720823066,21.0294625670606));
#18951=CARTESIAN_POINT('Ctrl Pts',(-8.23672961254721,-1.01710871441435,
21.0419435003088));
#18952=CARTESIAN_POINT('Ctrl Pts',(-7.97238846933417,-0.908541417083234,
21.054424433557));
#18953=CARTESIAN_POINT('Ctrl Pts',(-7.78383148002405,-0.72133492679923,
21.0669053668052));
#18954=CARTESIAN_POINT('Ctrl Pts',(-7.59527449071392,-0.534128436515226,
21.0793863000534));
#18955=CARTESIAN_POINT('Ctrl Pts',(-7.48480993131727,-0.270574496756652,
21.0918672333016));
#18956=CARTESIAN_POINT('Ctrl Pts',(-7.48353667075686,-0.00487092690916542,
21.1043481665498));
#18957=CARTESIAN_POINT('Ctrl Pts',(-7.48226341019645,0.260832642938322,
21.1168290997979));
#18958=CARTESIAN_POINT('Ctrl Pts',(-7.59019703546704,0.525433154239619,
21.1293100330461));
#18959=CARTESIAN_POINT('Ctrl Pts',(-7.77695120652454,0.714438148392628,
21.1417909662943));
#18960=CARTESIAN_POINT('Ctrl Pts',(-7.96370537758204,0.903443142545636,
21.1542718995425));
#18961=CARTESIAN_POINT('Ctrl Pts',(-8.22699388814738,1.01453885915635,21.1667528327907));
#18962=CARTESIAN_POINT('Ctrl Pts',(-8.49269364459069,1.01644874085988,21.1792337660389));
#18963=CARTESIAN_POINT('Ctrl Pts',(-8.75839340103399,1.01835862256341,21.1917146992871));
#18964=CARTESIAN_POINT('Ctrl Pts',(-9.02325176140307,0.911059288979446,
21.2041956325353));
#18965=CARTESIAN_POINT('Ctrl Pts',(-9.21270367535777,0.724758509268103,
21.2166765657835));
#18966=CARTESIAN_POINT('Ctrl Pts',(-9.40215558931247,0.53845772955676,21.2291574990317));
#18967=CARTESIAN_POINT('Ctrl Pts',(-9.51388182535818,0.275436159673187,
21.2416384322798));
#18968=CARTESIAN_POINT('Ctrl Pts',(-9.51642831724056,0.00974174196508744,
21.254119365528));
#18969=CARTESIAN_POINT('Ctrl Pts',(-9.51645943884196,0.00649459406747656,
21.2542718995425));
#18970=CARTESIAN_POINT('Ctrl Pts',(-9.516475,0.0032472970345479,21.254424433557));
#18971=CARTESIAN_POINT('Ctrl Pts',(-9.516475,1.16273683034641E-12,21.2545769675715));
#18972=CARTESIAN_POINT('Origin',(-8.5,0.,1.24542303242842));
#18973=CARTESIAN_POINT('',(-9.51649357373598,-1.11249508487427E-5,20.5954230324284));
#18974=CARTESIAN_POINT('',(-9.51648479396161,1.50281475572388E-5,20.6545769675715));
#18975=CARTESIAN_POINT('',(-9.516475,1.78524650477582E-12,1.24542303242842));
#18976=CARTESIAN_POINT('Ctrl Pts',(-9.516475,1.09196015198488E-12,20.5954230324284));
#18977=CARTESIAN_POINT('Ctrl Pts',(-9.51647500000029,-0.265706620582857,
20.6079039656766));
#18978=CARTESIAN_POINT('Ctrl Pts',(-9.40727465387254,-0.529786878176128,
20.6203848989248));
#18979=CARTESIAN_POINT('Ctrl Pts',(-9.21961691907837,-0.717894780174058,
20.632865832173));
#18980=CARTESIAN_POINT('Ctrl Pts',(-9.0319591842842,-0.906002682171989,
20.6453467654212));
#18981=CARTESIAN_POINT('Ctrl Pts',(-8.76814132834471,-1.01583545019884,
20.6578276986694));
#18982=CARTESIAN_POINT('Ctrl Pts',(-8.50243547044597,-1.0164720823066,20.6703086319176));
#18983=CARTESIAN_POINT('Ctrl Pts',(-8.23672961254724,-1.01710871441435,
20.6827895651658));
#18984=CARTESIAN_POINT('Ctrl Pts',(-7.97238846933421,-0.908541417083255,
20.695270498414));
#18985=CARTESIAN_POINT('Ctrl Pts',(-7.78383148002409,-0.721334926799277,
20.7077514316622));
#18986=CARTESIAN_POINT('Ctrl Pts',(-7.59527449071397,-0.534128436515299,
20.7202323649103));
#18987=CARTESIAN_POINT('Ctrl Pts',(-7.48480993131731,-0.270574496756757,
20.7327132981585));
#18988=CARTESIAN_POINT('Ctrl Pts',(-7.48353667075686,-0.0048709269092899,
20.7451942314067));
#18989=CARTESIAN_POINT('Ctrl Pts',(-7.48226341019642,0.260832642938178,
20.7576751646549));
#18990=CARTESIAN_POINT('Ctrl Pts',(-7.59019703546696,0.525433154239469,
20.7701560979031));
#18991=CARTESIAN_POINT('Ctrl Pts',(-7.77695120652442,0.714438148392498,
20.7826370311513));
#18992=CARTESIAN_POINT('Ctrl Pts',(-7.96370537758187,0.903443142545526,
20.7951179643995));
#18993=CARTESIAN_POINT('Ctrl Pts',(-8.22699388814716,1.01453885915629,20.8075988976477));
#18994=CARTESIAN_POINT('Ctrl Pts',(-8.49269364459045,1.01644874085988,20.8200798308959));
#18995=CARTESIAN_POINT('Ctrl Pts',(-8.75839340103373,1.01835862256347,20.832560764144));
#18996=CARTESIAN_POINT('Ctrl Pts',(-9.02325176140282,0.911059288979586,
20.8450416973922));
#18997=CARTESIAN_POINT('Ctrl Pts',(-9.21270367535756,0.724758509268312,
20.8575226306404));
#18998=CARTESIAN_POINT('Ctrl Pts',(-9.4021555893123,0.538457729557038,20.8700035638886));
#18999=CARTESIAN_POINT('Ctrl Pts',(-9.51388182535809,0.275436159673522,
20.8824844971368));
#19000=CARTESIAN_POINT('Ctrl Pts',(-9.51642831724056,0.00974174196544303,
20.894965430385));
#19001=CARTESIAN_POINT('Ctrl Pts',(-9.51645943884196,0.0064945940677166,
20.8951179643995));
#19002=CARTESIAN_POINT('Ctrl Pts',(-9.516475,0.00324729703467245,20.895270498414));
#19003=CARTESIAN_POINT('Ctrl Pts',(-9.516475,1.1716564985624E-12,20.8954230324284));
#19004=CARTESIAN_POINT('Ctrl Pts',(-9.51701410602559,0.000827220438096611,
20.6545769675715));
#19005=CARTESIAN_POINT('Ctrl Pts',(-9.51459385883776,-0.279828092863163,
20.6677864538149));
#19006=CARTESIAN_POINT('Ctrl Pts',(-9.24863288659975,-0.902577123736639,
20.6969032812101));
#19007=CARTESIAN_POINT('Ctrl Pts',(-8.19147423515819,-1.16238347934517,
20.7419274497567));
#19008=CARTESIAN_POINT('Ctrl Pts',(-7.49695823929343,-0.501575692631794,
20.7816958026358));
#19009=CARTESIAN_POINT('Ctrl Pts',(-7.46174696796193,0.196559475127261,
20.813510484939));
#19010=CARTESIAN_POINT('Ctrl Pts',(-7.74971360013524,0.833511408043322,
20.8453251672423));
#19011=CARTESIAN_POINT('Ctrl Pts',(-8.63771535503727,1.19472088021124,20.8850935201213));
#19012=CARTESIAN_POINT('Ctrl Pts',(-9.40914956869547,0.649570193703102,
20.924162010423));
#19013=CARTESIAN_POINT('Ctrl Pts',(-9.5152987801174,0.155174474396472,20.947323159573));
#19014=CARTESIAN_POINT('Ctrl Pts',(-9.51490137801837,0.000208656021816286,
20.9545769675715));
#19015=CARTESIAN_POINT('Origin',(-8.5,0.,1.24542303242842));
#19016=CARTESIAN_POINT('',(-9.5159845430734,-0.000147844677967088,20.2954230324284));
#19017=CARTESIAN_POINT('',(-9.516475,1.09698753317346E-12,20.3545769675715));
#19018=CARTESIAN_POINT('',(-9.516475,1.78524650477582E-12,1.24542303242842));
#19019=CARTESIAN_POINT('Ctrl Pts',(-9.51467624341893,-0.000542222108652152,
20.2954230324284));
#19020=CARTESIAN_POINT('Ctrl Pts',(-9.51530366581787,-0.14800524278466,
20.3023303884478));
#19021=CARTESIAN_POINT('Ctrl Pts',(-9.4166164222524,-0.634321150812596,
20.3251450856188));
#19022=CARTESIAN_POINT('Ctrl Pts',(-8.66406834236317,-1.1912915968917,20.3638671239414));
#19023=CARTESIAN_POINT('Ctrl Pts',(-7.58761183909353,-0.782029520380867,
20.4115891473963));
#19024=CARTESIAN_POINT('Ctrl Pts',(-7.34782400761312,0.344361107498901,
20.4593111708512));
#19025=CARTESIAN_POINT('Ctrl Pts',(-8.16803759563199,1.15590850101208,20.507033194306));
#19026=CARTESIAN_POINT('Ctrl Pts',(-9.10328679193923,0.945365535563934,
20.546801547185));
#19027=CARTESIAN_POINT('Ctrl Pts',(-9.46318133559031,0.407268310575454,
20.5762648265592));
#19028=CARTESIAN_POINT('Ctrl Pts',(-9.51665800623787,0.118514397257793,
20.5898207647817));
#19029=CARTESIAN_POINT('Ctrl Pts',(-9.51733834450537,-0.00051711008067569,
20.5954230324284));
#19030=CARTESIAN_POINT('Ctrl Pts',(-9.516475,1.15476744736E-12,20.3545769675715));
#19031=CARTESIAN_POINT('Ctrl Pts',(-9.5164750000003,-0.265706620582833,
20.3670579008197));
#19032=CARTESIAN_POINT('Ctrl Pts',(-9.40727465387254,-0.529786878176147,
20.3795388340679));
#19033=CARTESIAN_POINT('Ctrl Pts',(-9.21961691907833,-0.717894780174095,
20.392019767316));
#19034=CARTESIAN_POINT('Ctrl Pts',(-9.03195918428412,-0.906002682172043,
20.4045007005642));
#19035=CARTESIAN_POINT('Ctrl Pts',(-8.76814132834458,-1.01583545019888,
20.4169816338124));
#19036=CARTESIAN_POINT('Ctrl Pts',(-8.50243547044581,-1.0164720823066,20.4294625670606));
#19037=CARTESIAN_POINT('Ctrl Pts',(-8.23672961254703,-1.01710871441431,
20.4419435003088));
#19038=CARTESIAN_POINT('Ctrl Pts',(-7.97238846933399,-0.908541417083135,
20.454424433557));
#19039=CARTESIAN_POINT('Ctrl Pts',(-7.78383148002389,-0.721334926799077,
20.4669053668052));
#19040=CARTESIAN_POINT('Ctrl Pts',(-7.59527449071379,-0.534128436515019,
20.4793863000534));
#19041=CARTESIAN_POINT('Ctrl Pts',(-7.4848099313172,-0.270574496756397,
20.4918672333016));
#19042=CARTESIAN_POINT('Ctrl Pts',(-7.48353667075686,-0.00487092690889047,
20.5043481665498));
#19043=CARTESIAN_POINT('Ctrl Pts',(-7.48226341019652,0.260832642938616,
20.516829099798));
#19044=CARTESIAN_POINT('Ctrl Pts',(-7.5901970354672,0.525433154239903,20.5293100330461));
#19045=CARTESIAN_POINT('Ctrl Pts',(-7.77695120652478,0.714438148392864,
20.5417909662943));
#19046=CARTESIAN_POINT('Ctrl Pts',(-7.96370537758235,0.903443142545826,
20.5542718995425));
#19047=CARTESIAN_POINT('Ctrl Pts',(-8.22699388814775,1.01453885915645,20.5667528327907));
#19048=CARTESIAN_POINT('Ctrl Pts',(-8.49269364459108,1.01644874085988,20.5792337660389));
#19049=CARTESIAN_POINT('Ctrl Pts',(-8.7583934010344,1.01835862256331,20.5917146992871));
#19050=CARTESIAN_POINT('Ctrl Pts',(-9.02325176140346,0.911059288979229,
20.6041956325353));
#19051=CARTESIAN_POINT('Ctrl Pts',(-9.21270367535809,0.724758509267789,
20.6166765657835));
#19052=CARTESIAN_POINT('Ctrl Pts',(-9.40215558931272,0.538457729556348,
20.6291574990317));
#19053=CARTESIAN_POINT('Ctrl Pts',(-9.51388182535832,0.275436159672701,
20.6416384322799));
#19054=CARTESIAN_POINT('Ctrl Pts',(-9.51642831724057,0.0097417419645814,
20.6541193655281));
#19055=CARTESIAN_POINT('Ctrl Pts',(-9.51645943884197,0.00649459406712457,
20.6542718995425));
#19056=CARTESIAN_POINT('Ctrl Pts',(-9.516475,0.00324729703434999,20.654424433557));
#19057=CARTESIAN_POINT('Ctrl Pts',(-9.516475,1.11890396556444E-12,20.6545769675715));
#19058=CARTESIAN_POINT('Origin',(-8.5,0.,1.24542303242842));
#19059=CARTESIAN_POINT('',(-9.516475,1.04812728720291E-12,19.9954230324285));
#19060=CARTESIAN_POINT('',(-9.516475,1.07507110078247E-12,20.0545769675715));
#19061=CARTESIAN_POINT('',(-9.516475,1.78524650477582E-12,1.24542303242842));
#19062=CARTESIAN_POINT('Ctrl Pts',(-9.516475,1.04812728720291E-12,19.9954230324285));
#19063=CARTESIAN_POINT('Ctrl Pts',(-9.51647500000027,-0.26570662058294,
20.0079039656766));
#19064=CARTESIAN_POINT('Ctrl Pts',(-9.40727465387248,-0.529786878176243,
20.0203848989248));
#19065=CARTESIAN_POINT('Ctrl Pts',(-9.21961691907825,-0.717894780174171,
20.032865832173));
#19066=CARTESIAN_POINT('Ctrl Pts',(-9.03195918428402,-0.906002682172099,
20.0453467654212));
#19067=CARTESIAN_POINT('Ctrl Pts',(-8.76814132834447,-1.01583545019891,
20.0578276986694));
#19068=CARTESIAN_POINT('Ctrl Pts',(-8.5024354704457,-1.0164720823066,20.0703086319176));
#19069=CARTESIAN_POINT('Ctrl Pts',(-8.23672961254693,-1.01710871441428,
20.0827895651658));
#19070=CARTESIAN_POINT('Ctrl Pts',(-7.97238846933389,-0.90854141708308,
20.095270498414));
#19071=CARTESIAN_POINT('Ctrl Pts',(-7.78383148002382,-0.721334926799002,
20.1077514316622));
#19072=CARTESIAN_POINT('Ctrl Pts',(-7.59527449071374,-0.534128436514924,
20.1202323649104));
#19073=CARTESIAN_POINT('Ctrl Pts',(-7.48480993131717,-0.270574496756291,
20.1327132981586));
#19074=CARTESIAN_POINT('Ctrl Pts',(-7.48353667075686,-0.00487092690878383,
20.1451942314067));
#19075=CARTESIAN_POINT('Ctrl Pts',(-7.48226341019655,0.260832642938723,
20.1576751646549));
#19076=CARTESIAN_POINT('Ctrl Pts',(-7.59019703546726,0.525433154239998,
20.1701560979031));
#19077=CARTESIAN_POINT('Ctrl Pts',(-7.77695120652485,0.71443814839294,20.1826370311513));
#19078=CARTESIAN_POINT('Ctrl Pts',(-7.96370537758245,0.903443142545882,
20.1951179643995));
#19079=CARTESIAN_POINT('Ctrl Pts',(-8.22699388814786,1.01453885915648,20.2075988976477));
#19080=CARTESIAN_POINT('Ctrl Pts',(-8.49269364459118,1.01644874085988,20.2200798308959));
#19081=CARTESIAN_POINT('Ctrl Pts',(-8.75839340103451,1.01835862256328,20.2325607641441));
#19082=CARTESIAN_POINT('Ctrl Pts',(-9.02325176140356,0.911059288979174,
20.2450416973923));
#19083=CARTESIAN_POINT('Ctrl Pts',(-9.21270367535817,0.724758509267714,
20.2575226306405));
#19084=CARTESIAN_POINT('Ctrl Pts',(-9.40215558931278,0.538457729556254,
20.2700035638887));
#19085=CARTESIAN_POINT('Ctrl Pts',(-9.51388182535835,0.275436159672595,
20.2824844971369));
#19086=CARTESIAN_POINT('Ctrl Pts',(-9.51642831724057,0.00974174196447476,
20.294965430385));
#19087=CARTESIAN_POINT('Ctrl Pts',(-9.51645943884197,0.00649459406705645,
20.2951179643995));
#19088=CARTESIAN_POINT('Ctrl Pts',(-9.516475,0.00324729703432047,20.295270498414));
#19089=CARTESIAN_POINT('Ctrl Pts',(-9.516475,1.12782363378043E-12,20.2954230324284));
#19090=CARTESIAN_POINT('Ctrl Pts',(-9.516475,1.07507110078247E-12,20.0545769675715));
#19091=CARTESIAN_POINT('Ctrl Pts',(-9.51647500000028,-0.265706620582874,
20.0670579008197));
#19092=CARTESIAN_POINT('Ctrl Pts',(-9.40727465387253,-0.529786878176143,
20.0795388340679));
#19093=CARTESIAN_POINT('Ctrl Pts',(-9.21961691907836,-0.71789478017407,
20.092019767316));
#19094=CARTESIAN_POINT('Ctrl Pts',(-9.03195918428418,-0.906002682171997,
20.1045007005642));
#19095=CARTESIAN_POINT('Ctrl Pts',(-8.76814132834469,-1.01583545019884,
20.1169816338124));
#19096=CARTESIAN_POINT('Ctrl Pts',(-8.50243547044596,-1.0164720823066,20.1294625670606));
#19097=CARTESIAN_POINT('Ctrl Pts',(-8.23672961254722,-1.01710871441435,
20.1419435003088));
#19098=CARTESIAN_POINT('Ctrl Pts',(-7.9723884693342,-0.908541417083247,
20.154424433557));
#19099=CARTESIAN_POINT('Ctrl Pts',(-7.78383148002408,-0.721334926799265,
20.1669053668052));
#19100=CARTESIAN_POINT('Ctrl Pts',(-7.59527449071396,-0.534128436515283,
20.1793863000534));
#19101=CARTESIAN_POINT('Ctrl Pts',(-7.4848099313173,-0.270574496756741,
20.1918672333016));
#19102=CARTESIAN_POINT('Ctrl Pts',(-7.48353667075686,-0.00487092690927301,
20.2043481665497));
#19103=CARTESIAN_POINT('Ctrl Pts',(-7.48226341019642,0.260832642938195,
20.2168290997979));
#19104=CARTESIAN_POINT('Ctrl Pts',(-7.59019703546697,0.525433154239485,
20.2293100330461));
#19105=CARTESIAN_POINT('Ctrl Pts',(-7.77695120652443,0.71443814839251,20.2417909662943));
#19106=CARTESIAN_POINT('Ctrl Pts',(-7.96370537758188,0.903443142545535,
20.2542718995425));
#19107=CARTESIAN_POINT('Ctrl Pts',(-8.22699388814718,1.01453885915629,20.2667528327907));
#19108=CARTESIAN_POINT('Ctrl Pts',(-8.49269364459046,1.01644874085988,20.2792337660389));
#19109=CARTESIAN_POINT('Ctrl Pts',(-8.75839340103375,1.01835862256346,20.2917146992871));
#19110=CARTESIAN_POINT('Ctrl Pts',(-9.02325176140284,0.911059288979577,
20.3041956325353));
#19111=CARTESIAN_POINT('Ctrl Pts',(-9.21270367535757,0.7247585092683,20.3166765657835));
#19112=CARTESIAN_POINT('Ctrl Pts',(-9.40215558931231,0.538457729557023,
20.3291574990316));
#19113=CARTESIAN_POINT('Ctrl Pts',(-9.51388182535809,0.275436159673506,
20.3416384322798));
#19114=CARTESIAN_POINT('Ctrl Pts',(-9.51642831724056,0.00974174196542614,
20.354119365528));
#19115=CARTESIAN_POINT('Ctrl Pts',(-9.51645943884196,0.00649459406769971,
20.3542718995425));
#19116=CARTESIAN_POINT('Ctrl Pts',(-9.516475,0.00324729703465556,20.354424433557));
#19117=CARTESIAN_POINT('Ctrl Pts',(-9.516475,1.15476744736E-12,20.3545769675715));
#19118=CARTESIAN_POINT('Origin',(-8.5,0.,1.24542303242842));
#19119=CARTESIAN_POINT('',(-9.51688744271748,-4.25820637274689E-5,19.6954230324284));
#19120=CARTESIAN_POINT('',(-9.516475,1.05315466839149E-12,19.7545769675715));
#19121=CARTESIAN_POINT('',(-9.516475,1.78524650477582E-12,1.24542303242842));
#19122=CARTESIAN_POINT('Ctrl Pts',(-9.516475,1.02621085481192E-12,19.6954230324285));
#19123=CARTESIAN_POINT('Ctrl Pts',(-9.51647500000027,-0.265706620582943,
19.7079039656766));
#19124=CARTESIAN_POINT('Ctrl Pts',(-9.40727465387249,-0.529786878176224,
19.7203848989248));
#19125=CARTESIAN_POINT('Ctrl Pts',(-9.21961691907828,-0.717894780174146,
19.732865832173));
#19126=CARTESIAN_POINT('Ctrl Pts',(-9.03195918428407,-0.906002682172067,
19.7453467654212));
#19127=CARTESIAN_POINT('Ctrl Pts',(-8.76814132834455,-1.01583545019889,
19.7578276986694));
#19128=CARTESIAN_POINT('Ctrl Pts',(-8.50243547044579,-1.0164720823066,19.7703086319176));
#19129=CARTESIAN_POINT('Ctrl Pts',(-8.23672961254704,-1.01710871441431,
19.7827895651658));
#19130=CARTESIAN_POINT('Ctrl Pts',(-7.97238846933401,-0.908541417083145,
19.795270498414));
#19131=CARTESIAN_POINT('Ctrl Pts',(-7.78383148002392,-0.721334926799108,
19.8077514316622));
#19132=CARTESIAN_POINT('Ctrl Pts',(-7.59527449071383,-0.534128436515072,
19.8202323649104));
#19133=CARTESIAN_POINT('Ctrl Pts',(-7.48480993131723,-0.27057449675648,
19.8327132981585));
#19134=CARTESIAN_POINT('Ctrl Pts',(-7.48353667075686,-0.00487092690899303,
19.8451942314067));
#19135=CARTESIAN_POINT('Ctrl Pts',(-7.48226341019649,0.260832642938494,
19.8576751646549));
#19136=CARTESIAN_POINT('Ctrl Pts',(-7.59019703546713,0.525433154239773,
19.8701560979031));
#19137=CARTESIAN_POINT('Ctrl Pts',(-7.77695120652466,0.71443814839275,19.8826370311513));
#19138=CARTESIAN_POINT('Ctrl Pts',(-7.9637053775822,0.903443142545727,19.8951179643995));
#19139=CARTESIAN_POINT('Ctrl Pts',(-8.22699388814755,1.0145388591564,19.9075988976477));
#19140=CARTESIAN_POINT('Ctrl Pts',(-8.49269364459086,1.01644874085988,19.9200798308959));
#19141=CARTESIAN_POINT('Ctrl Pts',(-8.75839340103416,1.01835862256336,19.9325607641441));
#19142=CARTESIAN_POINT('Ctrl Pts',(-9.02325176140323,0.911059288979357,
19.9450416973923));
#19143=CARTESIAN_POINT('Ctrl Pts',(-9.2127036753579,0.724758509267982,19.9575226306405));
#19144=CARTESIAN_POINT('Ctrl Pts',(-9.40215558931256,0.538457729556607,
19.9700035638886));
#19145=CARTESIAN_POINT('Ctrl Pts',(-9.51388182535823,0.275436159673015,
19.9824844971368));
#19146=CARTESIAN_POINT('Ctrl Pts',(-9.51642831724057,0.00974174196491506,
19.994965430385));
#19147=CARTESIAN_POINT('Ctrl Pts',(-9.51645943884196,0.00649459406732343,
19.9951179643995));
#19148=CARTESIAN_POINT('Ctrl Pts',(-9.516475,0.00324729703441407,19.995270498414));
#19149=CARTESIAN_POINT('Ctrl Pts',(-9.516475,1.04812728720291E-12,19.9954230324285));
#19150=CARTESIAN_POINT('Ctrl Pts',(-9.516475,1.11093458257803E-12,19.7545769675715));
#19151=CARTESIAN_POINT('Ctrl Pts',(-9.51647500000029,-0.265706620582858,
19.7670579008197));
#19152=CARTESIAN_POINT('Ctrl Pts',(-9.40727465387253,-0.529786878176149,
19.7795388340678));
#19153=CARTESIAN_POINT('Ctrl Pts',(-9.21961691907834,-0.717894780174086,
19.792019767316));
#19154=CARTESIAN_POINT('Ctrl Pts',(-9.03195918428415,-0.906002682172022,
19.8045007005642));
#19155=CARTESIAN_POINT('Ctrl Pts',(-8.76814132834463,-1.01583545019886,
19.8169816338124));
#19156=CARTESIAN_POINT('Ctrl Pts',(-8.50243547044588,-1.0164720823066,19.8294625670606));
#19157=CARTESIAN_POINT('Ctrl Pts',(-8.23672961254712,-1.01710871441433,
19.8419435003088));
#19158=CARTESIAN_POINT('Ctrl Pts',(-7.97238846933409,-0.908541417083189,
19.854424433557));
#19159=CARTESIAN_POINT('Ctrl Pts',(-7.78383148002398,-0.721334926799168,
19.8669053668052));
#19160=CARTESIAN_POINT('Ctrl Pts',(-7.59527449071388,-0.534128436515148,
19.8793863000534));
#19161=CARTESIAN_POINT('Ctrl Pts',(-7.48480993131725,-0.270574496756565,
19.8918672333016));
#19162=CARTESIAN_POINT('Ctrl Pts',(-7.48353667075686,-0.00487092690907776,
19.9043481665498));
#19163=CARTESIAN_POINT('Ctrl Pts',(-7.48226341019647,0.260832642938409,
19.9168290997979));
#19164=CARTESIAN_POINT('Ctrl Pts',(-7.59019703546709,0.525433154239697,
19.9293100330461));
#19165=CARTESIAN_POINT('Ctrl Pts',(-7.7769512065246,0.71443814839269,19.9417909662943));
#19166=CARTESIAN_POINT('Ctrl Pts',(-7.96370537758212,0.903443142545683,
19.9542718995425));
#19167=CARTESIAN_POINT('Ctrl Pts',(-8.22699388814747,1.01453885915637,19.9667528327907));
#19168=CARTESIAN_POINT('Ctrl Pts',(-8.49269364459077,1.01644874085988,19.9792337660389));
#19169=CARTESIAN_POINT('Ctrl Pts',(-8.75839340103408,1.01835862256338,19.9917146992871));
#19170=CARTESIAN_POINT('Ctrl Pts',(-9.02325176140315,0.911059288979401,
20.0041956325353));
#19171=CARTESIAN_POINT('Ctrl Pts',(-9.21270367535783,0.724758509268041,
20.0166765657835));
#19172=CARTESIAN_POINT('Ctrl Pts',(-9.40215558931252,0.538457729556682,
20.0291574990317));
#19173=CARTESIAN_POINT('Ctrl Pts',(-9.51388182535821,0.2754361596731,20.0416384322798));
#19174=CARTESIAN_POINT('Ctrl Pts',(-9.51642831724057,0.00974174196499978,
20.054119365528));
#19175=CARTESIAN_POINT('Ctrl Pts',(-9.51645943884196,0.00649459406738889,
20.0542718995425));
#19176=CARTESIAN_POINT('Ctrl Pts',(-9.516475,0.00324729703446023,20.054424433557));
#19177=CARTESIAN_POINT('Ctrl Pts',(-9.516475,1.07507110078247E-12,20.0545769675715));
#19178=CARTESIAN_POINT('Origin',(-8.5,0.,1.24542303242842));
#19179=CARTESIAN_POINT('',(-9.51581279021529,-0.000874295316650707,19.3954230324285));
#19180=CARTESIAN_POINT('',(-9.516475,1.0312382360005E-12,19.4545769675715));
#19181=CARTESIAN_POINT('',(-9.516475,1.78524650477582E-12,1.24542303242842));
#19182=CARTESIAN_POINT('Ctrl Pts',(-9.51581279021529,-0.000874295316650814,
19.3954230324285));
#19183=CARTESIAN_POINT('Ctrl Pts',(-9.51660067785675,-0.100355318467702,
19.400090906567));
#19184=CARTESIAN_POINT('Ctrl Pts',(-9.45727900114472,-0.537898740061842,
19.4206661218572));
#19185=CARTESIAN_POINT('Ctrl Pts',(-8.83054984563462,-1.15621403266934,
19.457148678299));
#19186=CARTESIAN_POINT('Ctrl Pts',(-7.704974867994,-0.902362754165209,19.5048707017539));
#19187=CARTESIAN_POINT('Ctrl Pts',(-7.37854114860306,-0.000996887084833204,
19.5446390546329));
#19188=CARTESIAN_POINT('Ctrl Pts',(-7.65872158751808,0.639418187488004,
19.5764537369362));
#19189=CARTESIAN_POINT('Ctrl Pts',(-8.20076747273577,1.0808010195163,19.6082684192394));
#19190=CARTESIAN_POINT('Ctrl Pts',(-9.15393034110275,1.00776412933077,19.6479248510702));
#19191=CARTESIAN_POINT('Ctrl Pts',(-9.51797663774671,0.334619188771371,
19.6796276123251));
#19192=CARTESIAN_POINT('Ctrl Pts',(-9.51823730103989,-0.000181946276152444,
19.6954230324284));
#19193=CARTESIAN_POINT('Ctrl Pts',(-9.516475,1.0312382360005E-12,19.4545769675715));
#19194=CARTESIAN_POINT('Ctrl Pts',(-9.51647500000027,-0.265706620582918,
19.4670579008197));
#19195=CARTESIAN_POINT('Ctrl Pts',(-9.40727465387251,-0.529786878176182,
19.4795388340679));
#19196=CARTESIAN_POINT('Ctrl Pts',(-9.21961691907832,-0.717894780174101,
19.492019767316));
#19197=CARTESIAN_POINT('Ctrl Pts',(-9.03195918428414,-0.90600268217202,
19.5045007005642));
#19198=CARTESIAN_POINT('Ctrl Pts',(-8.76814132834465,-1.01583545019886,
19.5169816338124));
#19199=CARTESIAN_POINT('Ctrl Pts',(-8.50243547044591,-1.0164720823066,19.5294625670606));
#19200=CARTESIAN_POINT('Ctrl Pts',(-8.23672961254718,-1.01710871441434,
19.5419435003088));
#19201=CARTESIAN_POINT('Ctrl Pts',(-7.97238846933416,-0.908541417083224,
19.554424433557));
#19202=CARTESIAN_POINT('Ctrl Pts',(-7.78383148002405,-0.721334926799234,
19.5669053668052));
#19203=CARTESIAN_POINT('Ctrl Pts',(-7.59527449071394,-0.534128436515244,
19.5793863000534));
#19204=CARTESIAN_POINT('Ctrl Pts',(-7.48480993131729,-0.270574496756697,
19.5918672333016));
#19205=CARTESIAN_POINT('Ctrl Pts',(-7.48353667075686,-0.00487092690922918,
19.6043481665498));
#19206=CARTESIAN_POINT('Ctrl Pts',(-7.48226341019643,0.260832642938238,
19.6168290997979));
#19207=CARTESIAN_POINT('Ctrl Pts',(-7.59019703546699,0.525433154239524,
19.6293100330461));
#19208=CARTESIAN_POINT('Ctrl Pts',(-7.77695120652446,0.714438148392541,
19.6417909662943));
#19209=CARTESIAN_POINT('Ctrl Pts',(-7.96370537758192,0.903443142545558,
19.6542718995425));
#19210=CARTESIAN_POINT('Ctrl Pts',(-8.22699388814722,1.0145388591563,19.6667528327907));
#19211=CARTESIAN_POINT('Ctrl Pts',(-8.49269364459051,1.01644874085988,19.6792337660389));
#19212=CARTESIAN_POINT('Ctrl Pts',(-8.75839340103379,1.01835862256345,19.6917146992871));
#19213=CARTESIAN_POINT('Ctrl Pts',(-9.02325176140288,0.911059288979555,
19.7041956325353));
#19214=CARTESIAN_POINT('Ctrl Pts',(-9.2127036753576,0.724758509268269,19.7166765657835));
#19215=CARTESIAN_POINT('Ctrl Pts',(-9.40215558931233,0.538457729556984,
19.7291574990316));
#19216=CARTESIAN_POINT('Ctrl Pts',(-9.5138818253581,0.275436159673462,19.7416384322798));
#19217=CARTESIAN_POINT('Ctrl Pts',(-9.51642831724056,0.00974174196538231,
19.754119365528));
#19218=CARTESIAN_POINT('Ctrl Pts',(-9.51645943884196,0.00649459406765588,
19.7542718995425));
#19219=CARTESIAN_POINT('Ctrl Pts',(-9.516475,0.00324729703461173,19.754424433557));
#19220=CARTESIAN_POINT('Ctrl Pts',(-9.516475,1.11093458257803E-12,19.7545769675715));
#19221=CARTESIAN_POINT('Origin',(-8.5,0.,1.24542303242842));
#19222=CARTESIAN_POINT('',(-9.51601270277673,0.000133638117392702,19.0954230324284));
#19223=CARTESIAN_POINT('',(-9.516475,1.00932180360952E-12,19.1545769675715));
#19224=CARTESIAN_POINT('',(-9.516475,1.78524650477582E-12,1.24542303242842));
#19225=CARTESIAN_POINT('Ctrl Pts',(-9.51496883034704,0.000435394516211426,
19.0954230324284));
#19226=CARTESIAN_POINT('Ctrl Pts',(-9.51430705793103,-0.196566568372251,
19.1046468596573));
#19227=CARTESIAN_POINT('Ctrl Pts',(-9.36399077096857,-0.734371610655675,
19.1297780280378));
#19228=CARTESIAN_POINT('Ctrl Pts',(-8.48915653915779,-1.20258301999602,
19.1708165375699));
#19229=CARTESIAN_POINT('Ctrl Pts',(-7.65254526199483,-0.734500793868192,
19.2105848904489));
#19230=CARTESIAN_POINT('Ctrl Pts',(-7.44542256102972,-0.0668686100755817,
19.2423995727522));
#19231=CARTESIAN_POINT('Ctrl Pts',(-7.56655907558636,0.621577822794718,
19.2742142550554));
#19232=CARTESIAN_POINT('Ctrl Pts',(-8.33734740644836,1.19158198813036,19.3139826079345));
#19233=CARTESIAN_POINT('Ctrl Pts',(-9.3098427577801,0.820233931165877,19.3570367572507));
#19234=CARTESIAN_POINT('Ctrl Pts',(-9.51391568740291,0.238659514922684,
19.3841835654154));
#19235=CARTESIAN_POINT('Ctrl Pts',(-9.51581279021529,-0.000874295316650814,
19.3954230324285));
#19236=CARTESIAN_POINT('Ctrl Pts',(-9.516475,1.06710171779606E-12,19.1545769675715));
#19237=CARTESIAN_POINT('Ctrl Pts',(-9.51647500000028,-0.265706620582902,
19.1670579008197));
#19238=CARTESIAN_POINT('Ctrl Pts',(-9.40727465387251,-0.529786878176188,
19.1795388340679));
#19239=CARTESIAN_POINT('Ctrl Pts',(-9.21961691907831,-0.717894780174117,
19.192019767316));
#19240=CARTESIAN_POINT('Ctrl Pts',(-9.03195918428411,-0.906002682172045,
19.2045007005642));
#19241=CARTESIAN_POINT('Ctrl Pts',(-8.76814132834459,-1.01583545019888,
19.2169816338124));
#19242=CARTESIAN_POINT('Ctrl Pts',(-8.50243547044583,-1.0164720823066,19.2294625670606));
#19243=CARTESIAN_POINT('Ctrl Pts',(-8.23672961254708,-1.01710871441432,
19.2419435003088));
#19244=CARTESIAN_POINT('Ctrl Pts',(-7.97238846933405,-0.908541417083166,
19.254424433557));
#19245=CARTESIAN_POINT('Ctrl Pts',(-7.78383148002395,-0.721334926799137,
19.2669053668052));
#19246=CARTESIAN_POINT('Ctrl Pts',(-7.59527449071385,-0.534128436515108,
19.2793863000534));
#19247=CARTESIAN_POINT('Ctrl Pts',(-7.48480993131724,-0.270574496756521,
19.2918672333016));
#19248=CARTESIAN_POINT('Ctrl Pts',(-7.48353667075686,-0.00487092690903392,
19.3043481665498));
#19249=CARTESIAN_POINT('Ctrl Pts',(-7.48226341019648,0.260832642938453,
19.3168290997979));
#19250=CARTESIAN_POINT('Ctrl Pts',(-7.59019703546711,0.525433154239737,
19.3293100330461));
#19251=CARTESIAN_POINT('Ctrl Pts',(-7.77695120652464,0.714438148392721,
19.3417909662943));
#19252=CARTESIAN_POINT('Ctrl Pts',(-7.96370537758216,0.903443142545706,
19.3542718995425));
#19253=CARTESIAN_POINT('Ctrl Pts',(-8.22699388814751,1.01453885915638,19.3667528327907));
#19254=CARTESIAN_POINT('Ctrl Pts',(-8.49269364459082,1.01644874085988,19.3792337660389));
#19255=CARTESIAN_POINT('Ctrl Pts',(-8.75839340103412,1.01835862256337,19.3917146992871));
#19256=CARTESIAN_POINT('Ctrl Pts',(-9.02325176140319,0.911059288979378,
19.4041956325353));
#19257=CARTESIAN_POINT('Ctrl Pts',(-9.21270367535787,0.724758509268011,
19.4166765657835));
#19258=CARTESIAN_POINT('Ctrl Pts',(-9.40215558931254,0.538457729556643,
19.4291574990317));
#19259=CARTESIAN_POINT('Ctrl Pts',(-9.51388182535822,0.275436159673056,
19.4416384322799));
#19260=CARTESIAN_POINT('Ctrl Pts',(-9.51642831724057,0.00974174196495595,
19.454119365528));
#19261=CARTESIAN_POINT('Ctrl Pts',(-9.51645943884196,0.00649459406734506,
19.4542718995425));
#19262=CARTESIAN_POINT('Ctrl Pts',(-9.516475,0.0032472970344164,19.454424433557));
#19263=CARTESIAN_POINT('Ctrl Pts',(-9.516475,1.0312382360005E-12,19.4545769675715));
#19264=CARTESIAN_POINT('Origin',(-8.5,0.,1.24542303242842));
#19265=CARTESIAN_POINT('',(-9.516475,9.60461557638968E-13,18.7954230324285));
#19266=CARTESIAN_POINT('',(-9.516475,9.87405371218534E-13,18.8545769675715));
#19267=CARTESIAN_POINT('',(-9.516475,1.78524650477582E-12,1.24542303242842));
#19268=CARTESIAN_POINT('Ctrl Pts',(-9.516475,1.01824147182551E-12,18.7954230324285));
#19269=CARTESIAN_POINT('Ctrl Pts',(-9.51647500000027,-0.265706620582951,
18.8079039656766));
#19270=CARTESIAN_POINT('Ctrl Pts',(-9.40727465387248,-0.529786878176232,
18.8203848989248));
#19271=CARTESIAN_POINT('Ctrl Pts',(-9.21961691907827,-0.717894780174151,
18.832865832173));
#19272=CARTESIAN_POINT('Ctrl Pts',(-9.03195918428406,-0.906002682172071,
18.8453467654212));
#19273=CARTESIAN_POINT('Ctrl Pts',(-8.76814132834454,-1.01583545019889,
18.8578276986694));
#19274=CARTESIAN_POINT('Ctrl Pts',(-8.50243547044578,-1.0164720823066,18.8703086319176));
#19275=CARTESIAN_POINT('Ctrl Pts',(-8.23672961254703,-1.0171087144143,18.8827895651658));
#19276=CARTESIAN_POINT('Ctrl Pts',(-7.97238846933401,-0.908541417083141,
18.895270498414));
#19277=CARTESIAN_POINT('Ctrl Pts',(-7.78383148002392,-0.721334926799103,
18.9077514316622));
#19278=CARTESIAN_POINT('Ctrl Pts',(-7.59527449071383,-0.534128436515065,
18.9202323649104));
#19279=CARTESIAN_POINT('Ctrl Pts',(-7.48480993131723,-0.270574496756472,
18.9327132981585));
#19280=CARTESIAN_POINT('Ctrl Pts',(-7.48353667075686,-0.00487092690898506,
18.9451942314067));
#19281=CARTESIAN_POINT('Ctrl Pts',(-7.4822634101965,0.260832642938502,18.9576751646549));
#19282=CARTESIAN_POINT('Ctrl Pts',(-7.59019703546714,0.52543315423978,18.9701560979031));
#19283=CARTESIAN_POINT('Ctrl Pts',(-7.77695120652467,0.714438148392756,
18.9826370311513));
#19284=CARTESIAN_POINT('Ctrl Pts',(-7.9637053775822,0.903443142545731,18.9951179643995));
#19285=CARTESIAN_POINT('Ctrl Pts',(-8.22699388814756,1.0145388591564,19.0075988976477));
#19286=CARTESIAN_POINT('Ctrl Pts',(-8.49269364459087,1.01644874085988,19.0200798308959));
#19287=CARTESIAN_POINT('Ctrl Pts',(-8.75839340103417,1.01835862256336,19.0325607641441));
#19288=CARTESIAN_POINT('Ctrl Pts',(-9.02325176140323,0.911059288979353,
19.0450416973923));
#19289=CARTESIAN_POINT('Ctrl Pts',(-9.2127036753579,0.724758509267977,19.0575226306405));
#19290=CARTESIAN_POINT('Ctrl Pts',(-9.40215558931257,0.5384577295566,19.0700035638886));
#19291=CARTESIAN_POINT('Ctrl Pts',(-9.51388182535823,0.275436159673007,
19.0824844971368));
#19292=CARTESIAN_POINT('Ctrl Pts',(-9.51642831724057,0.00974174196490709,
19.094965430385));
#19293=CARTESIAN_POINT('Ctrl Pts',(-9.51645943884196,0.0064945940672962,
19.0951179643995));
#19294=CARTESIAN_POINT('Ctrl Pts',(-9.516475,0.00324729703436754,19.095270498414));
#19295=CARTESIAN_POINT('Ctrl Pts',(-9.516475,9.82377990029953E-13,19.0954230324285));
#19296=CARTESIAN_POINT('Ctrl Pts',(-9.516475,9.87405371218534E-13,18.8545769675715));
#19297=CARTESIAN_POINT('Ctrl Pts',(-9.51647500000026,-0.26570662058302,
18.8670579008197));
#19298=CARTESIAN_POINT('Ctrl Pts',(-9.40727465387243,-0.529786878176335,
18.8795388340679));
#19299=CARTESIAN_POINT('Ctrl Pts',(-9.21961691907817,-0.717894780174255,
18.8920197673161));
#19300=CARTESIAN_POINT('Ctrl Pts',(-9.03195918428391,-0.906002682172175,
18.9045007005642));
#19301=CARTESIAN_POINT('Ctrl Pts',(-8.76814132834432,-1.01583545019896,
18.9169816338124));
#19302=CARTESIAN_POINT('Ctrl Pts',(-8.50243547044552,-1.0164720823066,18.9294625670606));
#19303=CARTESIAN_POINT('Ctrl Pts',(-8.23672961254673,-1.01710871441424,
18.9419435003088));
#19304=CARTESIAN_POINT('Ctrl Pts',(-7.9723884693337,-0.908541417082972,
18.954424433557));
#19305=CARTESIAN_POINT('Ctrl Pts',(-7.78383148002365,-0.721334926798837,
18.9669053668052));
#19306=CARTESIAN_POINT('Ctrl Pts',(-7.5952744907136,-0.534128436514702,
18.9793863000534));
#19307=CARTESIAN_POINT('Ctrl Pts',(-7.48480993131709,-0.270574496756018,
18.9918672333016));
#19308=CARTESIAN_POINT('Ctrl Pts',(-7.48353667075686,-0.00487092690849199,
19.0043481665498));
#19309=CARTESIAN_POINT('Ctrl Pts',(-7.48226341019662,0.260832642939034,
19.016829099798));
#19310=CARTESIAN_POINT('Ctrl Pts',(-7.59019703546742,0.525433154240298,
19.0293100330462));
#19311=CARTESIAN_POINT('Ctrl Pts',(-7.7769512065251,0.714438148393189,19.0417909662944));
#19312=CARTESIAN_POINT('Ctrl Pts',(-7.96370537758277,0.90344314254608,19.0542718995426));
#19313=CARTESIAN_POINT('Ctrl Pts',(-8.22699388814824,1.01453885915659,19.0667528327907));
#19314=CARTESIAN_POINT('Ctrl Pts',(-8.49269364459159,1.01644874085989,19.0792337660389));
#19315=CARTESIAN_POINT('Ctrl Pts',(-8.75839340103493,1.01835862256318,19.0917146992871));
#19316=CARTESIAN_POINT('Ctrl Pts',(-9.02325176140396,0.911059288978948,
19.1041956325353));
#19317=CARTESIAN_POINT('Ctrl Pts',(-9.2127036753585,0.724758509267388,19.1166765657835));
#19318=CARTESIAN_POINT('Ctrl Pts',(-9.40215558931304,0.538457729555827,
19.1291574990317));
#19319=CARTESIAN_POINT('Ctrl Pts',(-9.51388182535849,0.275436159672093,
19.1416384322799));
#19320=CARTESIAN_POINT('Ctrl Pts',(-9.51642831724057,0.00974174196395182,
19.1541193655281));
#19321=CARTESIAN_POINT('Ctrl Pts',(-9.51645943884197,0.00649459406668756,
19.1542718995426));
#19322=CARTESIAN_POINT('Ctrl Pts',(-9.516475,0.00324729703410568,19.154424433557));
#19323=CARTESIAN_POINT('Ctrl Pts',(-9.516475,1.06710171779606E-12,19.1545769675715));
#19324=CARTESIAN_POINT('Origin',(-8.5,0.,1.24542303242842));
#19325=CARTESIAN_POINT('',(-9.516475,9.38545125247982E-13,18.4954230324285));
#19326=CARTESIAN_POINT('',(-9.516475,9.65488938827549E-13,18.5545769675715));
#19327=CARTESIAN_POINT('',(-9.516475,1.78524650477582E-12,1.24542303242842));
#19328=CARTESIAN_POINT('Ctrl Pts',(-9.516475,9.38545125247982E-13,18.4954230324285));
#19329=CARTESIAN_POINT('Ctrl Pts',(-9.51647500000024,-0.265706620583049,
18.5079039656766));
#19330=CARTESIAN_POINT('Ctrl Pts',(-9.40727465387243,-0.529786878176341,
18.5203848989248));
#19331=CARTESIAN_POINT('Ctrl Pts',(-9.21961691907818,-0.717894780174249,
18.532865832173));
#19332=CARTESIAN_POINT('Ctrl Pts',(-9.03195918428393,-0.906002682172157,
18.5453467654212));
#19333=CARTESIAN_POINT('Ctrl Pts',(-8.76814132834436,-1.01583545019894,
18.5578276986694));
#19334=CARTESIAN_POINT('Ctrl Pts',(-8.50243547044559,-1.0164720823066,18.5703086319176));
#19335=CARTESIAN_POINT('Ctrl Pts',(-8.23672961254682,-1.01710871441425,
18.5827895651658));
#19336=CARTESIAN_POINT('Ctrl Pts',(-7.9723884693338,-0.908541417083023,
18.595270498414));
#19337=CARTESIAN_POINT('Ctrl Pts',(-7.78383148002374,-0.721334926798925,
18.6077514316622));
#19338=CARTESIAN_POINT('Ctrl Pts',(-7.59527449071368,-0.534128436514826,
18.6202323649104));
#19339=CARTESIAN_POINT('Ctrl Pts',(-7.48480993131714,-0.270574496756181,
18.6327132981586));
#19340=CARTESIAN_POINT('Ctrl Pts',(-7.48353667075686,-0.00487092690867425,
18.6451942314068));
#19341=CARTESIAN_POINT('Ctrl Pts',(-7.48226341019657,0.260832642938833,
18.6576751646549));
#19342=CARTESIAN_POINT('Ctrl Pts',(-7.59019703546731,0.525433154240097,
18.6701560979031));
#19343=CARTESIAN_POINT('Ctrl Pts',(-7.77695120652493,0.714438148393018,
18.6826370311513));
#19344=CARTESIAN_POINT('Ctrl Pts',(-7.96370537758255,0.90344314254594,18.6951179643995));
#19345=CARTESIAN_POINT('Ctrl Pts',(-8.22699388814797,1.01453885915651,18.7075988976477));
#19346=CARTESIAN_POINT('Ctrl Pts',(-8.49269364459129,1.01644874085988,18.7200798308959));
#19347=CARTESIAN_POINT('Ctrl Pts',(-8.75839340103462,1.01835862256325,18.7325607641441));
#19348=CARTESIAN_POINT('Ctrl Pts',(-9.02325176140365,0.911059288979118,
18.7450416973923));
#19349=CARTESIAN_POINT('Ctrl Pts',(-9.21270367535825,0.724758509267637,
18.7575226306405));
#19350=CARTESIAN_POINT('Ctrl Pts',(-9.40215558931284,0.538457729556156,
18.7700035638887));
#19351=CARTESIAN_POINT('Ctrl Pts',(-9.51388182535838,0.275436159672486,
18.7824844971369));
#19352=CARTESIAN_POINT('Ctrl Pts',(-9.51642831724057,0.00974174196436518,
18.794965430385));
#19353=CARTESIAN_POINT('Ctrl Pts',(-9.51645943884197,0.00649459406694687,
18.7951179643995));
#19354=CARTESIAN_POINT('Ctrl Pts',(-9.516475,0.00324729703421089,18.795270498414));
#19355=CARTESIAN_POINT('Ctrl Pts',(-9.516475,1.01824147182551E-12,18.7954230324285));
#19356=CARTESIAN_POINT('Ctrl Pts',(-9.516475,9.65488938827549E-13,18.5545769675715));
#19357=CARTESIAN_POINT('Ctrl Pts',(-9.51647500000025,-0.265706620583022,
18.5670579008197));
#19358=CARTESIAN_POINT('Ctrl Pts',(-9.40727465387244,-0.529786878176317,
18.5795388340679));
#19359=CARTESIAN_POINT('Ctrl Pts',(-9.2196169190782,-0.717894780174229,
18.5920197673161));
#19360=CARTESIAN_POINT('Ctrl Pts',(-9.03195918428395,-0.906002682172142,
18.6045007005642));
#19361=CARTESIAN_POINT('Ctrl Pts',(-8.76814132834439,-1.01583545019893,
18.6169816338124));
#19362=CARTESIAN_POINT('Ctrl Pts',(-8.50243547044562,-1.0164720823066,18.6294625670606));
#19363=CARTESIAN_POINT('Ctrl Pts',(-8.23672961254684,-1.01710871441426,
18.6419435003088));
#19364=CARTESIAN_POINT('Ctrl Pts',(-7.97238846933382,-0.908541417083037,
18.654424433557));
#19365=CARTESIAN_POINT('Ctrl Pts',(-7.78383148002376,-0.721334926798944,
18.6669053668052));
#19366=CARTESIAN_POINT('Ctrl Pts',(-7.59527449071369,-0.53412843651485,
18.6793863000534));
#19367=CARTESIAN_POINT('Ctrl Pts',(-7.48480993131715,-0.270574496756208,
18.6918672333016));
#19368=CARTESIAN_POINT('Ctrl Pts',(-7.48353667075686,-0.0048709269087012,
18.7043481665498));
#19369=CARTESIAN_POINT('Ctrl Pts',(-7.48226341019657,0.260832642938806,
18.716829099798));
#19370=CARTESIAN_POINT('Ctrl Pts',(-7.5901970354673,0.525433154240073,18.7293100330462));
#19371=CARTESIAN_POINT('Ctrl Pts',(-7.77695120652491,0.714438148392999,
18.7417909662943));
#19372=CARTESIAN_POINT('Ctrl Pts',(-7.96370537758252,0.903443142545926,
18.7542718995425));
#19373=CARTESIAN_POINT('Ctrl Pts',(-8.22699388814794,1.01453885915651,18.7667528327907));
#19374=CARTESIAN_POINT('Ctrl Pts',(-8.49269364459126,1.01644874085988,18.7792337660389));
#19375=CARTESIAN_POINT('Ctrl Pts',(-8.75839340103459,1.01835862256326,18.7917146992871));
#19376=CARTESIAN_POINT('Ctrl Pts',(-9.02325176140363,0.911059288979131,
18.8041956325353));
#19377=CARTESIAN_POINT('Ctrl Pts',(-9.21270367535823,0.724758509267656,
18.8166765657835));
#19378=CARTESIAN_POINT('Ctrl Pts',(-9.40215558931282,0.53845772955618,18.8291574990317));
#19379=CARTESIAN_POINT('Ctrl Pts',(-9.51388182535837,0.275436159672513,
18.8416384322799));
#19380=CARTESIAN_POINT('Ctrl Pts',(-9.51642831724057,0.00974174196439213,
18.8541193655281));
#19381=CARTESIAN_POINT('Ctrl Pts',(-9.51645943884197,0.00649459406695455,
18.8542718995425));
#19382=CARTESIAN_POINT('Ctrl Pts',(-9.516475,0.00324729703419927,18.854424433557));
#19383=CARTESIAN_POINT('Ctrl Pts',(-9.516475,9.87405371218534E-13,18.8545769675715));
#19384=CARTESIAN_POINT('Origin',(-8.5,0.,1.24542303242842));
#19385=CARTESIAN_POINT('',(-9.516475,9.16628692856997E-13,18.1954230324285));
#19386=CARTESIAN_POINT('',(-9.516475,9.43572506436564E-13,18.2545769675715));
#19387=CARTESIAN_POINT('',(-9.516475,1.78524650477582E-12,1.24542303242842));
#19388=CARTESIAN_POINT('Ctrl Pts',(-9.516475,9.74408607043537E-13,18.1954230324285));
#19389=CARTESIAN_POINT('Ctrl Pts',(-9.51647500000025,-0.265706620583014,
18.2079039656766));
#19390=CARTESIAN_POINT('Ctrl Pts',(-9.40727465387245,-0.529786878176309,
18.2203848989248));
#19391=CARTESIAN_POINT('Ctrl Pts',(-9.2196169190782,-0.717894780174223,
18.232865832173));
#19392=CARTESIAN_POINT('Ctrl Pts',(-9.03195918428396,-0.906002682172138,
18.2453467654212));
#19393=CARTESIAN_POINT('Ctrl Pts',(-8.7681413283444,-1.01583545019893,18.2578276986694));
#19394=CARTESIAN_POINT('Ctrl Pts',(-8.50243547044563,-1.0164720823066,18.2703086319176));
#19395=CARTESIAN_POINT('Ctrl Pts',(-8.23672961254685,-1.01710871441426,
18.2827895651658));
#19396=CARTESIAN_POINT('Ctrl Pts',(-7.97238846933383,-0.908541417083041,
18.295270498414));
#19397=CARTESIAN_POINT('Ctrl Pts',(-7.78383148002376,-0.72133492679895,
18.3077514316622));
#19398=CARTESIAN_POINT('Ctrl Pts',(-7.5952744907137,-0.534128436514858,
18.3202323649104));
#19399=CARTESIAN_POINT('Ctrl Pts',(-7.48480993131715,-0.270574496756217,
18.3327132981586));
#19400=CARTESIAN_POINT('Ctrl Pts',(-7.48353667075686,-0.00487092690871011,
18.3451942314068));
#19401=CARTESIAN_POINT('Ctrl Pts',(-7.48226341019656,0.260832642938797,
18.3576751646549));
#19402=CARTESIAN_POINT('Ctrl Pts',(-7.59019703546729,0.525433154240064,
18.3701560979031));
#19403=CARTESIAN_POINT('Ctrl Pts',(-7.7769512065249,0.714438148392993,18.3826370311513));
#19404=CARTESIAN_POINT('Ctrl Pts',(-7.96370537758251,0.903443142545921,
18.3951179643995));
#19405=CARTESIAN_POINT('Ctrl Pts',(-8.22699388814793,1.0145388591565,18.4075988976477));
#19406=CARTESIAN_POINT('Ctrl Pts',(-8.49269364459126,1.01644874085988,18.4200798308959));
#19407=CARTESIAN_POINT('Ctrl Pts',(-8.75839340103458,1.01835862256326,18.4325607641441));
#19408=CARTESIAN_POINT('Ctrl Pts',(-9.02325176140362,0.911059288979136,
18.4450416973923));
#19409=CARTESIAN_POINT('Ctrl Pts',(-9.21270367535822,0.724758509267662,
18.4575226306405));
#19410=CARTESIAN_POINT('Ctrl Pts',(-9.40215558931282,0.538457729556188,
18.4700035638887));
#19411=CARTESIAN_POINT('Ctrl Pts',(-9.51388182535837,0.275436159672521,
18.4824844971369));
#19412=CARTESIAN_POINT('Ctrl Pts',(-9.51642831724057,0.00974174196440104,
18.494965430385));
#19413=CARTESIAN_POINT('Ctrl Pts',(-9.51645943884197,0.00649459406694421,
18.4951179643995));
#19414=CARTESIAN_POINT('Ctrl Pts',(-9.516475,0.00324729703416963,18.495270498414));
#19415=CARTESIAN_POINT('Ctrl Pts',(-9.516475,9.38545125247982E-13,18.4954230324285));
#19416=CARTESIAN_POINT('Ctrl Pts',(-9.516475,1.0013524206231E-12,18.2545769675715));
#19417=CARTESIAN_POINT('Ctrl Pts',(-9.51647500000026,-0.265706620582967,
18.2670579008197));
#19418=CARTESIAN_POINT('Ctrl Pts',(-9.40727465387248,-0.529786878176246,
18.2795388340679));
#19419=CARTESIAN_POINT('Ctrl Pts',(-9.21961691907826,-0.717894780174163,
18.292019767316));
#19420=CARTESIAN_POINT('Ctrl Pts',(-9.03195918428405,-0.90600268217208,
18.3045007005642));
#19421=CARTESIAN_POINT('Ctrl Pts',(-8.76814132834452,-1.01583545019889,
18.3169816338124));
#19422=CARTESIAN_POINT('Ctrl Pts',(-8.50243547044577,-1.0164720823066,18.3294625670606));
#19423=CARTESIAN_POINT('Ctrl Pts',(-8.23672961254701,-1.0171087144143,18.3419435003088));
#19424=CARTESIAN_POINT('Ctrl Pts',(-7.97238846933399,-0.908541417083132,
18.354424433557));
#19425=CARTESIAN_POINT('Ctrl Pts',(-7.78383148002391,-0.721334926799091,
18.3669053668052));
#19426=CARTESIAN_POINT('Ctrl Pts',(-7.59527449071382,-0.53412843651505,
18.3793863000534));
#19427=CARTESIAN_POINT('Ctrl Pts',(-7.48480993131722,-0.270574496756455,
18.3918672333016));
#19428=CARTESIAN_POINT('Ctrl Pts',(-7.48353667075686,-0.00487092690896818,
18.4043481665498));
#19429=CARTESIAN_POINT('Ctrl Pts',(-7.4822634101965,0.260832642938519,18.416829099798));
#19430=CARTESIAN_POINT('Ctrl Pts',(-7.59019703546714,0.525433154239796,
18.4293100330461));
#19431=CARTESIAN_POINT('Ctrl Pts',(-7.77695120652468,0.714438148392768,
18.4417909662943));
#19432=CARTESIAN_POINT('Ctrl Pts',(-7.96370537758222,0.90344314254574,18.4542718995425));
#19433=CARTESIAN_POINT('Ctrl Pts',(-8.22699388814758,1.0145388591564,18.4667528327907));
#19434=CARTESIAN_POINT('Ctrl Pts',(-8.49269364459088,1.01644874085988,18.4792337660389));
#19435=CARTESIAN_POINT('Ctrl Pts',(-8.75839340103419,1.01835862256336,18.4917146992871));
#19436=CARTESIAN_POINT('Ctrl Pts',(-9.02325176140325,0.911059288979345,
18.5041956325353));
#19437=CARTESIAN_POINT('Ctrl Pts',(-9.21270367535791,0.724758509267965,
18.5166765657835));
#19438=CARTESIAN_POINT('Ctrl Pts',(-9.40215558931258,0.538457729556585,
18.5291574990317));
#19439=CARTESIAN_POINT('Ctrl Pts',(-9.51388182535823,0.27543615967299,18.5416384322799));
#19440=CARTESIAN_POINT('Ctrl Pts',(-9.51642831724057,0.00974174196489021,
18.554119365528));
#19441=CARTESIAN_POINT('Ctrl Pts',(-9.51645943884196,0.00649459406727931,
18.5542718995425));
#19442=CARTESIAN_POINT('Ctrl Pts',(-9.516475,0.00324729703435065,18.554424433557));
#19443=CARTESIAN_POINT('Ctrl Pts',(-9.516475,9.65488938827549E-13,18.5545769675715));
#19444=CARTESIAN_POINT('Origin',(-8.5,0.,1.24542303242842));
#19445=CARTESIAN_POINT('',(-9.516475,8.94712260466012E-13,17.8954230324285));
#19446=CARTESIAN_POINT('',(-9.51621303022904,-8.85939138849132E-5,17.9545769675715));
#19447=CARTESIAN_POINT('',(-9.516475,1.78524650477582E-12,1.24542303242842));
#19448=CARTESIAN_POINT('Ctrl Pts',(-9.516475,9.52492174652552E-13,17.8954230324285));
#19449=CARTESIAN_POINT('Ctrl Pts',(-9.51647500000025,-0.265706620583055,
17.9079039656766));
#19450=CARTESIAN_POINT('Ctrl Pts',(-9.40727465387242,-0.529786878176366,
17.9203848989248));
#19451=CARTESIAN_POINT('Ctrl Pts',(-9.21961691907815,-0.71789478017428,
17.932865832173));
#19452=CARTESIAN_POINT('Ctrl Pts',(-9.03195918428387,-0.906002682172193,
17.9453467654212));
#19453=CARTESIAN_POINT('Ctrl Pts',(-8.76814132834428,-1.01583545019897,
17.9578276986694));
#19454=CARTESIAN_POINT('Ctrl Pts',(-8.50243547044549,-1.0164720823066,17.9703086319176));
#19455=CARTESIAN_POINT('Ctrl Pts',(-8.23672961254669,-1.01710871441423,
17.9827895651658));
#19456=CARTESIAN_POINT('Ctrl Pts',(-7.97238846933367,-0.908541417082954,
17.995270498414));
#19457=CARTESIAN_POINT('Ctrl Pts',(-7.78383148002362,-0.721334926798812,
18.0077514316622));
#19458=CARTESIAN_POINT('Ctrl Pts',(-7.59527449071358,-0.534128436514671,
18.0202323649104));
#19459=CARTESIAN_POINT('Ctrl Pts',(-7.48480993131709,-0.270574496755983,
18.0327132981586));
#19460=CARTESIAN_POINT('Ctrl Pts',(-7.48353667075686,-0.00487092690845708,
18.0451942314068));
#19461=CARTESIAN_POINT('Ctrl Pts',(-7.48226341019663,0.260832642939069,
18.057675164655));
#19462=CARTESIAN_POINT('Ctrl Pts',(-7.59019703546744,0.525433154240329,
18.0701560979031));
#19463=CARTESIAN_POINT('Ctrl Pts',(-7.77695120652512,0.714438148393214,
18.0826370311513));
#19464=CARTESIAN_POINT('Ctrl Pts',(-7.9637053775828,0.903443142546098,18.0951179643995));
#19465=CARTESIAN_POINT('Ctrl Pts',(-8.22699388814828,1.0145388591566,18.1075988976477));
#19466=CARTESIAN_POINT('Ctrl Pts',(-8.49269364459163,1.01644874085989,18.1200798308959));
#19467=CARTESIAN_POINT('Ctrl Pts',(-8.75839340103497,1.01835862256317,18.1325607641441));
#19468=CARTESIAN_POINT('Ctrl Pts',(-9.02325176140399,0.91105928897893,18.1450416973923));
#19469=CARTESIAN_POINT('Ctrl Pts',(-9.21270367535852,0.724758509267363,
18.1575226306405));
#19470=CARTESIAN_POINT('Ctrl Pts',(-9.40215558931306,0.538457729555796,
18.1700035638887));
#19471=CARTESIAN_POINT('Ctrl Pts',(-9.5138818253585,0.275436159672058,18.1824844971369));
#19472=CARTESIAN_POINT('Ctrl Pts',(-9.51642831724057,0.00974174196391691,
18.1949654303851));
#19473=CARTESIAN_POINT('Ctrl Pts',(-9.51645943884197,0.00649459406663339,
18.1951179643995));
#19474=CARTESIAN_POINT('Ctrl Pts',(-9.516475,0.0032472970340322,18.195270498414));
#19475=CARTESIAN_POINT('Ctrl Pts',(-9.516475,9.74408607043537E-13,18.1954230324285));
#19476=CARTESIAN_POINT('Ctrl Pts',(-9.516475,9.21656074045579E-13,17.9545769675715));
#19477=CARTESIAN_POINT('Ctrl Pts',(-9.51647500000024,-0.265706620583009,
17.9670579008197));
#19478=CARTESIAN_POINT('Ctrl Pts',(-9.40727465387247,-0.529786878176242,
17.9795388340679));
#19479=CARTESIAN_POINT('Ctrl Pts',(-9.21961691907829,-0.717894780174138,
17.992019767316));
#19480=CARTESIAN_POINT('Ctrl Pts',(-9.03195918428411,-0.906002682172034,
18.0045007005642));
#19481=CARTESIAN_POINT('Ctrl Pts',(-8.76814132834463,-1.01583545019885,
18.0169816338124));
#19482=CARTESIAN_POINT('Ctrl Pts',(-8.50243547044592,-1.0164720823066,18.0294625670606));
#19483=CARTESIAN_POINT('Ctrl Pts',(-8.2367296125472,-1.01710871441434,18.0419435003088));
#19484=CARTESIAN_POINT('Ctrl Pts',(-7.9723884693342,-0.908541417083243,
18.054424433557));
#19485=CARTESIAN_POINT('Ctrl Pts',(-7.7838314800241,-0.721334926799279,
18.0669053668052));
#19486=CARTESIAN_POINT('Ctrl Pts',(-7.59527449071399,-0.534128436515315,
18.0793863000534));
#19487=CARTESIAN_POINT('Ctrl Pts',(-7.48480993131732,-0.270574496756799,
18.0918672333016));
#19488=CARTESIAN_POINT('Ctrl Pts',(-7.48353667075686,-0.00487092690935071,
18.1043481665497));
#19489=CARTESIAN_POINT('Ctrl Pts',(-7.4822634101964,0.260832642938097,18.1168290997979));
#19490=CARTESIAN_POINT('Ctrl Pts',(-7.59019703546691,0.525433154239377,
18.1293100330461));
#19491=CARTESIAN_POINT('Ctrl Pts',(-7.77695120652433,0.714438148392414,
18.1417909662943));
#19492=CARTESIAN_POINT('Ctrl Pts',(-7.96370537758175,0.90344314254545,18.1542718995425));
#19493=CARTESIAN_POINT('Ctrl Pts',(-8.226993888147,1.01453885915624,18.1667528327907));
#19494=CARTESIAN_POINT('Ctrl Pts',(-8.49269364459027,1.01644874085988,18.1792337660389));
#19495=CARTESIAN_POINT('Ctrl Pts',(-8.75839340103353,1.01835862256351,18.1917146992871));
#19496=CARTESIAN_POINT('Ctrl Pts',(-9.02325176140262,0.911059288979693,
18.2041956325353));
#19497=CARTESIAN_POINT('Ctrl Pts',(-9.21270367535739,0.724758509268476,
18.2166765657834));
#19498=CARTESIAN_POINT('Ctrl Pts',(-9.40215558931216,0.538457729557259,
18.2291574990316));
#19499=CARTESIAN_POINT('Ctrl Pts',(-9.51388182535801,0.275436159673794,
18.2416384322798));
#19500=CARTESIAN_POINT('Ctrl Pts',(-9.51642831724056,0.00974174196573495,
18.254119365528));
#19501=CARTESIAN_POINT('Ctrl Pts',(-9.51645943884196,0.00649459406785445,
18.2542718995425));
#19502=CARTESIAN_POINT('Ctrl Pts',(-9.516475,0.00324729703465622,18.254424433557));
#19503=CARTESIAN_POINT('Ctrl Pts',(-9.516475,1.0013524206231E-12,18.2545769675715));
#19504=CARTESIAN_POINT('Origin',(-8.5,0.,1.24542303242842));
#19505=CARTESIAN_POINT('',(-9.516475,8.72795828075027E-13,17.5954230324285));
#19506=CARTESIAN_POINT('',(-9.51570671108984,0.000850778838430766,17.6545769675715));
#19507=CARTESIAN_POINT('',(-9.516475,1.78524650477582E-12,1.24542303242842));
#19508=CARTESIAN_POINT('Ctrl Pts',(-9.516475,9.30575742261567E-13,17.5954230324285));
#19509=CARTESIAN_POINT('Ctrl Pts',(-9.51647500000024,-0.265706620583019,
17.6079039656766));
#19510=CARTESIAN_POINT('Ctrl Pts',(-9.40727465387245,-0.529786878176272,
17.6203848989248));
#19511=CARTESIAN_POINT('Ctrl Pts',(-9.21961691907825,-0.717894780174172,
17.632865832173));
#19512=CARTESIAN_POINT('Ctrl Pts',(-9.03195918428405,-0.906002682172073,
17.6453467654212));
#19513=CARTESIAN_POINT('Ctrl Pts',(-8.76814132834455,-1.01583545019888,
17.6578276986694));
#19514=CARTESIAN_POINT('Ctrl Pts',(-8.50243547044581,-1.0164720823066,17.6703086319176));
#19515=CARTESIAN_POINT('Ctrl Pts',(-8.23672961254708,-1.01710871441431,
17.6827895651658));
#19516=CARTESIAN_POINT('Ctrl Pts',(-7.97238846933407,-0.908541417083172,
17.695270498414));
#19517=CARTESIAN_POINT('Ctrl Pts',(-7.78383148002398,-0.721334926799163,
17.7077514316622));
#19518=CARTESIAN_POINT('Ctrl Pts',(-7.59527449071389,-0.534128436515155,
17.7202323649103));
#19519=CARTESIAN_POINT('Ctrl Pts',(-7.48480993131726,-0.270574496756596,
17.7327132981585));
#19520=CARTESIAN_POINT('Ctrl Pts',(-7.48353667075686,-0.00487092690912852,
17.7451942314067));
#19521=CARTESIAN_POINT('Ctrl Pts',(-7.48226341019646,0.260832642938339,
17.7576751646549));
#19522=CARTESIAN_POINT('Ctrl Pts',(-7.59019703546705,0.525433154239614,
17.7701560979031));
#19523=CARTESIAN_POINT('Ctrl Pts',(-7.77695120652453,0.714438148392613,
17.7826370311513));
#19524=CARTESIAN_POINT('Ctrl Pts',(-7.96370537758201,0.903443142545612,
17.7951179643995));
#19525=CARTESIAN_POINT('Ctrl Pts',(-8.22699388814732,1.01453885915633,17.8075988976477));
#19526=CARTESIAN_POINT('Ctrl Pts',(-8.49269364459061,1.01644874085988,17.8200798308959));
#19527=CARTESIAN_POINT('Ctrl Pts',(-8.75839340103389,1.01835862256343,17.8325607641441));
#19528=CARTESIAN_POINT('Ctrl Pts',(-9.02325176140296,0.911059288979503,
17.8450416973922));
#19529=CARTESIAN_POINT('Ctrl Pts',(-9.21270367535767,0.724758509268199,
17.8575226306404));
#19530=CARTESIAN_POINT('Ctrl Pts',(-9.40215558931239,0.538457729556894,
17.8700035638886));
#19531=CARTESIAN_POINT('Ctrl Pts',(-9.51388182535813,0.275436159673361,
17.8824844971368));
#19532=CARTESIAN_POINT('Ctrl Pts',(-9.51642831724056,0.00974174196528165,
17.894965430385));
#19533=CARTESIAN_POINT('Ctrl Pts',(-9.51645943884196,0.00649459406753596,
17.8951179643995));
#19534=CARTESIAN_POINT('Ctrl Pts',(-9.516475,0.00324729703447251,17.895270498414));
#19535=CARTESIAN_POINT('Ctrl Pts',(-9.516475,9.52492174652552E-13,17.8954230324285));
#19536=CARTESIAN_POINT('Ctrl Pts',(-9.51570671108984,0.00085077883843071,
17.6545769675715));
#19537=CARTESIAN_POINT('Ctrl Pts',(-9.51391306809171,-0.234644624850221,
17.6656239612628));
#19538=CARTESIAN_POINT('Ctrl Pts',(-9.31537561793486,-0.812092956351842,
17.6925782961058));
#19539=CARTESIAN_POINT('Ctrl Pts',(-8.35176929286965,-1.19346183771808,
17.7354399721004));
#19540=CARTESIAN_POINT('Ctrl Pts',(-7.57414417389279,-0.632820621048115,
17.7752083249795));
#19541=CARTESIAN_POINT('Ctrl Pts',(-7.44469102409625,0.0541105458809273,
17.8070230072827));
#19542=CARTESIAN_POINT('Ctrl Pts',(-7.64372479594433,0.724198677214912,
17.8388376895859));
#19543=CARTESIAN_POINT('Ctrl Pts',(-8.47461430237912,1.20236394946876,17.878606042465));
#19544=CARTESIAN_POINT('Ctrl Pts',(-9.35917600400969,0.742620125736834,
17.9198370253188));
#19545=CARTESIAN_POINT('Ctrl Pts',(-9.51423527094977,0.200593991219319,
17.9451606670209));
#19546=CARTESIAN_POINT('Ctrl Pts',(-9.51501920748671,-0.000492325344205985,
17.9545769675715));
#19547=CARTESIAN_POINT('Origin',(-8.5,0.,1.24542303242842));
#19548=CARTESIAN_POINT('',(-9.516475,8.50879395684042E-13,17.2954230324285));
#19549=CARTESIAN_POINT('',(-9.51688182003018,5.98281162011358E-5,17.3545769675715));
#19550=CARTESIAN_POINT('',(-9.516475,1.78524650477582E-12,1.24542303242842));
#19551=CARTESIAN_POINT('Ctrl Pts',(-9.516475,8.50879395684042E-13,17.2954230324285));
#19552=CARTESIAN_POINT('Ctrl Pts',(-9.51647500000022,-0.265706620583098,
17.3079039656766));
#19553=CARTESIAN_POINT('Ctrl Pts',(-9.40727465387241,-0.529786878176343,
17.3203848989248));
#19554=CARTESIAN_POINT('Ctrl Pts',(-9.2196169190782,-0.717894780174229,
17.332865832173));
#19555=CARTESIAN_POINT('Ctrl Pts',(-9.03195918428398,-0.906002682172115,
17.3453467654212));
#19556=CARTESIAN_POINT('Ctrl Pts',(-8.76814132834447,-1.0158354501989,17.3578276986694));
#19557=CARTESIAN_POINT('Ctrl Pts',(-8.50243547044573,-1.0164720823066,17.3703086319176));
#19558=CARTESIAN_POINT('Ctrl Pts',(-8.236729612547,-1.01710871441429,17.3827895651658));
#19559=CARTESIAN_POINT('Ctrl Pts',(-7.972388469334,-0.90854141708313,17.395270498414));
#19560=CARTESIAN_POINT('Ctrl Pts',(-7.78383148002392,-0.721334926799107,
17.4077514316622));
#19561=CARTESIAN_POINT('Ctrl Pts',(-7.59527449071384,-0.534128436515084,
17.4202323649104));
#19562=CARTESIAN_POINT('Ctrl Pts',(-7.48480993131724,-0.270574496756517,
17.4327132981585));
#19563=CARTESIAN_POINT('Ctrl Pts',(-7.48353667075686,-0.00487092690904882,
17.4451942314067));
#19564=CARTESIAN_POINT('Ctrl Pts',(-7.48226341019648,0.260832642938419,
17.4576751646549));
#19565=CARTESIAN_POINT('Ctrl Pts',(-7.59019703546709,0.525433154239685,
17.4701560979031));
#19566=CARTESIAN_POINT('Ctrl Pts',(-7.77695120652458,0.71443814839267,17.4826370311513));
#19567=CARTESIAN_POINT('Ctrl Pts',(-7.96370537758208,0.903443142545654,
17.4951179643995));
#19568=CARTESIAN_POINT('Ctrl Pts',(-8.2269938881474,1.01453885915635,17.5075988976477));
#19569=CARTESIAN_POINT('Ctrl Pts',(-8.49269364459069,1.01644874085988,17.5200798308959));
#19570=CARTESIAN_POINT('Ctrl Pts',(-8.75839340103397,1.01835862256341,17.5325607641441));
#19571=CARTESIAN_POINT('Ctrl Pts',(-9.02325176140304,0.911059288979462,
17.5450416973923));
#19572=CARTESIAN_POINT('Ctrl Pts',(-9.21270367535773,0.724758509268143,
17.5575226306404));
#19573=CARTESIAN_POINT('Ctrl Pts',(-9.40215558931243,0.538457729556824,
17.5700035638886));
#19574=CARTESIAN_POINT('Ctrl Pts',(-9.51388182535815,0.275436159673282,
17.5824844971368));
#19575=CARTESIAN_POINT('Ctrl Pts',(-9.51642831724056,0.00974174196520196,
17.594965430385));
#19576=CARTESIAN_POINT('Ctrl Pts',(-9.51645943884196,0.00649459406747552,
17.5951179643995));
#19577=CARTESIAN_POINT('Ctrl Pts',(-9.516475,0.00324729703443137,17.595270498414));
#19578=CARTESIAN_POINT('Ctrl Pts',(-9.516475,9.30575742261567E-13,17.5954230324285));
#19579=CARTESIAN_POINT('Ctrl Pts',(-9.51821859738619,0.000256418416867737,
17.3545769675715));
#19580=CARTESIAN_POINT('Ctrl Pts',(-9.5176126438481,-0.330488117619876,
17.3701799143531));
#19581=CARTESIAN_POINT('Ctrl Pts',(-9.16144800526121,-1.00019275742554,
17.4016902022864));
#19582=CARTESIAN_POINT('Ctrl Pts',(-8.21385965450184,-1.08434065304146,
17.4411541607954));
#19583=CARTESIAN_POINT('Ctrl Pts',(-7.66651569284325,-0.649545145099307,
17.4729688430987));
#19584=CARTESIAN_POINT('Ctrl Pts',(-7.37861109970015,-0.0125651679117135,
17.5047835254019));
#19585=CARTESIAN_POINT('Ctrl Pts',(-7.69412058637172,0.892682402266311,
17.544551878281));
#19586=CARTESIAN_POINT('Ctrl Pts',(-8.81654339210534,1.16012687698589,17.5922739017358));
#19587=CARTESIAN_POINT('Ctrl Pts',(-9.45404978590041,0.546214074355226,
17.6289489314993));
#19588=CARTESIAN_POINT('Ctrl Pts',(-9.51649586046696,0.104461726685567,
17.6497166201112));
#19589=CARTESIAN_POINT('Ctrl Pts',(-9.51570671108984,0.00085077883843071,
17.6545769675715));
#19590=CARTESIAN_POINT('Origin',(-8.5,0.,1.24542303242842));
#19591=CARTESIAN_POINT('',(-9.516475,8.28962963293057E-13,16.9954230324285));
#19592=CARTESIAN_POINT('',(-9.516475,8.55906776872624E-13,17.0545769675715));
#19593=CARTESIAN_POINT('',(-9.516475,1.78524650477582E-12,1.24542303242842));
#19594=CARTESIAN_POINT('Ctrl Pts',(-9.516475,8.28962963293057E-13,16.9954230324285));
#19595=CARTESIAN_POINT('Ctrl Pts',(-9.51647500000022,-0.26570662058314,
17.0079039656767));
#19596=CARTESIAN_POINT('Ctrl Pts',(-9.40727465387238,-0.5297868781764,17.0203848989248));
#19597=CARTESIAN_POINT('Ctrl Pts',(-9.21961691907814,-0.717894780174285,
17.032865832173));
#19598=CARTESIAN_POINT('Ctrl Pts',(-9.0319591842839,-0.90600268217217,17.0453467654212));
#19599=CARTESIAN_POINT('Ctrl Pts',(-8.76814132834435,-1.01583545019894,
17.0578276986694));
#19600=CARTESIAN_POINT('Ctrl Pts',(-8.5024354704456,-1.0164720823066,17.0703086319176));
#19601=CARTESIAN_POINT('Ctrl Pts',(-8.23672961254684,-1.01710871441425,
17.0827895651658));
#19602=CARTESIAN_POINT('Ctrl Pts',(-7.97238846933384,-0.908541417083042,
17.095270498414));
#19603=CARTESIAN_POINT('Ctrl Pts',(-7.78383148002378,-0.721334926798969,
17.1077514316622));
#19604=CARTESIAN_POINT('Ctrl Pts',(-7.59527449071373,-0.534128436514896,
17.1202323649104));
#19605=CARTESIAN_POINT('Ctrl Pts',(-7.48480993131718,-0.270574496756283,
17.1327132981586));
#19606=CARTESIAN_POINT('Ctrl Pts',(-7.48353667075686,-0.00487092690879579,
17.1451942314067));
#19607=CARTESIAN_POINT('Ctrl Pts',(-7.48226341019654,0.260832642938692,
17.1576751646549));
#19608=CARTESIAN_POINT('Ctrl Pts',(-7.59019703546723,0.52543315423995,17.1701560979031));
#19609=CARTESIAN_POINT('Ctrl Pts',(-7.7769512065248,0.714438148392891,17.1826370311513));
#19610=CARTESIAN_POINT('Ctrl Pts',(-7.96370537758237,0.903443142545831,
17.1951179643995));
#19611=CARTESIAN_POINT('Ctrl Pts',(-8.22699388814775,1.01453885915645,17.2075988976477));
#19612=CARTESIAN_POINT('Ctrl Pts',(-8.49269364459106,1.01644874085988,17.2200798308959));
#19613=CARTESIAN_POINT('Ctrl Pts',(-8.75839340103436,1.01835862256331,17.2325607641441));
#19614=CARTESIAN_POINT('Ctrl Pts',(-9.0232517614034,0.911059288979256,17.2450416973923));
#19615=CARTESIAN_POINT('Ctrl Pts',(-9.21270367535804,0.724758509267844,
17.2575226306405));
#19616=CARTESIAN_POINT('Ctrl Pts',(-9.40215558931267,0.538457729556432,
17.2700035638887));
#19617=CARTESIAN_POINT('Ctrl Pts',(-9.51388182535828,0.275436159672818,
17.2824844971368));
#19618=CARTESIAN_POINT('Ctrl Pts',(-9.51642831724057,0.00974174196471782,
17.294965430385));
#19619=CARTESIAN_POINT('Ctrl Pts',(-9.51645943884197,0.00649459406712618,
17.2951179643995));
#19620=CARTESIAN_POINT('Ctrl Pts',(-9.516475,0.00324729703421682,17.295270498414));
#19621=CARTESIAN_POINT('Ctrl Pts',(-9.516475,8.50879395684042E-13,17.2954230324285));
#19622=CARTESIAN_POINT('Ctrl Pts',(-9.516475,9.13686691059164E-13,17.0545769675715));
#19623=CARTESIAN_POINT('Ctrl Pts',(-9.51647500000024,-0.265706620583055,
17.0670579008197));
#19624=CARTESIAN_POINT('Ctrl Pts',(-9.40727465387243,-0.529786878176325,
17.0795388340679));
#19625=CARTESIAN_POINT('Ctrl Pts',(-9.2196169190782,-0.717894780174225,
17.092019767316));
#19626=CARTESIAN_POINT('Ctrl Pts',(-9.03195918428397,-0.906002682172126,
17.1045007005642));
#19627=CARTESIAN_POINT('Ctrl Pts',(-8.76814132834443,-1.01583545019892,
17.1169816338124));
#19628=CARTESIAN_POINT('Ctrl Pts',(-8.50243547044568,-1.0164720823066,17.1294625670606));
#19629=CARTESIAN_POINT('Ctrl Pts',(-8.23672961254693,-1.01710871441428,
17.1419435003088));
#19630=CARTESIAN_POINT('Ctrl Pts',(-7.97238846933391,-0.908541417083087,
17.154424433557));
#19631=CARTESIAN_POINT('Ctrl Pts',(-7.78383148002384,-0.721334926799029,
17.1669053668052));
#19632=CARTESIAN_POINT('Ctrl Pts',(-7.59527449071377,-0.534128436514972,
17.1793863000534));
#19633=CARTESIAN_POINT('Ctrl Pts',(-7.4848099313172,-0.270574496756368,
17.1918672333016));
#19634=CARTESIAN_POINT('Ctrl Pts',(-7.48353667075686,-0.00487092690888051,
17.2043481665498));
#19635=CARTESIAN_POINT('Ctrl Pts',(-7.48226341019652,0.260832642938607,
17.216829099798));
#19636=CARTESIAN_POINT('Ctrl Pts',(-7.59019703546719,0.525433154239874,
17.2293100330461));
#19637=CARTESIAN_POINT('Ctrl Pts',(-7.77695120652474,0.71443814839283,17.2417909662943));
#19638=CARTESIAN_POINT('Ctrl Pts',(-7.9637053775823,0.903443142545787,17.2542718995425));
#19639=CARTESIAN_POINT('Ctrl Pts',(-8.22699388814766,1.01453885915643,17.2667528327907));
#19640=CARTESIAN_POINT('Ctrl Pts',(-8.49269364459097,1.01644874085988,17.2792337660389));
#19641=CARTESIAN_POINT('Ctrl Pts',(-8.75839340103428,1.01835862256333,17.2917146992871));
#19642=CARTESIAN_POINT('Ctrl Pts',(-9.02325176140333,0.911059288979299,
17.3041956325353));
#19643=CARTESIAN_POINT('Ctrl Pts',(-9.21270367535798,0.724758509267903,
17.3166765657835));
#19644=CARTESIAN_POINT('Ctrl Pts',(-9.40215558931262,0.538457729556507,
17.3291574990317));
#19645=CARTESIAN_POINT('Ctrl Pts',(-9.51388182535826,0.275436159672903,
17.3416384322799));
#19646=CARTESIAN_POINT('Ctrl Pts',(-9.51642831724057,0.00974174196480255,
17.3541193655281));
#19647=CARTESIAN_POINT('Ctrl Pts',(-9.51645943884197,0.00649459406719165,
17.3542718995425));
#19648=CARTESIAN_POINT('Ctrl Pts',(-9.516475,0.00324729703426298,17.354424433557));
#19649=CARTESIAN_POINT('Ctrl Pts',(-9.516475,8.77823209263609E-13,17.3545769675715));
#19650=CARTESIAN_POINT('Origin',(-8.5,0.,1.24542303242842));
#19651=CARTESIAN_POINT('',(-9.516475,8.07046530902072E-13,16.6954230324285));
#19652=CARTESIAN_POINT('',(-9.51596013594239,0.000134652220364405,16.7545769675715));
#19653=CARTESIAN_POINT('',(-9.516475,1.78524650477582E-12,1.24542303242842));
#19654=CARTESIAN_POINT('Ctrl Pts',(-9.516475,7.49266616715532E-13,16.6954230324285));
#19655=CARTESIAN_POINT('Ctrl Pts',(-9.5164750000002,-0.265706620583219,
16.7079039656767));
#19656=CARTESIAN_POINT('Ctrl Pts',(-9.40727465387234,-0.529786878176472,
16.7203848989248));
#19657=CARTESIAN_POINT('Ctrl Pts',(-9.21961691907808,-0.717894780174342,
16.732865832173));
#19658=CARTESIAN_POINT('Ctrl Pts',(-9.03195918428382,-0.906002682172212,
16.7453467654212));
#19659=CARTESIAN_POINT('Ctrl Pts',(-8.76814132834427,-1.01583545019896,
16.7578276986694));
#19660=CARTESIAN_POINT('Ctrl Pts',(-8.50243547044552,-1.0164720823066,16.7703086319176));
#19661=CARTESIAN_POINT('Ctrl Pts',(-8.23672961254676,-1.01710871441423,
16.7827895651658));
#19662=CARTESIAN_POINT('Ctrl Pts',(-7.97238846933377,-0.908541417083001,
16.795270498414));
#19663=CARTESIAN_POINT('Ctrl Pts',(-7.78383148002373,-0.721334926798913,
16.8077514316622));
#19664=CARTESIAN_POINT('Ctrl Pts',(-7.59527449071369,-0.534128436514826,
16.8202323649104));
#19665=CARTESIAN_POINT('Ctrl Pts',(-7.48480993131715,-0.270574496756204,
16.8327132981586));
#19666=CARTESIAN_POINT('Ctrl Pts',(-7.48353667075686,-0.00487092690871609,
16.8451942314067));
#19667=CARTESIAN_POINT('Ctrl Pts',(-7.48226341019656,0.260832642938771,
16.8576751646549));
#19668=CARTESIAN_POINT('Ctrl Pts',(-7.59019703546727,0.525433154240021,
16.8701560979031));
#19669=CARTESIAN_POINT('Ctrl Pts',(-7.77695120652486,0.714438148392947,
16.8826370311513));
#19670=CARTESIAN_POINT('Ctrl Pts',(-7.96370537758244,0.903443142545873,
16.8951179643995));
#19671=CARTESIAN_POINT('Ctrl Pts',(-8.22699388814783,1.01453885915647,16.9075988976477));
#19672=CARTESIAN_POINT('Ctrl Pts',(-8.49269364459114,1.01644874085988,16.9200798308959));
#19673=CARTESIAN_POINT('Ctrl Pts',(-8.75839340103444,1.01835862256329,16.9325607641441));
#19674=CARTESIAN_POINT('Ctrl Pts',(-9.02325176140348,0.911059288979215,
16.9450416973923));
#19675=CARTESIAN_POINT('Ctrl Pts',(-9.21270367535809,0.724758509267788,
16.9575226306405));
#19676=CARTESIAN_POINT('Ctrl Pts',(-9.40215558931271,0.538457729556361,
16.9700035638887));
#19677=CARTESIAN_POINT('Ctrl Pts',(-9.5138818253583,0.275436159672739,16.9824844971368));
#19678=CARTESIAN_POINT('Ctrl Pts',(-9.51642831724057,0.00974174196463813,
16.994965430385));
#19679=CARTESIAN_POINT('Ctrl Pts',(-9.51645943884197,0.00649459406706575,
16.9951179643995));
#19680=CARTESIAN_POINT('Ctrl Pts',(-9.516475,0.00324729703417569,16.995270498414));
#19681=CARTESIAN_POINT('Ctrl Pts',(-9.516475,8.28962963293057E-13,16.9954230324285));
#19682=CARTESIAN_POINT('Ctrl Pts',(-9.516475,8.33990344481639E-13,16.7545769675715));
#19683=CARTESIAN_POINT('Ctrl Pts',(-9.51647500000022,-0.265706620583135,
16.7670579008197));
#19684=CARTESIAN_POINT('Ctrl Pts',(-9.40727465387239,-0.529786878176396,
16.7795388340679));
#19685=CARTESIAN_POINT('Ctrl Pts',(-9.21961691907814,-0.717894780174282,
16.7920197673161));
#19686=CARTESIAN_POINT('Ctrl Pts',(-9.0319591842839,-0.906002682172167,
16.8045007005642));
#19687=CARTESIAN_POINT('Ctrl Pts',(-8.76814132834435,-1.01583545019894,
16.8169816338124));
#19688=CARTESIAN_POINT('Ctrl Pts',(-8.5024354704456,-1.0164720823066,16.8294625670606));
#19689=CARTESIAN_POINT('Ctrl Pts',(-8.23672961254685,-1.01710871441426,
16.8419435003088));
#19690=CARTESIAN_POINT('Ctrl Pts',(-7.97238846933384,-0.908541417083045,
16.854424433557));
#19691=CARTESIAN_POINT('Ctrl Pts',(-7.78383148002379,-0.721334926798973,
16.8669053668052));
#19692=CARTESIAN_POINT('Ctrl Pts',(-7.59527449071373,-0.534128436514901,
16.8793863000534));
#19693=CARTESIAN_POINT('Ctrl Pts',(-7.48480993131718,-0.270574496756288,
16.8918672333016));
#19694=CARTESIAN_POINT('Ctrl Pts',(-7.48353667075686,-0.00487092690880082,
16.9043481665498));
#19695=CARTESIAN_POINT('Ctrl Pts',(-7.48226341019654,0.260832642938687,
16.916829099798));
#19696=CARTESIAN_POINT('Ctrl Pts',(-7.59019703546723,0.525433154239945,
16.9293100330461));
#19697=CARTESIAN_POINT('Ctrl Pts',(-7.7769512065248,0.714438148392887,16.9417909662943));
#19698=CARTESIAN_POINT('Ctrl Pts',(-7.96370537758237,0.903443142545829,
16.9542718995425));
#19699=CARTESIAN_POINT('Ctrl Pts',(-8.22699388814774,1.01453885915645,16.9667528327907));
#19700=CARTESIAN_POINT('Ctrl Pts',(-8.49269364459105,1.01644874085988,16.9792337660389));
#19701=CARTESIAN_POINT('Ctrl Pts',(-8.75839340103436,1.01835862256331,16.9917146992871));
#19702=CARTESIAN_POINT('Ctrl Pts',(-9.0232517614034,0.911059288979258,17.0041956325353));
#19703=CARTESIAN_POINT('Ctrl Pts',(-9.21270367535803,0.724758509267847,
17.0166765657835));
#19704=CARTESIAN_POINT('Ctrl Pts',(-9.40215558931266,0.538457729556436,
17.0291574990317));
#19705=CARTESIAN_POINT('Ctrl Pts',(-9.51388182535828,0.275436159672823,
17.0416384322799));
#19706=CARTESIAN_POINT('Ctrl Pts',(-9.51642831724057,0.00974174196472285,
17.0541193655281));
#19707=CARTESIAN_POINT('Ctrl Pts',(-9.51645943884197,0.00649459406715047,
17.0542718995425));
#19708=CARTESIAN_POINT('Ctrl Pts',(-9.516475,0.00324729703426041,17.054424433557));
#19709=CARTESIAN_POINT('Ctrl Pts',(-9.516475,9.13686691059164E-13,17.0545769675715));
#19710=CARTESIAN_POINT('Origin',(-8.5,0.,1.24542303242842));
#19711=CARTESIAN_POINT('',(-9.5164968973349,-2.65839347229251E-5,16.3954230324285));
#19712=CARTESIAN_POINT('',(-9.51655837487022,5.83812892711161E-5,16.4545769675715));
#19713=CARTESIAN_POINT('',(-9.516475,1.78524650477582E-12,1.24542303242842));
#19714=CARTESIAN_POINT('Ctrl Pts',(-9.516475,7.85130098511087E-13,16.3954230324285));
#19715=CARTESIAN_POINT('Ctrl Pts',(-9.51647500000021,-0.265706620583203,
16.4079039656767));
#19716=CARTESIAN_POINT('Ctrl Pts',(-9.40727465387235,-0.529786878176478,
16.4203848989248));
#19717=CARTESIAN_POINT('Ctrl Pts',(-9.21961691907807,-0.717894780174357,
16.432865832173));
#19718=CARTESIAN_POINT('Ctrl Pts',(-9.03195918428379,-0.906002682172237,
16.4453467654212));
#19719=CARTESIAN_POINT('Ctrl Pts',(-8.76814132834421,-1.01583545019898,
16.4578276986694));
#19720=CARTESIAN_POINT('Ctrl Pts',(-8.50243547044544,-1.0164720823066,16.4703086319176));
#19721=CARTESIAN_POINT('Ctrl Pts',(-8.23672961254666,-1.01710871441421,
16.4827895651658));
#19722=CARTESIAN_POINT('Ctrl Pts',(-7.97238846933366,-0.908541417082943,
16.495270498414));
#19723=CARTESIAN_POINT('Ctrl Pts',(-7.78383148002363,-0.721334926798817,
16.5077514316622));
#19724=CARTESIAN_POINT('Ctrl Pts',(-7.5952744907136,-0.53412843651469,16.5202323649104));
#19725=CARTESIAN_POINT('Ctrl Pts',(-7.4848099313171,-0.270574496756028,
16.5327132981586));
#19726=CARTESIAN_POINT('Ctrl Pts',(-7.48353667075686,-0.00487092690852084,
16.5451942314068));
#19727=CARTESIAN_POINT('Ctrl Pts',(-7.48226341019661,0.260832642938986,
16.5576751646549));
#19728=CARTESIAN_POINT('Ctrl Pts',(-7.59019703546739,0.525433154240234,
16.5701560979031));
#19729=CARTESIAN_POINT('Ctrl Pts',(-7.77695120652504,0.714438148393127,
16.5826370311513));
#19730=CARTESIAN_POINT('Ctrl Pts',(-7.96370537758268,0.903443142546021,
16.5951179643995));
#19731=CARTESIAN_POINT('Ctrl Pts',(-8.22699388814812,1.01453885915655,16.6075988976477));
#19732=CARTESIAN_POINT('Ctrl Pts',(-8.49269364459145,1.01644874085988,16.6200798308959));
#19733=CARTESIAN_POINT('Ctrl Pts',(-8.75839340103477,1.01835862256321,16.6325607641441));
#19734=CARTESIAN_POINT('Ctrl Pts',(-9.02325176140379,0.911059288979039,
16.6450416973923));
#19735=CARTESIAN_POINT('Ctrl Pts',(-9.21270367535836,0.724758509267529,
16.6575226306405));
#19736=CARTESIAN_POINT('Ctrl Pts',(-9.40215558931292,0.53845772955602,16.6700035638887));
#19737=CARTESIAN_POINT('Ctrl Pts',(-9.51388182535842,0.275436159672333,
16.6824844971369));
#19738=CARTESIAN_POINT('Ctrl Pts',(-9.51642831724057,0.00974174196421177,
16.6949654303851));
#19739=CARTESIAN_POINT('Ctrl Pts',(-9.51645943884197,0.00649459406675493,
16.6951179643995));
#19740=CARTESIAN_POINT('Ctrl Pts',(-9.516475,0.00324729703398035,16.695270498414));
#19741=CARTESIAN_POINT('Ctrl Pts',(-9.516475,7.49266616715532E-13,16.6954230324285));
#19742=CARTESIAN_POINT('Ctrl Pts',(-9.51726025283138,0.000549854815502043,
16.4545769675715));
#19743=CARTESIAN_POINT('Ctrl Pts',(-9.51657489923479,-0.114420558160816,
16.4599867618965));
#19744=CARTESIAN_POINT('Ctrl Pts',(-9.46572759915602,-0.399134064589724,
16.4733502267973));
#19745=CARTESIAN_POINT('Ctrl Pts',(-9.11467520479983,-0.938000704161855,
16.5026210328498));
#19746=CARTESIAN_POINT('Ctrl Pts',(-8.18204041706793,-1.15983848287103,
16.5423893857288));
#19747=CARTESIAN_POINT('Ctrl Pts',(-7.35207269505694,-0.358269358953146,
16.5901114091837));
#19748=CARTESIAN_POINT('Ctrl Pts',(-7.57822133797448,0.770938669115475,
16.6378334326386));
#19749=CARTESIAN_POINT('Ctrl Pts',(-8.64964987006652,1.19318859338267,16.6855554560934));
#19750=CARTESIAN_POINT('Ctrl Pts',(-9.41265229748654,0.642636493326239,
16.7244699677377));
#19751=CARTESIAN_POINT('Ctrl Pts',(-9.5151794075,0.152076348271911,16.7474771382304));
#19752=CARTESIAN_POINT('Ctrl Pts',(-9.51462108838776,0.000484852865797483,
16.7545769675715));
#19753=CARTESIAN_POINT('Origin',(-8.5,0.,1.24542303242842));
#19754=CARTESIAN_POINT('',(-9.5160543088948,-7.03488242669728E-5,16.0954230324285));
#19755=CARTESIAN_POINT('',(-9.51662919665684,-7.0250937289264E-5,16.1545769675715));
#19756=CARTESIAN_POINT('',(-9.516475,1.78524650477582E-12,1.24542303242842));
#19757=CARTESIAN_POINT('Ctrl Pts',(-9.51497316338417,-0.000251140182777485,
16.0954230324285));
#19758=CARTESIAN_POINT('Ctrl Pts',(-9.51542015839452,-0.151106629532047,
16.1024843671052));
#19759=CARTESIAN_POINT('Ctrl Pts',(-9.41308036725428,-0.641309918179512,
16.1254530429335));
#19760=CARTESIAN_POINT('Ctrl Pts',(-8.65222970570018,-1.19292557033944,
16.1643290599136));
#19761=CARTESIAN_POINT('Ctrl Pts',(-7.75981223837764,-0.842543822233083,
16.2040974127926));
#19762=CARTESIAN_POINT('Ctrl Pts',(-7.46421470806744,-0.209092634934189,
16.2359120950958));
#19763=CARTESIAN_POINT('Ctrl Pts',(-7.49095487068437,0.48940290682626,16.2677267773991));
#19764=CARTESIAN_POINT('Ctrl Pts',(-8.17744624771311,1.15857095575367,16.3074951302781));
#19765=CARTESIAN_POINT('Ctrl Pts',(-9.24219277385032,0.910507051205119,
16.3527117721465));
#19766=CARTESIAN_POINT('Ctrl Pts',(-9.514732772302,0.283866876007315,16.3820210728633));
#19767=CARTESIAN_POINT('Ctrl Pts',(-9.51712864820514,-0.000793545963003017,
16.3954230324284));
#19768=CARTESIAN_POINT('Ctrl Pts',(-9.516475,8.47937393886208E-13,16.1545769675715));
#19769=CARTESIAN_POINT('Ctrl Pts',(-9.51647500000022,-0.265706620583101,
16.1670579008197));
#19770=CARTESIAN_POINT('Ctrl Pts',(-9.40727465387241,-0.529786878176346,
16.1795388340679));
#19771=CARTESIAN_POINT('Ctrl Pts',(-9.21961691907819,-0.717894780174231,
16.1920197673161));
#19772=CARTESIAN_POINT('Ctrl Pts',(-9.03195918428398,-0.906002682172116,
16.2045007005642));
#19773=CARTESIAN_POINT('Ctrl Pts',(-8.76814132834446,-1.0158354501989,16.2169816338124));
#19774=CARTESIAN_POINT('Ctrl Pts',(-8.50243547044573,-1.0164720823066,16.2294625670606));
#19775=CARTESIAN_POINT('Ctrl Pts',(-8.236729612547,-1.01710871441429,16.2419435003088));
#19776=CARTESIAN_POINT('Ctrl Pts',(-7.972388469334,-0.908541417083129,16.254424433557));
#19777=CARTESIAN_POINT('Ctrl Pts',(-7.78383148002392,-0.721334926799105,
16.2669053668052));
#19778=CARTESIAN_POINT('Ctrl Pts',(-7.59527449071384,-0.534128436515081,
16.2793863000534));
#19779=CARTESIAN_POINT('Ctrl Pts',(-7.48480993131724,-0.270574496756514,
16.2918672333016));
#19780=CARTESIAN_POINT('Ctrl Pts',(-7.48353667075686,-0.00487092690904588,
16.3043481665498));
#19781=CARTESIAN_POINT('Ctrl Pts',(-7.48226341019648,0.260832642938422,
16.3168290997979));
#19782=CARTESIAN_POINT('Ctrl Pts',(-7.59019703546709,0.525433154239688,
16.3293100330461));
#19783=CARTESIAN_POINT('Ctrl Pts',(-7.77695120652459,0.714438148392672,
16.3417909662943));
#19784=CARTESIAN_POINT('Ctrl Pts',(-7.96370537758209,0.903443142545655,
16.3542718995425));
#19785=CARTESIAN_POINT('Ctrl Pts',(-8.2269938881474,1.01453885915635,16.3667528327907));
#19786=CARTESIAN_POINT('Ctrl Pts',(-8.49269364459069,1.01644874085988,16.3792337660389));
#19787=CARTESIAN_POINT('Ctrl Pts',(-8.75839340103398,1.01835862256341,16.3917146992871));
#19788=CARTESIAN_POINT('Ctrl Pts',(-9.02325176140304,0.91105928897946,16.4041956325353));
#19789=CARTESIAN_POINT('Ctrl Pts',(-9.21270367535773,0.724758509268141,
16.4166765657835));
#19790=CARTESIAN_POINT('Ctrl Pts',(-9.40215558931243,0.538457729556821,
16.4291574990316));
#19791=CARTESIAN_POINT('Ctrl Pts',(-9.51388182535815,0.275436159673279,
16.4416384322798));
#19792=CARTESIAN_POINT('Ctrl Pts',(-9.51642831724056,0.00974174196519902,
16.454119365528));
#19793=CARTESIAN_POINT('Ctrl Pts',(-9.51645943884197,0.00649459406745332,
16.4542718995425));
#19794=CARTESIAN_POINT('Ctrl Pts',(-9.516475,0.00324729703438987,16.454424433557));
#19795=CARTESIAN_POINT('Ctrl Pts',(-9.516475,8.69853826277193E-13,16.4545769675715));
#19796=CARTESIAN_POINT('Origin',(-8.5,0.,1.24542303242842));
#19797=CARTESIAN_POINT('',(-9.516475,7.41297233729117E-13,15.7954230324285));
#19798=CARTESIAN_POINT('',(-9.51632173115293,-4.86293170693105E-5,15.8545769675715));
#19799=CARTESIAN_POINT('',(-9.516475,1.78524650477582E-12,1.24542303242842));
#19800=CARTESIAN_POINT('Ctrl Pts',(-9.516475,7.41297233729117E-13,15.7954230324285));
#19801=CARTESIAN_POINT('Ctrl Pts',(-9.51647500000019,-0.265706620583227,
15.8079039656767));
#19802=CARTESIAN_POINT('Ctrl Pts',(-9.40727465387234,-0.529786878176479,
15.8203848989248));
#19803=CARTESIAN_POINT('Ctrl Pts',(-9.21961691907808,-0.717894780174347,
15.832865832173));
#19804=CARTESIAN_POINT('Ctrl Pts',(-9.03195918428382,-0.906002682172216,
15.8453467654212));
#19805=CARTESIAN_POINT('Ctrl Pts',(-8.76814132834426,-1.01583545019896,
15.8578276986694));
#19806=CARTESIAN_POINT('Ctrl Pts',(-8.50243547044551,-1.0164720823066,15.8703086319176));
#19807=CARTESIAN_POINT('Ctrl Pts',(-8.23672961254675,-1.01710871441423,
15.8827895651658));
#19808=CARTESIAN_POINT('Ctrl Pts',(-7.97238846933376,-0.908541417082997,
15.895270498414));
#19809=CARTESIAN_POINT('Ctrl Pts',(-7.78383148002372,-0.721334926798908,
15.9077514316622));
#19810=CARTESIAN_POINT('Ctrl Pts',(-7.59527449071368,-0.534128436514818,
15.9202323649104));
#19811=CARTESIAN_POINT('Ctrl Pts',(-7.48480993131715,-0.270574496756196,
15.9327132981586));
#19812=CARTESIAN_POINT('Ctrl Pts',(-7.48353667075686,-0.00487092690870812,
15.9451942314067));
#19813=CARTESIAN_POINT('Ctrl Pts',(-7.48226341019657,0.260832642938779,
15.9576751646549));
#19814=CARTESIAN_POINT('Ctrl Pts',(-7.59019703546728,0.525433154240028,
15.9701560979031));
#19815=CARTESIAN_POINT('Ctrl Pts',(-7.77695120652487,0.714438148392953,
15.9826370311513));
#19816=CARTESIAN_POINT('Ctrl Pts',(-7.96370537758245,0.903443142545878,
15.9951179643995));
#19817=CARTESIAN_POINT('Ctrl Pts',(-8.22699388814784,1.01453885915647,16.0075988976477));
#19818=CARTESIAN_POINT('Ctrl Pts',(-8.49269364459114,1.01644874085988,16.0200798308959));
#19819=CARTESIAN_POINT('Ctrl Pts',(-8.75839340103445,1.01835862256329,16.0325607641441));
#19820=CARTESIAN_POINT('Ctrl Pts',(-9.02325176140348,0.911059288979211,
16.0450416973923));
#19821=CARTESIAN_POINT('Ctrl Pts',(-9.2127036753581,0.724758509267782,16.0575226306405));
#19822=CARTESIAN_POINT('Ctrl Pts',(-9.40215558931271,0.538457729556354,
16.0700035638887));
#19823=CARTESIAN_POINT('Ctrl Pts',(-9.51388182535831,0.275436159672731,
16.0824844971368));
#19824=CARTESIAN_POINT('Ctrl Pts',(-9.51642831724057,0.00974174196463016,
16.094965430385));
#19825=CARTESIAN_POINT('Ctrl Pts',(-9.51645943884197,0.00649459406705778,
16.0951179643995));
#19826=CARTESIAN_POINT('Ctrl Pts',(-9.516475,0.00324729703416772,16.095270498414));
#19827=CARTESIAN_POINT('Ctrl Pts',(-9.516475,8.20993580306641E-13,16.0954230324285));
#19828=CARTESIAN_POINT('Ctrl Pts',(-9.51501971928355,-0.000461733140268747,
15.8545769675715));
#19829=CARTESIAN_POINT('Ctrl Pts',(-9.5155994996451,-0.140751556887071,
15.8611449975012));
#19830=CARTESIAN_POINT('Ctrl Pts',(-9.42291436670724,-0.620084892104978,
15.8836203685826));
#19831=CARTESIAN_POINT('Ctrl Pts',(-8.68981880352144,-1.18720590861504,
15.9220030808156));
#19832=CARTESIAN_POINT('Ctrl Pts',(-7.60428317324231,-0.801471685911831,
15.9697251042705));
#19833=CARTESIAN_POINT('Ctrl Pts',(-7.34085844261802,0.319812236206833,
16.0174471277253));
#19834=CARTESIAN_POINT('Ctrl Pts',(-8.14340243192267,1.1485135933495,16.0651691511802));
#19835=CARTESIAN_POINT('Ctrl Pts',(-9.08302755349385,0.958038040322845,
16.1049375040593));
#19836=CARTESIAN_POINT('Ctrl Pts',(-9.45854569172234,0.421593892220246,
16.134740109523));
#19837=CARTESIAN_POINT('Ctrl Pts',(-9.51681144570197,0.125735362396135,
16.1486353738352));
#19838=CARTESIAN_POINT('Ctrl Pts',(-9.51746519719392,-0.000451127041978173,
16.1545769675715));
#19839=CARTESIAN_POINT('Origin',(-8.5,0.,1.24542303242842));
#19840=CARTESIAN_POINT('',(-9.51673427260373,-1.76325846619593E-5,15.4954230324285));
#19841=CARTESIAN_POINT('',(-9.516475,7.46324614917698E-13,15.5545769675715));
#19842=CARTESIAN_POINT('',(-9.516475,1.78524650477582E-12,1.24542303242842));
#19843=CARTESIAN_POINT('Ctrl Pts',(-9.516475,7.77160715524671E-13,15.4954230324285));
#19844=CARTESIAN_POINT('Ctrl Pts',(-9.5164750000002,-0.265706620583192,
15.5079039656767));
#19845=CARTESIAN_POINT('Ctrl Pts',(-9.40727465387236,-0.529786878176447,
15.5203848989248));
#19846=CARTESIAN_POINT('Ctrl Pts',(-9.2196169190781,-0.717894780174322,
15.532865832173));
#19847=CARTESIAN_POINT('Ctrl Pts',(-9.03195918428385,-0.906002682172197,
15.5453467654212));
#19848=CARTESIAN_POINT('Ctrl Pts',(-8.7681413283443,-1.01583545019895,15.5578276986694));
#19849=CARTESIAN_POINT('Ctrl Pts',(-8.50243547044554,-1.0164720823066,15.5703086319176));
#19850=CARTESIAN_POINT('Ctrl Pts',(-8.23672961254679,-1.01710871441424,
15.5827895651658));
#19851=CARTESIAN_POINT('Ctrl Pts',(-7.97238846933379,-0.908541417083016,
15.595270498414));
#19852=CARTESIAN_POINT('Ctrl Pts',(-7.78383148002375,-0.721334926798933,
15.6077514316622));
#19853=CARTESIAN_POINT('Ctrl Pts',(-7.5952744907137,-0.53412843651485,15.6202323649104));
#19854=CARTESIAN_POINT('Ctrl Pts',(-7.48480993131716,-0.270574496756232,
15.6327132981586));
#19855=CARTESIAN_POINT('Ctrl Pts',(-7.48353667075686,-0.00487092690874399,
15.6451942314067));
#19856=CARTESIAN_POINT('Ctrl Pts',(-7.48226341019656,0.260832642938744,
15.6576751646549));
#19857=CARTESIAN_POINT('Ctrl Pts',(-7.59019703546726,0.525433154239996,
15.6701560979031));
#19858=CARTESIAN_POINT('Ctrl Pts',(-7.77695120652484,0.714438148392927,
15.6826370311513));
#19859=CARTESIAN_POINT('Ctrl Pts',(-7.96370537758242,0.903443142545859,
15.6951179643995));
#19860=CARTESIAN_POINT('Ctrl Pts',(-8.2269938881478,1.01453885915646,15.7075988976477));
#19861=CARTESIAN_POINT('Ctrl Pts',(-8.49269364459111,1.01644874085988,15.7200798308959));
#19862=CARTESIAN_POINT('Ctrl Pts',(-8.75839340103441,1.0183586225633,15.7325607641441));
#19863=CARTESIAN_POINT('Ctrl Pts',(-9.02325176140345,0.911059288979229,
15.7450416973923));
#19864=CARTESIAN_POINT('Ctrl Pts',(-9.21270367535807,0.724758509267807,
15.7575226306405));
#19865=CARTESIAN_POINT('Ctrl Pts',(-9.4021555893127,0.538457729556386,15.7700035638887));
#19866=CARTESIAN_POINT('Ctrl Pts',(-9.5138818253583,0.275436159672767,15.7824844971368));
#19867=CARTESIAN_POINT('Ctrl Pts',(-9.51642831724057,0.00974174196466602,
15.794965430385));
#19868=CARTESIAN_POINT('Ctrl Pts',(-9.51645943884197,0.00649459406705512,
15.7951179643995));
#19869=CARTESIAN_POINT('Ctrl Pts',(-9.516475,0.00324729703412654,15.795270498414));
#19870=CARTESIAN_POINT('Ctrl Pts',(-9.516475,7.41297233729117E-13,15.7954230324285));
#19871=CARTESIAN_POINT('Ctrl Pts',(-9.516475,8.04104529104238E-13,15.5545769675715));
#19872=CARTESIAN_POINT('Ctrl Pts',(-9.51647500000021,-0.265706620583184,
15.5670579008197));
#19873=CARTESIAN_POINT('Ctrl Pts',(-9.40727465387236,-0.529786878176461,
15.5795388340679));
#19874=CARTESIAN_POINT('Ctrl Pts',(-9.21961691907808,-0.717894780174344,
15.5920197673161));
#19875=CARTESIAN_POINT('Ctrl Pts',(-9.03195918428381,-0.906002682172227,
15.6045007005642));
#19876=CARTESIAN_POINT('Ctrl Pts',(-8.76814132834423,-1.01583545019898,
15.6169816338124));
#19877=CARTESIAN_POINT('Ctrl Pts',(-8.50243547044546,-1.0164720823066,15.6294625670606));
#19878=CARTESIAN_POINT('Ctrl Pts',(-8.23672961254668,-1.01710871441422,
15.6419435003088));
#19879=CARTESIAN_POINT('Ctrl Pts',(-7.97238846933367,-0.908541417082953,
15.654424433557));
#19880=CARTESIAN_POINT('Ctrl Pts',(-7.78383148002364,-0.72133492679883,
15.6669053668052));
#19881=CARTESIAN_POINT('Ctrl Pts',(-7.59527449071361,-0.534128436514707,
15.6793863000534));
#19882=CARTESIAN_POINT('Ctrl Pts',(-7.48480993131711,-0.270574496756047,
15.6918672333016));
#19883=CARTESIAN_POINT('Ctrl Pts',(-7.48353667075686,-0.00487092690853981,
15.7043481665498));
#19884=CARTESIAN_POINT('Ctrl Pts',(-7.48226341019661,0.260832642938967,
15.716829099798));
#19885=CARTESIAN_POINT('Ctrl Pts',(-7.59019703546738,0.525433154240217,
15.7293100330462));
#19886=CARTESIAN_POINT('Ctrl Pts',(-7.77695120652502,0.714438148393114,
15.7417909662944));
#19887=CARTESIAN_POINT('Ctrl Pts',(-7.96370537758267,0.903443142546011,
15.7542718995425));
#19888=CARTESIAN_POINT('Ctrl Pts',(-8.2269938881481,1.01453885915655,15.7667528327907));
#19889=CARTESIAN_POINT('Ctrl Pts',(-8.49269364459143,1.01644874085988,15.7792337660389));
#19890=CARTESIAN_POINT('Ctrl Pts',(-8.75839340103475,1.01835862256322,15.7917146992871));
#19891=CARTESIAN_POINT('Ctrl Pts',(-9.02325176140378,0.911059288979048,
15.8041956325353));
#19892=CARTESIAN_POINT('Ctrl Pts',(-9.21270367535834,0.724758509267543,
15.8166765657835));
#19893=CARTESIAN_POINT('Ctrl Pts',(-9.40215558931291,0.538457729556037,
15.8291574990317));
#19894=CARTESIAN_POINT('Ctrl Pts',(-9.51388182535841,0.275436159672352,
15.8416384322799));
#19895=CARTESIAN_POINT('Ctrl Pts',(-9.51642831724057,0.00974174196423075,
15.8541193655281));
#19896=CARTESIAN_POINT('Ctrl Pts',(-9.51645943884197,0.00649459406679317,
15.8542718995425));
#19897=CARTESIAN_POINT('Ctrl Pts',(-9.516475,0.00324729703403789,15.854424433557));
#19898=CARTESIAN_POINT('Ctrl Pts',(-9.516475,8.26020961495223E-13,15.8545769675715));
#19899=CARTESIAN_POINT('Origin',(-8.5,0.,1.24542303242842));
#19900=CARTESIAN_POINT('',(-9.516475,6.97464221793842E-13,15.1954230324285));
#19901=CARTESIAN_POINT('',(-9.516475,7.24408182526713E-13,15.2545769675715));
#19902=CARTESIAN_POINT('',(-9.516475,1.78524650477582E-12,1.24542303242842));
#19903=CARTESIAN_POINT('Ctrl Pts',(-9.51588249276368,-0.000783484411897156,
15.1954230324285));
#19904=CARTESIAN_POINT('Ctrl Pts',(-9.51674493951057,-0.10355898154087,
15.2002448852244));
#19905=CARTESIAN_POINT('Ctrl Pts',(-9.45513167617793,-0.544468194336532,
15.220974079172));
#19906=CARTESIAN_POINT('Ctrl Pts',(-8.81795958293278,-1.15983848287083,
15.2576106142711));
#19907=CARTESIAN_POINT('Ctrl Pts',(-7.88532479520075,-0.938000704162233,
15.2973789671502));
#19908=CARTESIAN_POINT('Ctrl Pts',(-7.50376303095584,-0.352302076284569,
15.3291936494535));
#19909=CARTESIAN_POINT('Ctrl Pts',(-7.43230033380396,0.343058292157666,
15.3610083317567));
#19910=CARTESIAN_POINT('Ctrl Pts',(-8.01814288331926,1.10187833907963,15.4007766846357));
#19911=CARTESIAN_POINT('Ctrl Pts',(-9.161100060691,1.0008324173858,15.4482328083849));
#19912=CARTESIAN_POINT('Ctrl Pts',(-9.51752766989334,0.331365264287844,
15.4797815909825));
#19913=CARTESIAN_POINT('Ctrl Pts',(-9.5180041082211,-0.000103991438988233,
15.4954230324285));
#19914=CARTESIAN_POINT('Ctrl Pts',(-9.516475,7.24408182526713E-13,15.2545769675715));
#19915=CARTESIAN_POINT('Ctrl Pts',(-9.51647500000019,-0.265706620583264,
15.2670579008197));
#19916=CARTESIAN_POINT('Ctrl Pts',(-9.40727465387231,-0.529786878176532,
15.2795388340679));
#19917=CARTESIAN_POINT('Ctrl Pts',(-9.21961691907802,-0.7178947801744,15.2920197673161));
#19918=CARTESIAN_POINT('Ctrl Pts',(-9.03195918428374,-0.906002682172269,
15.3045007005643));
#19919=CARTESIAN_POINT('Ctrl Pts',(-8.76814132834415,-1.015835450199,15.3169816338124));
#19920=CARTESIAN_POINT('Ctrl Pts',(-8.50243547044538,-1.0164720823066,15.3294625670606));
#19921=CARTESIAN_POINT('Ctrl Pts',(-8.2367296125466,-1.0171087144142,15.3419435003088));
#19922=CARTESIAN_POINT('Ctrl Pts',(-7.9723884693336,-0.908541417082912,
15.354424433557));
#19923=CARTESIAN_POINT('Ctrl Pts',(-7.78383148002359,-0.721334926798774,
15.3669053668052));
#19924=CARTESIAN_POINT('Ctrl Pts',(-7.59527449071357,-0.534128436514636,
15.3793863000534));
#19925=CARTESIAN_POINT('Ctrl Pts',(-7.48480993131709,-0.270574496755967,
15.3918672333016));
#19926=CARTESIAN_POINT('Ctrl Pts',(-7.48353667075686,-0.00487092690846012,
15.4043481665498));
#19927=CARTESIAN_POINT('Ctrl Pts',(-7.48226341019663,0.260832642939047,
15.416829099798));
#19928=CARTESIAN_POINT('Ctrl Pts',(-7.59019703546742,0.525433154240288,
15.4293100330462));
#19929=CARTESIAN_POINT('Ctrl Pts',(-7.77695120652508,0.71443814839317,15.4417909662944));
#19930=CARTESIAN_POINT('Ctrl Pts',(-7.96370537758274,0.903443142546053,
15.4542718995426));
#19931=CARTESIAN_POINT('Ctrl Pts',(-8.22699388814818,1.01453885915657,15.4667528327907));
#19932=CARTESIAN_POINT('Ctrl Pts',(-8.49269364459151,1.01644874085988,15.4792337660389));
#19933=CARTESIAN_POINT('Ctrl Pts',(-8.75839340103483,1.0183586225632,15.4917146992871));
#19934=CARTESIAN_POINT('Ctrl Pts',(-9.02325176140385,0.911059288979007,
15.5041956325353));
#19935=CARTESIAN_POINT('Ctrl Pts',(-9.2127036753584,0.724758509267487,15.5166765657835));
#19936=CARTESIAN_POINT('Ctrl Pts',(-9.40215558931295,0.538457729555966,
15.5291574990317));
#19937=CARTESIAN_POINT('Ctrl Pts',(-9.51388182535844,0.275436159672272,
15.5416384322799));
#19938=CARTESIAN_POINT('Ctrl Pts',(-9.51642831724057,0.00974174196415106,
15.5541193655281));
#19939=CARTESIAN_POINT('Ctrl Pts',(-9.51645943884197,0.00649459406673273,
15.5542718995425));
#19940=CARTESIAN_POINT('Ctrl Pts',(-9.516475,0.00324729703399675,15.554424433557));
#19941=CARTESIAN_POINT('Ctrl Pts',(-9.516475,8.04104529104238E-13,15.5545769675715));
#19942=CARTESIAN_POINT('Origin',(-8.5,0.,1.24542303242842));
#19943=CARTESIAN_POINT('',(-9.516475,6.75547936556161E-13,14.8954230324285));
#19944=CARTESIAN_POINT('',(-9.516475,7.02491750135728E-13,14.9545769675715));
#19945=CARTESIAN_POINT('',(-9.516475,1.78524650477582E-12,1.24542303242842));
#19946=CARTESIAN_POINT('Ctrl Pts',(-9.516475,6.75547936556161E-13,14.8954230324285));
#19947=CARTESIAN_POINT('Ctrl Pts',(-9.51647500000018,-0.265706620583293,
14.9079039656767));
#19948=CARTESIAN_POINT('Ctrl Pts',(-9.4072746538723,-0.529786878176537,
14.9203848989248));
#19949=CARTESIAN_POINT('Ctrl Pts',(-9.21961691907803,-0.717894780174394,
14.932865832173));
#19950=CARTESIAN_POINT('Ctrl Pts',(-9.03195918428376,-0.90600268217225,
14.9453467654212));
#19951=CARTESIAN_POINT('Ctrl Pts',(-8.76814132834419,-1.01583545019898,
14.9578276986694));
#19952=CARTESIAN_POINT('Ctrl Pts',(-8.50243547044544,-1.0164720823066,14.9703086319176));
#19953=CARTESIAN_POINT('Ctrl Pts',(-8.23672961254669,-1.01710871441421,
14.9827895651658));
#19954=CARTESIAN_POINT('Ctrl Pts',(-7.9723884693337,-0.908541417082963,
14.995270498414));
#19955=CARTESIAN_POINT('Ctrl Pts',(-7.78383148002367,-0.721334926798861,
15.0077514316622));
#19956=CARTESIAN_POINT('Ctrl Pts',(-7.59527449071365,-0.53412843651476,
15.0202323649104));
#19957=CARTESIAN_POINT('Ctrl Pts',(-7.48480993131714,-0.27057449675613,
15.0327132981586));
#19958=CARTESIAN_POINT('Ctrl Pts',(-7.48353667075686,-0.00487092690864238,
15.0451942314068));
#19959=CARTESIAN_POINT('Ctrl Pts',(-7.48226341019658,0.260832642938845,
15.0576751646549));
#19960=CARTESIAN_POINT('Ctrl Pts',(-7.59019703546731,0.525433154240087,
15.0701560979031));
#19961=CARTESIAN_POINT('Ctrl Pts',(-7.77695120652491,0.714438148393,15.0826370311513));
#19962=CARTESIAN_POINT('Ctrl Pts',(-7.96370537758251,0.903443142545912,
15.0951179643995));
#19963=CARTESIAN_POINT('Ctrl Pts',(-8.2269938881479,1.01453885915649,15.1075988976477));
#19964=CARTESIAN_POINT('Ctrl Pts',(-8.49269364459121,1.01644874085988,15.1200798308959));
#19965=CARTESIAN_POINT('Ctrl Pts',(-8.75839340103451,1.01835862256327,15.1325607641441));
#19966=CARTESIAN_POINT('Ctrl Pts',(-9.02325176140354,0.911059288979177,
15.1450416973923));
#19967=CARTESIAN_POINT('Ctrl Pts',(-9.21270367535815,0.724758509267736,
15.1575226306405));
#19968=CARTESIAN_POINT('Ctrl Pts',(-9.40215558931275,0.538457729556296,
15.1700035638887));
#19969=CARTESIAN_POINT('Ctrl Pts',(-9.51388182535832,0.275436159672665,
15.1824844971368));
#19970=CARTESIAN_POINT('Ctrl Pts',(-9.51642831724057,0.00974174196456442,
15.194965430385));
#19971=CARTESIAN_POINT('Ctrl Pts',(-9.51645943884197,0.00649459406697277,
15.1951179643995));
#19972=CARTESIAN_POINT('Ctrl Pts',(-9.516475,0.0032472970340634,15.195270498414));
#19973=CARTESIAN_POINT('Ctrl Pts',(-9.516475,6.97464368947146E-13,15.1954230324285));
#19974=CARTESIAN_POINT('Ctrl Pts',(-9.516475,8.18051578508808E-13,14.9545769675715));
#19975=CARTESIAN_POINT('Ctrl Pts',(-9.51647500000021,-0.265706620583151,
14.9670579008197));
#19976=CARTESIAN_POINT('Ctrl Pts',(-9.40727465387238,-0.52978687817641,
14.9795388340679));
#19977=CARTESIAN_POINT('Ctrl Pts',(-9.21961691907813,-0.717894780174293,
14.9920197673161));
#19978=CARTESIAN_POINT('Ctrl Pts',(-9.03195918428389,-0.906002682172176,
15.0045007005642));
#19979=CARTESIAN_POINT('Ctrl Pts',(-8.76814132834434,-1.01583545019894,
15.0169816338124));
#19980=CARTESIAN_POINT('Ctrl Pts',(-8.50243547044558,-1.0164720823066,15.0294625670606));
#19981=CARTESIAN_POINT('Ctrl Pts',(-8.23672961254683,-1.01710871441425,
15.0419435003088));
#19982=CARTESIAN_POINT('Ctrl Pts',(-7.97238846933383,-0.908541417083037,
15.054424433557));
#19983=CARTESIAN_POINT('Ctrl Pts',(-7.78383148002378,-0.721334926798962,
15.0669053668052));
#19984=CARTESIAN_POINT('Ctrl Pts',(-7.59527449071372,-0.534128436514887,
15.0793863000534));
#19985=CARTESIAN_POINT('Ctrl Pts',(-7.48480993131717,-0.270574496756272,
15.0918672333016));
#19986=CARTESIAN_POINT('Ctrl Pts',(-7.48353667075686,-0.00487092690878488,
15.1043481665498));
#19987=CARTESIAN_POINT('Ctrl Pts',(-7.48226341019655,0.260832642938703,
15.116829099798));
#19988=CARTESIAN_POINT('Ctrl Pts',(-7.59019703546724,0.52543315423996,15.1293100330462));
#19989=CARTESIAN_POINT('Ctrl Pts',(-7.77695120652481,0.714438148392898,
15.1417909662943));
#19990=CARTESIAN_POINT('Ctrl Pts',(-7.96370537758238,0.903443142545837,
15.1542718995425));
#19991=CARTESIAN_POINT('Ctrl Pts',(-8.22699388814776,1.01453885915645,15.1667528327907));
#19992=CARTESIAN_POINT('Ctrl Pts',(-8.49269364459107,1.01644874085988,15.1792337660389));
#19993=CARTESIAN_POINT('Ctrl Pts',(-8.75839340103437,1.01835862256331,15.1917146992871));
#19994=CARTESIAN_POINT('Ctrl Pts',(-9.02325176140341,0.91105928897925,15.2041956325353));
#19995=CARTESIAN_POINT('Ctrl Pts',(-9.21270367535804,0.724758509267836,
15.2166765657835));
#19996=CARTESIAN_POINT('Ctrl Pts',(-9.40215558931267,0.538457729556422,
15.2291574990317));
#19997=CARTESIAN_POINT('Ctrl Pts',(-9.51388182535828,0.275436159672807,
15.2416384322799));
#19998=CARTESIAN_POINT('Ctrl Pts',(-9.51642831724057,0.00974174196470691,
15.2541193655281));
#19999=CARTESIAN_POINT('Ctrl Pts',(-9.51645943884197,0.00649459406707676,
15.2542718995425));
#20000=CARTESIAN_POINT('Ctrl Pts',(-9.516475,0.00324729703412887,15.254424433557));
#20001=CARTESIAN_POINT('Ctrl Pts',(-9.516475,7.24408182526713E-13,15.2545769675715));
#20002=CARTESIAN_POINT('Origin',(-8.5,0.,1.24542303242842));
#20003=CARTESIAN_POINT('',(-9.516475,6.53631504165176E-13,14.5954230324285));
#20004=CARTESIAN_POINT('',(-9.516475,6.80575317744743E-13,14.6545769675715));
#20005=CARTESIAN_POINT('',(-9.516475,1.78524650477582E-12,1.24542303242842));
#20006=CARTESIAN_POINT('Ctrl Pts',(-9.516475,7.11411418351716E-13,14.5954230324285));
#20007=CARTESIAN_POINT('Ctrl Pts',(-9.51647500000019,-0.265706620583277,
14.6079039656767));
#20008=CARTESIAN_POINT('Ctrl Pts',(-9.40727465387231,-0.529786878176543,
14.6203848989248));
#20009=CARTESIAN_POINT('Ctrl Pts',(-9.21961691907802,-0.717894780174409,
14.632865832173));
#20010=CARTESIAN_POINT('Ctrl Pts',(-9.03195918428372,-0.906002682172275,
14.6453467654212));
#20011=CARTESIAN_POINT('Ctrl Pts',(-8.76814132834414,-1.015835450199,14.6578276986694));
#20012=CARTESIAN_POINT('Ctrl Pts',(-8.50243547044536,-1.0164720823066,14.6703086319176));
#20013=CARTESIAN_POINT('Ctrl Pts',(-8.23672961254659,-1.01710871441419,
14.6827895651658));
#20014=CARTESIAN_POINT('Ctrl Pts',(-7.97238846933359,-0.908541417082905,
14.695270498414));
#20015=CARTESIAN_POINT('Ctrl Pts',(-7.78383148002358,-0.721334926798765,
14.7077514316622));
#20016=CARTESIAN_POINT('Ctrl Pts',(-7.59527449071356,-0.534128436514624,
14.7202323649104));
#20017=CARTESIAN_POINT('Ctrl Pts',(-7.48480993131708,-0.270574496755954,
14.7327132981586));
#20018=CARTESIAN_POINT('Ctrl Pts',(-7.48353667075686,-0.00487092690844712,
14.7451942314068));
#20019=CARTESIAN_POINT('Ctrl Pts',(-7.48226341019663,0.26083264293906,14.757675164655));
#20020=CARTESIAN_POINT('Ctrl Pts',(-7.59019703546743,0.5254331542403,14.7701560979031));
#20021=CARTESIAN_POINT('Ctrl Pts',(-7.77695120652509,0.71443814839318,14.7826370311513));
#20022=CARTESIAN_POINT('Ctrl Pts',(-7.96370537758275,0.903443142546059,
14.7951179643995));
#20023=CARTESIAN_POINT('Ctrl Pts',(-8.22699388814819,1.01453885915657,14.8075988976477));
#20024=CARTESIAN_POINT('Ctrl Pts',(-8.49269364459152,1.01644874085988,14.8200798308959));
#20025=CARTESIAN_POINT('Ctrl Pts',(-8.75839340103484,1.0183586225632,14.8325607641441));
#20026=CARTESIAN_POINT('Ctrl Pts',(-9.02325176140386,0.911059288979001,
14.8450416973923));
#20027=CARTESIAN_POINT('Ctrl Pts',(-9.21270367535841,0.724758509267478,
14.8575226306405));
#20028=CARTESIAN_POINT('Ctrl Pts',(-9.40215558931296,0.538457729555955,
14.8700035638887));
#20029=CARTESIAN_POINT('Ctrl Pts',(-9.51388182535844,0.275436159672259,
14.8824844971369));
#20030=CARTESIAN_POINT('Ctrl Pts',(-9.51642831724057,0.00974174196413806,
14.8949654303851));
#20031=CARTESIAN_POINT('Ctrl Pts',(-9.51645943884197,0.00649459406668122,
14.8951179643995));
#20032=CARTESIAN_POINT('Ctrl Pts',(-9.516475,0.00324729703390672,14.895270498414));
#20033=CARTESIAN_POINT('Ctrl Pts',(-9.516475,6.75547936556161E-13,14.8954230324285));
#20034=CARTESIAN_POINT('Ctrl Pts',(-9.516475,6.80575317744743E-13,14.6545769675715));
#20035=CARTESIAN_POINT('Ctrl Pts',(-9.51647500000018,-0.265706620583288,
14.6670579008197));
#20036=CARTESIAN_POINT('Ctrl Pts',(-9.40727465387231,-0.529786878176533,
14.6795388340679));
#20037=CARTESIAN_POINT('Ctrl Pts',(-9.21961691907804,-0.71789478017439,
14.6920197673161));
#20038=CARTESIAN_POINT('Ctrl Pts',(-9.03195918428376,-0.906002682172248,
14.7045007005643));
#20039=CARTESIAN_POINT('Ctrl Pts',(-8.7681413283442,-1.01583545019898,14.7169816338124));
#20040=CARTESIAN_POINT('Ctrl Pts',(-8.50243547044545,-1.0164720823066,14.7294625670606));
#20041=CARTESIAN_POINT('Ctrl Pts',(-8.23672961254669,-1.01710871441422,
14.7419435003088));
#20042=CARTESIAN_POINT('Ctrl Pts',(-7.97238846933371,-0.908541417082965,
14.754424433557));
#20043=CARTESIAN_POINT('Ctrl Pts',(-7.78383148002368,-0.721334926798865,
14.7669053668052));
#20044=CARTESIAN_POINT('Ctrl Pts',(-7.59527449071365,-0.534128436514764,
14.7793863000534));
#20045=CARTESIAN_POINT('Ctrl Pts',(-7.48480993131714,-0.270574496756135,
14.7918672333016));
#20046=CARTESIAN_POINT('Ctrl Pts',(-7.48353667075686,-0.0048709269086474,
14.8043481665498));
#20047=CARTESIAN_POINT('Ctrl Pts',(-7.48226341019658,0.26083264293884,14.816829099798));
#20048=CARTESIAN_POINT('Ctrl Pts',(-7.59019703546731,0.525433154240083,
14.8293100330462));
#20049=CARTESIAN_POINT('Ctrl Pts',(-7.77695120652491,0.714438148392996,
14.8417909662943));
#20050=CARTESIAN_POINT('Ctrl Pts',(-7.9637053775825,0.90344314254591,14.8542718995425));
#20051=CARTESIAN_POINT('Ctrl Pts',(-8.2269938881479,1.01453885915649,14.8667528327907));
#20052=CARTESIAN_POINT('Ctrl Pts',(-8.4926936445912,1.01644874085988,14.8792337660389));
#20053=CARTESIAN_POINT('Ctrl Pts',(-8.75839340103451,1.01835862256328,14.8917146992871));
#20054=CARTESIAN_POINT('Ctrl Pts',(-9.02325176140354,0.91105928897918,14.9041956325353));
#20055=CARTESIAN_POINT('Ctrl Pts',(-9.21270367535814,0.72475850926774,14.9166765657835));
#20056=CARTESIAN_POINT('Ctrl Pts',(-9.40215558931275,0.5384577295563,14.9291574990317));
#20057=CARTESIAN_POINT('Ctrl Pts',(-9.51388182535832,0.27543615967267,14.9416384322799));
#20058=CARTESIAN_POINT('Ctrl Pts',(-9.51642831724057,0.00974174196456944,
14.9541193655281));
#20059=CARTESIAN_POINT('Ctrl Pts',(-9.51645943884197,0.00649459406701632,
14.9542718995425));
#20060=CARTESIAN_POINT('Ctrl Pts',(-9.516475,0.00324729703414547,14.954424433557));
#20061=CARTESIAN_POINT('Ctrl Pts',(-9.516475,8.18051578508808E-13,14.9545769675715));
#20062=CARTESIAN_POINT('Origin',(-8.5,0.,1.24542303242842));
#20063=CARTESIAN_POINT('',(-9.516475,6.31715071774191E-13,14.2954230324285));
#20064=CARTESIAN_POINT('',(-9.516475,6.58658885353758E-13,14.3545769675715));
#20065=CARTESIAN_POINT('',(-9.516475,1.78524650477582E-12,1.24542303242842));
#20066=CARTESIAN_POINT('Ctrl Pts',(-9.516475,6.31715071774191E-13,14.2954230324285));
#20067=CARTESIAN_POINT('Ctrl Pts',(-9.51647500000016,-0.265706620583337,
14.3079039656767));
#20068=CARTESIAN_POINT('Ctrl Pts',(-9.40727465387228,-0.529786878176576,
14.3203848989248));
#20069=CARTESIAN_POINT('Ctrl Pts',(-9.219616919078,-0.717894780174425,14.332865832173));
#20070=CARTESIAN_POINT('Ctrl Pts',(-9.03195918428372,-0.906002682172273,
14.3453467654212));
#20071=CARTESIAN_POINT('Ctrl Pts',(-8.76814132834415,-1.01583545019899,
14.3578276986694));
#20072=CARTESIAN_POINT('Ctrl Pts',(-8.5024354704454,-1.0164720823066,14.3703086319176));
#20073=CARTESIAN_POINT('Ctrl Pts',(-8.23672961254664,-1.0171087144142,14.3827895651658));
#20074=CARTESIAN_POINT('Ctrl Pts',(-7.97238846933366,-0.90854141708294,
14.395270498414));
#20075=CARTESIAN_POINT('Ctrl Pts',(-7.78383148002364,-0.72133492679883,
14.4077514316622));
#20076=CARTESIAN_POINT('Ctrl Pts',(-7.59527449071362,-0.534128436514721,
14.4202323649104));
#20077=CARTESIAN_POINT('Ctrl Pts',(-7.48480993131712,-0.270574496756086,
14.4327132981586));
#20078=CARTESIAN_POINT('Ctrl Pts',(-7.48353667075686,-0.00487092690859854,
14.4451942314068));
#20079=CARTESIAN_POINT('Ctrl Pts',(-7.48226341019659,0.260832642938889,
14.4576751646549));
#20080=CARTESIAN_POINT('Ctrl Pts',(-7.59019703546734,0.525433154240126,
14.4701560979031));
#20081=CARTESIAN_POINT('Ctrl Pts',(-7.77695120652494,0.714438148393031,
14.4826370311513));
#20082=CARTESIAN_POINT('Ctrl Pts',(-7.96370537758255,0.903443142545935,
14.4951179643995));
#20083=CARTESIAN_POINT('Ctrl Pts',(-8.22699388814795,1.0145388591565,14.5075988976477));
#20084=CARTESIAN_POINT('Ctrl Pts',(-8.49269364459125,1.01644874085988,14.5200798308959));
#20085=CARTESIAN_POINT('Ctrl Pts',(-8.75839340103456,1.01835862256326,14.5325607641441));
#20086=CARTESIAN_POINT('Ctrl Pts',(-9.02325176140358,0.911059288979154,
14.5450416973923));
#20087=CARTESIAN_POINT('Ctrl Pts',(-9.21270367535818,0.724758509267706,
14.5575226306405));
#20088=CARTESIAN_POINT('Ctrl Pts',(-9.40215558931277,0.538457729556257,
14.5700035638887));
#20089=CARTESIAN_POINT('Ctrl Pts',(-9.51388182535834,0.275436159672622,
14.5824844971368));
#20090=CARTESIAN_POINT('Ctrl Pts',(-9.51642831724057,0.00974174196452058,
14.594965430385));
#20091=CARTESIAN_POINT('Ctrl Pts',(-9.51645943884197,0.0064945940669482,
14.5951179643995));
#20092=CARTESIAN_POINT('Ctrl Pts',(-9.516475,0.00324729703405813,14.595270498414));
#20093=CARTESIAN_POINT('Ctrl Pts',(-9.516475,7.11411418351716E-13,14.5954230324285));
#20094=CARTESIAN_POINT('Ctrl Pts',(-9.516475,7.16438799540298E-13,14.3545769675715));
#20095=CARTESIAN_POINT('Ctrl Pts',(-9.51647500000019,-0.265706620583272,
14.3670579008197));
#20096=CARTESIAN_POINT('Ctrl Pts',(-9.40727465387231,-0.529786878176539,
14.3795388340679));
#20097=CARTESIAN_POINT('Ctrl Pts',(-9.21961691907802,-0.717894780174406,
14.3920197673161));
#20098=CARTESIAN_POINT('Ctrl Pts',(-9.03195918428373,-0.906002682172273,
14.4045007005643));
#20099=CARTESIAN_POINT('Ctrl Pts',(-8.76814132834414,-1.015835450199,14.4169816338124));
#20100=CARTESIAN_POINT('Ctrl Pts',(-8.50243547044537,-1.0164720823066,14.4294625670606));
#20101=CARTESIAN_POINT('Ctrl Pts',(-8.23672961254659,-1.0171087144142,14.4419435003088));
#20102=CARTESIAN_POINT('Ctrl Pts',(-7.9723884693336,-0.908541417082908,
14.454424433557));
#20103=CARTESIAN_POINT('Ctrl Pts',(-7.78383148002358,-0.721334926798768,
14.4669053668052));
#20104=CARTESIAN_POINT('Ctrl Pts',(-7.59527449071356,-0.534128436514628,
14.4793863000534));
#20105=CARTESIAN_POINT('Ctrl Pts',(-7.48480993131709,-0.270574496755959,
14.4918672333016));
#20106=CARTESIAN_POINT('Ctrl Pts',(-7.48353667075686,-0.00487092690845215,
14.5043481665498));
#20107=CARTESIAN_POINT('Ctrl Pts',(-7.48226341019663,0.260832642939055,
14.516829099798));
#20108=CARTESIAN_POINT('Ctrl Pts',(-7.59019703546743,0.525433154240295,
14.5293100330462));
#20109=CARTESIAN_POINT('Ctrl Pts',(-7.77695120652509,0.714438148393176,
14.5417909662944));
#20110=CARTESIAN_POINT('Ctrl Pts',(-7.96370537758274,0.903443142546057,
14.5542718995425));
#20111=CARTESIAN_POINT('Ctrl Pts',(-8.22699388814819,1.01453885915657,14.5667528327907));
#20112=CARTESIAN_POINT('Ctrl Pts',(-8.49269364459151,1.01644874085988,14.5792337660389));
#20113=CARTESIAN_POINT('Ctrl Pts',(-8.75839340103484,1.0183586225632,14.5917146992871));
#20114=CARTESIAN_POINT('Ctrl Pts',(-9.02325176140386,0.911059288979003,
14.6041956325353));
#20115=CARTESIAN_POINT('Ctrl Pts',(-9.21270367535841,0.724758509267481,
14.6166765657835));
#20116=CARTESIAN_POINT('Ctrl Pts',(-9.40215558931295,0.538457729555959,
14.6291574990317));
#20117=CARTESIAN_POINT('Ctrl Pts',(-9.51388182535844,0.275436159672264,
14.6416384322799));
#20118=CARTESIAN_POINT('Ctrl Pts',(-9.51642831724057,0.00974174196414309,
14.6541193655281));
#20119=CARTESIAN_POINT('Ctrl Pts',(-9.51645943884197,0.00649459406668624,
14.6542718995426));
#20120=CARTESIAN_POINT('Ctrl Pts',(-9.516475,0.00324729703391174,14.654424433557));
#20121=CARTESIAN_POINT('Ctrl Pts',(-9.516475,6.80575317744743E-13,14.6545769675715));
#20122=CARTESIAN_POINT('Origin',(-8.5,0.,1.24542303242842));
#20123=CARTESIAN_POINT('',(-9.516475,6.09798639383206E-13,13.9954230324285));
#20124=CARTESIAN_POINT('',(-9.51650473276395,-2.35768713140684E-5,14.0545769675715));
#20125=CARTESIAN_POINT('',(-9.516475,1.78524650477582E-12,1.24542303242842));
#20126=CARTESIAN_POINT('Ctrl Pts',(-9.516475,6.67578553569746E-13,13.9954230324285));
#20127=CARTESIAN_POINT('Ctrl Pts',(-9.51647500000017,-0.265706620583301,
14.0079039656767));
#20128=CARTESIAN_POINT('Ctrl Pts',(-9.4072746538723,-0.529786878176544,
14.0203848989248));
#20129=CARTESIAN_POINT('Ctrl Pts',(-9.21961691907803,-0.717894780174399,
14.032865832173));
#20130=CARTESIAN_POINT('Ctrl Pts',(-9.03195918428375,-0.906002682172254,
14.0453467654212));
#20131=CARTESIAN_POINT('Ctrl Pts',(-8.76814132834419,-1.01583545019898,
14.0578276986694));
#20132=CARTESIAN_POINT('Ctrl Pts',(-8.50243547044543,-1.0164720823066,14.0703086319176));
#20133=CARTESIAN_POINT('Ctrl Pts',(-8.23672961254668,-1.01710871441421,
14.0827895651658));
#20134=CARTESIAN_POINT('Ctrl Pts',(-7.9723884693337,-0.908541417082959,
14.095270498414));
#20135=CARTESIAN_POINT('Ctrl Pts',(-7.78383148002367,-0.721334926798856,
14.1077514316622));
#20136=CARTESIAN_POINT('Ctrl Pts',(-7.59527449071364,-0.534128436514753,
14.1202323649104));
#20137=CARTESIAN_POINT('Ctrl Pts',(-7.48480993131713,-0.270574496756122,
14.1327132981586));
#20138=CARTESIAN_POINT('Ctrl Pts',(-7.48353667075686,-0.0048709269086344,
14.1451942314067));
#20139=CARTESIAN_POINT('Ctrl Pts',(-7.48226341019658,0.260832642938853,
14.1576751646549));
#20140=CARTESIAN_POINT('Ctrl Pts',(-7.59019703546732,0.525433154240094,
14.1701560979031));
#20141=CARTESIAN_POINT('Ctrl Pts',(-7.77695120652492,0.714438148393005,
14.1826370311513));
#20142=CARTESIAN_POINT('Ctrl Pts',(-7.96370537758252,0.903443142545917,
14.1951179643995));
#20143=CARTESIAN_POINT('Ctrl Pts',(-8.22699388814791,1.01453885915649,14.2075988976477));
#20144=CARTESIAN_POINT('Ctrl Pts',(-8.49269364459122,1.01644874085988,14.2200798308959));
#20145=CARTESIAN_POINT('Ctrl Pts',(-8.75839340103452,1.01835862256327,14.2325607641441));
#20146=CARTESIAN_POINT('Ctrl Pts',(-9.02325176140355,0.911059288979173,
14.2450416973923));
#20147=CARTESIAN_POINT('Ctrl Pts',(-9.21270367535815,0.724758509267731,
14.2575226306405));
#20148=CARTESIAN_POINT('Ctrl Pts',(-9.40215558931275,0.538457729556288,
14.2700035638887));
#20149=CARTESIAN_POINT('Ctrl Pts',(-9.51388182535833,0.275436159672657,
14.2824844971368));
#20150=CARTESIAN_POINT('Ctrl Pts',(-9.51642831724057,0.00974174196455645,
14.294965430385));
#20151=CARTESIAN_POINT('Ctrl Pts',(-9.51645943884197,0.00649459406694554,
14.2951179643995));
#20152=CARTESIAN_POINT('Ctrl Pts',(-9.516475,0.00324729703401696,14.295270498414));
#20153=CARTESIAN_POINT('Ctrl Pts',(-9.516475,6.31715071774191E-13,14.2954230324285));
#20154=CARTESIAN_POINT('Ctrl Pts',(-9.516475,6.36742452962773E-13,14.0545769675715));
#20155=CARTESIAN_POINT('Ctrl Pts',(-9.51647500000017,-0.265706620583313,
14.0670579008197));
#20156=CARTESIAN_POINT('Ctrl Pts',(-9.4072746538723,-0.529786878176534,
14.0795388340679));
#20157=CARTESIAN_POINT('Ctrl Pts',(-9.21961691907805,-0.71789478017438,
14.0920197673161));
#20158=CARTESIAN_POINT('Ctrl Pts',(-9.03195918428379,-0.906002682172227,
14.1045007005642));
#20159=CARTESIAN_POINT('Ctrl Pts',(-8.76814132834425,-1.01583545019896,
14.1169816338124));
#20160=CARTESIAN_POINT('Ctrl Pts',(-8.50243547044552,-1.0164720823066,14.1294625670606));
#20161=CARTESIAN_POINT('Ctrl Pts',(-8.23672961254679,-1.01710871441423,
14.1419435003088));
#20162=CARTESIAN_POINT('Ctrl Pts',(-7.97238846933381,-0.908541417083019,
14.154424433557));
#20163=CARTESIAN_POINT('Ctrl Pts',(-7.78383148002377,-0.721334926798956,
14.1669053668052));
#20164=CARTESIAN_POINT('Ctrl Pts',(-7.59527449071373,-0.534128436514893,
14.1793863000534));
#20165=CARTESIAN_POINT('Ctrl Pts',(-7.48480993131719,-0.270574496756303,
14.1918672333016));
#20166=CARTESIAN_POINT('Ctrl Pts',(-7.48353667075686,-0.00487092690883469,
14.2043481665498));
#20167=CARTESIAN_POINT('Ctrl Pts',(-7.48226341019653,0.260832642938633,
14.216829099798));
#20168=CARTESIAN_POINT('Ctrl Pts',(-7.5901970354672,0.525433154239877,14.2293100330461));
#20169=CARTESIAN_POINT('Ctrl Pts',(-7.77695120652474,0.714438148392822,
14.2417909662943));
#20170=CARTESIAN_POINT('Ctrl Pts',(-7.96370537758227,0.903443142545767,
14.2542718995425));
#20171=CARTESIAN_POINT('Ctrl Pts',(-8.22699388814761,1.01453885915641,14.2667528327907));
#20172=CARTESIAN_POINT('Ctrl Pts',(-8.4926936445909,1.01644874085988,14.2792337660389));
#20173=CARTESIAN_POINT('Ctrl Pts',(-8.75839340103419,1.01835862256335,14.2917146992871));
#20174=CARTESIAN_POINT('Ctrl Pts',(-9.02325176140323,0.911059288979352,
14.3041956325353));
#20175=CARTESIAN_POINT('Ctrl Pts',(-9.21270367535788,0.724758509267993,
14.3166765657835));
#20176=CARTESIAN_POINT('Ctrl Pts',(-9.40215558931254,0.538457729556634,
14.3291574990317));
#20177=CARTESIAN_POINT('Ctrl Pts',(-9.51388182535821,0.275436159673068,
14.3416384322799));
#20178=CARTESIAN_POINT('Ctrl Pts',(-9.51642831724057,0.00974174196498783,
14.354119365528));
#20179=CARTESIAN_POINT('Ctrl Pts',(-9.51645943884197,0.00649459406726139,
14.3542718995425));
#20180=CARTESIAN_POINT('Ctrl Pts',(-9.516475,0.00324729703421724,14.354424433557));
#20181=CARTESIAN_POINT('Ctrl Pts',(-9.516475,7.16438799540298E-13,14.3545769675715));
#20182=CARTESIAN_POINT('Origin',(-8.5,0.,1.24542303242842));
#20183=CARTESIAN_POINT('',(-9.516475,5.87882206992221E-13,13.6954230324285));
#20184=CARTESIAN_POINT('',(-9.51614186447112,-9.25009508935906E-5,13.7545769675715));
#20185=CARTESIAN_POINT('',(-9.516475,1.78524650477582E-12,1.24542303242842));
#20186=CARTESIAN_POINT('Ctrl Pts',(-9.516475,5.87882206992221E-13,13.6954230324285));
#20187=CARTESIAN_POINT('Ctrl Pts',(-9.51647500000015,-0.265706620583381,
13.7079039656767));
#20188=CARTESIAN_POINT('Ctrl Pts',(-9.40727465387226,-0.529786878176616,
13.7203848989249));
#20189=CARTESIAN_POINT('Ctrl Pts',(-9.21961691907797,-0.717894780174456,
13.732865832173));
#20190=CARTESIAN_POINT('Ctrl Pts',(-9.03195918428368,-0.906002682172296,
13.7453467654212));
#20191=CARTESIAN_POINT('Ctrl Pts',(-8.76814132834411,-1.015835450199,13.7578276986694));
#20192=CARTESIAN_POINT('Ctrl Pts',(-8.50243547044535,-1.0164720823066,13.7703086319176));
#20193=CARTESIAN_POINT('Ctrl Pts',(-8.2367296125466,-1.01710871441419,13.7827895651658));
#20194=CARTESIAN_POINT('Ctrl Pts',(-7.97238846933362,-0.908541417082917,
13.795270498414));
#20195=CARTESIAN_POINT('Ctrl Pts',(-7.78383148002361,-0.7213349267988,13.8077514316622));
#20196=CARTESIAN_POINT('Ctrl Pts',(-7.5952744907136,-0.534128436514682,
13.8202323649104));
#20197=CARTESIAN_POINT('Ctrl Pts',(-7.48480993131711,-0.270574496756043,
13.8327132981586));
#20198=CARTESIAN_POINT('Ctrl Pts',(-7.48353667075686,-0.00487092690855471,
13.8451942314068));
#20199=CARTESIAN_POINT('Ctrl Pts',(-7.48226341019661,0.260832642938933,
13.8576751646549));
#20200=CARTESIAN_POINT('Ctrl Pts',(-7.59019703546736,0.525433154240165,
13.8701560979031));
#20201=CARTESIAN_POINT('Ctrl Pts',(-7.77695120652497,0.714438148393062,
13.8826370311513));
#20202=CARTESIAN_POINT('Ctrl Pts',(-7.96370537758259,0.903443142545958,
13.8951179643995));
#20203=CARTESIAN_POINT('Ctrl Pts',(-8.22699388814799,1.01453885915651,13.9075988976477));
#20204=CARTESIAN_POINT('Ctrl Pts',(-8.4926936445913,1.01644874085988,13.9200798308959));
#20205=CARTESIAN_POINT('Ctrl Pts',(-8.7583934010346,1.01835862256325,13.9325607641441));
#20206=CARTESIAN_POINT('Ctrl Pts',(-9.02325176140362,0.911059288979132,
13.9450416973923));
#20207=CARTESIAN_POINT('Ctrl Pts',(-9.21270367535821,0.724758509267675,
13.9575226306405));
#20208=CARTESIAN_POINT('Ctrl Pts',(-9.40215558931279,0.538457729556218,
13.9700035638887));
#20209=CARTESIAN_POINT('Ctrl Pts',(-9.51388182535835,0.275436159672578,
13.9824844971369));
#20210=CARTESIAN_POINT('Ctrl Pts',(-9.51642831724057,0.00974174196447676,
13.994965430385));
#20211=CARTESIAN_POINT('Ctrl Pts',(-9.51645943884197,0.00649459406690437,
13.9951179643995));
#20212=CARTESIAN_POINT('Ctrl Pts',(-9.516475,0.0032472970340143,13.995270498414));
#20213=CARTESIAN_POINT('Ctrl Pts',(-9.516475,6.67578553569746E-13,13.9954230324285));
#20214=CARTESIAN_POINT('Ctrl Pts',(-9.51504772062611,-0.000396309267489167,
13.7545769675715));
#20215=CARTESIAN_POINT('Ctrl Pts',(-9.51566105818666,-0.142309670683462,
13.7612219868299));
#20216=CARTESIAN_POINT('Ctrl Pts',(-9.42163809550689,-0.623275699977225,
13.78377434724));
#20217=CARTESIAN_POINT('Ctrl Pts',(-8.68330312999737,-1.18858044034005,
13.8222340488017));
#20218=CARTESIAN_POINT('Ctrl Pts',(-7.78213757023688,-0.861594151033408,
13.8620024016807));
#20219=CARTESIAN_POINT('Ctrl Pts',(-7.47002326942581,-0.236120563005943,
13.893817083984));
#20220=CARTESIAN_POINT('Ctrl Pts',(-7.47851070073035,0.462850473304309,
13.9256317662872));
#20221=CARTESIAN_POINT('Ctrl Pts',(-8.14724805356803,1.14973456280755,13.9654001191663));
#20222=CARTESIAN_POINT('Ctrl Pts',(-9.22798704108243,0.927582382414148,
14.011033076453));
#20223=CARTESIAN_POINT('Ctrl Pts',(-9.51508506382702,0.292620752306052,
14.040758692588));
#20224=CARTESIAN_POINT('Ctrl Pts',(-9.51736327555368,-0.000704366368343423,
14.0545769675715));
#20225=CARTESIAN_POINT('Origin',(-8.5,0.,1.24542303242842));
#20226=CARTESIAN_POINT('',(-9.516475,5.65965774601236E-13,13.3954230324285));
#20227=CARTESIAN_POINT('',(-9.516475,5.92909588180802E-13,13.4545769675715));
#20228=CARTESIAN_POINT('',(-9.516475,1.78524650477582E-12,1.24542303242842));
#20229=CARTESIAN_POINT('Ctrl Pts',(-9.516475,5.65965774601236E-13,13.3954230324285));
#20230=CARTESIAN_POINT('Ctrl Pts',(-9.51647500000015,-0.265706620583383,
13.4079039656767));
#20231=CARTESIAN_POINT('Ctrl Pts',(-9.40727465387226,-0.529786878176597,
13.4203848989248));
#20232=CARTESIAN_POINT('Ctrl Pts',(-9.21961691907799,-0.71789478017443,
13.432865832173));
#20233=CARTESIAN_POINT('Ctrl Pts',(-9.03195918428372,-0.906002682172264,
13.4453467654212));
#20234=CARTESIAN_POINT('Ctrl Pts',(-8.76814132834418,-1.01583545019898,
13.4578276986694));
#20235=CARTESIAN_POINT('Ctrl Pts',(-8.50243547044545,-1.0164720823066,13.4703086319176));
#20236=CARTESIAN_POINT('Ctrl Pts',(-8.23672961254671,-1.01710871441422,
13.4827895651658));
#20237=CARTESIAN_POINT('Ctrl Pts',(-7.97238846933374,-0.908541417082982,
13.495270498414));
#20238=CARTESIAN_POINT('Ctrl Pts',(-7.78383148002372,-0.721334926798906,
13.5077514316622));
#20239=CARTESIAN_POINT('Ctrl Pts',(-7.59527449071369,-0.53412843651483,
13.5202323649104));
#20240=CARTESIAN_POINT('Ctrl Pts',(-7.48480993131717,-0.270574496756232,
13.5327132981586));
#20241=CARTESIAN_POINT('Ctrl Pts',(-7.48353667075686,-0.00487092690876391,
13.5451942314067));
#20242=CARTESIAN_POINT('Ctrl Pts',(-7.48226341019655,0.260832642938704,
13.5576751646549));
#20243=CARTESIAN_POINT('Ctrl Pts',(-7.59019703546723,0.52543315423994,13.5701560979031));
#20244=CARTESIAN_POINT('Ctrl Pts',(-7.77695120652479,0.714438148392872,
13.5826370311513));
#20245=CARTESIAN_POINT('Ctrl Pts',(-7.96370537758234,0.903443142545804,
13.5951179643995));
#20246=CARTESIAN_POINT('Ctrl Pts',(-8.22699388814769,1.01453885915643,13.6075988976477));
#20247=CARTESIAN_POINT('Ctrl Pts',(-8.49269364459097,1.01644874085988,13.6200798308959));
#20248=CARTESIAN_POINT('Ctrl Pts',(-8.75839340103426,1.01835862256333,13.6325607641441));
#20249=CARTESIAN_POINT('Ctrl Pts',(-9.02325176140329,0.911059288979315,
13.6450416973923));
#20250=CARTESIAN_POINT('Ctrl Pts',(-9.21270367535793,0.724758509267943,
13.6575226306405));
#20251=CARTESIAN_POINT('Ctrl Pts',(-9.40215558931258,0.538457729556571,
13.6700035638886));
#20252=CARTESIAN_POINT('Ctrl Pts',(-9.51388182535823,0.275436159672998,
13.6824844971368));
#20253=CARTESIAN_POINT('Ctrl Pts',(-9.51642831724057,0.00974174196491706,
13.694965430385));
#20254=CARTESIAN_POINT('Ctrl Pts',(-9.51645943884197,0.00649459406717135,
13.6951179643995));
#20255=CARTESIAN_POINT('Ctrl Pts',(-9.516475,0.0032472970341079,13.695270498414));
#20256=CARTESIAN_POINT('Ctrl Pts',(-9.516475,5.87882206992221E-13,13.6954230324285));
#20257=CARTESIAN_POINT('Ctrl Pts',(-9.516475,6.21799545274072E-13,13.4545769675715));
#20258=CARTESIAN_POINT('Ctrl Pts',(-9.51647500000016,-0.265706620583337,
13.4670579008197));
#20259=CARTESIAN_POINT('Ctrl Pts',(-9.40727465387229,-0.529786878176566,
13.4795388340679));
#20260=CARTESIAN_POINT('Ctrl Pts',(-9.21961691907801,-0.717894780174411,
13.4920197673161));
#20261=CARTESIAN_POINT('Ctrl Pts',(-9.03195918428375,-0.90600268217225,
13.5045007005643));
#20262=CARTESIAN_POINT('Ctrl Pts',(-8.76814132834421,-1.01583545019897,
13.5169816338124));
#20263=CARTESIAN_POINT('Ctrl Pts',(-8.50243547044547,-1.0164720823066,13.5294625670606));
#20264=CARTESIAN_POINT('Ctrl Pts',(-8.23672961254674,-1.01710871441422,
13.5419435003088));
#20265=CARTESIAN_POINT('Ctrl Pts',(-7.97238846933377,-0.908541417082996,
13.554424433557));
#20266=CARTESIAN_POINT('Ctrl Pts',(-7.78383148002374,-0.721334926798925,
13.5669053668052));
#20267=CARTESIAN_POINT('Ctrl Pts',(-7.59527449071371,-0.534128436514854,
13.5793863000534));
#20268=CARTESIAN_POINT('Ctrl Pts',(-7.48480993131717,-0.270574496756259,
13.5918672333016));
#20269=CARTESIAN_POINT('Ctrl Pts',(-7.48353667075686,-0.00487092690879085,
13.6043481665498));
#20270=CARTESIAN_POINT('Ctrl Pts',(-7.48226341019654,0.260832642938677,
13.616829099798));
#20271=CARTESIAN_POINT('Ctrl Pts',(-7.59019703546722,0.525433154239916,
13.6293100330461));
#20272=CARTESIAN_POINT('Ctrl Pts',(-7.77695120652477,0.714438148392853,
13.6417909662943));
#20273=CARTESIAN_POINT('Ctrl Pts',(-7.96370537758231,0.90344314254579,13.6542718995425));
#20274=CARTESIAN_POINT('Ctrl Pts',(-8.22699388814766,1.01453885915642,13.6667528327907));
#20275=CARTESIAN_POINT('Ctrl Pts',(-8.49269364459095,1.01644874085988,13.6792337660389));
#20276=CARTESIAN_POINT('Ctrl Pts',(-8.75839340103423,1.01835862256334,13.6917146992871));
#20277=CARTESIAN_POINT('Ctrl Pts',(-9.02325176140327,0.911059288979329,
13.7041956325353));
#20278=CARTESIAN_POINT('Ctrl Pts',(-9.21270367535791,0.724758509267962,
13.7166765657835));
#20279=CARTESIAN_POINT('Ctrl Pts',(-9.40215558931256,0.538457729556595,
13.7291574990317));
#20280=CARTESIAN_POINT('Ctrl Pts',(-9.51388182535822,0.275436159673025,
13.7416384322799));
#20281=CARTESIAN_POINT('Ctrl Pts',(-9.51642831724057,0.009741741964944,
13.754119365528));
#20282=CARTESIAN_POINT('Ctrl Pts',(-9.51645943884197,0.00649459406721755,
13.7542718995425));
#20283=CARTESIAN_POINT('Ctrl Pts',(-9.516475,0.0032472970341734,13.754424433557));
#20284=CARTESIAN_POINT('Ctrl Pts',(-9.516475,6.72605934758328E-13,13.7545769675715));
#20285=CARTESIAN_POINT('Origin',(-8.5,0.,1.24542303242842));
#20286=CARTESIAN_POINT('',(-9.516475,5.44049342210251E-13,13.0954230324285));
#20287=CARTESIAN_POINT('',(-9.516475,5.70993155789817E-13,13.1545769675715));
#20288=CARTESIAN_POINT('',(-9.516475,1.78524650477582E-12,1.24542303242842));
#20289=CARTESIAN_POINT('Ctrl Pts',(-9.516475,5.72939299303521E-13,13.0954230324285));
#20290=CARTESIAN_POINT('Ctrl Pts',(-9.51647500000015,-0.265706620583386,
13.1079039656767));
#20291=CARTESIAN_POINT('Ctrl Pts',(-9.40727465387226,-0.52978687817661,
13.1203848989248));
#20292=CARTESIAN_POINT('Ctrl Pts',(-9.21961691907798,-0.717894780174446,
13.132865832173));
#20293=CARTESIAN_POINT('Ctrl Pts',(-9.0319591842837,-0.906002682172282,
13.1453467654212));
#20294=CARTESIAN_POINT('Ctrl Pts',(-8.76814132834414,-1.01583545019899,
13.1578276986694));
#20295=CARTESIAN_POINT('Ctrl Pts',(-8.5024354704454,-1.0164720823066,13.1703086319176));
#20296=CARTESIAN_POINT('Ctrl Pts',(-8.23672961254665,-1.0171087144142,13.1827895651658));
#20297=CARTESIAN_POINT('Ctrl Pts',(-7.97238846933368,-0.908541417082948,
13.195270498414));
#20298=CARTESIAN_POINT('Ctrl Pts',(-7.78383148002366,-0.72133492679885,
13.2077514316622));
#20299=CARTESIAN_POINT('Ctrl Pts',(-7.59527449071365,-0.534128436514753,
13.2202323649104));
#20300=CARTESIAN_POINT('Ctrl Pts',(-7.48480993131714,-0.270574496756133,
13.2327132981586));
#20301=CARTESIAN_POINT('Ctrl Pts',(-7.48353667075686,-0.00487092690865533,
13.2451942314067));
#20302=CARTESIAN_POINT('Ctrl Pts',(-7.48226341019658,0.260832642938823,
13.2576751646549));
#20303=CARTESIAN_POINT('Ctrl Pts',(-7.5901970354673,0.525433154240057,13.2701560979031));
#20304=CARTESIAN_POINT('Ctrl Pts',(-7.77695120652488,0.71443814839297,13.2826370311513));
#20305=CARTESIAN_POINT('Ctrl Pts',(-7.96370537758247,0.903443142545883,
13.2951179643995));
#20306=CARTESIAN_POINT('Ctrl Pts',(-8.22699388814784,1.01453885915647,13.3075988976477));
#20307=CARTESIAN_POINT('Ctrl Pts',(-8.49269364459114,1.01644874085988,13.3200798308959));
#20308=CARTESIAN_POINT('Ctrl Pts',(-8.75839340103443,1.01835862256329,13.3325607641441));
#20309=CARTESIAN_POINT('Ctrl Pts',(-9.02325176140346,0.911059288979222,
13.3450416973923));
#20310=CARTESIAN_POINT('Ctrl Pts',(-9.21270367535807,0.724758509267806,
13.3575226306405));
#20311=CARTESIAN_POINT('Ctrl Pts',(-9.40215558931269,0.538457729556391,
13.3700035638887));
#20312=CARTESIAN_POINT('Ctrl Pts',(-9.51388182535829,0.275436159672784,
13.3824844971368));
#20313=CARTESIAN_POINT('Ctrl Pts',(-9.51642831724057,0.00974174196469292,
13.394965430385));
#20314=CARTESIAN_POINT('Ctrl Pts',(-9.51645943884197,0.00649459406701462,
13.3951179643995));
#20315=CARTESIAN_POINT('Ctrl Pts',(-9.516475,0.00324729703401863,13.395270498414));
#20316=CARTESIAN_POINT('Ctrl Pts',(-9.516475,5.65965774601236E-13,13.3954230324285));
#20317=CARTESIAN_POINT('Ctrl Pts',(-9.516475,6.28773069976357E-13,13.1545769675715));
#20318=CARTESIAN_POINT('Ctrl Pts',(-9.51647500000016,-0.26570662058334,
13.1670579008197));
#20319=CARTESIAN_POINT('Ctrl Pts',(-9.40727465387228,-0.529786878176579,
13.1795388340679));
#20320=CARTESIAN_POINT('Ctrl Pts',(-9.219616919078,-0.717894780174427,13.1920197673161));
#20321=CARTESIAN_POINT('Ctrl Pts',(-9.03195918428372,-0.906002682172275,
13.2045007005643));
#20322=CARTESIAN_POINT('Ctrl Pts',(-8.76814132834415,-1.01583545019899,
13.2169816338124));
#20323=CARTESIAN_POINT('Ctrl Pts',(-8.50243547044539,-1.0164720823066,13.2294625670606));
#20324=CARTESIAN_POINT('Ctrl Pts',(-8.23672961254664,-1.0171087144142,13.2419435003088));
#20325=CARTESIAN_POINT('Ctrl Pts',(-7.97238846933366,-0.908541417082939,
13.254424433557));
#20326=CARTESIAN_POINT('Ctrl Pts',(-7.78383148002364,-0.721334926798828,
13.2669053668052));
#20327=CARTESIAN_POINT('Ctrl Pts',(-7.59527449071362,-0.534128436514718,
13.2793863000534));
#20328=CARTESIAN_POINT('Ctrl Pts',(-7.48480993131712,-0.270574496756083,
13.2918672333016));
#20329=CARTESIAN_POINT('Ctrl Pts',(-7.48353667075686,-0.0048709269085956,
13.3043481665498));
#20330=CARTESIAN_POINT('Ctrl Pts',(-7.48226341019659,0.260832642938892,
13.316829099798));
#20331=CARTESIAN_POINT('Ctrl Pts',(-7.59019703546734,0.525433154240129,
13.3293100330462));
#20332=CARTESIAN_POINT('Ctrl Pts',(-7.77695120652494,0.714438148393033,
13.3417909662943));
#20333=CARTESIAN_POINT('Ctrl Pts',(-7.96370537758255,0.903443142545937,
13.3542718995425));
#20334=CARTESIAN_POINT('Ctrl Pts',(-8.22699388814795,1.0145388591565,13.3667528327907));
#20335=CARTESIAN_POINT('Ctrl Pts',(-8.49269364459126,1.01644874085988,13.3792337660389));
#20336=CARTESIAN_POINT('Ctrl Pts',(-8.75839340103456,1.01835862256326,13.3917146992871));
#20337=CARTESIAN_POINT('Ctrl Pts',(-9.02325176140358,0.911059288979153,
13.4041956325353));
#20338=CARTESIAN_POINT('Ctrl Pts',(-9.21270367535818,0.724758509267703,
13.4166765657835));
#20339=CARTESIAN_POINT('Ctrl Pts',(-9.40215558931277,0.538457729556254,
13.4291574990317));
#20340=CARTESIAN_POINT('Ctrl Pts',(-9.51388182535834,0.275436159672619,
13.4416384322799));
#20341=CARTESIAN_POINT('Ctrl Pts',(-9.51642831724057,0.00974174196451764,
13.4541193655281));
#20342=CARTESIAN_POINT('Ctrl Pts',(-9.51645943884197,0.00649459406691637,
13.4542718995425));
#20343=CARTESIAN_POINT('Ctrl Pts',(-9.516475,0.00324729703399743,13.454424433557));
#20344=CARTESIAN_POINT('Ctrl Pts',(-9.516475,6.21799545274072E-13,13.4545769675715));
#20345=CARTESIAN_POINT('Origin',(-8.5,0.,1.24542303242842));
#20346=CARTESIAN_POINT('',(-9.51612357761841,0.000116121315980709,12.7954230324285));
#20347=CARTESIAN_POINT('',(-9.516475,5.49076723398832E-13,12.8545769675715));
#20348=CARTESIAN_POINT('',(-9.516475,1.78524650477582E-12,1.24542303242842));
#20349=CARTESIAN_POINT('Ctrl Pts',(-9.516475,5.22132909819266E-13,12.7954230324285));
#20350=CARTESIAN_POINT('Ctrl Pts',(-9.51647500000014,-0.265706620583447,
12.8079039656767));
#20351=CARTESIAN_POINT('Ctrl Pts',(-9.40727465387222,-0.529786878176674,
12.8203848989249));
#20352=CARTESIAN_POINT('Ctrl Pts',(-9.21961691907792,-0.717894780174502,
12.832865832173));
#20353=CARTESIAN_POINT('Ctrl Pts',(-9.03195918428362,-0.906002682172331,
12.8453467654212));
#20354=CARTESIAN_POINT('Ctrl Pts',(-8.76814132834404,-1.01583545019902,
12.8578276986694));
#20355=CARTESIAN_POINT('Ctrl Pts',(-8.50243547044529,-1.0164720823066,12.8703086319176));
#20356=CARTESIAN_POINT('Ctrl Pts',(-8.23672961254653,-1.01710871441417,
12.8827895651658));
#20357=CARTESIAN_POINT('Ctrl Pts',(-7.97238846933356,-0.908541417082883,
12.895270498414));
#20358=CARTESIAN_POINT('Ctrl Pts',(-7.78383148002357,-0.721334926798753,
12.9077514316622));
#20359=CARTESIAN_POINT('Ctrl Pts',(-7.59527449071357,-0.534128436514623,
12.9202323649104));
#20360=CARTESIAN_POINT('Ctrl Pts',(-7.48480993131709,-0.270574496755977,
12.9327132981586));
#20361=CARTESIAN_POINT('Ctrl Pts',(-7.48353667075686,-0.00487092690848896,
12.9451942314068));
#20362=CARTESIAN_POINT('Ctrl Pts',(-7.48226341019662,0.260832642938999,
12.9576751646549));
#20363=CARTESIAN_POINT('Ctrl Pts',(-7.59019703546739,0.525433154240224,
12.9701560979031));
#20364=CARTESIAN_POINT('Ctrl Pts',(-7.77695120652502,0.714438148393109,
12.9826370311513));
#20365=CARTESIAN_POINT('Ctrl Pts',(-7.96370537758265,0.903443142545993,
12.9951179643995));
#20366=CARTESIAN_POINT('Ctrl Pts',(-8.22699388814806,1.01453885915653,13.0075988976477));
#20367=CARTESIAN_POINT('Ctrl Pts',(-8.49269364459136,1.01644874085988,13.0200798308959));
#20368=CARTESIAN_POINT('Ctrl Pts',(-8.75839340103467,1.01835862256324,13.0325607641441));
#20369=CARTESIAN_POINT('Ctrl Pts',(-9.02325176140368,0.911059288979098,
13.0450416973923));
#20370=CARTESIAN_POINT('Ctrl Pts',(-9.21270367535825,0.724758509267629,
13.0575226306405));
#20371=CARTESIAN_POINT('Ctrl Pts',(-9.40215558931283,0.538457729556159,
13.0700035638887));
#20372=CARTESIAN_POINT('Ctrl Pts',(-9.51388182535837,0.275436159672512,
13.0824844971369));
#20373=CARTESIAN_POINT('Ctrl Pts',(-9.51642831724057,0.00974174196441101,
13.094965430385));
#20374=CARTESIAN_POINT('Ctrl Pts',(-9.51645943884197,0.00649459406682899,
13.0951179643995));
#20375=CARTESIAN_POINT('Ctrl Pts',(-9.516475,0.00324729703392927,13.095270498414));
#20376=CARTESIAN_POINT('Ctrl Pts',(-9.516475,5.72939299303521E-13,13.0954230324285));
#20377=CARTESIAN_POINT('Ctrl Pts',(-9.516475,5.20186766305562E-13,12.8545769675715));
#20378=CARTESIAN_POINT('Ctrl Pts',(-9.51647500000014,-0.265706620583449,
12.8670579008197));
#20379=CARTESIAN_POINT('Ctrl Pts',(-9.40727465387222,-0.529786878176676,
12.8795388340679));
#20380=CARTESIAN_POINT('Ctrl Pts',(-9.21961691907792,-0.717894780174504,
12.8920197673161));
#20381=CARTESIAN_POINT('Ctrl Pts',(-9.03195918428362,-0.906002682172331,
12.9045007005643));
#20382=CARTESIAN_POINT('Ctrl Pts',(-8.76814132834404,-1.01583545019902,
12.9169816338124));
#20383=CARTESIAN_POINT('Ctrl Pts',(-8.50243547044529,-1.0164720823066,12.9294625670606));
#20384=CARTESIAN_POINT('Ctrl Pts',(-8.23672961254653,-1.01710871441417,
12.9419435003088));
#20385=CARTESIAN_POINT('Ctrl Pts',(-7.97238846933356,-0.908541417082882,
12.954424433557));
#20386=CARTESIAN_POINT('Ctrl Pts',(-7.78383148002356,-0.721334926798752,
12.9669053668052));
#20387=CARTESIAN_POINT('Ctrl Pts',(-7.59527449071357,-0.534128436514622,
12.9793863000534));
#20388=CARTESIAN_POINT('Ctrl Pts',(-7.48480993131709,-0.270574496755975,
12.9918672333016));
#20389=CARTESIAN_POINT('Ctrl Pts',(-7.48353667075686,-0.00487092690848702,
13.0043481665498));
#20390=CARTESIAN_POINT('Ctrl Pts',(-7.48226341019662,0.260832642939001,
13.016829099798));
#20391=CARTESIAN_POINT('Ctrl Pts',(-7.59019703546739,0.525433154240226,
13.0293100330462));
#20392=CARTESIAN_POINT('Ctrl Pts',(-7.77695120652502,0.71443814839311,13.0417909662944));
#20393=CARTESIAN_POINT('Ctrl Pts',(-7.96370537758265,0.903443142545994,
13.0542718995425));
#20394=CARTESIAN_POINT('Ctrl Pts',(-8.22699388814806,1.01453885915653,13.0667528327907));
#20395=CARTESIAN_POINT('Ctrl Pts',(-8.49269364459136,1.01644874085988,13.0792337660389));
#20396=CARTESIAN_POINT('Ctrl Pts',(-8.75839340103467,1.01835862256323,13.0917146992871));
#20397=CARTESIAN_POINT('Ctrl Pts',(-9.02325176140368,0.911059288979097,
13.1041956325353));
#20398=CARTESIAN_POINT('Ctrl Pts',(-9.21270367535826,0.724758509267627,
13.1166765657835));
#20399=CARTESIAN_POINT('Ctrl Pts',(-9.40215558931283,0.538457729556157,
13.1291574990317));
#20400=CARTESIAN_POINT('Ctrl Pts',(-9.51388182535837,0.27543615967251,13.1416384322799));
#20401=CARTESIAN_POINT('Ctrl Pts',(-9.51642831724057,0.00974174196440906,
13.1541193655281));
#20402=CARTESIAN_POINT('Ctrl Pts',(-9.51645943884197,0.0064945940668463,
13.1542718995425));
#20403=CARTESIAN_POINT('Ctrl Pts',(-9.516475,0.00324729703396589,13.154424433557));
#20404=CARTESIAN_POINT('Ctrl Pts',(-9.516475,6.28773069976357E-13,13.1545769675715));
#20405=CARTESIAN_POINT('Origin',(-8.5,0.,1.24542303242842));
#20406=CARTESIAN_POINT('',(-9.51653950885578,4.27590676786889E-5,12.4954230324285));
#20407=CARTESIAN_POINT('',(-9.516475,5.27160291007847E-13,12.5545769675715));
#20408=CARTESIAN_POINT('',(-9.516475,1.78524650477582E-12,1.24542303242842));
#20409=CARTESIAN_POINT('Ctrl Pts',(-9.51746434211765,0.000655775794156509,
12.4954230324285));
#20410=CARTESIAN_POINT('Ctrl Pts',(-9.51527198270641,-0.296676988704239,
12.5094337807337));
#20411=CARTESIAN_POINT('Ctrl Pts',(-9.22128580559795,-0.935436405005595,
12.5393518701905));
#20412=CARTESIAN_POINT('Ctrl Pts',(-8.13336992371389,-1.14538460256293,
12.5851773007989));
#20413=CARTESIAN_POINT('Ctrl Pts',(-7.47298807192611,-0.450463593150824,
12.6249456536779));
#20414=CARTESIAN_POINT('Ctrl Pts',(-7.47295403032462,0.248558970813969,
12.6567603359812));
#20415=CARTESIAN_POINT('Ctrl Pts',(-7.79260946040346,0.87021237272846,12.6885750182844));
#20416=CARTESIAN_POINT('Ctrl Pts',(-8.69766342022542,1.1862768112589,12.7283433711635));
#20417=CARTESIAN_POINT('Ctrl Pts',(-9.42544752600762,0.614958176341259,
12.7666105994034));
#20418=CARTESIAN_POINT('Ctrl Pts',(-9.51577746299321,0.138234549146154,
12.7889704864918));
#20419=CARTESIAN_POINT('Ctrl Pts',(-9.51510940460441,0.00045123686540878,
12.7954230324285));
#20420=CARTESIAN_POINT('Ctrl Pts',(-9.516475,5.84940205194387E-13,12.5545769675715));
#20421=CARTESIAN_POINT('Ctrl Pts',(-9.51647500000015,-0.265706620583384,
12.5670579008197));
#20422=CARTESIAN_POINT('Ctrl Pts',(-9.40727465387226,-0.529786878176618,
12.5795388340679));
#20423=CARTESIAN_POINT('Ctrl Pts',(-9.21961691907797,-0.717894780174458,
12.5920197673161));
#20424=CARTESIAN_POINT('Ctrl Pts',(-9.03195918428368,-0.906002682172298,
12.6045007005643));
#20425=CARTESIAN_POINT('Ctrl Pts',(-8.7681413283441,-1.015835450199,12.6169816338124));
#20426=CARTESIAN_POINT('Ctrl Pts',(-8.50243547044535,-1.0164720823066,12.6294625670606));
#20427=CARTESIAN_POINT('Ctrl Pts',(-8.2367296125466,-1.01710871441419,12.6419435003088));
#20428=CARTESIAN_POINT('Ctrl Pts',(-7.97238846933362,-0.908541417082916,
12.654424433557));
#20429=CARTESIAN_POINT('Ctrl Pts',(-7.78383148002361,-0.721334926798798,
12.6669053668052));
#20430=CARTESIAN_POINT('Ctrl Pts',(-7.5952744907136,-0.534128436514679,
12.6793863000534));
#20431=CARTESIAN_POINT('Ctrl Pts',(-7.48480993131711,-0.27057449675604,
12.6918672333016));
#20432=CARTESIAN_POINT('Ctrl Pts',(-7.48353667075686,-0.00487092690855177,
12.7043481665498));
#20433=CARTESIAN_POINT('Ctrl Pts',(-7.48226341019661,0.260832642938936,
12.716829099798));
#20434=CARTESIAN_POINT('Ctrl Pts',(-7.59019703546736,0.525433154240168,
12.7293100330462));
#20435=CARTESIAN_POINT('Ctrl Pts',(-7.77695120652497,0.714438148393064,
12.7417909662943));
#20436=CARTESIAN_POINT('Ctrl Pts',(-7.96370537758259,0.90344314254596,12.7542718995425));
#20437=CARTESIAN_POINT('Ctrl Pts',(-8.22699388814799,1.01453885915651,12.7667528327907));
#20438=CARTESIAN_POINT('Ctrl Pts',(-8.4926936445913,1.01644874085988,12.7792337660389));
#20439=CARTESIAN_POINT('Ctrl Pts',(-8.7583934010346,1.01835862256325,12.7917146992871));
#20440=CARTESIAN_POINT('Ctrl Pts',(-9.02325176140362,0.91105928897913,12.8041956325353));
#20441=CARTESIAN_POINT('Ctrl Pts',(-9.21270367535821,0.724758509267673,
12.8166765657835));
#20442=CARTESIAN_POINT('Ctrl Pts',(-9.4021555893128,0.538457729556215,12.8291574990317));
#20443=CARTESIAN_POINT('Ctrl Pts',(-9.51388182535835,0.275436159672575,
12.8416384322799));
#20444=CARTESIAN_POINT('Ctrl Pts',(-9.51642831724057,0.00974174196447381,
12.8541193655281));
#20445=CARTESIAN_POINT('Ctrl Pts',(-9.51645943884197,0.00649459406685328,
12.8542718995425));
#20446=CARTESIAN_POINT('Ctrl Pts',(-9.516475,0.00324729703391504,12.854424433557));
#20447=CARTESIAN_POINT('Ctrl Pts',(-9.516475,5.20186766305562E-13,12.8545769675715));
#20448=CARTESIAN_POINT('Origin',(-8.5,0.,1.24542303242842));
#20449=CARTESIAN_POINT('',(-9.516475,4.78300045037296E-13,12.1954230324285));
#20450=CARTESIAN_POINT('',(-9.516475,5.05243858616862E-13,12.2545769675715));
#20451=CARTESIAN_POINT('',(-9.516475,1.78524650477582E-12,1.24542303242842));
#20452=CARTESIAN_POINT('Ctrl Pts',(-9.516475,4.78300045037296E-13,12.1954230324285));
#20453=CARTESIAN_POINT('Ctrl Pts',(-9.51647500000012,-0.265706620583481,
12.2079039656767));
#20454=CARTESIAN_POINT('Ctrl Pts',(-9.40727465387221,-0.529786878176695,
12.2203848989249));
#20455=CARTESIAN_POINT('Ctrl Pts',(-9.21961691907791,-0.717894780174513,
12.232865832173));
#20456=CARTESIAN_POINT('Ctrl Pts',(-9.03195918428361,-0.906002682172331,
12.2453467654212));
#20457=CARTESIAN_POINT('Ctrl Pts',(-8.76814132834405,-1.01583545019902,
12.2578276986694));
#20458=CARTESIAN_POINT('Ctrl Pts',(-8.5024354704453,-1.0164720823066,12.2703086319176));
#20459=CARTESIAN_POINT('Ctrl Pts',(-8.23672961254656,-1.01710871441418,
12.2827895651658));
#20460=CARTESIAN_POINT('Ctrl Pts',(-7.9723884693336,-0.908541417082899,
12.295270498414));
#20461=CARTESIAN_POINT('Ctrl Pts',(-7.7838314800236,-0.721334926798783,
12.3077514316622));
#20462=CARTESIAN_POINT('Ctrl Pts',(-7.5952744907136,-0.534128436514668,
12.3202323649104));
#20463=CARTESIAN_POINT('Ctrl Pts',(-7.48480993131711,-0.270574496756039,
12.3327132981586));
#20464=CARTESIAN_POINT('Ctrl Pts',(-7.48353667075686,-0.00487092690856069,
12.3451942314068));
#20465=CARTESIAN_POINT('Ctrl Pts',(-7.4822634101966,0.260832642938917,12.3576751646549));
#20466=CARTESIAN_POINT('Ctrl Pts',(-7.59019703546735,0.525433154240141,
12.3701560979031));
#20467=CARTESIAN_POINT('Ctrl Pts',(-7.77695120652495,0.714438148393037,
12.3826370311513));
#20468=CARTESIAN_POINT('Ctrl Pts',(-7.96370537758255,0.903443142545933,
12.3951179643995));
#20469=CARTESIAN_POINT('Ctrl Pts',(-8.22699388814794,1.0145388591565,12.4075988976477));
#20470=CARTESIAN_POINT('Ctrl Pts',(-8.49269364459123,1.01644874085988,12.4200798308959));
#20471=CARTESIAN_POINT('Ctrl Pts',(-8.75839340103453,1.01835862256327,12.4325607641441));
#20472=CARTESIAN_POINT('Ctrl Pts',(-9.02325176140354,0.911059288979173,
12.4450416973923));
#20473=CARTESIAN_POINT('Ctrl Pts',(-9.21270367535814,0.72475850926774,12.4575226306405));
#20474=CARTESIAN_POINT('Ctrl Pts',(-9.40215558931274,0.538457729556307,
12.4700035638887));
#20475=CARTESIAN_POINT('Ctrl Pts',(-9.51388182535831,0.275436159672689,
12.4824844971368));
#20476=CARTESIAN_POINT('Ctrl Pts',(-9.51642831724057,0.00974174196459828,
12.494965430385));
#20477=CARTESIAN_POINT('Ctrl Pts',(-9.51645943884197,0.00649459406691998,
12.4951179643995));
#20478=CARTESIAN_POINT('Ctrl Pts',(-9.516475,0.003247297033924,12.495270498414));
#20479=CARTESIAN_POINT('Ctrl Pts',(-9.516475,4.71326520335011E-13,12.4954230324285));
#20480=CARTESIAN_POINT('Ctrl Pts',(-9.516475,5.05243858616862E-13,12.2545769675715));
#20481=CARTESIAN_POINT('Ctrl Pts',(-9.51647500000013,-0.265706620583483,
12.2670579008197));
#20482=CARTESIAN_POINT('Ctrl Pts',(-9.4072746538722,-0.529786878176727,
12.2795388340679));
#20483=CARTESIAN_POINT('Ctrl Pts',(-9.21961691907787,-0.717894780174555,
12.2920197673161));
#20484=CARTESIAN_POINT('Ctrl Pts',(-9.03195918428354,-0.906002682172383,
12.3045007005643));
#20485=CARTESIAN_POINT('Ctrl Pts',(-8.76814132834393,-1.01583545019905,
12.3169816338125));
#20486=CARTESIAN_POINT('Ctrl Pts',(-8.50243547044516,-1.0164720823066,12.3294625670606));
#20487=CARTESIAN_POINT('Ctrl Pts',(-8.23672961254638,-1.01710871441414,
12.3419435003088));
#20488=CARTESIAN_POINT('Ctrl Pts',(-7.97238846933341,-0.908541417082798,
12.354424433557));
#20489=CARTESIAN_POINT('Ctrl Pts',(-7.78383148002343,-0.721334926798619,
12.3669053668052));
#20490=CARTESIAN_POINT('Ctrl Pts',(-7.59527449071345,-0.534128436514441,
12.3793863000534));
#20491=CARTESIAN_POINT('Ctrl Pts',(-7.48480993131703,-0.270574496755748,
12.3918672333016));
#20492=CARTESIAN_POINT('Ctrl Pts',(-7.48353667075686,-0.00487092690824096,
12.4043481665498));
#20493=CARTESIAN_POINT('Ctrl Pts',(-7.48226341019669,0.260832642939266,
12.416829099798));
#20494=CARTESIAN_POINT('Ctrl Pts',(-7.59019703546754,0.525433154240484,
12.4293100330462));
#20495=CARTESIAN_POINT('Ctrl Pts',(-7.77695120652523,0.714438148393326,
12.4417909662944));
#20496=CARTESIAN_POINT('Ctrl Pts',(-7.96370537758293,0.903443142546168,
12.4542718995426));
#20497=CARTESIAN_POINT('Ctrl Pts',(-8.2269938881484,1.01453885915663,12.4667528327907));
#20498=CARTESIAN_POINT('Ctrl Pts',(-8.49269364459172,1.01644874085989,12.4792337660389));
#20499=CARTESIAN_POINT('Ctrl Pts',(-8.75839340103505,1.01835862256314,12.4917146992871));
#20500=CARTESIAN_POINT('Ctrl Pts',(-9.02325176140404,0.911059288978894,
12.5041956325353));
#20501=CARTESIAN_POINT('Ctrl Pts',(-9.21270367535855,0.724758509267333,
12.5166765657835));
#20502=CARTESIAN_POINT('Ctrl Pts',(-9.40215558931307,0.538457729555772,
12.5291574990317));
#20503=CARTESIAN_POINT('Ctrl Pts',(-9.51388182535849,0.275436159672054,
12.5416384322799));
#20504=CARTESIAN_POINT('Ctrl Pts',(-9.51642831724057,0.0097417419639319,
12.5541193655281));
#20505=CARTESIAN_POINT('Ctrl Pts',(-9.51645943884197,0.00649459406651357,
12.5542718995426));
#20506=CARTESIAN_POINT('Ctrl Pts',(-9.516475,0.00324729703377759,12.554424433557));
#20507=CARTESIAN_POINT('Ctrl Pts',(-9.516475,5.84940205194387E-13,12.5545769675715));
#20508=CARTESIAN_POINT('Origin',(-8.5,0.,1.24542303242842));
#20509=CARTESIAN_POINT('',(-9.516475,4.5638361264631E-13,11.8954230324285));
#20510=CARTESIAN_POINT('',(-9.516475,4.83327426225877E-13,11.9545769675715));
#20511=CARTESIAN_POINT('',(-9.516475,1.78524650477582E-12,1.24542303242842));
#20512=CARTESIAN_POINT('Ctrl Pts',(-9.516475,4.2749365555304E-13,11.8954230324285));
#20513=CARTESIAN_POINT('Ctrl Pts',(-9.51647500000011,-0.265706620583551,
11.9079039656767));
#20514=CARTESIAN_POINT('Ctrl Pts',(-9.40727465387217,-0.529786878176778,
11.9203848989249));
#20515=CARTESIAN_POINT('Ctrl Pts',(-9.21961691907784,-0.71789478017459,
11.932865832173));
#20516=CARTESIAN_POINT('Ctrl Pts',(-9.0319591842835,-0.906002682172402,
11.9453467654212));
#20517=CARTESIAN_POINT('Ctrl Pts',(-8.7681413283439,-1.01583545019906,11.9578276986694));
#20518=CARTESIAN_POINT('Ctrl Pts',(-8.50243547044514,-1.0164720823066,11.9703086319176));
#20519=CARTESIAN_POINT('Ctrl Pts',(-8.23672961254637,-1.01710871441414,
11.9827895651658));
#20520=CARTESIAN_POINT('Ctrl Pts',(-7.97238846933341,-0.908541417082796,
11.995270498414));
#20521=CARTESIAN_POINT('Ctrl Pts',(-7.78383148002344,-0.721334926798626,
12.0077514316622));
#20522=CARTESIAN_POINT('Ctrl Pts',(-7.59527449071346,-0.534128436514455,
12.0202323649104));
#20523=CARTESIAN_POINT('Ctrl Pts',(-7.48480993131704,-0.270574496755776,
12.0327132981586));
#20524=CARTESIAN_POINT('Ctrl Pts',(-7.48353667075686,-0.00487092690827876,
12.0451942314068));
#20525=CARTESIAN_POINT('Ctrl Pts',(-7.48226341019668,0.260832642939219,
12.057675164655));
#20526=CARTESIAN_POINT('Ctrl Pts',(-7.59019703546751,0.525433154240432,
12.0701560979031));
#20527=CARTESIAN_POINT('Ctrl Pts',(-7.77695120652519,0.714438148393279,
12.0826370311513));
#20528=CARTESIAN_POINT('Ctrl Pts',(-7.96370537758286,0.903443142546126,
12.0951179643995));
#20529=CARTESIAN_POINT('Ctrl Pts',(-8.22699388814831,1.0145388591566,12.1075988976477));
#20530=CARTESIAN_POINT('Ctrl Pts',(-8.49269364459163,1.01644874085989,12.1200798308959));
#20531=CARTESIAN_POINT('Ctrl Pts',(-8.75839340103495,1.01835862256317,12.1325607641441));
#20532=CARTESIAN_POINT('Ctrl Pts',(-9.02325176140394,0.911059288978952,
12.1450416973923));
#20533=CARTESIAN_POINT('Ctrl Pts',(-9.21270367535847,0.72475850926742,12.1575226306405));
#20534=CARTESIAN_POINT('Ctrl Pts',(-9.40215558931299,0.538457729555889,
12.1700035638887));
#20535=CARTESIAN_POINT('Ctrl Pts',(-9.51388182535845,0.275436159672197,
12.1824844971369));
#20536=CARTESIAN_POINT('Ctrl Pts',(-9.51642831724057,0.00974174196408526,
12.1949654303851));
#20537=CARTESIAN_POINT('Ctrl Pts',(-9.51645943884197,0.00649459406658027,
12.1951179643995));
#20538=CARTESIAN_POINT('Ctrl Pts',(-9.516475,0.00324729703375759,12.195270498414));
#20539=CARTESIAN_POINT('Ctrl Pts',(-9.516475,4.78300045037296E-13,12.1954230324285));
#20540=CARTESIAN_POINT('Ctrl Pts',(-9.516475,5.12217383319147E-13,11.9545769675715));
#20541=CARTESIAN_POINT('Ctrl Pts',(-9.51647500000013,-0.265706620583457,
11.9670579008197));
#20542=CARTESIAN_POINT('Ctrl Pts',(-9.40727465387222,-0.529786878176683,
11.9795388340679));
#20543=CARTESIAN_POINT('Ctrl Pts',(-9.21961691907792,-0.717894780174509,
11.9920197673161));
#20544=CARTESIAN_POINT('Ctrl Pts',(-9.03195918428361,-0.906002682172336,
12.0045007005643));
#20545=CARTESIAN_POINT('Ctrl Pts',(-8.76814132834403,-1.01583545019902,
12.0169816338125));
#20546=CARTESIAN_POINT('Ctrl Pts',(-8.50243547044528,-1.0164720823066,12.0294625670606));
#20547=CARTESIAN_POINT('Ctrl Pts',(-8.23672961254653,-1.01710871441417,
12.0419435003088));
#20548=CARTESIAN_POINT('Ctrl Pts',(-7.97238846933355,-0.908541417082878,
12.054424433557));
#20549=CARTESIAN_POINT('Ctrl Pts',(-7.78383148002356,-0.721334926798746,
12.0669053668052));
#20550=CARTESIAN_POINT('Ctrl Pts',(-7.59527449071356,-0.534128436514615,
12.0793863000534));
#20551=CARTESIAN_POINT('Ctrl Pts',(-7.48480993131709,-0.270574496755967,
12.0918672333016));
#20552=CARTESIAN_POINT('Ctrl Pts',(-7.48353667075686,-0.00487092690847905,
12.1043481665498));
#20553=CARTESIAN_POINT('Ctrl Pts',(-7.48226341019662,0.260832642939009,
12.116829099798));
#20554=CARTESIAN_POINT('Ctrl Pts',(-7.5901970354674,0.525433154240233,12.1293100330462));
#20555=CARTESIAN_POINT('Ctrl Pts',(-7.77695120652503,0.714438148393116,
12.1417909662944));
#20556=CARTESIAN_POINT('Ctrl Pts',(-7.96370537758265,0.903443142545999,
12.1542718995425));
#20557=CARTESIAN_POINT('Ctrl Pts',(-8.22699388814807,1.01453885915653,12.1667528327907));
#20558=CARTESIAN_POINT('Ctrl Pts',(-8.49269364459137,1.01644874085988,12.1792337660389));
#20559=CARTESIAN_POINT('Ctrl Pts',(-8.75839340103468,1.01835862256323,12.1917146992871));
#20560=CARTESIAN_POINT('Ctrl Pts',(-9.02325176140369,0.911059288979093,
12.2041956325353));
#20561=CARTESIAN_POINT('Ctrl Pts',(-9.21270367535826,0.724758509267622,
12.2166765657835));
#20562=CARTESIAN_POINT('Ctrl Pts',(-9.40215558931283,0.53845772955615,12.2291574990317));
#20563=CARTESIAN_POINT('Ctrl Pts',(-9.51388182535837,0.275436159672502,
12.2416384322799));
#20564=CARTESIAN_POINT('Ctrl Pts',(-9.51642831724057,0.00974174196440109,
12.2541193655281));
#20565=CARTESIAN_POINT('Ctrl Pts',(-9.51645943884197,0.00649459406679982,
12.2542718995425));
#20566=CARTESIAN_POINT('Ctrl Pts',(-9.516475,0.00324729703388088,12.254424433557));
#20567=CARTESIAN_POINT('Ctrl Pts',(-9.516475,5.05243858616862E-13,12.2545769675715));
#20568=CARTESIAN_POINT('Origin',(-8.5,0.,1.24542303242842));
#20569=CARTESIAN_POINT('',(-9.516475,4.34467180255325E-13,11.5954230324285));
#20570=CARTESIAN_POINT('',(-9.516475,4.61410993834892E-13,11.6545769675715));
#20571=CARTESIAN_POINT('',(-9.516475,1.78524650477582E-12,1.24542303242842));
#20572=CARTESIAN_POINT('Ctrl Pts',(-9.516475,4.63357137348595E-13,11.5954230324285));
#20573=CARTESIAN_POINT('Ctrl Pts',(-9.51647500000012,-0.265706620583515,
11.6079039656767));
#20574=CARTESIAN_POINT('Ctrl Pts',(-9.40727465387219,-0.529786878176746,
11.6203848989249));
#20575=CARTESIAN_POINT('Ctrl Pts',(-9.21961691907786,-0.717894780174565,
11.632865832173));
#20576=CARTESIAN_POINT('Ctrl Pts',(-9.03195918428354,-0.906002682172383,
11.6453467654212));
#20577=CARTESIAN_POINT('Ctrl Pts',(-8.76814132834394,-1.01583545019905,
11.6578276986694));
#20578=CARTESIAN_POINT('Ctrl Pts',(-8.50243547044517,-1.0164720823066,11.6703086319176));
#20579=CARTESIAN_POINT('Ctrl Pts',(-8.23672961254641,-1.01710871441414,
11.6827895651658));
#20580=CARTESIAN_POINT('Ctrl Pts',(-7.97238846933344,-0.908541417082815,
11.695270498414));
#20581=CARTESIAN_POINT('Ctrl Pts',(-7.78383148002346,-0.721334926798651,
11.7077514316622));
#20582=CARTESIAN_POINT('Ctrl Pts',(-7.59527449071348,-0.534128436514487,
11.7202323649104));
#20583=CARTESIAN_POINT('Ctrl Pts',(-7.48480993131705,-0.270574496755812,
11.7327132981586));
#20584=CARTESIAN_POINT('Ctrl Pts',(-7.48353667075686,-0.00487092690831463,
11.7451942314068));
#20585=CARTESIAN_POINT('Ctrl Pts',(-7.48226341019667,0.260832642939183,
11.757675164655));
#20586=CARTESIAN_POINT('Ctrl Pts',(-7.59019703546749,0.525433154240399,
11.7701560979031));
#20587=CARTESIAN_POINT('Ctrl Pts',(-7.77695120652516,0.714438148393253,
11.7826370311513));
#20588=CARTESIAN_POINT('Ctrl Pts',(-7.96370537758283,0.903443142546107,
11.7951179643995));
#20589=CARTESIAN_POINT('Ctrl Pts',(-8.22699388814828,1.01453885915659,11.8075988976477));
#20590=CARTESIAN_POINT('Ctrl Pts',(-8.49269364459159,1.01644874085989,11.8200798308959));
#20591=CARTESIAN_POINT('Ctrl Pts',(-8.75839340103491,1.01835862256318,11.8325607641441));
#20592=CARTESIAN_POINT('Ctrl Pts',(-9.02325176140391,0.91105928897897,11.8450416973923));
#20593=CARTESIAN_POINT('Ctrl Pts',(-9.21270367535844,0.724758509267446,
11.8575226306405));
#20594=CARTESIAN_POINT('Ctrl Pts',(-9.40215558931297,0.538457729555921,
11.8700035638887));
#20595=CARTESIAN_POINT('Ctrl Pts',(-9.51388182535844,0.275436159672233,
11.8824844971369));
#20596=CARTESIAN_POINT('Ctrl Pts',(-9.51642831724057,0.00974174196412112,
11.8949654303851));
#20597=CARTESIAN_POINT('Ctrl Pts',(-9.51645943884197,0.00649459406658725,
11.8951179643995));
#20598=CARTESIAN_POINT('Ctrl Pts',(-9.516475,0.0032472970337357,11.895270498414));
#20599=CARTESIAN_POINT('Ctrl Pts',(-9.516475,4.2749365555304E-13,11.8954230324285));
#20600=CARTESIAN_POINT('Ctrl Pts',(-9.516475,4.61410993834892E-13,11.6545769675715));
#20601=CARTESIAN_POINT('Ctrl Pts',(-9.51647500000012,-0.265706620583517,
11.6670579008197));
#20602=CARTESIAN_POINT('Ctrl Pts',(-9.40727465387218,-0.529786878176748,
11.6795388340679));
#20603=CARTESIAN_POINT('Ctrl Pts',(-9.21961691907786,-0.717894780174566,
11.6920197673161));
#20604=CARTESIAN_POINT('Ctrl Pts',(-9.03195918428353,-0.906002682172384,
11.7045007005643));
#20605=CARTESIAN_POINT('Ctrl Pts',(-8.76814132834393,-1.01583545019905,
11.7169816338125));
#20606=CARTESIAN_POINT('Ctrl Pts',(-8.50243547044517,-1.0164720823066,11.7294625670606));
#20607=CARTESIAN_POINT('Ctrl Pts',(-8.23672961254641,-1.01710871441414,
11.7419435003088));
#20608=CARTESIAN_POINT('Ctrl Pts',(-7.97238846933344,-0.908541417082814,
11.754424433557));
#20609=CARTESIAN_POINT('Ctrl Pts',(-7.78383148002346,-0.72133492679865,
11.7669053668052));
#20610=CARTESIAN_POINT('Ctrl Pts',(-7.59527449071348,-0.534128436514485,
11.7793863000534));
#20611=CARTESIAN_POINT('Ctrl Pts',(-7.48480993131705,-0.27057449675581,
11.7918672333016));
#20612=CARTESIAN_POINT('Ctrl Pts',(-7.48353667075686,-0.00487092690831268,
11.8043481665498));
#20613=CARTESIAN_POINT('Ctrl Pts',(-7.48226341019667,0.260832642939185,
11.816829099798));
#20614=CARTESIAN_POINT('Ctrl Pts',(-7.59019703546749,0.525433154240401,
11.8293100330462));
#20615=CARTESIAN_POINT('Ctrl Pts',(-7.77695120652516,0.714438148393255,
11.8417909662944));
#20616=CARTESIAN_POINT('Ctrl Pts',(-7.96370537758284,0.903443142546108,
11.8542718995426));
#20617=CARTESIAN_POINT('Ctrl Pts',(-8.22699388814828,1.01453885915659,11.8667528327907));
#20618=CARTESIAN_POINT('Ctrl Pts',(-8.4926936445916,1.01644874085989,11.8792337660389));
#20619=CARTESIAN_POINT('Ctrl Pts',(-8.75839340103491,1.01835862256318,11.8917146992871));
#20620=CARTESIAN_POINT('Ctrl Pts',(-9.02325176140391,0.911059288978969,
11.9041956325353));
#20621=CARTESIAN_POINT('Ctrl Pts',(-9.21270367535844,0.724758509267444,
11.9166765657835));
#20622=CARTESIAN_POINT('Ctrl Pts',(-9.40215558931298,0.538457729555919,
11.9291574990317));
#20623=CARTESIAN_POINT('Ctrl Pts',(-9.51388182535845,0.275436159672231,
11.9416384322799));
#20624=CARTESIAN_POINT('Ctrl Pts',(-9.51642831724057,0.00974174196411918,
11.9541193655281));
#20625=CARTESIAN_POINT('Ctrl Pts',(-9.51645943884197,0.00649459406661419,
11.9542718995426));
#20626=CARTESIAN_POINT('Ctrl Pts',(-9.516475,0.00324729703379151,11.954424433557));
#20627=CARTESIAN_POINT('Ctrl Pts',(-9.516475,5.12217383319147E-13,11.9545769675715));
#20628=CARTESIAN_POINT('Origin',(-8.5,0.,1.24542303242842));
#20629=CARTESIAN_POINT('',(-9.51672394194905,-5.37065327258883E-5,11.2954230324285));
#20630=CARTESIAN_POINT('',(-9.516475,4.39494561443907E-13,11.3545769675715));
#20631=CARTESIAN_POINT('',(-9.516475,1.78524650477582E-12,1.24542303242842));
#20632=CARTESIAN_POINT('Ctrl Pts',(-9.516475,4.4144070495761E-13,11.2954230324285));
#20633=CARTESIAN_POINT('Ctrl Pts',(-9.51647500000012,-0.265706620583537,
11.3079039656767));
#20634=CARTESIAN_POINT('Ctrl Pts',(-9.40727465387217,-0.529786878176765,
11.3203848989249));
#20635=CARTESIAN_POINT('Ctrl Pts',(-9.21961691907785,-0.71789478017458,
11.332865832173));
#20636=CARTESIAN_POINT('Ctrl Pts',(-9.03195918428352,-0.906002682172395,
11.3453467654212));
#20637=CARTESIAN_POINT('Ctrl Pts',(-8.76814132834391,-1.01583545019906,
11.3578276986694));
#20638=CARTESIAN_POINT('Ctrl Pts',(-8.50243547044515,-1.0164720823066,11.3703086319176));
#20639=CARTESIAN_POINT('Ctrl Pts',(-8.23672961254639,-1.01710871441414,
11.3827895651658));
#20640=CARTESIAN_POINT('Ctrl Pts',(-7.97238846933342,-0.908541417082803,
11.395270498414));
#20641=CARTESIAN_POINT('Ctrl Pts',(-7.78383148002345,-0.721334926798635,
11.4077514316622));
#20642=CARTESIAN_POINT('Ctrl Pts',(-7.59527449071347,-0.534128436514468,
11.4202323649104));
#20643=CARTESIAN_POINT('Ctrl Pts',(-7.48480993131704,-0.27057449675579,
11.4327132981586));
#20644=CARTESIAN_POINT('Ctrl Pts',(-7.48353667075686,-0.00487092690829271,
11.4451942314068));
#20645=CARTESIAN_POINT('Ctrl Pts',(-7.48226341019667,0.260832642939205,
11.457675164655));
#20646=CARTESIAN_POINT('Ctrl Pts',(-7.5901970354675,0.525433154240419,11.4701560979031));
#20647=CARTESIAN_POINT('Ctrl Pts',(-7.77695120652518,0.714438148393269,
11.4826370311513));
#20648=CARTESIAN_POINT('Ctrl Pts',(-7.96370537758285,0.903443142546119,
11.4951179643995));
#20649=CARTESIAN_POINT('Ctrl Pts',(-8.2269938881483,1.0145388591566,11.5075988976477));
#20650=CARTESIAN_POINT('Ctrl Pts',(-8.49269364459162,1.01644874085989,11.5200798308959));
#20651=CARTESIAN_POINT('Ctrl Pts',(-8.75839340103493,1.01835862256317,11.5325607641441));
#20652=CARTESIAN_POINT('Ctrl Pts',(-9.02325176140393,0.911059288978959,
11.5450416973923));
#20653=CARTESIAN_POINT('Ctrl Pts',(-9.21270367535846,0.72475850926743,11.5575226306405));
#20654=CARTESIAN_POINT('Ctrl Pts',(-9.40215558931299,0.538457729555902,
11.5700035638887));
#20655=CARTESIAN_POINT('Ctrl Pts',(-9.51388182535845,0.275436159672211,
11.5824844971369));
#20656=CARTESIAN_POINT('Ctrl Pts',(-9.51642831724057,0.00974174196409921,
11.5949654303851));
#20657=CARTESIAN_POINT('Ctrl Pts',(-9.51645943884197,0.00649459406658459,
11.5951179643995));
#20658=CARTESIAN_POINT('Ctrl Pts',(-9.516475,0.00324729703375226,11.595270498414));
#20659=CARTESIAN_POINT('Ctrl Pts',(-9.516475,4.63357137348595E-13,11.5954230324285));
#20660=CARTESIAN_POINT('Ctrl Pts',(-9.516475,4.68384518537177E-13,11.3545769675715));
#20661=CARTESIAN_POINT('Ctrl Pts',(-9.51647500000012,-0.26570662058351,
11.3670579008197));
#20662=CARTESIAN_POINT('Ctrl Pts',(-9.40727465387219,-0.529786878176741,
11.3795388340679));
#20663=CARTESIAN_POINT('Ctrl Pts',(-9.21961691907786,-0.717894780174561,
11.3920197673161));
#20664=CARTESIAN_POINT('Ctrl Pts',(-9.03195918428354,-0.906002682172381,
11.4045007005643));
#20665=CARTESIAN_POINT('Ctrl Pts',(-8.76814132834394,-1.01583545019905,
11.4169816338125));
#20666=CARTESIAN_POINT('Ctrl Pts',(-8.50243547044518,-1.0164720823066,11.4294625670606));
#20667=CARTESIAN_POINT('Ctrl Pts',(-8.23672961254641,-1.01710871441415,
11.4419435003088));
#20668=CARTESIAN_POINT('Ctrl Pts',(-7.97238846933345,-0.908541417082817,
11.454424433557));
#20669=CARTESIAN_POINT('Ctrl Pts',(-7.78383148002347,-0.721334926798654,
11.4669053668052));
#20670=CARTESIAN_POINT('Ctrl Pts',(-7.59527449071349,-0.534128436514492,
11.4793863000534));
#20671=CARTESIAN_POINT('Ctrl Pts',(-7.48480993131705,-0.270574496755817,
11.4918672333016));
#20672=CARTESIAN_POINT('Ctrl Pts',(-7.48353667075686,-0.00487092690831965,
11.5043481665498));
#20673=CARTESIAN_POINT('Ctrl Pts',(-7.48226341019666,0.260832642939178,
11.516829099798));
#20674=CARTESIAN_POINT('Ctrl Pts',(-7.59019703546749,0.525433154240395,
11.5293100330462));
#20675=CARTESIAN_POINT('Ctrl Pts',(-7.77695120652516,0.71443814839325,11.5417909662944));
#20676=CARTESIAN_POINT('Ctrl Pts',(-7.96370537758283,0.903443142546105,
11.5542718995426));
#20677=CARTESIAN_POINT('Ctrl Pts',(-8.22699388814827,1.01453885915659,11.5667528327907));
#20678=CARTESIAN_POINT('Ctrl Pts',(-8.49269364459159,1.01644874085988,11.5792337660389));
#20679=CARTESIAN_POINT('Ctrl Pts',(-8.7583934010349,1.01835862256318,11.5917146992871));
#20680=CARTESIAN_POINT('Ctrl Pts',(-9.0232517614039,0.911059288978973,11.6041956325353));
#20681=CARTESIAN_POINT('Ctrl Pts',(-9.21270367535844,0.724758509267449,
11.6166765657835));
#20682=CARTESIAN_POINT('Ctrl Pts',(-9.40215558931297,0.538457729555925,
11.6291574990317));
#20683=CARTESIAN_POINT('Ctrl Pts',(-9.51388182535844,0.275436159672238,
11.6416384322799));
#20684=CARTESIAN_POINT('Ctrl Pts',(-9.51642831724057,0.00974174196412615,
11.6541193655281));
#20685=CARTESIAN_POINT('Ctrl Pts',(-9.51645943884197,0.0064945940666019,
11.6542718995426));
#20686=CARTESIAN_POINT('Ctrl Pts',(-9.516475,0.00324729703376001,11.654424433557));
#20687=CARTESIAN_POINT('Ctrl Pts',(-9.516475,4.61410993834892E-13,11.6545769675715));
#20688=CARTESIAN_POINT('Origin',(-8.5,0.,1.24542303242842));
#20689=CARTESIAN_POINT('',(-9.516475,4.19524224387624E-13,10.9954230324285));
#20690=CARTESIAN_POINT('',(-9.516475,4.17578129052922E-13,11.0545769675715));
#20691=CARTESIAN_POINT('',(-9.516475,1.78524650477582E-12,1.24542303242842));
#20692=CARTESIAN_POINT('Ctrl Pts',(-9.51619870214038,-0.000607203370645813,
10.9954230324285));
#20693=CARTESIAN_POINT('Ctrl Pts',(-9.51677980361449,-0.106684728097461,
11.0003988638818));
#20694=CARTESIAN_POINT('Ctrl Pts',(-9.45103666736097,-0.551056728109718,
11.0212820364867));
#20695=CARTESIAN_POINT('Ctrl Pts',(-8.80852576484242,-1.162383479345,11.0580725502433));
#20696=CARTESIAN_POINT('Ctrl Pts',(-7.68802200901459,-0.88700948808109,
11.1057945736981));
#20697=CARTESIAN_POINT('Ctrl Pts',(-7.31554839363375,0.202723257387539,
11.153516597153));
#20698=CARTESIAN_POINT('Ctrl Pts',(-8.02922823218693,1.10655683650717,11.2012386206079));
#20699=CARTESIAN_POINT('Ctrl Pts',(-9.16742973518675,0.994609589396969,
11.2485407656997));
#20700=CARTESIAN_POINT('Ctrl Pts',(-9.51644808261045,0.328213381768027,
11.2799355696399));
#20701=CARTESIAN_POINT('Ctrl Pts',(-9.51769479449051,-0.000263157468651742,
11.2954230324285));
#20702=CARTESIAN_POINT('Ctrl Pts',(-9.516475,5.04248000332732E-13,11.0545769675715));
#20703=CARTESIAN_POINT('Ctrl Pts',(-9.51647500000013,-0.265706620583474,
11.0670579008197));
#20704=CARTESIAN_POINT('Ctrl Pts',(-9.40727465387221,-0.529786878176709,
11.0795388340679));
#20705=CARTESIAN_POINT('Ctrl Pts',(-9.21961691907789,-0.717894780174535,
11.0920197673161));
#20706=CARTESIAN_POINT('Ctrl Pts',(-9.03195918428357,-0.906002682172362,
11.1045007005643));
#20707=CARTESIAN_POINT('Ctrl Pts',(-8.76814132834398,-1.01583545019904,
11.1169816338125));
#20708=CARTESIAN_POINT('Ctrl Pts',(-8.50243547044521,-1.0164720823066,11.1294625670606));
#20709=CARTESIAN_POINT('Ctrl Pts',(-8.23672961254645,-1.01710871441416,
11.1419435003088));
#20710=CARTESIAN_POINT('Ctrl Pts',(-7.97238846933348,-0.908541417082836,
11.154424433557));
#20711=CARTESIAN_POINT('Ctrl Pts',(-7.78383148002349,-0.72133492679868,
11.1669053668052));
#20712=CARTESIAN_POINT('Ctrl Pts',(-7.5952744907135,-0.534128436514524,
11.1793863000534));
#20713=CARTESIAN_POINT('Ctrl Pts',(-7.48480993131706,-0.270574496755853,
11.1918672333016));
#20714=CARTESIAN_POINT('Ctrl Pts',(-7.48353667075686,-0.00487092690835552,
11.2043481665498));
#20715=CARTESIAN_POINT('Ctrl Pts',(-7.48226341019666,0.260832642939142,
11.216829099798));
#20716=CARTESIAN_POINT('Ctrl Pts',(-7.59019703546747,0.525433154240363,
11.2293100330462));
#20717=CARTESIAN_POINT('Ctrl Pts',(-7.77695120652513,0.714438148393224,
11.2417909662944));
#20718=CARTESIAN_POINT('Ctrl Pts',(-7.9637053775828,0.903443142546086,11.2542718995426));
#20719=CARTESIAN_POINT('Ctrl Pts',(-8.22699388814824,1.01453885915658,11.2667528327907));
#20720=CARTESIAN_POINT('Ctrl Pts',(-8.49269364459155,1.01644874085988,11.2792337660389));
#20721=CARTESIAN_POINT('Ctrl Pts',(-8.75839340103487,1.01835862256319,11.2917146992871));
#20722=CARTESIAN_POINT('Ctrl Pts',(-9.02325176140387,0.911059288978991,
11.3041956325353));
#20723=CARTESIAN_POINT('Ctrl Pts',(-9.21270367535841,0.724758509267474,
11.3166765657835));
#20724=CARTESIAN_POINT('Ctrl Pts',(-9.40215558931295,0.538457729555957,
11.3291574990317));
#20725=CARTESIAN_POINT('Ctrl Pts',(-9.51388182535843,0.275436159672273,
11.3416384322799));
#20726=CARTESIAN_POINT('Ctrl Pts',(-9.51642831724057,0.00974174196416202,
11.3541193655281));
#20727=CARTESIAN_POINT('Ctrl Pts',(-9.51645943884197,0.00649459406662814,
11.3542718995426));
#20728=CARTESIAN_POINT('Ctrl Pts',(-9.516475,0.00324729703377659,11.354424433557));
#20729=CARTESIAN_POINT('Ctrl Pts',(-9.516475,4.68384518537177E-13,11.3545769675715));
#20730=CARTESIAN_POINT('Origin',(-8.5,0.,1.24542303242842));
#20731=CARTESIAN_POINT('',(-9.51589299709112,9.73851207509147E-5,10.6954230324285));
#20732=CARTESIAN_POINT('',(-9.516475,3.95661696661937E-13,10.7545769675715));
#20733=CARTESIAN_POINT('',(-9.516475,1.78524650477582E-12,1.24542303242842));
#20734=CARTESIAN_POINT('Ctrl Pts',(-9.516475,3.9760784017564E-13,10.6954230324285));
#20735=CARTESIAN_POINT('Ctrl Pts',(-9.5164750000001,-0.265706620583571,
10.7079039656767));
#20736=CARTESIAN_POINT('Ctrl Pts',(-9.40727465387216,-0.529786878176785,
10.7203848989249));
#20737=CARTESIAN_POINT('Ctrl Pts',(-9.21961691907784,-0.717894780174591,
10.732865832173));
#20738=CARTESIAN_POINT('Ctrl Pts',(-9.03195918428351,-0.906002682172396,
10.7453467654212));
#20739=CARTESIAN_POINT('Ctrl Pts',(-8.76814132834392,-1.01583545019905,
10.7578276986694));
#20740=CARTESIAN_POINT('Ctrl Pts',(-8.50243547044516,-1.0164720823066,10.7703086319176));
#20741=CARTESIAN_POINT('Ctrl Pts',(-8.23672961254641,-1.01710871441414,
10.7827895651658));
#20742=CARTESIAN_POINT('Ctrl Pts',(-7.97238846933345,-0.908541417082819,
10.795270498414));
#20743=CARTESIAN_POINT('Ctrl Pts',(-7.78383148002348,-0.721334926798666,
10.8077514316622));
#20744=CARTESIAN_POINT('Ctrl Pts',(-7.5952744907135,-0.534128436514513,
10.8202323649104));
#20745=CARTESIAN_POINT('Ctrl Pts',(-7.48480993131706,-0.270574496755852,
10.8327132981586));
#20746=CARTESIAN_POINT('Ctrl Pts',(-7.48353667075686,-0.00487092690836444,
10.8451942314068));
#20747=CARTESIAN_POINT('Ctrl Pts',(-7.48226341019665,0.260832642939124,
10.857675164655));
#20748=CARTESIAN_POINT('Ctrl Pts',(-7.59019703546746,0.525433154240336,
10.8701560979031));
#20749=CARTESIAN_POINT('Ctrl Pts',(-7.77695120652511,0.714438148393197,
10.8826370311513));
#20750=CARTESIAN_POINT('Ctrl Pts',(-7.96370537758276,0.903443142546059,
10.8951179643995));
#20751=CARTESIAN_POINT('Ctrl Pts',(-8.22699388814818,1.01453885915656,10.9075988976477));
#20752=CARTESIAN_POINT('Ctrl Pts',(-8.49269364459149,1.01644874085988,10.9200798308959));
#20753=CARTESIAN_POINT('Ctrl Pts',(-8.75839340103479,1.0183586225632,10.9325607641441));
#20754=CARTESIAN_POINT('Ctrl Pts',(-9.02325176140379,0.911059288979034,
10.9450416973923));
#20755=CARTESIAN_POINT('Ctrl Pts',(-9.21270367535834,0.724758509267541,
10.9575226306405));
#20756=CARTESIAN_POINT('Ctrl Pts',(-9.4021555893129,0.538457729556049,10.9700035638887));
#20757=CARTESIAN_POINT('Ctrl Pts',(-9.5138818253584,0.275436159672388,10.9824844971369));
#20758=CARTESIAN_POINT('Ctrl Pts',(-9.51642831724057,0.00974174196428649,
10.994965430385));
#20759=CARTESIAN_POINT('Ctrl Pts',(-9.51645943884197,0.00649459406669484,
10.9951179643995));
#20760=CARTESIAN_POINT('Ctrl Pts',(-9.516475,0.00324729703378546,10.995270498414));
#20761=CARTESIAN_POINT('Ctrl Pts',(-9.516475,4.19524272566625E-13,10.9954230324285));
#20762=CARTESIAN_POINT('Ctrl Pts',(-9.516475,4.24551653755207E-13,10.7545769675715));
#20763=CARTESIAN_POINT('Ctrl Pts',(-9.51647500000011,-0.265706620583535,
10.7670579008197));
#20764=CARTESIAN_POINT('Ctrl Pts',(-9.40727465387218,-0.529786878176742,
10.7795388340679));
#20765=CARTESIAN_POINT('Ctrl Pts',(-9.21961691907788,-0.717894780174551,
10.7920197673161));
#20766=CARTESIAN_POINT('Ctrl Pts',(-9.03195918428357,-0.90600268217236,
10.8045007005643));
#20767=CARTESIAN_POINT('Ctrl Pts',(-8.76814132834399,-1.01583545019903,
10.8169816338125));
#20768=CARTESIAN_POINT('Ctrl Pts',(-8.50243547044525,-1.0164720823066,10.8294625670606));
#20769=CARTESIAN_POINT('Ctrl Pts',(-8.2367296125465,-1.01710871441416,10.8419435003088));
#20770=CARTESIAN_POINT('Ctrl Pts',(-7.97238846933355,-0.908541417082871,
10.854424433557));
#20771=CARTESIAN_POINT('Ctrl Pts',(-7.78383148002356,-0.721334926798746,
10.8669053668052));
#20772=CARTESIAN_POINT('Ctrl Pts',(-7.59527449071357,-0.534128436514621,
10.8793863000534));
#20773=CARTESIAN_POINT('Ctrl Pts',(-7.4848099313171,-0.270574496755985,
10.8918672333016));
#20774=CARTESIAN_POINT('Ctrl Pts',(-7.48353667075686,-0.00487092690850694,
10.9043481665498));
#20775=CARTESIAN_POINT('Ctrl Pts',(-7.48226341019662,0.260832642938971,
10.916829099798));
#20776=CARTESIAN_POINT('Ctrl Pts',(-7.59019703546737,0.525433154240189,
10.9293100330462));
#20777=CARTESIAN_POINT('Ctrl Pts',(-7.77695120652499,0.714438148393076,
10.9417909662944));
#20778=CARTESIAN_POINT('Ctrl Pts',(-7.9637053775826,0.903443142545962,10.9542718995425));
#20779=CARTESIAN_POINT('Ctrl Pts',(-8.22699388814799,1.01453885915651,10.9667528327907));
#20780=CARTESIAN_POINT('Ctrl Pts',(-8.49269364459129,1.01644874085988,10.9792337660389));
#20781=CARTESIAN_POINT('Ctrl Pts',(-8.75839340103458,1.01835862256325,10.9917146992871));
#20782=CARTESIAN_POINT('Ctrl Pts',(-9.02325176140359,0.911059288979145,
11.0041956325353));
#20783=CARTESIAN_POINT('Ctrl Pts',(-9.21270367535818,0.724758509267702,
11.0166765657835));
#20784=CARTESIAN_POINT('Ctrl Pts',(-9.40215558931277,0.538457729556259,
11.0291574990317));
#20785=CARTESIAN_POINT('Ctrl Pts',(-9.51388182535833,0.275436159672636,
11.0416384322799));
#20786=CARTESIAN_POINT('Ctrl Pts',(-9.51642831724057,0.00974174196454454,
11.0541193655281));
#20787=CARTESIAN_POINT('Ctrl Pts',(-9.51645943884197,0.00649459406689512,
11.0542718995425));
#20788=CARTESIAN_POINT('Ctrl Pts',(-9.516475,0.00324729703392801,11.054424433557));
#20789=CARTESIAN_POINT('Ctrl Pts',(-9.516475,5.04248000332732E-13,11.0545769675715));
#20790=CARTESIAN_POINT('Origin',(-8.5,0.,1.24542303242842));
#20791=CARTESIAN_POINT('',(-9.51672077363507,0.000183314671464046,10.3954230324285));
#20792=CARTESIAN_POINT('',(-9.516475,3.73745264270951E-13,10.4545769675715));
#20793=CARTESIAN_POINT('',(-9.516475,1.78524650477582E-12,1.24542303242842));
#20794=CARTESIAN_POINT('Ctrl Pts',(-9.51772011037067,0.000928687888346325,
10.3954230324285));
#20795=CARTESIAN_POINT('Ctrl Pts',(-9.51551864793062,-0.297960855620615,
10.4095107700623));
#20796=CARTESIAN_POINT('Ctrl Pts',(-9.21783085496887,-0.93919810709799,
10.4395058488478));
#20797=CARTESIAN_POINT('Ctrl Pts',(-8.12901546541348,-1.14297541618665,
10.4854082687849));
#20798=CARTESIAN_POINT('Ctrl Pts',(-7.33723505164926,-0.306711207290376,
10.5331302922398));
#20799=CARTESIAN_POINT('Ctrl Pts',(-7.61417160911282,0.813407377962594,
10.5808523156946));
#20800=CARTESIAN_POINT('Ctrl Pts',(-8.52205763101126,1.12124235117773,10.6206206685737));
#20801=CARTESIAN_POINT('Ctrl Pts',(-9.1565775804327,0.82795583618433,10.6524353508769));
#20802=CARTESIAN_POINT('Ctrl Pts',(-9.45785075121687,0.442033743097962,
10.6747182486366));
#20803=CARTESIAN_POINT('Ctrl Pts',(-9.51514599649507,0.136437782201491,
10.6890474758204));
#20804=CARTESIAN_POINT('Ctrl Pts',(-9.51462354101672,0.000309800094462256,
10.6954230324285));
#20805=CARTESIAN_POINT('Ctrl Pts',(-9.516475,4.31525178457491E-13,10.4545769675715));
#20806=CARTESIAN_POINT('Ctrl Pts',(-9.51647500000011,-0.265706620583547,
10.4670579008197));
#20807=CARTESIAN_POINT('Ctrl Pts',(-9.40727465387217,-0.529786878176774,
10.4795388340679));
#20808=CARTESIAN_POINT('Ctrl Pts',(-9.21961691907784,-0.717894780174587,
10.4920197673161));
#20809=CARTESIAN_POINT('Ctrl Pts',(-9.03195918428351,-0.9060026821724,10.5045007005643));
#20810=CARTESIAN_POINT('Ctrl Pts',(-8.7681413283439,-1.01583545019906,10.5169816338125));
#20811=CARTESIAN_POINT('Ctrl Pts',(-8.50243547044514,-1.0164720823066,10.5294625670606));
#20812=CARTESIAN_POINT('Ctrl Pts',(-8.23672961254638,-1.01710871441414,
10.5419435003088));
#20813=CARTESIAN_POINT('Ctrl Pts',(-7.97238846933341,-0.908541417082798,
10.554424433557));
#20814=CARTESIAN_POINT('Ctrl Pts',(-7.78383148002344,-0.721334926798628,
10.5669053668052));
#20815=CARTESIAN_POINT('Ctrl Pts',(-7.59527449071347,-0.534128436514459,
10.5793863000534));
#20816=CARTESIAN_POINT('Ctrl Pts',(-7.48480993131704,-0.27057449675578,
10.5918672333016));
#20817=CARTESIAN_POINT('Ctrl Pts',(-7.48353667075686,-0.0048709269082828,
10.6043481665498));
#20818=CARTESIAN_POINT('Ctrl Pts',(-7.48226341019667,0.260832642939215,
10.616829099798));
#20819=CARTESIAN_POINT('Ctrl Pts',(-7.59019703546751,0.525433154240428,
10.6293100330462));
#20820=CARTESIAN_POINT('Ctrl Pts',(-7.77695120652518,0.714438148393276,
10.6417909662944));
#20821=CARTESIAN_POINT('Ctrl Pts',(-7.96370537758286,0.903443142546124,
10.6542718995426));
#20822=CARTESIAN_POINT('Ctrl Pts',(-8.22699388814831,1.0145388591566,10.6667528327907));
#20823=CARTESIAN_POINT('Ctrl Pts',(-8.49269364459163,1.01644874085989,10.6792337660389));
#20824=CARTESIAN_POINT('Ctrl Pts',(-8.75839340103494,1.01835862256317,10.6917146992871));
#20825=CARTESIAN_POINT('Ctrl Pts',(-9.02325176140394,0.911059288978954,
10.7041956325353));
#20826=CARTESIAN_POINT('Ctrl Pts',(-9.21270367535846,0.724758509267423,
10.7166765657835));
#20827=CARTESIAN_POINT('Ctrl Pts',(-9.40215558931299,0.538457729555893,
10.7291574990317));
#20828=CARTESIAN_POINT('Ctrl Pts',(-9.51388182535845,0.275436159672201,
10.7416384322799));
#20829=CARTESIAN_POINT('Ctrl Pts',(-9.51642831724057,0.0097417419640893,
10.7541193655281));
#20830=CARTESIAN_POINT('Ctrl Pts',(-9.51645943884197,0.00649459406656504,
10.7542718995426));
#20831=CARTESIAN_POINT('Ctrl Pts',(-9.516475,0.00324729703372315,10.754424433557));
#20832=CARTESIAN_POINT('Ctrl Pts',(-9.516475,4.24551653755207E-13,10.7545769675715));
#20833=CARTESIAN_POINT('Origin',(-8.5,0.,1.24542303242842));
#20834=CARTESIAN_POINT('',(-9.516475,3.248850183004E-13,10.0954230324285));
#20835=CARTESIAN_POINT('',(-9.516475,3.51828831879967E-13,10.1545769675715));
#20836=CARTESIAN_POINT('',(-9.516475,1.78524650477582E-12,1.24542303242842));
#20837=CARTESIAN_POINT('Ctrl Pts',(-9.516475,3.5377497539367E-13,10.0954230324285));
#20838=CARTESIAN_POINT('Ctrl Pts',(-9.51647500000009,-0.265706620583625,
10.1079039656767));
#20839=CARTESIAN_POINT('Ctrl Pts',(-9.40727465387213,-0.529786878176844,
10.1203848989249));
#20840=CARTESIAN_POINT('Ctrl Pts',(-9.21961691907778,-0.717894780174642,
10.1328658321731));
#20841=CARTESIAN_POINT('Ctrl Pts',(-9.03195918428344,-0.906002682172441,
10.1453467654212));
#20842=CARTESIAN_POINT('Ctrl Pts',(-8.76814132834383,-1.01583545019908,
10.1578276986694));
#20843=CARTESIAN_POINT('Ctrl Pts',(-8.50243547044506,-1.0164720823066,10.1703086319176));
#20844=CARTESIAN_POINT('Ctrl Pts',(-8.2367296125463,-1.01710871441412,10.1827895651658));
#20845=CARTESIAN_POINT('Ctrl Pts',(-7.97238846933334,-0.908541417082758,
10.195270498414));
#20846=CARTESIAN_POINT('Ctrl Pts',(-7.78383148002338,-0.721334926798574,
10.2077514316622));
#20847=CARTESIAN_POINT('Ctrl Pts',(-7.59527449071343,-0.53412843651439,
10.2202323649104));
#20848=CARTESIAN_POINT('Ctrl Pts',(-7.48480993131702,-0.270574496755703,
10.2327132981586));
#20849=CARTESIAN_POINT('Ctrl Pts',(-7.48353667075686,-0.00487092690820505,
10.2451942314068));
#20850=CARTESIAN_POINT('Ctrl Pts',(-7.48226341019669,0.260832642939293,
10.257675164655));
#20851=CARTESIAN_POINT('Ctrl Pts',(-7.59019703546755,0.525433154240497,
10.2701560979032));
#20852=CARTESIAN_POINT('Ctrl Pts',(-7.77695120652524,0.714438148393331,
10.2826370311513));
#20853=CARTESIAN_POINT('Ctrl Pts',(-7.96370537758293,0.903443142546165,
10.2951179643995));
#20854=CARTESIAN_POINT('Ctrl Pts',(-8.22699388814839,1.01453885915662,10.3075988976477));
#20855=CARTESIAN_POINT('Ctrl Pts',(-8.4926936445917,1.01644874085989,10.3200798308959));
#20856=CARTESIAN_POINT('Ctrl Pts',(-8.75839340103502,1.01835862256315,10.3325607641441));
#20857=CARTESIAN_POINT('Ctrl Pts',(-9.023251761404,0.911059288978914,10.3450416973923));
#20858=CARTESIAN_POINT('Ctrl Pts',(-9.21270367535852,0.724758509267369,
10.3575226306405));
#20859=CARTESIAN_POINT('Ctrl Pts',(-9.40215558931303,0.538457729555824,
10.3700035638887));
#20860=CARTESIAN_POINT('Ctrl Pts',(-9.51388182535847,0.275436159672123,
10.3824844971369));
#20861=CARTESIAN_POINT('Ctrl Pts',(-9.51642831724057,0.00974174196401155,
10.3949654303851));
#20862=CARTESIAN_POINT('Ctrl Pts',(-9.51645943884197,0.00649459406649692,
10.3951179643995));
#20863=CARTESIAN_POINT('Ctrl Pts',(-9.516475,0.00324729703366459,10.395270498414));
#20864=CARTESIAN_POINT('Ctrl Pts',(-9.516475,3.75691407784655E-13,10.3954230324285));
#20865=CARTESIAN_POINT('Ctrl Pts',(-9.516475,3.80718788973236E-13,10.1545769675715));
#20866=CARTESIAN_POINT('Ctrl Pts',(-9.5164750000001,-0.265706620583598,
10.1670579008197));
#20867=CARTESIAN_POINT('Ctrl Pts',(-9.40727465387214,-0.529786878176819,
10.1795388340679));
#20868=CARTESIAN_POINT('Ctrl Pts',(-9.2196169190778,-0.717894780174623,
10.1920197673161));
#20869=CARTESIAN_POINT('Ctrl Pts',(-9.03195918428346,-0.906002682172426,
10.2045007005643));
#20870=CARTESIAN_POINT('Ctrl Pts',(-8.76814132834385,-1.01583545019907,
10.2169816338125));
#20871=CARTESIAN_POINT('Ctrl Pts',(-8.50243547044509,-1.0164720823066,10.2294625670606));
#20872=CARTESIAN_POINT('Ctrl Pts',(-8.23672961254633,-1.01710871441412,
10.2419435003088));
#20873=CARTESIAN_POINT('Ctrl Pts',(-7.97238846933337,-0.908541417082772,
10.254424433557));
#20874=CARTESIAN_POINT('Ctrl Pts',(-7.7838314800234,-0.721334926798593,
10.2669053668052));
#20875=CARTESIAN_POINT('Ctrl Pts',(-7.59527449071344,-0.534128436514414,
10.2793863000534));
#20876=CARTESIAN_POINT('Ctrl Pts',(-7.48480993131703,-0.27057449675573,
10.2918672333016));
#20877=CARTESIAN_POINT('Ctrl Pts',(-7.48353667075686,-0.00487092690823199,
10.3043481665498));
#20878=CARTESIAN_POINT('Ctrl Pts',(-7.48226341019669,0.260832642939266,
10.316829099798));
#20879=CARTESIAN_POINT('Ctrl Pts',(-7.59019703546753,0.525433154240473,
10.3293100330462));
#20880=CARTESIAN_POINT('Ctrl Pts',(-7.77695120652522,0.714438148393312,
10.3417909662944));
#20881=CARTESIAN_POINT('Ctrl Pts',(-7.96370537758291,0.903443142546151,
10.3542718995426));
#20882=CARTESIAN_POINT('Ctrl Pts',(-8.22699388814836,1.01453885915662,10.3667528327907));
#20883=CARTESIAN_POINT('Ctrl Pts',(-8.49269364459168,1.01644874085989,10.3792337660389));
#20884=CARTESIAN_POINT('Ctrl Pts',(-8.75839340103499,1.01835862256316,10.3917146992871));
#20885=CARTESIAN_POINT('Ctrl Pts',(-9.02325176140398,0.911059288978928,
10.4041956325353));
#20886=CARTESIAN_POINT('Ctrl Pts',(-9.2127036753585,0.724758509267388,10.4166765657835));
#20887=CARTESIAN_POINT('Ctrl Pts',(-9.40215558931302,0.538457729555847,
10.4291574990317));
#20888=CARTESIAN_POINT('Ctrl Pts',(-9.51388182535847,0.27543615967215,10.4416384322799));
#20889=CARTESIAN_POINT('Ctrl Pts',(-9.51642831724057,0.00974174196403849,
10.4541193655281));
#20890=CARTESIAN_POINT('Ctrl Pts',(-9.51645943884197,0.0064945940665335,
10.4542718995426));
#20891=CARTESIAN_POINT('Ctrl Pts',(-9.516475,0.00324729703371082,10.454424433557));
#20892=CARTESIAN_POINT('Ctrl Pts',(-9.516475,4.31525178457491E-13,10.4545769675715));
#20893=CARTESIAN_POINT('Origin',(-8.5,0.,1.24542303242842));
#20894=CARTESIAN_POINT('',(-9.51618379816054,-4.38257510333499E-5,9.79542303242848));
#20895=CARTESIAN_POINT('',(-9.516475,3.29912399488981E-13,9.8545769675715));
#20896=CARTESIAN_POINT('',(-9.516475,1.78524650477582E-12,1.24542303242842));
#20897=CARTESIAN_POINT('Ctrl Pts',(-9.516475,3.31858543002685E-13,9.79542303242848));
#20898=CARTESIAN_POINT('Ctrl Pts',(-9.51647500000009,-0.265706620583637,
9.80790396567667));
#20899=CARTESIAN_POINT('Ctrl Pts',(-9.40727465387213,-0.529786878176844,
9.82038489892486));
#20900=CARTESIAN_POINT('Ctrl Pts',(-9.21961691907779,-0.717894780174637,
9.83286583217305));
#20901=CARTESIAN_POINT('Ctrl Pts',(-9.03195918428345,-0.90600268217243,
9.84534676542124));
#20902=CARTESIAN_POINT('Ctrl Pts',(-8.76814132834385,-1.01583545019907,
9.85782769866943));
#20903=CARTESIAN_POINT('Ctrl Pts',(-8.5024354704451,-1.0164720823066,9.87030863191762));
#20904=CARTESIAN_POINT('Ctrl Pts',(-8.23672961254634,-1.01710871441413,
9.88278956516581));
#20905=CARTESIAN_POINT('Ctrl Pts',(-7.97238846933339,-0.908541417082785,
9.895270498414));
#20906=CARTESIAN_POINT('Ctrl Pts',(-7.78383148002343,-0.721334926798619,
9.90775143166219));
#20907=CARTESIAN_POINT('Ctrl Pts',(-7.59527449071347,-0.534128436514454,
9.92023236491038));
#20908=CARTESIAN_POINT('Ctrl Pts',(-7.48480993131704,-0.270574496755787,
9.93271329815857));
#20909=CARTESIAN_POINT('Ctrl Pts',(-7.48353667075686,-0.00487092690829869,
9.94519423140676));
#20910=CARTESIAN_POINT('Ctrl Pts',(-7.48226341019667,0.260832642939189,
9.95767516465495));
#20911=CARTESIAN_POINT('Ctrl Pts',(-7.59019703546749,0.525433154240395,
9.97015609790315));
#20912=CARTESIAN_POINT('Ctrl Pts',(-7.77695120652515,0.714438148393244,
9.98263703115134));
#20913=CARTESIAN_POINT('Ctrl Pts',(-7.96370537758281,0.903443142546094,
9.99511796439953));
#20914=CARTESIAN_POINT('Ctrl Pts',(-8.22699388814825,1.01453885915658,10.0075988976477));
#20915=CARTESIAN_POINT('Ctrl Pts',(-8.49269364459155,1.01644874085988,10.0200798308959));
#20916=CARTESIAN_POINT('Ctrl Pts',(-8.75839340103486,1.01835862256319,10.0325607641441));
#20917=CARTESIAN_POINT('Ctrl Pts',(-9.02325176140385,0.911059288979,10.0450416973923));
#20918=CARTESIAN_POINT('Ctrl Pts',(-9.21270367535839,0.724758509267495,
10.0575226306405));
#20919=CARTESIAN_POINT('Ctrl Pts',(-9.40215558931293,0.53845772955599,10.0700035638887));
#20920=CARTESIAN_POINT('Ctrl Pts',(-9.51388182535842,0.275436159672322,
10.0824844971369));
#20921=CARTESIAN_POINT('Ctrl Pts',(-9.51642831724057,0.00974174196422074,
10.0949654303851));
#20922=CARTESIAN_POINT('Ctrl Pts',(-9.51645943884197,0.00649459406662909,
10.0951179643995));
#20923=CARTESIAN_POINT('Ctrl Pts',(-9.516475,0.00324729703371972,10.095270498414));
#20924=CARTESIAN_POINT('Ctrl Pts',(-9.516475,3.5377497539367E-13,10.0954230324285));
#20925=CARTESIAN_POINT('Ctrl Pts',(-9.516475,3.87692313675521E-13,9.8545769675715));
#20926=CARTESIAN_POINT('Ctrl Pts',(-9.5164750000001,-0.265706620583571,
9.86705790081969));
#20927=CARTESIAN_POINT('Ctrl Pts',(-9.40727465387216,-0.529786878176775,
9.87953883406788));
#20928=CARTESIAN_POINT('Ctrl Pts',(-9.21961691907785,-0.717894780174577,
9.89201976731607));
#20929=CARTESIAN_POINT('Ctrl Pts',(-9.03195918428353,-0.906002682172379,
9.90450070056426));
#20930=CARTESIAN_POINT('Ctrl Pts',(-8.76814132834396,-1.01583545019904,
9.91698163381245));
#20931=CARTESIAN_POINT('Ctrl Pts',(-8.50243547044521,-1.0164720823066,9.92946256706064));
#20932=CARTESIAN_POINT('Ctrl Pts',(-8.23672961254647,-1.01710871441415,
9.94194350030883));
#20933=CARTESIAN_POINT('Ctrl Pts',(-7.97238846933351,-0.908541417082852,
9.95442443355702));
#20934=CARTESIAN_POINT('Ctrl Pts',(-7.78383148002353,-0.72133492679872,
9.96690536680521));
#20935=CARTESIAN_POINT('Ctrl Pts',(-7.59527449071355,-0.534128436514588,
9.9793863000534));
#20936=CARTESIAN_POINT('Ctrl Pts',(-7.48480993131709,-0.270574496755948,
9.99186723330159));
#20937=CARTESIAN_POINT('Ctrl Pts',(-7.48353667075686,-0.00487092690847008,
10.0043481665498));
#20938=CARTESIAN_POINT('Ctrl Pts',(-7.48226341019663,0.260832642939008,
10.016829099798));
#20939=CARTESIAN_POINT('Ctrl Pts',(-7.59019703546739,0.525433154240222,
10.0293100330462));
#20940=CARTESIAN_POINT('Ctrl Pts',(-7.77695120652501,0.714438148393102,
10.0417909662944));
#20941=CARTESIAN_POINT('Ctrl Pts',(-7.96370537758263,0.903443142545981,
10.0542718995425));
#20942=CARTESIAN_POINT('Ctrl Pts',(-8.22699388814803,1.01453885915652,10.0667528327907));
#20943=CARTESIAN_POINT('Ctrl Pts',(-8.49269364459132,1.01644874085988,10.0792337660389));
#20944=CARTESIAN_POINT('Ctrl Pts',(-8.75839340103462,1.01835862256325,10.0917146992871));
#20945=CARTESIAN_POINT('Ctrl Pts',(-9.02325176140362,0.911059288979126,
10.1041956325353));
#20946=CARTESIAN_POINT('Ctrl Pts',(-9.21270367535821,0.724758509267676,
10.1166765657835));
#20947=CARTESIAN_POINT('Ctrl Pts',(-9.40215558931279,0.538457729556226,
10.1291574990317));
#20948=CARTESIAN_POINT('Ctrl Pts',(-9.51388182535834,0.275436159672599,
10.1416384322799));
#20949=CARTESIAN_POINT('Ctrl Pts',(-9.51642831724057,0.00974174196450768,
10.1541193655281));
#20950=CARTESIAN_POINT('Ctrl Pts',(-9.51645943884197,0.00649459406682937,
10.1542718995425));
#20951=CARTESIAN_POINT('Ctrl Pts',(-9.516475,0.00324729703383339,10.154424433557));
#20952=CARTESIAN_POINT('Ctrl Pts',(-9.516475,3.80718788973236E-13,10.1545769675715));
#20953=CARTESIAN_POINT('Origin',(-8.5,0.,1.24542303242842));
#20954=CARTESIAN_POINT('',(-9.51617051050046,0.000917125635492296,9.49542303242848));
#20955=CARTESIAN_POINT('',(-9.516475,3.07995967097996E-13,9.55457696757151));
#20956=CARTESIAN_POINT('',(-9.516475,1.78524650477582E-12,1.24542303242842));
#20957=CARTESIAN_POINT('Ctrl Pts',(-9.51617051050046,0.000917125635492358,
9.49542303242848));
#20958=CARTESIAN_POINT('Ctrl Pts',(-9.51399210699604,-0.251361202752491,
9.50727128818155));
#20959=CARTESIAN_POINT('Ctrl Pts',(-9.29182487903127,-0.845882765186451,
9.53502688508624));
#20960=CARTESIAN_POINT('Ctrl Pts',(-8.29189791040081,-1.18449019452684,
9.57868982314254));
#20961=CARTESIAN_POINT('Ctrl Pts',(-7.54347150337463,-0.585426497780913,
9.61845817602161));
#20962=CARTESIAN_POINT('Ctrl Pts',(-7.44875116596018,0.10714884380356,9.65027285832483));
#20963=CARTESIAN_POINT('Ctrl Pts',(-7.68125394638234,0.766371873730981,
9.6820875406281));
#20964=CARTESIAN_POINT('Ctrl Pts',(-8.5351536477378,1.20211801487063,9.72185589350713));
#20965=CARTESIAN_POINT('Ctrl Pts',(-9.37873992468116,0.708230622368606,
9.76228561429921));
#20966=CARTESIAN_POINT('Ctrl Pts',(-9.51456966231208,0.18381057644297,9.78680799393966));
#20967=CARTESIAN_POINT('Ctrl Pts',(-9.51485924948736,-0.00024316975562387,
9.79542303242848));
#20968=CARTESIAN_POINT('Ctrl Pts',(-9.516475,3.07995967097996E-13,9.55457696757151));
#20969=CARTESIAN_POINT('Ctrl Pts',(-9.51647500000008,-0.26570662058367,
9.5670579008197));
#20970=CARTESIAN_POINT('Ctrl Pts',(-9.4072746538721,-0.529786878176884,
9.57953883406789));
#20971=CARTESIAN_POINT('Ctrl Pts',(-9.21961691907775,-0.717894780174674,
9.59201976731608));
#20972=CARTESIAN_POINT('Ctrl Pts',(-9.0319591842834,-0.906002682172464,
9.60450070056427));
#20973=CARTESIAN_POINT('Ctrl Pts',(-8.76814132834378,-1.01583545019909,
9.61698163381246));
#20974=CARTESIAN_POINT('Ctrl Pts',(-8.50243547044502,-1.0164720823066,9.62946256706065));
#20975=CARTESIAN_POINT('Ctrl Pts',(-8.23672961254625,-1.0171087144141,9.64194350030884));
#20976=CARTESIAN_POINT('Ctrl Pts',(-7.9723884693333,-0.908541417082734,
9.65442443355703));
#20977=CARTESIAN_POINT('Ctrl Pts',(-7.78383148002335,-0.721334926798541,
9.66690536680522));
#20978=CARTESIAN_POINT('Ctrl Pts',(-7.5952744907134,-0.534128436514349,
9.67938630005342));
#20979=CARTESIAN_POINT('Ctrl Pts',(-7.48480993131701,-0.270574496755657,
9.6918672333016));
#20980=CARTESIAN_POINT('Ctrl Pts',(-7.48353667075686,-0.00487092690815927,
9.7043481665498));
#20981=CARTESIAN_POINT('Ctrl Pts',(-7.48226341019671,0.260832642939339,
9.71682909979799));
#20982=CARTESIAN_POINT('Ctrl Pts',(-7.59019703546757,0.525433154240539,
9.72931003304618));
#20983=CARTESIAN_POINT('Ctrl Pts',(-7.77695120652527,0.714438148393364,
9.74179096629437));
#20984=CARTESIAN_POINT('Ctrl Pts',(-7.96370537758297,0.903443142546189,
9.75427189954256));
#20985=CARTESIAN_POINT('Ctrl Pts',(-8.22699388814843,1.01453885915664,9.76675283279075));
#20986=CARTESIAN_POINT('Ctrl Pts',(-8.49269364459175,1.01644874085989,9.77923376603894));
#20987=CARTESIAN_POINT('Ctrl Pts',(-8.75839340103507,1.01835862256314,9.79171469928713));
#20988=CARTESIAN_POINT('Ctrl Pts',(-9.02325176140405,0.91105928897889,9.80419563253533));
#20989=CARTESIAN_POINT('Ctrl Pts',(-9.21270367535855,0.724758509267337,
9.81667656578352));
#20990=CARTESIAN_POINT('Ctrl Pts',(-9.40215558931306,0.538457729555783,
9.82915749903171));
#20991=CARTESIAN_POINT('Ctrl Pts',(-9.51388182535849,0.275436159672078,
9.8416384322799));
#20992=CARTESIAN_POINT('Ctrl Pts',(-9.51642831724057,0.00974174196396577,
9.85411936552809));
#20993=CARTESIAN_POINT('Ctrl Pts',(-9.51645943884197,0.0064945940664704,
9.85427189954256));
#20994=CARTESIAN_POINT('Ctrl Pts',(-9.516475,0.00324729703365738,9.85442443355703));
#20995=CARTESIAN_POINT('Ctrl Pts',(-9.516475,3.87692313675521E-13,9.8545769675715));
#20996=CARTESIAN_POINT('Origin',(-8.5,0.,1.24542303242842));
#20997=CARTESIAN_POINT('',(-9.51691224954345,-1.40868099694123E-5,9.19542303242848));
#20998=CARTESIAN_POINT('',(-9.516475,2.86079534707011E-13,9.25457696757151));
#20999=CARTESIAN_POINT('',(-9.516475,1.78524650477582E-12,1.24542303242842));
#21000=CARTESIAN_POINT('Ctrl Pts',(-9.51820343362973,-5.56847155661899E-5,
9.19542303242848));
#21001=CARTESIAN_POINT('Ctrl Pts',(-9.51823033311794,-0.0105875877906328,
9.19591990012021));
#21002=CARTESIAN_POINT('Ctrl Pts',(-9.51326527171217,-0.358286048382976,
9.21232410896355));
#21003=CARTESIAN_POINT('Ctrl Pts',(-9.11760907802098,-1.03193145478362,
9.24463565895851));
#21004=CARTESIAN_POINT('Ctrl Pts',(-8.15965436942419,-1.06856717192152,
9.28440401183757));
#21005=CARTESIAN_POINT('Ctrl Pts',(-7.63488434792032,-0.606778290914648,
9.3162186941408));
#21006=CARTESIAN_POINT('Ctrl Pts',(-7.37939961054365,0.0438829842956811,
9.34803337644406));
#21007=CARTESIAN_POINT('Ctrl Pts',(-7.74006457714768,0.932106031371996,
9.38780172932309));
#21008=CARTESIAN_POINT('Ctrl Pts',(-8.87452398480516,1.1427273841981,9.43552375277797));
#21009=CARTESIAN_POINT('Ctrl Pts',(-9.46709300437131,0.511607309487474,
9.47139752047976));
#21010=CARTESIAN_POINT('Ctrl Pts',(-9.5169168081869,0.0873449763227789,
9.49136394702993));
#21011=CARTESIAN_POINT('Ctrl Pts',(-9.51617051050046,0.000917125635492358,
9.49542303242848));
#21012=CARTESIAN_POINT('Ctrl Pts',(-9.516475,3.14969491800281E-13,9.25457696757151));
#21013=CARTESIAN_POINT('Ctrl Pts',(-9.51647500000008,-0.265706620583654,
9.2670579008197));
#21014=CARTESIAN_POINT('Ctrl Pts',(-9.40727465387212,-0.529786878176859,
9.27953883406789));
#21015=CARTESIAN_POINT('Ctrl Pts',(-9.21961691907778,-0.717894780174649,
9.29201976731608));
#21016=CARTESIAN_POINT('Ctrl Pts',(-9.03195918428344,-0.906002682172439,
9.30450070056427));
#21017=CARTESIAN_POINT('Ctrl Pts',(-8.76814132834383,-1.01583545019907,
9.31698163381246));
#21018=CARTESIAN_POINT('Ctrl Pts',(-8.50243547044508,-1.0164720823066,9.32946256706065));
#21019=CARTESIAN_POINT('Ctrl Pts',(-8.23672961254633,-1.01710871441412,
9.34194350030884));
#21020=CARTESIAN_POINT('Ctrl Pts',(-7.97238846933338,-0.908541417082776,
9.35442443355703));
#21021=CARTESIAN_POINT('Ctrl Pts',(-7.78383148002342,-0.721334926798607,
9.36690536680522));
#21022=CARTESIAN_POINT('Ctrl Pts',(-7.59527449071346,-0.534128436514439,
9.37938630005341));
#21023=CARTESIAN_POINT('Ctrl Pts',(-7.48480993131704,-0.27057449675577,
9.3918672333016));
#21024=CARTESIAN_POINT('Ctrl Pts',(-7.48353667075686,-0.0048709269082818,
9.40434816654979));
#21025=CARTESIAN_POINT('Ctrl Pts',(-7.48226341019668,0.260832642939206,
9.41682909979798));
#21026=CARTESIAN_POINT('Ctrl Pts',(-7.5901970354675,0.52543315424041,9.42931003304617));
#21027=CARTESIAN_POINT('Ctrl Pts',(-7.77695120652516,0.714438148393256,
9.44179096629436));
#21028=CARTESIAN_POINT('Ctrl Pts',(-7.96370537758283,0.903443142546102,
9.45427189954255));
#21029=CARTESIAN_POINT('Ctrl Pts',(-8.22699388814826,1.01453885915659,9.46675283279074));
#21030=CARTESIAN_POINT('Ctrl Pts',(-8.49269364459157,1.01644874085988,9.47923376603893));
#21031=CARTESIAN_POINT('Ctrl Pts',(-8.75839340103487,1.01835862256318,9.49171469928712));
#21032=CARTESIAN_POINT('Ctrl Pts',(-9.02325176140386,0.911059288978991,
9.50419563253532));
#21033=CARTESIAN_POINT('Ctrl Pts',(-9.2127036753584,0.724758509267483,9.51667656578351));
#21034=CARTESIAN_POINT('Ctrl Pts',(-9.40215558931294,0.538457729555975,
9.5291574990317));
#21035=CARTESIAN_POINT('Ctrl Pts',(-9.51388182535842,0.275436159672306,
9.54163843227989));
#21036=CARTESIAN_POINT('Ctrl Pts',(-9.51642831724057,0.00974174196420385,
9.55411936552808));
#21037=CARTESIAN_POINT('Ctrl Pts',(-9.51645943884197,0.00649459406660257,
9.55427189954255));
#21038=CARTESIAN_POINT('Ctrl Pts',(-9.516475,0.00324729703368363,9.55442443355703));
#21039=CARTESIAN_POINT('Ctrl Pts',(-9.516475,3.07995967097996E-13,9.55457696757151));
#21040=CARTESIAN_POINT('Origin',(-8.5,0.,1.24542303242842));
#21041=CARTESIAN_POINT('',(-9.516475,2.3721928873646E-13,8.89542303242848));
#21042=CARTESIAN_POINT('',(-9.516475,2.64163102316026E-13,8.95457696757151));
#21043=CARTESIAN_POINT('',(-9.516475,1.78524650477582E-12,1.24542303242842));
#21044=CARTESIAN_POINT('Ctrl Pts',(-9.516475,2.66109245829729E-13,8.89542303242848));
#21045=CARTESIAN_POINT('Ctrl Pts',(-9.51647500000007,-0.265706620583703,
8.90790396567667));
#21046=CARTESIAN_POINT('Ctrl Pts',(-9.40727465387209,-0.529786878176903,
8.92038489892486));
#21047=CARTESIAN_POINT('Ctrl Pts',(-9.21961691907774,-0.717894780174684,
8.93286583217305));
#21048=CARTESIAN_POINT('Ctrl Pts',(-9.03195918428339,-0.906002682172464,
8.94534676542124));
#21049=CARTESIAN_POINT('Ctrl Pts',(-8.76814132834379,-1.01583545019909,
8.95782769866944));
#21050=CARTESIAN_POINT('Ctrl Pts',(-8.50243547044503,-1.0164720823066,8.97030863191763));
#21051=CARTESIAN_POINT('Ctrl Pts',(-8.23672961254628,-1.01710871441411,
8.98278956516581));
#21052=CARTESIAN_POINT('Ctrl Pts',(-7.97238846933334,-0.90854141708275,
8.99527049841401));
#21053=CARTESIAN_POINT('Ctrl Pts',(-7.78383148002338,-0.721334926798573,
9.0077514316622));
#21054=CARTESIAN_POINT('Ctrl Pts',(-7.59527449071343,-0.534128436514395,
9.02023236491039));
#21055=CARTESIAN_POINT('Ctrl Pts',(-7.48480993131703,-0.270574496755721,
9.03271329815858));
#21056=CARTESIAN_POINT('Ctrl Pts',(-7.48353667075686,-0.00487092690823294,
9.04519423140677));
#21057=CARTESIAN_POINT('Ctrl Pts',(-7.48226341019669,0.260832642939255,
9.05767516465496));
#21058=CARTESIAN_POINT('Ctrl Pts',(-7.59019703546752,0.525433154240453,
9.07015609790315));
#21059=CARTESIAN_POINT('Ctrl Pts',(-7.7769512065252,0.714438148393291,9.08263703115134));
#21060=CARTESIAN_POINT('Ctrl Pts',(-7.96370537758287,0.903443142546128,
9.09511796439953));
#21061=CARTESIAN_POINT('Ctrl Pts',(-8.22699388814831,1.0145388591566,9.10759889764772));
#21062=CARTESIAN_POINT('Ctrl Pts',(-8.49269364459162,1.01644874085989,9.12007983089591));
#21063=CARTESIAN_POINT('Ctrl Pts',(-8.75839340103493,1.01835862256317,9.1325607641441));
#21064=CARTESIAN_POINT('Ctrl Pts',(-9.02325176140391,0.911059288978966,
9.14504169739229));
#21065=CARTESIAN_POINT('Ctrl Pts',(-9.21270367535844,0.724758509267449,
9.15752263064048));
#21066=CARTESIAN_POINT('Ctrl Pts',(-9.40215558931297,0.538457729555932,
9.17000356388867));
#21067=CARTESIAN_POINT('Ctrl Pts',(-9.51388182535843,0.275436159672257,
9.18248449713686));
#21068=CARTESIAN_POINT('Ctrl Pts',(-9.51642831724057,0.009741741964155,
9.19496543038505));
#21069=CARTESIAN_POINT('Ctrl Pts',(-9.51645943884197,0.00649459406656334,
9.19511796439953));
#21070=CARTESIAN_POINT('Ctrl Pts',(-9.516475,0.00324729703365397,9.19527049841401));
#21071=CARTESIAN_POINT('Ctrl Pts',(-9.516475,2.88025678220714E-13,9.19542303242848));
#21072=CARTESIAN_POINT('Ctrl Pts',(-9.516475,2.64163102316026E-13,8.95457696757151));
#21073=CARTESIAN_POINT('Ctrl Pts',(-9.51647500000007,-0.265706620583705,
8.9670579008197));
#21074=CARTESIAN_POINT('Ctrl Pts',(-9.40727465387209,-0.529786878176905,
8.97953883406789));
#21075=CARTESIAN_POINT('Ctrl Pts',(-9.21961691907774,-0.717894780174685,
8.99201976731608));
#21076=CARTESIAN_POINT('Ctrl Pts',(-9.03195918428339,-0.906002682172465,
9.00450070056427));
#21077=CARTESIAN_POINT('Ctrl Pts',(-8.76814132834378,-1.01583545019909,
9.01698163381246));
#21078=CARTESIAN_POINT('Ctrl Pts',(-8.50243547044503,-1.0164720823066,9.02946256706065));
#21079=CARTESIAN_POINT('Ctrl Pts',(-8.23672961254628,-1.01710871441411,
9.04194350030884));
#21080=CARTESIAN_POINT('Ctrl Pts',(-7.97238846933333,-0.908541417082749,
9.05442443355703));
#21081=CARTESIAN_POINT('Ctrl Pts',(-7.78383148002338,-0.721334926798572,
9.06690536680522));
#21082=CARTESIAN_POINT('Ctrl Pts',(-7.59527449071343,-0.534128436514394,
9.07938630005341));
#21083=CARTESIAN_POINT('Ctrl Pts',(-7.48480993131703,-0.270574496755719,
9.0918672333016));
#21084=CARTESIAN_POINT('Ctrl Pts',(-7.48353667075686,-0.004870926908231,
9.10434816654979));
#21085=CARTESIAN_POINT('Ctrl Pts',(-7.48226341019669,0.260832642939257,
9.11682909979798));
#21086=CARTESIAN_POINT('Ctrl Pts',(-7.59019703546753,0.525433154240455,
9.12931003304618));
#21087=CARTESIAN_POINT('Ctrl Pts',(-7.7769512065252,0.714438148393292,9.14179096629437));
#21088=CARTESIAN_POINT('Ctrl Pts',(-7.96370537758287,0.903443142546129,
9.15427189954256));
#21089=CARTESIAN_POINT('Ctrl Pts',(-8.22699388814831,1.0145388591566,9.16675283279075));
#21090=CARTESIAN_POINT('Ctrl Pts',(-8.49269364459162,1.01644874085989,9.17923376603894));
#21091=CARTESIAN_POINT('Ctrl Pts',(-8.75839340103493,1.01835862256317,9.19171469928713));
#21092=CARTESIAN_POINT('Ctrl Pts',(-9.02325176140391,0.911059288978965,
9.20419563253532));
#21093=CARTESIAN_POINT('Ctrl Pts',(-9.21270367535844,0.724758509267448,
9.21667656578351));
#21094=CARTESIAN_POINT('Ctrl Pts',(-9.40215558931297,0.53845772955593,9.2291574990317));
#21095=CARTESIAN_POINT('Ctrl Pts',(-9.51388182535844,0.275436159672255,
9.24163843227989));
#21096=CARTESIAN_POINT('Ctrl Pts',(-9.51642831724057,0.00974174196415305,
9.25411936552808));
#21097=CARTESIAN_POINT('Ctrl Pts',(-9.51645943884197,0.00649459406657102,
9.25427189954256));
#21098=CARTESIAN_POINT('Ctrl Pts',(-9.516475,0.0032472970336713,9.25442443355703));
#21099=CARTESIAN_POINT('Ctrl Pts',(-9.516475,3.14969491800281E-13,9.25457696757151));
#21100=CARTESIAN_POINT('Origin',(-8.5,0.,1.24542303242842));
#21101=CARTESIAN_POINT('',(-9.51616255555685,0.000140128590502373,8.59542303242849));
#21102=CARTESIAN_POINT('',(-9.516475,2.42246669925041E-13,8.65457696757151));
#21103=CARTESIAN_POINT('',(-9.516475,1.78524650477582E-12,1.24542303242842));
#21104=CARTESIAN_POINT('Ctrl Pts',(-9.516475,2.15302856345474E-13,8.59542303242849));
#21105=CARTESIAN_POINT('Ctrl Pts',(-9.51647500000006,-0.265706620583753,
8.60790396567667));
#21106=CARTESIAN_POINT('Ctrl Pts',(-9.40727465387207,-0.529786878176948,
8.62038489892487));
#21107=CARTESIAN_POINT('Ctrl Pts',(-9.21961691907771,-0.71789478017472,
8.63286583217306));
#21108=CARTESIAN_POINT('Ctrl Pts',(-9.03195918428335,-0.906002682172491,
8.64534676542125));
#21109=CARTESIAN_POINT('Ctrl Pts',(-8.76814132834373,-1.0158354501991,8.65782769866944));
#21110=CARTESIAN_POINT('Ctrl Pts',(-8.50243547044498,-1.0164720823066,8.67030863191763));
#21111=CARTESIAN_POINT('Ctrl Pts',(-8.23672961254623,-1.0171087144141,8.68278956516582));
#21112=CARTESIAN_POINT('Ctrl Pts',(-7.97238846933329,-0.908541417082724,
8.69527049841401));
#21113=CARTESIAN_POINT('Ctrl Pts',(-7.78383148002335,-0.721334926798537,
8.7077514316622));
#21114=CARTESIAN_POINT('Ctrl Pts',(-7.5952744907134,-0.53412843651435,8.72023236491039));
#21115=CARTESIAN_POINT('Ctrl Pts',(-7.48480993131701,-0.27057449675567,
8.73271329815858));
#21116=CARTESIAN_POINT('Ctrl Pts',(-7.48353667075686,-0.00487092690818213,
8.74519423140677));
#21117=CARTESIAN_POINT('Ctrl Pts',(-7.4822634101967,0.260832642939306,8.75767516465496));
#21118=CARTESIAN_POINT('Ctrl Pts',(-7.59019703546755,0.525433154240499,
8.77015609790315));
#21119=CARTESIAN_POINT('Ctrl Pts',(-7.77695120652523,0.714438148393327,
8.78263703115134));
#21120=CARTESIAN_POINT('Ctrl Pts',(-7.96370537758292,0.903443142546155,
8.79511796439953));
#21121=CARTESIAN_POINT('Ctrl Pts',(-8.22699388814836,1.01453885915661,8.80759889764772));
#21122=CARTESIAN_POINT('Ctrl Pts',(-8.49269364459167,1.01644874085989,8.82007983089591));
#21123=CARTESIAN_POINT('Ctrl Pts',(-8.75839340103498,1.01835862256316,8.8325607641441));
#21124=CARTESIAN_POINT('Ctrl Pts',(-9.02325176140395,0.91105928897894,8.8450416973923));
#21125=CARTESIAN_POINT('Ctrl Pts',(-9.21270367535847,0.724758509267413,
8.85752263064049));
#21126=CARTESIAN_POINT('Ctrl Pts',(-9.40215558931299,0.538457729555887,
8.87000356388867));
#21127=CARTESIAN_POINT('Ctrl Pts',(-9.51388182535845,0.275436159672206,
8.88248449713687));
#21128=CARTESIAN_POINT('Ctrl Pts',(-9.51642831724057,0.00974174196410419,
8.89496543038506));
#21129=CARTESIAN_POINT('Ctrl Pts',(-9.51645943884197,0.00649459406652216,
8.89511796439953));
#21130=CARTESIAN_POINT('Ctrl Pts',(-9.516475,0.00324729703362244,8.89527049841401));
#21131=CARTESIAN_POINT('Ctrl Pts',(-9.516475,2.66109245829729E-13,8.89542303242848));
#21132=CARTESIAN_POINT('Ctrl Pts',(-9.516475,2.71136627018311E-13,8.65457696757151));
#21133=CARTESIAN_POINT('Ctrl Pts',(-9.51647500000007,-0.265706620583707,
8.6670579008197));
#21134=CARTESIAN_POINT('Ctrl Pts',(-9.40727465387209,-0.529786878176917,
8.67953883406789));
#21135=CARTESIAN_POINT('Ctrl Pts',(-9.21961691907773,-0.717894780174701,
8.69201976731608));
#21136=CARTESIAN_POINT('Ctrl Pts',(-9.03195918428337,-0.906002682172484,
8.70450070056427));
#21137=CARTESIAN_POINT('Ctrl Pts',(-8.76814132834374,-1.0158354501991,8.71698163381246));
#21138=CARTESIAN_POINT('Ctrl Pts',(-8.50243547044498,-1.0164720823066,8.72946256706065));
#21139=CARTESIAN_POINT('Ctrl Pts',(-8.23672961254622,-1.01710871441409,
8.74194350030884));
#21140=CARTESIAN_POINT('Ctrl Pts',(-7.97238846933327,-0.908541417082715,
8.75442443355703));
#21141=CARTESIAN_POINT('Ctrl Pts',(-7.78383148002333,-0.721334926798515,
8.76690536680523));
#21142=CARTESIAN_POINT('Ctrl Pts',(-7.59527449071338,-0.534128436514316,
8.77938630005342));
#21143=CARTESIAN_POINT('Ctrl Pts',(-7.484809931317,-0.27057449675562,8.79186723330161));
#21144=CARTESIAN_POINT('Ctrl Pts',(-7.48353667075686,-0.00487092690812241,
8.8043481665498));
#21145=CARTESIAN_POINT('Ctrl Pts',(-7.48226341019672,0.260832642939375,
8.81682909979799));
#21146=CARTESIAN_POINT('Ctrl Pts',(-7.59019703546759,0.525433154240572,
8.82931003304618));
#21147=CARTESIAN_POINT('Ctrl Pts',(-7.7769512065253,0.71443814839339,8.84179096629437));
#21148=CARTESIAN_POINT('Ctrl Pts',(-7.963705377583,0.903443142546209,8.85427189954256));
#21149=CARTESIAN_POINT('Ctrl Pts',(-8.22699388814847,1.01453885915665,8.86675283279075));
#21150=CARTESIAN_POINT('Ctrl Pts',(-8.49269364459179,1.01644874085989,8.87923376603894));
#21151=CARTESIAN_POINT('Ctrl Pts',(-8.7583934010351,1.01835862256313,8.89171469928714));
#21152=CARTESIAN_POINT('Ctrl Pts',(-9.02325176140408,0.911059288978871,
8.90419563253533));
#21153=CARTESIAN_POINT('Ctrl Pts',(-9.21270367535858,0.724758509267311,
8.91667656578352));
#21154=CARTESIAN_POINT('Ctrl Pts',(-9.40215558931308,0.53845772955575,8.92915749903171));
#21155=CARTESIAN_POINT('Ctrl Pts',(-9.5138818253585,0.275436159672041,8.9416384322799));
#21156=CARTESIAN_POINT('Ctrl Pts',(-9.51642831724057,0.00974174196392891,
8.95411936552809));
#21157=CARTESIAN_POINT('Ctrl Pts',(-9.51645943884197,0.00649459406640466,
8.95427189954256));
#21158=CARTESIAN_POINT('Ctrl Pts',(-9.516475,0.00324729703356276,8.95442443355704));
#21159=CARTESIAN_POINT('Ctrl Pts',(-9.516475,2.64163102316026E-13,8.95457696757151));
#21160=CARTESIAN_POINT('Origin',(-8.5,0.,1.24542303242842));
#21161=CARTESIAN_POINT('',(-9.51660746771427,4.7561522507508E-5,8.29542303242849));
#21162=CARTESIAN_POINT('',(-9.51622101958584,6.09791478407872E-5,8.35457696757151));
#21163=CARTESIAN_POINT('',(-9.516475,1.78524650477582E-12,1.24542303242842));
#21164=CARTESIAN_POINT('Ctrl Pts',(-9.51755758975633,0.000388695593763897,
8.29542303242849));
#21165=CARTESIAN_POINT('Ctrl Pts',(-9.5169508547152,-0.131482241807455,
8.30163408881522));
#21166=CARTESIAN_POINT('Ctrl Pts',(-9.45475814244576,-0.43297838743787,
8.31579881577777));
#21167=CARTESIAN_POINT('Ctrl Pts',(-9.06669282573335,-0.967744899455822,
8.34587088389194));
#21168=CARTESIAN_POINT('Ctrl Pts',(-8.12407617387874,-1.14236805696769,
8.385639236771));
#21169=CARTESIAN_POINT('Ctrl Pts',(-7.3354977594041,-0.300047698604244,
8.43336126022585));
#21170=CARTESIAN_POINT('Ctrl Pts',(-7.61818561524077,0.816349017112872,
8.48108328368072));
#21171=CARTESIAN_POINT('Ctrl Pts',(-8.70950569765978,1.18414587464495,8.52880530713558));
#21172=CARTESIAN_POINT('Ctrl Pts',(-9.42871558275495,0.608006666036184,
8.56691855671817));
#21173=CARTESIAN_POINT('Ctrl Pts',(-9.51570104621182,0.135102786595141,
8.58912446514914));
#21174=CARTESIAN_POINT('Ctrl Pts',(-9.51489988985996,0.000706423072568199,
8.59542303242848));
#21175=CARTESIAN_POINT('Ctrl Pts',(-9.516475,2.20330237534056E-13,8.35457696757151));
#21176=CARTESIAN_POINT('Ctrl Pts',(-9.51647500000006,-0.265706620583758,
8.3670579008197));
#21177=CARTESIAN_POINT('Ctrl Pts',(-9.40727465387206,-0.529786878176963,
8.37953883406789));
#21178=CARTESIAN_POINT('Ctrl Pts',(-9.21961691907769,-0.717894780174737,
8.39201976731608));
#21179=CARTESIAN_POINT('Ctrl Pts',(-9.03195918428332,-0.90600268217251,
8.40450070056427));
#21180=CARTESIAN_POINT('Ctrl Pts',(-8.76814132834369,-1.01583545019911,
8.41698163381246));
#21181=CARTESIAN_POINT('Ctrl Pts',(-8.50243547044493,-1.0164720823066,8.42946256706066));
#21182=CARTESIAN_POINT('Ctrl Pts',(-8.23672961254617,-1.01710871441408,
8.44194350030885));
#21183=CARTESIAN_POINT('Ctrl Pts',(-7.97238846933322,-0.908541417082688,
8.45442443355704));
#21184=CARTESIAN_POINT('Ctrl Pts',(-7.78383148002329,-0.72133492679848,
8.46690536680523));
#21185=CARTESIAN_POINT('Ctrl Pts',(-7.59527449071336,-0.534128436514271,
8.47938630005342));
#21186=CARTESIAN_POINT('Ctrl Pts',(-7.48480993131698,-0.27057449675557,
8.49186723330161));
#21187=CARTESIAN_POINT('Ctrl Pts',(-7.48353667075686,-0.0048709269080716,
8.5043481665498));
#21188=CARTESIAN_POINT('Ctrl Pts',(-7.48226341019673,0.260832642939426,
8.51682909979799));
#21189=CARTESIAN_POINT('Ctrl Pts',(-7.59019703546762,0.525433154240617,
8.52931003304618));
#21190=CARTESIAN_POINT('Ctrl Pts',(-7.77695120652533,0.714438148393426,
8.54179096629437));
#21191=CARTESIAN_POINT('Ctrl Pts',(-7.96370537758305,0.903443142546235,
8.55427189954256));
#21192=CARTESIAN_POINT('Ctrl Pts',(-8.22699388814852,1.01453885915666,8.56675283279075));
#21193=CARTESIAN_POINT('Ctrl Pts',(-8.49269364459184,1.01644874085989,8.57923376603895));
#21194=CARTESIAN_POINT('Ctrl Pts',(-8.75839340103515,1.01835862256311,8.59171469928714));
#21195=CARTESIAN_POINT('Ctrl Pts',(-9.02325176140413,0.911059288978845,
8.60419563253533));
#21196=CARTESIAN_POINT('Ctrl Pts',(-9.21270367535861,0.724758509267275,
8.61667656578352));
#21197=CARTESIAN_POINT('Ctrl Pts',(-9.4021555893131,0.538457729555705,8.62915749903171));
#21198=CARTESIAN_POINT('Ctrl Pts',(-9.51388182535851,0.27543615967199,8.6416384322799));
#21199=CARTESIAN_POINT('Ctrl Pts',(-9.51642831724058,0.00974174196387811,
8.65411936552809));
#21200=CARTESIAN_POINT('Ctrl Pts',(-9.51645943884197,0.00649459406637311,
8.65427189954256));
#21201=CARTESIAN_POINT('Ctrl Pts',(-9.516475,0.00324729703355043,8.65442443355704));
#21202=CARTESIAN_POINT('Ctrl Pts',(-9.516475,2.71136627018311E-13,8.65457696757151));
#21203=CARTESIAN_POINT('Origin',(-8.5,0.,1.24542303242842));
#21204=CARTESIAN_POINT('',(-9.516475,1.71469991563504E-13,7.99542303242849));
#21205=CARTESIAN_POINT('',(-9.5164935018391,1.69134969809854E-5,8.05457696757151));
#21206=CARTESIAN_POINT('',(-9.516475,1.78524650477582E-12,1.24542303242842));
#21207=CARTESIAN_POINT('Ctrl Pts',(-9.516475,1.71469991563504E-13,7.99542303242849));
#21208=CARTESIAN_POINT('Ctrl Pts',(-9.51647500000004,-0.265706620583807,
8.00790396567668));
#21209=CARTESIAN_POINT('Ctrl Pts',(-9.40727465387203,-0.529786878177006,
8.02038489892487));
#21210=CARTESIAN_POINT('Ctrl Pts',(-9.21961691907766,-0.717894780174771,
8.03286583217306));
#21211=CARTESIAN_POINT('Ctrl Pts',(-9.03195918428328,-0.906002682172536,
8.04534676542125));
#21212=CARTESIAN_POINT('Ctrl Pts',(-8.76814132834364,-1.01583545019913,
8.05782769866944));
#21213=CARTESIAN_POINT('Ctrl Pts',(-8.50243547044488,-1.0164720823066,8.07030863191763));
#21214=CARTESIAN_POINT('Ctrl Pts',(-8.23672961254612,-1.01710871441407,
8.08278956516583));
#21215=CARTESIAN_POINT('Ctrl Pts',(-7.97238846933318,-0.908541417082663,
8.09527049841401));
#21216=CARTESIAN_POINT('Ctrl Pts',(-7.78383148002326,-0.721334926798445,
8.10775143166221));
#21217=CARTESIAN_POINT('Ctrl Pts',(-7.59527449071333,-0.534128436514227,
8.1202323649104));
#21218=CARTESIAN_POINT('Ctrl Pts',(-7.48480993131697,-0.270574496755521,
8.13271329815859));
#21219=CARTESIAN_POINT('Ctrl Pts',(-7.48353667075686,-0.00487092690802274,
8.14519423140678));
#21220=CARTESIAN_POINT('Ctrl Pts',(-7.48226341019674,0.260832642939475,
8.15767516465497));
#21221=CARTESIAN_POINT('Ctrl Pts',(-7.59019703546764,0.525433154240661,
8.17015609790316));
#21222=CARTESIAN_POINT('Ctrl Pts',(-7.77695120652537,0.714438148393461,
8.18263703115135));
#21223=CARTESIAN_POINT('Ctrl Pts',(-7.96370537758309,0.903443142546261,
8.19511796439954));
#21224=CARTESIAN_POINT('Ctrl Pts',(-8.22699388814857,1.01453885915667,8.20759889764773));
#21225=CARTESIAN_POINT('Ctrl Pts',(-8.49269364459189,1.01644874085989,8.22007983089592));
#21226=CARTESIAN_POINT('Ctrl Pts',(-8.7583934010352,1.0183586225631,8.23256076414412));
#21227=CARTESIAN_POINT('Ctrl Pts',(-9.02325176140417,0.91105928897882,8.2450416973923));
#21228=CARTESIAN_POINT('Ctrl Pts',(-9.21270367535865,0.724758509267241,
8.2575226306405));
#21229=CARTESIAN_POINT('Ctrl Pts',(-9.40215558931313,0.538457729555662,
8.27000356388869));
#21230=CARTESIAN_POINT('Ctrl Pts',(-9.51388182535852,0.275436159671942,
8.28248449713688));
#21231=CARTESIAN_POINT('Ctrl Pts',(-9.51642831724058,0.00974174196382925,
8.29496543038507));
#21232=CARTESIAN_POINT('Ctrl Pts',(-9.51645943884197,0.00649459406632425,
8.29511796439954));
#21233=CARTESIAN_POINT('Ctrl Pts',(-9.516475,0.00324729703350157,8.29527049841401));
#21234=CARTESIAN_POINT('Ctrl Pts',(-9.516475,2.22276381047759E-13,8.29542303242848));
#21235=CARTESIAN_POINT('Ctrl Pts',(-9.51728273352218,0.000738391526869241,
8.05457696757151));
#21236=CARTESIAN_POINT('Ctrl Pts',(-9.51495287138475,-0.289530015017073,
8.06824838978708));
#21237=CARTESIAN_POINT('Ctrl Pts',(-9.23304354846487,-0.921572807151517,
8.09782715315426));
#21238=CARTESIAN_POINT('Ctrl Pts',(-8.15787155631456,-1.15294042718917,
8.14331325767308));
#21239=CARTESIAN_POINT('Ctrl Pts',(-7.48282485956976,-0.472255950572485,
8.18308161055214));
#21240=CARTESIAN_POINT('Ctrl Pts',(-7.4678884532851,0.226607018726978,8.21489629285537));
#21241=CARTESIAN_POINT('Ctrl Pts',(-7.77421828515018,0.854933828755218,
8.24671097515861));
#21242=CARTESIAN_POINT('Ctrl Pts',(-8.67232841342475,1.19022116371383,8.28647932803768));
#21243=CARTESIAN_POINT('Ctrl Pts',(-9.41868698066376,0.629620601799731,
8.32508588236723));
#21244=CARTESIAN_POINT('Ctrl Pts',(-9.51557266316435,0.145416359173903,
8.34778509554518));
#21245=CARTESIAN_POINT('Ctrl Pts',(-9.51500553128436,0.000352810471975287,
8.35457696757151));
#21246=CARTESIAN_POINT('Origin',(-8.5,0.,1.24542303242842));
#21247=CARTESIAN_POINT('',(-9.516475,1.49553559172519E-13,7.69542303242849));
#21248=CARTESIAN_POINT('',(-9.516475,1.76497372752086E-13,7.75457696757151));
#21249=CARTESIAN_POINT('',(-9.516475,1.78524650477582E-12,1.24542303242842));
#21250=CARTESIAN_POINT('Ctrl Pts',(-9.516475,1.78443516265789E-13,7.69542303242849));
#21251=CARTESIAN_POINT('Ctrl Pts',(-9.51647500000005,-0.2657066205838,7.70790396567668));
#21252=CARTESIAN_POINT('Ctrl Pts',(-9.40727465387204,-0.529786878177,7.72038489892487));
#21253=CARTESIAN_POINT('Ctrl Pts',(-9.21961691907766,-0.717894780174766,
7.73286583217306));
#21254=CARTESIAN_POINT('Ctrl Pts',(-9.03195918428328,-0.906002682172532,
7.74534676542125));
#21255=CARTESIAN_POINT('Ctrl Pts',(-8.76814132834365,-1.01583545019913,
7.75782769866944));
#21256=CARTESIAN_POINT('Ctrl Pts',(-8.50243547044489,-1.0164720823066,7.77030863191763));
#21257=CARTESIAN_POINT('Ctrl Pts',(-8.23672961254612,-1.01710871441407,
7.78278956516582));
#21258=CARTESIAN_POINT('Ctrl Pts',(-7.97238846933319,-0.908541417082667,
7.79527049841401));
#21259=CARTESIAN_POINT('Ctrl Pts',(-7.78383148002326,-0.72133492679845,
7.80775143166221));
#21260=CARTESIAN_POINT('Ctrl Pts',(-7.59527449071333,-0.534128436514233,
7.8202323649104));
#21261=CARTESIAN_POINT('Ctrl Pts',(-7.48480993131697,-0.270574496755528,
7.83271329815859));
#21262=CARTESIAN_POINT('Ctrl Pts',(-7.48353667075686,-0.00487092690802972,
7.84519423140678));
#21263=CARTESIAN_POINT('Ctrl Pts',(-7.48226341019674,0.260832642939468,
7.85767516465497));
#21264=CARTESIAN_POINT('Ctrl Pts',(-7.59019703546764,0.525433154240655,
7.87015609790316));
#21265=CARTESIAN_POINT('Ctrl Pts',(-7.77695120652536,0.714438148393456,
7.88263703115135));
#21266=CARTESIAN_POINT('Ctrl Pts',(-7.96370537758309,0.903443142546258,
7.89511796439954));
#21267=CARTESIAN_POINT('Ctrl Pts',(-8.22699388814856,1.01453885915667,7.90759889764773));
#21268=CARTESIAN_POINT('Ctrl Pts',(-8.49269364459188,1.01644874085989,7.92007983089592));
#21269=CARTESIAN_POINT('Ctrl Pts',(-8.7583934010352,1.0183586225631,7.93256076414411));
#21270=CARTESIAN_POINT('Ctrl Pts',(-9.02325176140416,0.911059288978824,
7.94504169739231));
#21271=CARTESIAN_POINT('Ctrl Pts',(-9.21270367535864,0.724758509267246,
7.9575226306405));
#21272=CARTESIAN_POINT('Ctrl Pts',(-9.40215558931313,0.538457729555668,
7.97000356388869));
#21273=CARTESIAN_POINT('Ctrl Pts',(-9.51388182535852,0.275436159671948,
7.98248449713688));
#21274=CARTESIAN_POINT('Ctrl Pts',(-9.51642831724058,0.00974174196383622,
7.99496543038507));
#21275=CARTESIAN_POINT('Ctrl Pts',(-9.51645943884197,0.00649459406631196,
7.99511796439954));
#21276=CARTESIAN_POINT('Ctrl Pts',(-9.516475,0.00324729703347002,7.99527049841402));
#21277=CARTESIAN_POINT('Ctrl Pts',(-9.516475,1.71469991563504E-13,7.99542303242849));
#21278=CARTESIAN_POINT('Ctrl Pts',(-9.516475,1.76497372752086E-13,7.75457696757151));
#21279=CARTESIAN_POINT('Ctrl Pts',(-9.51647500000005,-0.265706620583783,
7.7670579008197));
#21280=CARTESIAN_POINT('Ctrl Pts',(-9.40727465387205,-0.529786878176964,
7.77953883406789));
#21281=CARTESIAN_POINT('Ctrl Pts',(-9.2196169190777,-0.717894780174727,
7.79201976731608));
#21282=CARTESIAN_POINT('Ctrl Pts',(-9.03195918428335,-0.906002682172489,
7.80450070056427));
#21283=CARTESIAN_POINT('Ctrl Pts',(-8.76814132834375,-1.0158354501991,7.81698163381246));
#21284=CARTESIAN_POINT('Ctrl Pts',(-8.502435470445,-1.0164720823066,7.82946256706065));
#21285=CARTESIAN_POINT('Ctrl Pts',(-8.23672961254626,-1.0171087144141,7.84194350030884));
#21286=CARTESIAN_POINT('Ctrl Pts',(-7.97238846933333,-0.908541417082742,
7.85442443355703));
#21287=CARTESIAN_POINT('Ctrl Pts',(-7.78383148002338,-0.721334926798571,
7.86690536680522));
#21288=CARTESIAN_POINT('Ctrl Pts',(-7.59527449071344,-0.5341284365144,7.87938630005341));
#21289=CARTESIAN_POINT('Ctrl Pts',(-7.48480993131703,-0.270574496755737,
7.8918672333016));
#21290=CARTESIAN_POINT('Ctrl Pts',(-7.48353667075686,-0.00487092690825889,
7.90434816654979));
#21291=CARTESIAN_POINT('Ctrl Pts',(-7.48226341019668,0.26083264293922,7.91682909979798));
#21292=CARTESIAN_POINT('Ctrl Pts',(-7.5901970354675,0.525433154240411,7.92931003304617));
#21293=CARTESIAN_POINT('Ctrl Pts',(-7.77695120652516,0.714438148393252,
7.94179096629436));
#21294=CARTESIAN_POINT('Ctrl Pts',(-7.96370537758282,0.903443142546093,
7.95427189954255));
#21295=CARTESIAN_POINT('Ctrl Pts',(-8.22699388814824,1.01453885915658,7.96675283279074));
#21296=CARTESIAN_POINT('Ctrl Pts',(-8.49269364459153,1.01644874085988,7.97923376603893));
#21297=CARTESIAN_POINT('Ctrl Pts',(-8.75839340103483,1.01835862256319,7.99171469928712));
#21298=CARTESIAN_POINT('Ctrl Pts',(-9.02325176140381,0.911059288979017,
8.00419563253531));
#21299=CARTESIAN_POINT('Ctrl Pts',(-9.21270367535836,0.724758509267528,
8.0166765657835));
#21300=CARTESIAN_POINT('Ctrl Pts',(-9.4021555893129,0.538457729556039,8.02915749903169));
#21301=CARTESIAN_POINT('Ctrl Pts',(-9.5138818253584,0.275436159672388,8.04163843227988));
#21302=CARTESIAN_POINT('Ctrl Pts',(-9.51642831724057,0.0097417419642965,
8.05411936552807));
#21303=CARTESIAN_POINT('Ctrl Pts',(-9.51645943884197,0.00649459406663744,
8.05427189954255));
#21304=CARTESIAN_POINT('Ctrl Pts',(-9.516475,0.00324729703366067,8.05442443355703));
#21305=CARTESIAN_POINT('Ctrl Pts',(-9.516475,2.27303762236341E-13,8.05457696757151));
#21306=CARTESIAN_POINT('Origin',(-8.5,0.,1.24542303242842));
#21307=CARTESIAN_POINT('',(-9.516475,1.27637126781534E-13,7.39542303242849));
#21308=CARTESIAN_POINT('',(-9.516475,1.54580940361101E-13,7.45457696757151));
#21309=CARTESIAN_POINT('',(-9.516475,1.78524650477582E-12,1.24542303242842));
#21310=CARTESIAN_POINT('Ctrl Pts',(-9.516475,1.56527083874804E-13,7.39542303242849));
#21311=CARTESIAN_POINT('Ctrl Pts',(-9.51647500000004,-0.265706620583803,
7.40790396567668));
#21312=CARTESIAN_POINT('Ctrl Pts',(-9.40727465387204,-0.529786878176982,
7.42038489892487));
#21313=CARTESIAN_POINT('Ctrl Pts',(-9.21961691907769,-0.717894780174741,
7.43286583217306));
#21314=CARTESIAN_POINT('Ctrl Pts',(-9.03195918428333,-0.9060026821725,7.44534676542125));
#21315=CARTESIAN_POINT('Ctrl Pts',(-8.76814132834373,-1.0158354501991,7.45782769866944));
#21316=CARTESIAN_POINT('Ctrl Pts',(-8.50243547044498,-1.0164720823066,7.47030863191763));
#21317=CARTESIAN_POINT('Ctrl Pts',(-8.23672961254624,-1.01710871441409,
7.48278956516582));
#21318=CARTESIAN_POINT('Ctrl Pts',(-7.97238846933331,-0.908541417082732,
7.49527049841401));
#21319=CARTESIAN_POINT('Ctrl Pts',(-7.78383148002337,-0.721334926798557,
7.5077514316622));
#21320=CARTESIAN_POINT('Ctrl Pts',(-7.59527449071343,-0.534128436514382,
7.52023236491039));
#21321=CARTESIAN_POINT('Ctrl Pts',(-7.48480993131703,-0.270574496755717,
7.53271329815858));
#21322=CARTESIAN_POINT('Ctrl Pts',(-7.48353667075686,-0.00487092690823892,
7.54519423140677));
#21323=CARTESIAN_POINT('Ctrl Pts',(-7.48226341019669,0.26083264293924,7.55767516465496));
#21324=CARTESIAN_POINT('Ctrl Pts',(-7.59019703546751,0.525433154240429,
7.57015609790315));
#21325=CARTESIAN_POINT('Ctrl Pts',(-7.77695120652517,0.714438148393266,
7.58263703115134));
#21326=CARTESIAN_POINT('Ctrl Pts',(-7.96370537758284,0.903443142546103,
7.59511796439953));
#21327=CARTESIAN_POINT('Ctrl Pts',(-8.22699388814826,1.01453885915658,7.60759889764772));
#21328=CARTESIAN_POINT('Ctrl Pts',(-8.49269364459155,1.01644874085988,7.62007983089591));
#21329=CARTESIAN_POINT('Ctrl Pts',(-8.75839340103485,1.01835862256319,7.6325607641441));
#21330=CARTESIAN_POINT('Ctrl Pts',(-9.02325176140383,0.911059288979007,
7.64504169739229));
#21331=CARTESIAN_POINT('Ctrl Pts',(-9.21270367535837,0.724758509267514,
7.65752263064048));
#21332=CARTESIAN_POINT('Ctrl Pts',(-9.40215558931291,0.538457729556021,
7.67000356388867));
#21333=CARTESIAN_POINT('Ctrl Pts',(-9.5138818253584,0.275436159672368,7.68248449713686));
#21334=CARTESIAN_POINT('Ctrl Pts',(-9.51642831724057,0.00974174196427653,
7.69496543038505));
#21335=CARTESIAN_POINT('Ctrl Pts',(-9.51645943884197,0.00649459406660784,
7.69511796439953));
#21336=CARTESIAN_POINT('Ctrl Pts',(-9.516475,0.00324729703362146,7.69527049841401));
#21337=CARTESIAN_POINT('Ctrl Pts',(-9.516475,1.78443516265789E-13,7.69542303242849));
#21338=CARTESIAN_POINT('Ctrl Pts',(-9.516475,1.54580940361101E-13,7.45457696757151));
#21339=CARTESIAN_POINT('Ctrl Pts',(-9.51647500000004,-0.265706620583805,
7.4670579008197));
#21340=CARTESIAN_POINT('Ctrl Pts',(-9.40727465387204,-0.529786878176983,
7.47953883406789));
#21341=CARTESIAN_POINT('Ctrl Pts',(-9.21961691907768,-0.717894780174742,
7.49201976731608));
#21342=CARTESIAN_POINT('Ctrl Pts',(-9.03195918428333,-0.906002682172501,
7.50450070056427));
#21343=CARTESIAN_POINT('Ctrl Pts',(-8.76814132834372,-1.0158354501991,7.51698163381246));
#21344=CARTESIAN_POINT('Ctrl Pts',(-8.50243547044498,-1.0164720823066,7.52946256706065));
#21345=CARTESIAN_POINT('Ctrl Pts',(-8.23672961254623,-1.01710871441409,
7.54194350030884));
#21346=CARTESIAN_POINT('Ctrl Pts',(-7.97238846933331,-0.908541417082731,
7.55442443355703));
#21347=CARTESIAN_POINT('Ctrl Pts',(-7.78383148002337,-0.721334926798555,
7.56690536680522));
#21348=CARTESIAN_POINT('Ctrl Pts',(-7.59527449071343,-0.53412843651438,
7.57938630005341));
#21349=CARTESIAN_POINT('Ctrl Pts',(-7.48480993131703,-0.270574496755715,
7.5918672333016));
#21350=CARTESIAN_POINT('Ctrl Pts',(-7.48353667075686,-0.00487092690823697,
7.60434816654979));
#21351=CARTESIAN_POINT('Ctrl Pts',(-7.48226341019669,0.260832642939241,
7.61682909979798));
#21352=CARTESIAN_POINT('Ctrl Pts',(-7.59019703546752,0.525433154240431,
7.62931003304617));
#21353=CARTESIAN_POINT('Ctrl Pts',(-7.77695120652518,0.714438148393268,
7.64179096629436));
#21354=CARTESIAN_POINT('Ctrl Pts',(-7.96370537758284,0.903443142546104,
7.65427189954255));
#21355=CARTESIAN_POINT('Ctrl Pts',(-8.22699388814826,1.01453885915658,7.66675283279074));
#21356=CARTESIAN_POINT('Ctrl Pts',(-8.49269364459156,1.01644874085988,7.67923376603893));
#21357=CARTESIAN_POINT('Ctrl Pts',(-8.75839340103485,1.01835862256319,7.69171469928712));
#21358=CARTESIAN_POINT('Ctrl Pts',(-9.02325176140384,0.911059288979006,
7.70419563253531));
#21359=CARTESIAN_POINT('Ctrl Pts',(-9.21270367535837,0.724758509267513,
7.7166765657835));
#21360=CARTESIAN_POINT('Ctrl Pts',(-9.40215558931291,0.538457729556019,
7.72915749903169));
#21361=CARTESIAN_POINT('Ctrl Pts',(-9.5138818253584,0.275436159672367,7.74163843227988));
#21362=CARTESIAN_POINT('Ctrl Pts',(-9.51642831724057,0.00974174196427458,
7.75411936552807));
#21363=CARTESIAN_POINT('Ctrl Pts',(-9.51645943884197,0.00649459406660589,
7.75427189954255));
#21364=CARTESIAN_POINT('Ctrl Pts',(-9.516475,0.00324729703361952,7.75442443355703));
#21365=CARTESIAN_POINT('Ctrl Pts',(-9.516475,1.76497372752086E-13,7.75457696757151));
#21366=CARTESIAN_POINT('Origin',(-8.5,0.,1.24542303242842));
#21367=CARTESIAN_POINT('',(-9.51687640138522,-8.48276715981014E-5,7.09542303242849));
#21368=CARTESIAN_POINT('',(-9.516475,1.61554465063385E-13,7.15457696757151));
#21369=CARTESIAN_POINT('',(-9.516475,1.78524650477582E-12,1.24542303242842));
#21370=CARTESIAN_POINT('Ctrl Pts',(-9.516475,1.34610651483819E-13,7.09542303242849));
#21371=CARTESIAN_POINT('Ctrl Pts',(-9.51647500000004,-0.265706620583844,
7.10790396567668));
#21372=CARTESIAN_POINT('Ctrl Pts',(-9.40727465387201,-0.529786878177039,
7.12038489892487));
#21373=CARTESIAN_POINT('Ctrl Pts',(-9.21961691907763,-0.717894780174797,
7.13286583217306));
#21374=CARTESIAN_POINT('Ctrl Pts',(-9.03195918428324,-0.906002682172555,
7.14534676542125));
#21375=CARTESIAN_POINT('Ctrl Pts',(-8.76814132834361,-1.01583545019914,
7.15782769866944));
#21376=CARTESIAN_POINT('Ctrl Pts',(-8.50243547044484,-1.0164720823066,7.17030863191764));
#21377=CARTESIAN_POINT('Ctrl Pts',(-8.23672961254608,-1.01710871441406,
7.18278956516583));
#21378=CARTESIAN_POINT('Ctrl Pts',(-7.97238846933315,-0.908541417082644,
7.19527049841402));
#21379=CARTESIAN_POINT('Ctrl Pts',(-7.78383148002323,-0.721334926798419,
7.20775143166221));
#21380=CARTESIAN_POINT('Ctrl Pts',(-7.59527449071331,-0.534128436514195,
7.2202323649104));
#21381=CARTESIAN_POINT('Ctrl Pts',(-7.48480993131696,-0.270574496755484,
7.23271329815859));
#21382=CARTESIAN_POINT('Ctrl Pts',(-7.48353667075686,-0.00487092690798588,
7.24519423140678));
#21383=CARTESIAN_POINT('Ctrl Pts',(-7.48226341019675,0.260832642939512,
7.25767516465497));
#21384=CARTESIAN_POINT('Ctrl Pts',(-7.59019703546766,0.525433154240694,
7.27015609790316));
#21385=CARTESIAN_POINT('Ctrl Pts',(-7.77695120652539,0.714438148393487,
7.28263703115135));
#21386=CARTESIAN_POINT('Ctrl Pts',(-7.96370537758312,0.903443142546281,
7.29511796439954));
#21387=CARTESIAN_POINT('Ctrl Pts',(-8.22699388814861,1.01453885915668,7.30759889764774));
#21388=CARTESIAN_POINT('Ctrl Pts',(-8.49269364459192,1.01644874085989,7.32007983089593));
#21389=CARTESIAN_POINT('Ctrl Pts',(-8.75839340103524,1.01835862256309,7.33256076414412));
#21390=CARTESIAN_POINT('Ctrl Pts',(-9.0232517614042,0.911059288978801,7.34504169739231));
#21391=CARTESIAN_POINT('Ctrl Pts',(-9.21270367535868,0.724758509267215,
7.3575226306405));
#21392=CARTESIAN_POINT('Ctrl Pts',(-9.40215558931315,0.538457729555629,
7.37000356388869));
#21393=CARTESIAN_POINT('Ctrl Pts',(-9.51388182535853,0.275436159671905,
7.38248449713688));
#21394=CARTESIAN_POINT('Ctrl Pts',(-9.51642831724058,0.00974174196379239,
7.39496543038507));
#21395=CARTESIAN_POINT('Ctrl Pts',(-9.51645943884197,0.00649459406627776,
7.39511796439954));
#21396=CARTESIAN_POINT('Ctrl Pts',(-9.516475,0.00324729703344547,7.39527049841402));
#21397=CARTESIAN_POINT('Ctrl Pts',(-9.516475,1.56527083874804E-13,7.39542303242849));
#21398=CARTESIAN_POINT('Ctrl Pts',(-9.516475,1.61554465063385E-13,7.15457696757151));
#21399=CARTESIAN_POINT('Ctrl Pts',(-9.51647500000004,-0.265706620583822,
7.1670579008197));
#21400=CARTESIAN_POINT('Ctrl Pts',(-9.40727465387202,-0.529786878177025,
7.17953883406789));
#21401=CARTESIAN_POINT('Ctrl Pts',(-9.21961691907764,-0.717894780174788,
7.19201976731609));
#21402=CARTESIAN_POINT('Ctrl Pts',(-9.03195918428325,-0.906002682172552,
7.20450070056428));
#21403=CARTESIAN_POINT('Ctrl Pts',(-8.76814132834361,-1.01583545019914,
7.21698163381247));
#21404=CARTESIAN_POINT('Ctrl Pts',(-8.50243547044484,-1.0164720823066,7.22946256706066));
#21405=CARTESIAN_POINT('Ctrl Pts',(-8.23672961254607,-1.01710871441406,
7.24194350030885));
#21406=CARTESIAN_POINT('Ctrl Pts',(-7.97238846933314,-0.908541417082639,
7.25442443355704));
#21407=CARTESIAN_POINT('Ctrl Pts',(-7.78383148002322,-0.721334926798408,
7.26690536680523));
#21408=CARTESIAN_POINT('Ctrl Pts',(-7.5952744907133,-0.534128436514177,
7.27938630005342));
#21409=CARTESIAN_POINT('Ctrl Pts',(-7.48480993131695,-0.270574496755458,
7.29186723330162));
#21410=CARTESIAN_POINT('Ctrl Pts',(-7.48353667075686,-0.00487092690795505,
7.30434816654981));
#21411=CARTESIAN_POINT('Ctrl Pts',(-7.48226341019676,0.260832642939548,
7.316829099798));
#21412=CARTESIAN_POINT('Ctrl Pts',(-7.59019703546768,0.525433154240731,
7.32931003304619));
#21413=CARTESIAN_POINT('Ctrl Pts',(-7.77695120652542,0.714438148393519,
7.34179096629438));
#21414=CARTESIAN_POINT('Ctrl Pts',(-7.96370537758317,0.903443142546308,
7.35427189954257));
#21415=CARTESIAN_POINT('Ctrl Pts',(-8.22699388814866,1.0145388591567,7.36675283279076));
#21416=CARTESIAN_POINT('Ctrl Pts',(-8.49269364459198,1.01644874085989,7.37923376603895));
#21417=CARTESIAN_POINT('Ctrl Pts',(-8.75839340103531,1.01835862256308,7.39171469928714));
#21418=CARTESIAN_POINT('Ctrl Pts',(-9.02325176140427,0.911059288978762,
7.40419563253534));
#21419=CARTESIAN_POINT('Ctrl Pts',(-9.21270367535874,0.724758509267153,
7.41667656578353));
#21420=CARTESIAN_POINT('Ctrl Pts',(-9.4021555893132,0.538457729555544,7.42915749903172));
#21421=CARTESIAN_POINT('Ctrl Pts',(-9.51388182535857,0.275436159671797,
7.44163843227991));
#21422=CARTESIAN_POINT('Ctrl Pts',(-9.51642831724058,0.0097417419636749,
7.4541193655281));
#21423=CARTESIAN_POINT('Ctrl Pts',(-9.51645943884197,0.00649459406619878,
7.45427189954257));
#21424=CARTESIAN_POINT('Ctrl Pts',(-9.516475,0.00324729703340501,7.45442443355704));
#21425=CARTESIAN_POINT('Ctrl Pts',(-9.516475,1.54580940361101E-13,7.45457696757151));
#21426=CARTESIAN_POINT('Origin',(-8.5,0.,1.24542303242842));
#21427=CARTESIAN_POINT('',(-9.51556541541323,-0.000810312451272878,6.79542303242848));
#21428=CARTESIAN_POINT('',(-9.516475,1.6852798976567E-13,6.85457696757151));
#21429=CARTESIAN_POINT('',(-9.516475,1.78524650477582E-12,1.24542303242842));
#21430=CARTESIAN_POINT('Ctrl Pts',(-9.51556541541323,-0.000810312451272902,
6.79542303242848));
#21431=CARTESIAN_POINT('Ctrl Pts',(-9.51634597973439,-0.110204889627698,
6.80055284253917));
#21432=CARTESIAN_POINT('Ctrl Pts',(-9.44942527604987,-0.557857220545352,
6.82158999380147));
#21433=CARTESIAN_POINT('Ctrl Pts',(-8.7968570426639,-1.16531969262148,6.85853448621541));
#21434=CARTESIAN_POINT('Ctrl Pts',(-7.67912294882438,-0.878910898486879,
6.90625650967025));
#21435=CARTESIAN_POINT('Ctrl Pts',(-7.37898454940943,0.0315485133979244,
6.94602486254932));
#21436=CARTESIAN_POINT('Ctrl Pts',(-7.67763196849479,0.663562963521021,
6.97783954485255));
#21437=CARTESIAN_POINT('Ctrl Pts',(-8.23225858352771,1.08902960614752,7.0096542271558));
#21438=CARTESIAN_POINT('Ctrl Pts',(-9.17182695227493,0.989535098804095,
7.04884872301444));
#21439=CARTESIAN_POINT('Ctrl Pts',(-9.51713519569878,0.324724529807011,
7.08008954829728));
#21440=CARTESIAN_POINT('Ctrl Pts',(-9.51817020583245,-0.000358245808598775,
7.09542303242849));
#21441=CARTESIAN_POINT('Ctrl Pts',(-9.516475,1.6852798976567E-13,6.85457696757151));
#21442=CARTESIAN_POINT('Ctrl Pts',(-9.51647500000004,-0.26570662058381,
6.8670579008197));
#21443=CARTESIAN_POINT('Ctrl Pts',(-9.40727465387203,-0.529786878177009,
6.87953883406789));
#21444=CARTESIAN_POINT('Ctrl Pts',(-9.21961691907765,-0.717894780174773,
6.89201976731608));
#21445=CARTESIAN_POINT('Ctrl Pts',(-9.03195918428327,-0.906002682172537,
6.90450070056428));
#21446=CARTESIAN_POINT('Ctrl Pts',(-8.76814132834364,-1.01583545019913,
6.91698163381247));
#21447=CARTESIAN_POINT('Ctrl Pts',(-8.50243547044488,-1.0164720823066,6.92946256706066));
#21448=CARTESIAN_POINT('Ctrl Pts',(-8.23672961254611,-1.01710871441407,
6.94194350030885));
#21449=CARTESIAN_POINT('Ctrl Pts',(-7.97238846933318,-0.908541417082661,
6.95442443355704));
#21450=CARTESIAN_POINT('Ctrl Pts',(-7.78383148002325,-0.721334926798443,
6.96690536680523));
#21451=CARTESIAN_POINT('Ctrl Pts',(-7.59527449071333,-0.534128436514225,
6.97938630005342));
#21452=CARTESIAN_POINT('Ctrl Pts',(-7.48480993131697,-0.270574496755518,
6.99186723330161));
#21453=CARTESIAN_POINT('Ctrl Pts',(-7.48353667075686,-0.0048709269080198,
7.0043481665498));
#21454=CARTESIAN_POINT('Ctrl Pts',(-7.48226341019674,0.260832642939478,
7.01682909979799));
#21455=CARTESIAN_POINT('Ctrl Pts',(-7.59019703546764,0.525433154240663,
7.02931003304619));
#21456=CARTESIAN_POINT('Ctrl Pts',(-7.77695120652537,0.714438148393463,
7.04179096629438));
#21457=CARTESIAN_POINT('Ctrl Pts',(-7.96370537758309,0.903443142546263,
7.05427189954257));
#21458=CARTESIAN_POINT('Ctrl Pts',(-8.22699388814857,1.01453885915667,7.06675283279076));
#21459=CARTESIAN_POINT('Ctrl Pts',(-8.49269364459189,1.01644874085989,7.07923376603895));
#21460=CARTESIAN_POINT('Ctrl Pts',(-8.7583934010352,1.0183586225631,7.09171469928714));
#21461=CARTESIAN_POINT('Ctrl Pts',(-9.02325176140417,0.911059288978819,
7.10419563253533));
#21462=CARTESIAN_POINT('Ctrl Pts',(-9.21270367535865,0.724758509267239,
7.11667656578352));
#21463=CARTESIAN_POINT('Ctrl Pts',(-9.40215558931313,0.538457729555659,
7.12915749903171));
#21464=CARTESIAN_POINT('Ctrl Pts',(-9.51388182535852,0.275436159671939,
7.1416384322799));
#21465=CARTESIAN_POINT('Ctrl Pts',(-9.51642831724058,0.00974174196382631,
7.15411936552809));
#21466=CARTESIAN_POINT('Ctrl Pts',(-9.51645943884197,0.00649459406630205,
7.15427189954257));
#21467=CARTESIAN_POINT('Ctrl Pts',(-9.516475,0.00324729703346011,7.15442443355704));
#21468=CARTESIAN_POINT('Ctrl Pts',(-9.516475,1.61554465063385E-13,7.15457696757151));
#21469=CARTESIAN_POINT('Origin',(-8.5,0.,1.24542303242842));
#21470=CARTESIAN_POINT('',(-9.51625672877642,9.02772980376447E-5,6.49542303242849));
#21471=CARTESIAN_POINT('',(-9.516475,1.75501514467955E-13,6.55457696757151));
#21472=CARTESIAN_POINT('',(-9.516475,1.78524650477582E-12,1.24542303242842));
#21473=CARTESIAN_POINT('Ctrl Pts',(-9.51510181470517,0.000567951450037713,
6.49542303242849));
#21474=CARTESIAN_POINT('Ctrl Pts',(-9.51414510430117,-0.206228520727224,
6.50510879562945));
#21475=CARTESIAN_POINT('Ctrl Pts',(-9.35231132463273,-0.754153240087441,
6.53070189998202));
#21476=CARTESIAN_POINT('Ctrl Pts',(-8.45426188445871,-1.20176184221855,
6.57220234548622));
#21477=CARTESIAN_POINT('Ctrl Pts',(-7.63158681559905,-0.709598118880692,
6.61197069836528));
#21478=CARTESIAN_POINT('Ctrl Pts',(-7.44392618126472,-0.0362363792399661,
6.64378538066852));
#21479=CARTESIAN_POINT('Ctrl Pts',(-7.58499054185306,0.648404688957481,
6.67560006297176));
#21480=CARTESIAN_POINT('Ctrl Pts',(-8.37199588104198,1.19580033707788,6.71536841585081));
#21481=CARTESIAN_POINT('Ctrl Pts',(-9.32299097508662,0.800672039024471,
6.75796062919499));
#21482=CARTESIAN_POINT('Ctrl Pts',(-9.5139254802072,0.229023429108448,6.78464550138755));
#21483=CARTESIAN_POINT('Ctrl Pts',(-9.51556541541323,-0.000810312451272902,
6.79542303242848));
#21484=CARTESIAN_POINT('Ctrl Pts',(-9.516475,1.75501514467955E-13,6.55457696757151));
#21485=CARTESIAN_POINT('Ctrl Pts',(-9.51647500000005,-0.265706620583793,
6.5670579008197));
#21486=CARTESIAN_POINT('Ctrl Pts',(-9.40727465387204,-0.529786878176984,
6.57953883406789));
#21487=CARTESIAN_POINT('Ctrl Pts',(-9.21961691907768,-0.717894780174748,
6.59201976731608));
#21488=CARTESIAN_POINT('Ctrl Pts',(-9.03195918428331,-0.906002682172512,
6.60450070056427));
#21489=CARTESIAN_POINT('Ctrl Pts',(-8.7681413283437,-1.01583545019911,6.61698163381246));
#21490=CARTESIAN_POINT('Ctrl Pts',(-8.50243547044494,-1.0164720823066,6.62946256706065));
#21491=CARTESIAN_POINT('Ctrl Pts',(-8.23672961254619,-1.01710871441409,
6.64194350030885));
#21492=CARTESIAN_POINT('Ctrl Pts',(-7.97238846933326,-0.908541417082703,
6.65442443355704));
#21493=CARTESIAN_POINT('Ctrl Pts',(-7.78383148002332,-0.721334926798509,
6.66690536680523));
#21494=CARTESIAN_POINT('Ctrl Pts',(-7.59527449071338,-0.534128436514315,
6.67938630005342));
#21495=CARTESIAN_POINT('Ctrl Pts',(-7.484809931317,-0.270574496755631,6.69186723330161));
#21496=CARTESIAN_POINT('Ctrl Pts',(-7.48353667075686,-0.00487092690814233,
6.7043481665498));
#21497=CARTESIAN_POINT('Ctrl Pts',(-7.48226341019671,0.260832642939346,
6.71682909979799));
#21498=CARTESIAN_POINT('Ctrl Pts',(-7.59019703546757,0.525433154240535,
6.72931003304618));
#21499=CARTESIAN_POINT('Ctrl Pts',(-7.77695120652526,0.714438148393355,
6.74179096629437));
#21500=CARTESIAN_POINT('Ctrl Pts',(-7.96370537758295,0.903443142546176,
6.75427189954256));
#21501=CARTESIAN_POINT('Ctrl Pts',(-8.2269938881484,1.01453885915662,6.76675283279075));
#21502=CARTESIAN_POINT('Ctrl Pts',(-8.49269364459171,1.01644874085989,6.77923376603894));
#21503=CARTESIAN_POINT('Ctrl Pts',(-8.75839340103502,1.01835862256315,6.79171469928713));
#21504=CARTESIAN_POINT('Ctrl Pts',(-9.02325176140399,0.91105928897892,6.80419563253532));
#21505=CARTESIAN_POINT('Ctrl Pts',(-9.2127036753585,0.724758509267386,6.81667656578351));
#21506=CARTESIAN_POINT('Ctrl Pts',(-9.40215558931301,0.538457729555852,
6.8291574990317));
#21507=CARTESIAN_POINT('Ctrl Pts',(-9.51388182535846,0.275436159672167,
6.84163843227989));
#21508=CARTESIAN_POINT('Ctrl Pts',(-9.51642831724057,0.00974174196406439,
6.85411936552808));
#21509=CARTESIAN_POINT('Ctrl Pts',(-9.51645943884197,0.0064945940664631,
6.85427189954256));
#21510=CARTESIAN_POINT('Ctrl Pts',(-9.516475,0.00324729703354412,6.85442443355704));
#21511=CARTESIAN_POINT('Ctrl Pts',(-9.516475,1.6852798976567E-13,6.85457696757151));
#21512=CARTESIAN_POINT('Origin',(-8.5,0.,1.24542303242842));
#21513=CARTESIAN_POINT('',(-9.516475,1.55531225590673E-13,6.19542303242849));
#21514=CARTESIAN_POINT('',(-9.516475,1.8247503917024E-13,6.25457696757151));
#21515=CARTESIAN_POINT('',(-9.516475,1.78524650477582E-12,1.24542303242842));
#21516=CARTESIAN_POINT('Ctrl Pts',(-9.516475,1.55531225590673E-13,6.19542303242849));
#21517=CARTESIAN_POINT('Ctrl Pts',(-9.51647500000004,-0.265706620583813,
6.20790396567668));
#21518=CARTESIAN_POINT('Ctrl Pts',(-9.40727465387203,-0.529786878177001,
6.22038489892487));
#21519=CARTESIAN_POINT('Ctrl Pts',(-9.21961691907766,-0.717894780174762,
6.23286583217306));
#21520=CARTESIAN_POINT('Ctrl Pts',(-9.03195918428329,-0.906002682172522,
6.24534676542125));
#21521=CARTESIAN_POINT('Ctrl Pts',(-8.76814132834368,-1.01583545019912,
6.25782769866944));
#21522=CARTESIAN_POINT('Ctrl Pts',(-8.50243547044492,-1.0164720823066,6.27030863191763));
#21523=CARTESIAN_POINT('Ctrl Pts',(-8.23672961254617,-1.01710871441408,
6.28278956516582));
#21524=CARTESIAN_POINT('Ctrl Pts',(-7.97238846933324,-0.908541417082693,
6.29527049841401));
#21525=CARTESIAN_POINT('Ctrl Pts',(-7.78383148002331,-0.721334926798495,
6.3077514316622));
#21526=CARTESIAN_POINT('Ctrl Pts',(-7.59527449071337,-0.534128436514297,
6.32023236491039));
#21527=CARTESIAN_POINT('Ctrl Pts',(-7.484809931317,-0.270574496755611,6.33271329815858));
#21528=CARTESIAN_POINT('Ctrl Pts',(-7.48353667075686,-0.00487092690812236,
6.34519423140677));
#21529=CARTESIAN_POINT('Ctrl Pts',(-7.48226341019672,0.260832642939366,
6.35767516465496));
#21530=CARTESIAN_POINT('Ctrl Pts',(-7.59019703546758,0.525433154240553,
6.37015609790315));
#21531=CARTESIAN_POINT('Ctrl Pts',(-7.77695120652528,0.71443814839337,6.38263703115135));
#21532=CARTESIAN_POINT('Ctrl Pts',(-7.96370537758297,0.903443142546187,
6.39511796439954));
#21533=CARTESIAN_POINT('Ctrl Pts',(-8.22699388814842,1.01453885915663,6.40759889764773));
#21534=CARTESIAN_POINT('Ctrl Pts',(-8.49269364459173,1.01644874085989,6.42007983089592));
#21535=CARTESIAN_POINT('Ctrl Pts',(-8.75839340103504,1.01835862256314,6.43256076414411));
#21536=CARTESIAN_POINT('Ctrl Pts',(-9.02325176140401,0.911059288978909,
6.4450416973923));
#21537=CARTESIAN_POINT('Ctrl Pts',(-9.21270367535852,0.724758509267372,
6.45752263064049));
#21538=CARTESIAN_POINT('Ctrl Pts',(-9.40215558931302,0.538457729555834,
6.47000356388868));
#21539=CARTESIAN_POINT('Ctrl Pts',(-9.51388182535847,0.275436159672147,
6.48248449713687));
#21540=CARTESIAN_POINT('Ctrl Pts',(-9.51642831724057,0.00974174196404442,
6.49496543038506));
#21541=CARTESIAN_POINT('Ctrl Pts',(-9.51645943884197,0.00649459406644795,
6.49511796439954));
#21542=CARTESIAN_POINT('Ctrl Pts',(-9.516475,0.00324729703353379,6.49527049841401));
#21543=CARTESIAN_POINT('Ctrl Pts',(-9.516475,1.63002679435024E-13,6.49542303242849));
#21544=CARTESIAN_POINT('Ctrl Pts',(-9.516475,1.8247503917024E-13,6.25457696757151));
#21545=CARTESIAN_POINT('Ctrl Pts',(-9.51647500000005,-0.265706620583796,
6.2670579008197));
#21546=CARTESIAN_POINT('Ctrl Pts',(-9.40727465387204,-0.529786878176997,
6.27953883406789));
#21547=CARTESIAN_POINT('Ctrl Pts',(-9.21961691907766,-0.717894780174763,
6.29201976731608));
#21548=CARTESIAN_POINT('Ctrl Pts',(-9.03195918428329,-0.90600268217253,
6.30450070056427));
#21549=CARTESIAN_POINT('Ctrl Pts',(-8.76814132834365,-1.01583545019912,
6.31698163381247));
#21550=CARTESIAN_POINT('Ctrl Pts',(-8.50243547044489,-1.0164720823066,6.32946256706066));
#21551=CARTESIAN_POINT('Ctrl Pts',(-8.23672961254613,-1.01710871441407,
6.34194350030885));
#21552=CARTESIAN_POINT('Ctrl Pts',(-7.97238846933319,-0.908541417082669,
6.35442443355704));
#21553=CARTESIAN_POINT('Ctrl Pts',(-7.78383148002326,-0.721334926798453,
6.36690536680523));
#21554=CARTESIAN_POINT('Ctrl Pts',(-7.59527449071334,-0.534128436514237,
6.37938630005342));
#21555=CARTESIAN_POINT('Ctrl Pts',(-7.48480993131697,-0.270574496755532,
6.39186723330161));
#21556=CARTESIAN_POINT('Ctrl Pts',(-7.48353667075686,-0.00487092690803375,
6.4043481665498));
#21557=CARTESIAN_POINT('Ctrl Pts',(-7.48226341019674,0.260832642939464,
6.41682909979799));
#21558=CARTESIAN_POINT('Ctrl Pts',(-7.59019703546764,0.525433154240651,
6.42931003304618));
#21559=CARTESIAN_POINT('Ctrl Pts',(-7.77695120652536,0.714438148393453,
6.44179096629438));
#21560=CARTESIAN_POINT('Ctrl Pts',(-7.96370537758308,0.903443142546255,
6.45427189954257));
#21561=CARTESIAN_POINT('Ctrl Pts',(-8.22699388814856,1.01453885915667,6.46675283279076));
#21562=CARTESIAN_POINT('Ctrl Pts',(-8.49269364459187,1.01644874085989,6.47923376603895));
#21563=CARTESIAN_POINT('Ctrl Pts',(-8.75839340103519,1.0183586225631,6.49171469928714));
#21564=CARTESIAN_POINT('Ctrl Pts',(-9.02325176140416,0.911059288978826,
6.50419563253533));
#21565=CARTESIAN_POINT('Ctrl Pts',(-9.21270367535864,0.724758509267249,
6.51667656578352));
#21566=CARTESIAN_POINT('Ctrl Pts',(-9.40215558931312,0.538457729555672,
6.52915749903171));
#21567=CARTESIAN_POINT('Ctrl Pts',(-9.51388182535852,0.275436159671953,
6.5416384322799));
#21568=CARTESIAN_POINT('Ctrl Pts',(-9.51642831724058,0.00974174196384026,
6.55411936552809));
#21569=CARTESIAN_POINT('Ctrl Pts',(-9.51645943884197,0.006494594066316,
6.55427189954257));
#21570=CARTESIAN_POINT('Ctrl Pts',(-9.516475,0.00324729703347406,6.55442443355704));
#21571=CARTESIAN_POINT('Ctrl Pts',(-9.516475,1.75501514467955E-13,6.55457696757151));
#21572=CARTESIAN_POINT('Origin',(-8.5,0.,1.24542303242842));
#21573=CARTESIAN_POINT('',(-9.516475,1.62504750292958E-13,5.89542303242849));
#21574=CARTESIAN_POINT('',(-9.516475,1.89448563872525E-13,5.95457696757151));
#21575=CARTESIAN_POINT('',(-9.516475,1.78524650477582E-12,1.24542303242842));
#21576=CARTESIAN_POINT('Ctrl Pts',(-9.516475,1.62504750292958E-13,5.89542303242849));
#21577=CARTESIAN_POINT('Ctrl Pts',(-9.51647500000004,-0.265706620583806,
5.90790396567668));
#21578=CARTESIAN_POINT('Ctrl Pts',(-9.40727465387204,-0.529786878176995,
5.92038489892487));
#21579=CARTESIAN_POINT('Ctrl Pts',(-9.21961691907767,-0.717894780174757,
5.93286583217306));
#21580=CARTESIAN_POINT('Ctrl Pts',(-9.0319591842833,-0.906002682172519,
5.94534676542125));
#21581=CARTESIAN_POINT('Ctrl Pts',(-8.76814132834368,-1.01583545019911,
5.95782769866944));
#21582=CARTESIAN_POINT('Ctrl Pts',(-8.50243547044493,-1.0164720823066,5.97030863191763));
#21583=CARTESIAN_POINT('Ctrl Pts',(-8.23672961254618,-1.01710871441408,
5.98278956516582));
#21584=CARTESIAN_POINT('Ctrl Pts',(-7.97238846933324,-0.908541417082697,
5.99527049841401));
#21585=CARTESIAN_POINT('Ctrl Pts',(-7.78383148002331,-0.7213349267985,6.0077514316622));
#21586=CARTESIAN_POINT('Ctrl Pts',(-7.59527449071338,-0.534128436514303,
6.02023236491039));
#21587=CARTESIAN_POINT('Ctrl Pts',(-7.484809931317,-0.270574496755618,6.03271329815858));
#21588=CARTESIAN_POINT('Ctrl Pts',(-7.48353667075686,-0.00487092690812934,
6.04519423140677));
#21589=CARTESIAN_POINT('Ctrl Pts',(-7.48226341019671,0.260832642939359,
6.05767516465496));
#21590=CARTESIAN_POINT('Ctrl Pts',(-7.59019703546758,0.525433154240546,
6.07015609790315));
#21591=CARTESIAN_POINT('Ctrl Pts',(-7.77695120652527,0.714438148393365,
6.08263703115134));
#21592=CARTESIAN_POINT('Ctrl Pts',(-7.96370537758296,0.903443142546183,
6.09511796439954));
#21593=CARTESIAN_POINT('Ctrl Pts',(-8.22699388814841,1.01453885915663,6.10759889764773));
#21594=CARTESIAN_POINT('Ctrl Pts',(-8.49269364459172,1.01644874085989,6.12007983089592));
#21595=CARTESIAN_POINT('Ctrl Pts',(-8.75839340103503,1.01835862256314,6.13256076414411));
#21596=CARTESIAN_POINT('Ctrl Pts',(-9.023251761404,0.911059288978913,6.1450416973923));
#21597=CARTESIAN_POINT('Ctrl Pts',(-9.21270367535851,0.724758509267377,
6.15752263064049));
#21598=CARTESIAN_POINT('Ctrl Pts',(-9.40215558931302,0.53845772955584,6.17000356388868));
#21599=CARTESIAN_POINT('Ctrl Pts',(-9.51388182535846,0.275436159672154,
6.18248449713687));
#21600=CARTESIAN_POINT('Ctrl Pts',(-9.51642831724057,0.0097417419640514,
6.19496543038506));
#21601=CARTESIAN_POINT('Ctrl Pts',(-9.51645943884197,0.00649459406645011,
6.19511796439954));
#21602=CARTESIAN_POINT('Ctrl Pts',(-9.516475,0.00324729703353112,6.19527049841401));
#21603=CARTESIAN_POINT('Ctrl Pts',(-9.516475,1.55531225590673E-13,6.19542303242849));
#21604=CARTESIAN_POINT('Ctrl Pts',(-9.516475,2.0389354241916E-13,5.95457696757151));
#21605=CARTESIAN_POINT('Ctrl Pts',(-9.51647500000005,-0.265706620583774,
5.9670579008197));
#21606=CARTESIAN_POINT('Ctrl Pts',(-9.40727465387205,-0.529786878176977,
5.97953883406789));
#21607=CARTESIAN_POINT('Ctrl Pts',(-9.21961691907768,-0.717894780174748,
5.99201976731608));
#21608=CARTESIAN_POINT('Ctrl Pts',(-9.03195918428331,-0.906002682172519,
6.00450070056427));
#21609=CARTESIAN_POINT('Ctrl Pts',(-8.76814132834368,-1.01583545019912,
6.01698163381247));
#21610=CARTESIAN_POINT('Ctrl Pts',(-8.50243547044491,-1.0164720823066,6.02946256706066));
#21611=CARTESIAN_POINT('Ctrl Pts',(-8.23672961254615,-1.01710871441408,
6.04194350030885));
#21612=CARTESIAN_POINT('Ctrl Pts',(-7.97238846933321,-0.90854141708268,
6.05442443355704));
#21613=CARTESIAN_POINT('Ctrl Pts',(-7.78383148002328,-0.721334926798468,
6.06690536680523));
#21614=CARTESIAN_POINT('Ctrl Pts',(-7.59527449071335,-0.534128436514256,
6.07938630005342));
#21615=CARTESIAN_POINT('Ctrl Pts',(-7.48480993131698,-0.270574496755553,
6.09186723330161));
#21616=CARTESIAN_POINT('Ctrl Pts',(-7.48353667075686,-0.00487092690805517,
6.1043481665498));
#21617=CARTESIAN_POINT('Ctrl Pts',(-7.48226341019673,0.260832642939443,
6.11682909979799));
#21618=CARTESIAN_POINT('Ctrl Pts',(-7.59019703546762,0.525433154240632,
6.12931003304618));
#21619=CARTESIAN_POINT('Ctrl Pts',(-7.77695120652534,0.714438148393438,
6.14179096629437));
#21620=CARTESIAN_POINT('Ctrl Pts',(-7.96370537758306,0.903443142546244,
6.15427189954256));
#21621=CARTESIAN_POINT('Ctrl Pts',(-8.22699388814854,1.01453885915666,6.16675283279076));
#21622=CARTESIAN_POINT('Ctrl Pts',(-8.49269364459185,1.01644874085989,6.17923376603895));
#21623=CARTESIAN_POINT('Ctrl Pts',(-8.75839340103517,1.01835862256311,6.19171469928714));
#21624=CARTESIAN_POINT('Ctrl Pts',(-9.02325176140414,0.911059288978837,
6.20419563253533));
#21625=CARTESIAN_POINT('Ctrl Pts',(-9.21270367535863,0.724758509267264,
6.21667656578352));
#21626=CARTESIAN_POINT('Ctrl Pts',(-9.40215558931311,0.53845772955569,6.22915749903171));
#21627=CARTESIAN_POINT('Ctrl Pts',(-9.51388182535852,0.275436159671974,
6.2416384322799));
#21628=CARTESIAN_POINT('Ctrl Pts',(-9.51642831724058,0.00974174196386167,
6.25411936552809));
#21629=CARTESIAN_POINT('Ctrl Pts',(-9.51645943884197,0.0064945940663326,
6.25427189954257));
#21630=CARTESIAN_POINT('Ctrl Pts',(-9.516475,0.00324729703348583,6.25442443355704));
#21631=CARTESIAN_POINT('Ctrl Pts',(-9.516475,1.8247503917024E-13,6.25457696757151));
#21632=CARTESIAN_POINT('Origin',(-8.5,0.,1.24542303242842));
#21633=CARTESIAN_POINT('',(-9.516475,1.69478274995243E-13,5.59542303242849));
#21634=CARTESIAN_POINT('',(-9.516475,1.9642208857481E-13,5.65457696757151));
#21635=CARTESIAN_POINT('',(-9.516475,1.78524650477582E-12,1.24542303242842));
#21636=CARTESIAN_POINT('Ctrl Pts',(-9.516475,1.83923253541878E-13,5.59542303242849));
#21637=CARTESIAN_POINT('Ctrl Pts',(-9.51647500000005,-0.26570662058379,
5.60790396567668));
#21638=CARTESIAN_POINT('Ctrl Pts',(-9.40727465387205,-0.529786878176986,
5.62038489892487));
#21639=CARTESIAN_POINT('Ctrl Pts',(-9.21961691907767,-0.717894780174752,
5.63286583217306));
#21640=CARTESIAN_POINT('Ctrl Pts',(-9.0319591842833,-0.906002682172518,
5.64534676542125));
#21641=CARTESIAN_POINT('Ctrl Pts',(-8.76814132834368,-1.01583545019912,
5.65782769866944));
#21642=CARTESIAN_POINT('Ctrl Pts',(-8.50243547044492,-1.0164720823066,5.67030863191763));
#21643=CARTESIAN_POINT('Ctrl Pts',(-8.23672961254616,-1.01710871441408,
5.68278956516582));
#21644=CARTESIAN_POINT('Ctrl Pts',(-7.97238846933323,-0.908541417082689,
5.69527049841401));
#21645=CARTESIAN_POINT('Ctrl Pts',(-7.7838314800233,-0.721334926798484,
5.7077514316622));
#21646=CARTESIAN_POINT('Ctrl Pts',(-7.59527449071336,-0.53412843651428,
5.72023236491039));
#21647=CARTESIAN_POINT('Ctrl Pts',(-7.48480993131699,-0.270574496755586,
5.73271329815858));
#21648=CARTESIAN_POINT('Ctrl Pts',(-7.48353667075686,-0.00487092690809298,
5.74519423140678));
#21649=CARTESIAN_POINT('Ctrl Pts',(-7.48226341019672,0.2608326429394,5.75767516465497));
#21650=CARTESIAN_POINT('Ctrl Pts',(-7.5901970354676,0.525433154240588,5.77015609790316));
#21651=CARTESIAN_POINT('Ctrl Pts',(-7.77695120652531,0.714438148393401,
5.78263703115135));
#21652=CARTESIAN_POINT('Ctrl Pts',(-7.96370537758301,0.903443142546213,
5.79511796439954));
#21653=CARTESIAN_POINT('Ctrl Pts',(-8.22699388814848,1.01453885915665,5.80759889764773));
#21654=CARTESIAN_POINT('Ctrl Pts',(-8.49269364459179,1.01644874085989,5.82007983089592));
#21655=CARTESIAN_POINT('Ctrl Pts',(-8.7583934010351,1.01835862256313,5.83256076414411));
#21656=CARTESIAN_POINT('Ctrl Pts',(-9.02325176140407,0.911059288978875,
5.8450416973923));
#21657=CARTESIAN_POINT('Ctrl Pts',(-9.21270367535857,0.724758509267321,
5.85752263064049));
#21658=CARTESIAN_POINT('Ctrl Pts',(-9.40215558931307,0.538457729555766,
5.87000356388868));
#21659=CARTESIAN_POINT('Ctrl Pts',(-9.51388182535849,0.275436159672064,
5.88248449713687));
#21660=CARTESIAN_POINT('Ctrl Pts',(-9.51642831724057,0.00974174196395726,
5.89496543038506));
#21661=CARTESIAN_POINT('Ctrl Pts',(-9.51645943884197,0.00649459406638967,
5.89511796439954));
#21662=CARTESIAN_POINT('Ctrl Pts',(-9.516475,0.00324729703350438,5.89527049841401));
#21663=CARTESIAN_POINT('Ctrl Pts',(-9.516475,1.62504750292958E-13,5.89542303242849));
#21664=CARTESIAN_POINT('Ctrl Pts',(-9.516475,1.9642208857481E-13,5.65457696757151));
#21665=CARTESIAN_POINT('Ctrl Pts',(-9.51647500000005,-0.265706620583782,
5.6670579008197));
#21666=CARTESIAN_POINT('Ctrl Pts',(-9.40727465387205,-0.529786878176984,
5.67953883406789));
#21667=CARTESIAN_POINT('Ctrl Pts',(-9.21961691907767,-0.717894780174753,
5.69201976731608));
#21668=CARTESIAN_POINT('Ctrl Pts',(-9.0319591842833,-0.906002682172523,
5.70450070056427));
#21669=CARTESIAN_POINT('Ctrl Pts',(-8.76814132834367,-1.01583545019912,
5.71698163381247));
#21670=CARTESIAN_POINT('Ctrl Pts',(-8.5024354704449,-1.0164720823066,5.72946256706066));
#21671=CARTESIAN_POINT('Ctrl Pts',(-8.23672961254614,-1.01710871441408,
5.74194350030885));
#21672=CARTESIAN_POINT('Ctrl Pts',(-7.9723884693332,-0.908541417082676,
5.75442443355704));
#21673=CARTESIAN_POINT('Ctrl Pts',(-7.78383148002327,-0.721334926798463,
5.76690536680523));
#21674=CARTESIAN_POINT('Ctrl Pts',(-7.59527449071334,-0.53412843651425,
5.77938630005342));
#21675=CARTESIAN_POINT('Ctrl Pts',(-7.48480993131698,-0.270574496755546,
5.79186723330161));
#21676=CARTESIAN_POINT('Ctrl Pts',(-7.48353667075686,-0.0048709269080477,
5.8043481665498));
#21677=CARTESIAN_POINT('Ctrl Pts',(-7.48226341019673,0.26083264293945,5.81682909979799));
#21678=CARTESIAN_POINT('Ctrl Pts',(-7.59019703546763,0.525433154240638,
5.82931003304618));
#21679=CARTESIAN_POINT('Ctrl Pts',(-7.77695120652535,0.714438148393443,
5.84179096629437));
#21680=CARTESIAN_POINT('Ctrl Pts',(-7.96370537758307,0.903443142546248,
5.85427189954256));
#21681=CARTESIAN_POINT('Ctrl Pts',(-8.22699388814855,1.01453885915667,5.86675283279076));
#21682=CARTESIAN_POINT('Ctrl Pts',(-8.49269364459186,1.01644874085989,5.87923376603895));
#21683=CARTESIAN_POINT('Ctrl Pts',(-8.75839340103518,1.01835862256311,5.89171469928714));
#21684=CARTESIAN_POINT('Ctrl Pts',(-9.02325176140415,0.911059288978833,
5.90419563253533));
#21685=CARTESIAN_POINT('Ctrl Pts',(-9.21270367535863,0.724758509267258,
5.91667656578352));
#21686=CARTESIAN_POINT('Ctrl Pts',(-9.40215558931312,0.538457729555684,
5.92915749903171));
#21687=CARTESIAN_POINT('Ctrl Pts',(-9.51388182535852,0.275436159671966,
5.9416384322799));
#21688=CARTESIAN_POINT('Ctrl Pts',(-9.51642831724058,0.0097417419638542,
5.95411936552809));
#21689=CARTESIAN_POINT('Ctrl Pts',(-9.51645943884197,0.00649459406633476,
5.95427189954257));
#21690=CARTESIAN_POINT('Ctrl Pts',(-9.516475,0.00324729703349764,5.95442443355704));
#21691=CARTESIAN_POINT('Ctrl Pts',(-9.516475,2.0389354241916E-13,5.95457696757151));
#21692=CARTESIAN_POINT('Origin',(-8.5,0.,1.24542303242842));
#21693=CARTESIAN_POINT('',(-9.516475,1.76451799697528E-13,5.29542303242849));
#21694=CARTESIAN_POINT('',(-9.51597631883388,-0.000112310372824663,5.35457696757151));
#21695=CARTESIAN_POINT('',(-9.516475,1.78524650477582E-12,1.24542303242842));
#21696=CARTESIAN_POINT('Ctrl Pts',(-9.516475,1.76451799697528E-13,5.29542303242849));
#21697=CARTESIAN_POINT('Ctrl Pts',(-9.51647500000005,-0.265706620583792,
5.30790396567668));
#21698=CARTESIAN_POINT('Ctrl Pts',(-9.40727465387205,-0.529786878176983,
5.32038489892487));
#21699=CARTESIAN_POINT('Ctrl Pts',(-9.21961691907768,-0.717894780174747,
5.33286583217306));
#21700=CARTESIAN_POINT('Ctrl Pts',(-9.03195918428331,-0.906002682172511,
5.34534676542125));
#21701=CARTESIAN_POINT('Ctrl Pts',(-8.7681413283437,-1.01583545019911,5.35782769866944));
#21702=CARTESIAN_POINT('Ctrl Pts',(-8.50243547044494,-1.0164720823066,5.37030863191763));
#21703=CARTESIAN_POINT('Ctrl Pts',(-8.23672961254619,-1.01710871441409,
5.38278956516582));
#21704=CARTESIAN_POINT('Ctrl Pts',(-7.97238846933326,-0.908541417082704,
5.39527049841401));
#21705=CARTESIAN_POINT('Ctrl Pts',(-7.78383148002332,-0.72133492679851,
5.4077514316622));
#21706=CARTESIAN_POINT('Ctrl Pts',(-7.59527449071338,-0.534128436514316,
5.42023236491039));
#21707=CARTESIAN_POINT('Ctrl Pts',(-7.484809931317,-0.270574496755632,5.43271329815858));
#21708=CARTESIAN_POINT('Ctrl Pts',(-7.48353667075686,-0.00487092690814328,
5.44519423140677));
#21709=CARTESIAN_POINT('Ctrl Pts',(-7.48226341019671,0.260832642939345,
5.45767516465496));
#21710=CARTESIAN_POINT('Ctrl Pts',(-7.59019703546757,0.525433154240534,
5.47015609790315));
#21711=CARTESIAN_POINT('Ctrl Pts',(-7.77695120652526,0.714438148393355,
5.48263703115134));
#21712=CARTESIAN_POINT('Ctrl Pts',(-7.96370537758295,0.903443142546176,
5.49511796439953));
#21713=CARTESIAN_POINT('Ctrl Pts',(-8.2269938881484,1.01453885915662,5.50759889764772));
#21714=CARTESIAN_POINT('Ctrl Pts',(-8.49269364459171,1.01644874085989,5.52007983089592));
#21715=CARTESIAN_POINT('Ctrl Pts',(-8.75839340103501,1.01835862256315,5.53256076414411));
#21716=CARTESIAN_POINT('Ctrl Pts',(-9.02325176140399,0.91105928897892,5.5450416973923));
#21717=CARTESIAN_POINT('Ctrl Pts',(-9.2127036753585,0.724758509267386,5.55752263064049));
#21718=CARTESIAN_POINT('Ctrl Pts',(-9.40215558931301,0.538457729555853,
5.57000356388868));
#21719=CARTESIAN_POINT('Ctrl Pts',(-9.51388182535846,0.275436159672167,
5.58248449713687));
#21720=CARTESIAN_POINT('Ctrl Pts',(-9.51642831724057,0.00974174196406534,
5.59496543038506));
#21721=CARTESIAN_POINT('Ctrl Pts',(-9.51645943884197,0.00649459406646887,
5.59511796439953));
#21722=CARTESIAN_POINT('Ctrl Pts',(-9.516475,0.00324729703355471,5.59527049841401));
#21723=CARTESIAN_POINT('Ctrl Pts',(-9.516475,1.83923253541878E-13,5.59542303242849));
#21724=CARTESIAN_POINT('Ctrl Pts',(-9.516475,2.17840591823729E-13,5.35457696757151));
#21725=CARTESIAN_POINT('Ctrl Pts',(-9.51647500000006,-0.265706620583756,
5.3670579008197));
#21726=CARTESIAN_POINT('Ctrl Pts',(-9.40727465387206,-0.529786878176955,
5.37953883406789));
#21727=CARTESIAN_POINT('Ctrl Pts',(-9.2196169190777,-0.717894780174728,
5.39201976731608));
#21728=CARTESIAN_POINT('Ctrl Pts',(-9.03195918428333,-0.906002682172501,
5.40450070056427));
#21729=CARTESIAN_POINT('Ctrl Pts',(-8.76814132834371,-1.01583545019911,
5.41698163381246));
#21730=CARTESIAN_POINT('Ctrl Pts',(-8.50243547044496,-1.0164720823066,5.42946256706065));
#21731=CARTESIAN_POINT('Ctrl Pts',(-8.2367296125462,-1.01710871441409,5.44194350030884));
#21732=CARTESIAN_POINT('Ctrl Pts',(-7.97238846933326,-0.908541417082706,
5.45442443355703));
#21733=CARTESIAN_POINT('Ctrl Pts',(-7.78383148002332,-0.721334926798508,
5.46690536680522));
#21734=CARTESIAN_POINT('Ctrl Pts',(-7.59527449071338,-0.534128436514311,
5.47938630005342));
#21735=CARTESIAN_POINT('Ctrl Pts',(-7.484809931317,-0.27057449675562,5.49186723330161));
#21736=CARTESIAN_POINT('Ctrl Pts',(-7.48353667075686,-0.00487092690812689,
5.5043481665498));
#21737=CARTESIAN_POINT('Ctrl Pts',(-7.48226341019671,0.260832642939366,
5.51682909979799));
#21738=CARTESIAN_POINT('Ctrl Pts',(-7.59019703546758,0.525433154240558,
5.52931003304618));
#21739=CARTESIAN_POINT('Ctrl Pts',(-7.77695120652528,0.714438148393377,
5.54179096629437));
#21740=CARTESIAN_POINT('Ctrl Pts',(-7.96370537758298,0.903443142546195,
5.55427189954256));
#21741=CARTESIAN_POINT('Ctrl Pts',(-8.22699388814844,1.01453885915664,5.56675283279075));
#21742=CARTESIAN_POINT('Ctrl Pts',(-8.49269364459175,1.01644874085989,5.57923376603894));
#21743=CARTESIAN_POINT('Ctrl Pts',(-8.75839340103506,1.01835862256314,5.59171469928713));
#21744=CARTESIAN_POINT('Ctrl Pts',(-9.02325176140404,0.911059288978893,
5.60419563253532));
#21745=CARTESIAN_POINT('Ctrl Pts',(-9.21270367535854,0.724758509267344,
5.61667656578351));
#21746=CARTESIAN_POINT('Ctrl Pts',(-9.40215558931305,0.538457729555796,
5.62915749903171));
#21747=CARTESIAN_POINT('Ctrl Pts',(-9.51388182535848,0.275436159672098,
5.64163843227989));
#21748=CARTESIAN_POINT('Ctrl Pts',(-9.51642831724057,0.00974174196399118,
5.65411936552809));
#21749=CARTESIAN_POINT('Ctrl Pts',(-9.51645943884197,0.00649459406642359,
5.65427189954256));
#21750=CARTESIAN_POINT('Ctrl Pts',(-9.516475,0.0032472970335383,5.65442443355704));
#21751=CARTESIAN_POINT('Ctrl Pts',(-9.516475,1.9642208857481E-13,5.65457696757151));
#21752=CARTESIAN_POINT('Origin',(-8.5,0.,1.24542303242842));
#21753=CARTESIAN_POINT('',(-9.51651055362945,-2.20920755512588E-6,4.99542303242849));
#21754=CARTESIAN_POINT('',(-9.51596748085183,0.000899308347576677,5.05457696757151));
#21755=CARTESIAN_POINT('',(-9.516475,1.78524650477582E-12,1.24542303242842));
#21756=CARTESIAN_POINT('Ctrl Pts',(-9.516475,1.83425324399812E-13,4.99542303242849));
#21757=CARTESIAN_POINT('Ctrl Pts',(-9.51647500000005,-0.265706620583785,
5.00790396567668));
#21758=CARTESIAN_POINT('Ctrl Pts',(-9.40727465387205,-0.529786878176977,
5.02038489892487));
#21759=CARTESIAN_POINT('Ctrl Pts',(-9.21961691907768,-0.717894780174742,
5.03286583217306));
#21760=CARTESIAN_POINT('Ctrl Pts',(-9.03195918428332,-0.906002682172508,
5.04534676542125));
#21761=CARTESIAN_POINT('Ctrl Pts',(-8.7681413283437,-1.01583545019911,5.05782769866944));
#21762=CARTESIAN_POINT('Ctrl Pts',(-8.50243547044495,-1.0164720823066,5.07030863191763));
#21763=CARTESIAN_POINT('Ctrl Pts',(-8.2367296125462,-1.01710871441409,5.08278956516582));
#21764=CARTESIAN_POINT('Ctrl Pts',(-7.97238846933326,-0.908541417082708,
5.09527049841401));
#21765=CARTESIAN_POINT('Ctrl Pts',(-7.78383148002333,-0.721334926798515,
5.1077514316622));
#21766=CARTESIAN_POINT('Ctrl Pts',(-7.59527449071339,-0.534128436514322,
5.12023236491039));
#21767=CARTESIAN_POINT('Ctrl Pts',(-7.484809931317,-0.270574496755639,5.13271329815858));
#21768=CARTESIAN_POINT('Ctrl Pts',(-7.48353667075686,-0.00487092690815026,
5.14519423140677));
#21769=CARTESIAN_POINT('Ctrl Pts',(-7.48226341019671,0.260832642939338,
5.15767516465496));
#21770=CARTESIAN_POINT('Ctrl Pts',(-7.59019703546757,0.525433154240528,
5.17015609790315));
#21771=CARTESIAN_POINT('Ctrl Pts',(-7.77695120652526,0.71443814839335,5.18263703115134));
#21772=CARTESIAN_POINT('Ctrl Pts',(-7.96370537758295,0.903443142546172,
5.19511796439953));
#21773=CARTESIAN_POINT('Ctrl Pts',(-8.22699388814839,1.01453885915662,5.20759889764772));
#21774=CARTESIAN_POINT('Ctrl Pts',(-8.4926936445917,1.01644874085989,5.22007983089591));
#21775=CARTESIAN_POINT('Ctrl Pts',(-8.75839340103501,1.01835862256315,5.23256076414411));
#21776=CARTESIAN_POINT('Ctrl Pts',(-9.02325176140398,0.911059288978924,
5.2450416973923));
#21777=CARTESIAN_POINT('Ctrl Pts',(-9.2127036753585,0.724758509267391,5.25752263064049));
#21778=CARTESIAN_POINT('Ctrl Pts',(-9.40215558931301,0.538457729555859,
5.27000356388868));
#21779=CARTESIAN_POINT('Ctrl Pts',(-9.51388182535846,0.275436159672174,
5.28248449713687));
#21780=CARTESIAN_POINT('Ctrl Pts',(-9.51642831724057,0.00974174196407231,
5.29496543038506));
#21781=CARTESIAN_POINT('Ctrl Pts',(-9.51645943884197,0.00649459406647103,
5.29511796439953));
#21782=CARTESIAN_POINT('Ctrl Pts',(-9.516475,0.00324729703355204,5.29527049841401));
#21783=CARTESIAN_POINT('Ctrl Pts',(-9.516475,1.76451799697528E-13,5.29542303242849));
#21784=CARTESIAN_POINT('Ctrl Pts',(-9.51596748085183,0.000899308347576649,
5.05457696757151));
#21785=CARTESIAN_POINT('Ctrl Pts',(-9.51393632712024,-0.244280703320957,
5.06608589723497));
#21786=CARTESIAN_POINT('Ctrl Pts',(-9.30196512874467,-0.831606259329029,
5.09350216805006));
#21787=CARTESIAN_POINT('Ctrl Pts',(-8.31719720097595,-1.18865749368552,
5.13682578001674));
#21788=CARTESIAN_POINT('Ctrl Pts',(-7.55616952889954,-0.605685554543534,
5.17659413289581));
#21789=CARTESIAN_POINT('Ctrl Pts',(-7.44670579394524,0.0847130526542142,
5.20840881519905));
#21790=CARTESIAN_POINT('Ctrl Pts',(-7.66510184151263,0.748742955970089,
5.2402234975023));
#21791=CARTESIAN_POINT('Ctrl Pts',(-8.50951785842748,1.20259424204374,5.27999185038134));
#21792=CARTESIAN_POINT('Ctrl Pts',(-9.37060850264513,0.722810098535887,
5.32076089726302));
#21793=CARTESIAN_POINT('Ctrl Pts',(-9.51441702760733,0.190923916089248,
5.34562260299307));
#21794=CARTESIAN_POINT('Ctrl Pts',(-9.51491083301307,-0.000352273535940736,
5.35457696757151));
#21795=CARTESIAN_POINT('Origin',(-8.5,0.,1.24542303242842));
#21796=CARTESIAN_POINT('',(-9.51625559736582,-0.000198078035846429,4.69542303242848));
#21797=CARTESIAN_POINT('',(-9.5168797764423,1.75559250602679E-5,4.75457696757151));
#21798=CARTESIAN_POINT('',(-9.516475,1.78524650477582E-12,1.24542303242842));
#21799=CARTESIAN_POINT('Ctrl Pts',(-9.51546470589177,-0.000912099681457321,
4.69542303242849));
#21800=CARTESIAN_POINT('Ctrl Pts',(-9.51640331012323,-0.11186706289642,
4.70062983186786));
#21801=CARTESIAN_POINT('Ctrl Pts',(-9.44878420264641,-0.560795848238884,
4.72174397245884));
#21802=CARTESIAN_POINT('Ctrl Pts',(-8.79017906601008,-1.16700051389882,
4.75876545420146));
#21803=CARTESIAN_POINT('Ctrl Pts',(-7.6762153949145,-0.874872134276515,
4.80648747765633));
#21804=CARTESIAN_POINT('Ctrl Pts',(-7.3176700873064,0.219522361823356,4.85420950111118));
#21805=CARTESIAN_POINT('Ctrl Pts',(-8.04665782451571,1.11391398795103,4.90193152456605));
#21806=CARTESIAN_POINT('Ctrl Pts',(-8.99902690165246,1.00431225253282,4.9416998774451));
#21807=CARTESIAN_POINT('Ctrl Pts',(-9.43822092306757,0.478999650422338,
4.97286371339925));
#21808=CARTESIAN_POINT('Ctrl Pts',(-9.51760254656266,0.154825683554372,
4.98812020820177));
#21809=CARTESIAN_POINT('Ctrl Pts',(-9.51778639424793,-8.14865418414124E-5,
4.99542303242849));
#21810=CARTESIAN_POINT('Ctrl Pts',(-9.51823949807117,7.65296501495289E-5,
4.75457696757151));
#21811=CARTESIAN_POINT('Ctrl Pts',(-9.51824207547116,-0.0032626182231765,
4.75473450917363));
#21812=CARTESIAN_POINT('Ctrl Pts',(-9.51666993996602,-0.343764340190618,
4.77079939192736));
#21813=CARTESIAN_POINT('Ctrl Pts',(-9.13946832655052,-1.01853019590215,
4.80277161583271));
#21814=CARTESIAN_POINT('Ctrl Pts',(-8.18251236732564,-1.0755801003455,4.84253996871177));
#21815=CARTESIAN_POINT('Ctrl Pts',(-7.64801679391654,-0.625083676278862,
4.87435465101502));
#21816=CARTESIAN_POINT('Ctrl Pts',(-7.37871875701052,0.0199830748479729,
4.90616933331825));
#21817=CARTESIAN_POINT('Ctrl Pts',(-7.72036584095294,0.915693223013455,
4.94593768619731));
#21818=CARTESIAN_POINT('Ctrl Pts',(-8.85007720703,1.15045210196194,4.99365970965217));
#21819=CARTESIAN_POINT('Ctrl Pts',(-9.46169735923061,0.526259520213707,
5.02987280344356));
#21820=CARTESIAN_POINT('Ctrl Pts',(-9.5167437346103,0.0946006873223545,
5.05017855608335));
#21821=CARTESIAN_POINT('Ctrl Pts',(-9.51596748085183,0.000899308347576649,
5.05457696757151));
#21822=CARTESIAN_POINT('Origin',(-8.5,0.,1.24542303242842));
#21823=CARTESIAN_POINT('',(-9.51614091975708,0.000208621397402929,4.39542303242849));
#21824=CARTESIAN_POINT('',(-9.516475,2.24316187383949E-13,4.45457696757151));
#21825=CARTESIAN_POINT('',(-9.516475,1.78524650477582E-12,1.24542303242842));
#21826=CARTESIAN_POINT('Ctrl Pts',(-9.516475,1.97372373804382E-13,4.39542303242849));
#21827=CARTESIAN_POINT('Ctrl Pts',(-9.51647500000005,-0.265706620583771,
4.40790396567668));
#21828=CARTESIAN_POINT('Ctrl Pts',(-9.40727465387206,-0.529786878176964,
4.42038489892487));
#21829=CARTESIAN_POINT('Ctrl Pts',(-9.21961691907769,-0.717894780174732,
4.43286583217306));
#21830=CARTESIAN_POINT('Ctrl Pts',(-9.03195918428333,-0.9060026821725,4.44534676542125));
#21831=CARTESIAN_POINT('Ctrl Pts',(-8.76814132834372,-1.01583545019911,
4.45782769866944));
#21832=CARTESIAN_POINT('Ctrl Pts',(-8.50243547044496,-1.0164720823066,4.47030863191763));
#21833=CARTESIAN_POINT('Ctrl Pts',(-8.23672961254621,-1.01710871441409,
4.48278956516582));
#21834=CARTESIAN_POINT('Ctrl Pts',(-7.97238846933327,-0.908541417082715,
4.49527049841401));
#21835=CARTESIAN_POINT('Ctrl Pts',(-7.78383148002334,-0.721334926798525,
4.5077514316622));
#21836=CARTESIAN_POINT('Ctrl Pts',(-7.5952744907134,-0.534128436514334,
4.52023236491039));
#21837=CARTESIAN_POINT('Ctrl Pts',(-7.48480993131701,-0.270574496755652,
4.53271329815858));
#21838=CARTESIAN_POINT('Ctrl Pts',(-7.48353667075686,-0.0048709269081642,
4.54519423140677));
#21839=CARTESIAN_POINT('Ctrl Pts',(-7.48226341019671,0.260832642939324,
4.55767516465496));
#21840=CARTESIAN_POINT('Ctrl Pts',(-7.59019703546756,0.525433154240515,
4.57015609790315));
#21841=CARTESIAN_POINT('Ctrl Pts',(-7.77695120652525,0.71443814839334,4.58263703115134));
#21842=CARTESIAN_POINT('Ctrl Pts',(-7.96370537758293,0.903443142546165,
4.59511796439953));
#21843=CARTESIAN_POINT('Ctrl Pts',(-8.22699388814838,1.01453885915662,4.60759889764772));
#21844=CARTESIAN_POINT('Ctrl Pts',(-8.49269364459169,1.01644874085989,4.62007983089591));
#21845=CARTESIAN_POINT('Ctrl Pts',(-8.75839340103499,1.01835862256315,4.63256076414411));
#21846=CARTESIAN_POINT('Ctrl Pts',(-9.02325176140397,0.911059288978931,
4.64504169739229));
#21847=CARTESIAN_POINT('Ctrl Pts',(-9.21270367535849,0.724758509267401,
4.65752263064049));
#21848=CARTESIAN_POINT('Ctrl Pts',(-9.402155589313,0.538457729555871,4.67000356388868));
#21849=CARTESIAN_POINT('Ctrl Pts',(-9.51388182535845,0.275436159672188,
4.68248449713687));
#21850=CARTESIAN_POINT('Ctrl Pts',(-9.51642831724057,0.00974174196408626,
4.69496543038506));
#21851=CARTESIAN_POINT('Ctrl Pts',(-9.51645943884197,0.00649459406648979,
4.69511796439953));
#21852=CARTESIAN_POINT('Ctrl Pts',(-9.516475,0.00324729703357563,4.69527049841401));
#21853=CARTESIAN_POINT('Ctrl Pts',(-9.516475,2.04843827648732E-13,4.69542303242848));
#21854=CARTESIAN_POINT('Ctrl Pts',(-9.516475,2.24316187383949E-13,4.45457696757151));
#21855=CARTESIAN_POINT('Ctrl Pts',(-9.51647500000006,-0.265706620583744,
4.4670579008197));
#21856=CARTESIAN_POINT('Ctrl Pts',(-9.40727465387207,-0.52978687817694,
4.47953883406789));
#21857=CARTESIAN_POINT('Ctrl Pts',(-9.21961691907771,-0.717894780174713,
4.49201976731608));
#21858=CARTESIAN_POINT('Ctrl Pts',(-9.03195918428336,-0.906002682172486,
4.50450070056427));
#21859=CARTESIAN_POINT('Ctrl Pts',(-8.76814132834374,-1.0158354501991,4.51698163381246));
#21860=CARTESIAN_POINT('Ctrl Pts',(-8.50243547044499,-1.0164720823066,4.52946256706065));
#21861=CARTESIAN_POINT('Ctrl Pts',(-8.23672961254624,-1.0171087144141,4.54194350030884));
#21862=CARTESIAN_POINT('Ctrl Pts',(-7.9723884693333,-0.908541417082729,
4.55442443355703));
#21863=CARTESIAN_POINT('Ctrl Pts',(-7.78383148002335,-0.721334926798543,
4.56690536680522));
#21864=CARTESIAN_POINT('Ctrl Pts',(-7.59527449071341,-0.534128436514358,
4.57938630005341));
#21865=CARTESIAN_POINT('Ctrl Pts',(-7.48480993131702,-0.270574496755679,
4.5918672333016));
#21866=CARTESIAN_POINT('Ctrl Pts',(-7.48353667075686,-0.00487092690819115,
4.60434816654979));
#21867=CARTESIAN_POINT('Ctrl Pts',(-7.4822634101967,0.260832642939297,4.61682909979799));
#21868=CARTESIAN_POINT('Ctrl Pts',(-7.59019703546755,0.525433154240491,
4.62931003304617));
#21869=CARTESIAN_POINT('Ctrl Pts',(-7.77695120652523,0.714438148393321,
4.64179096629437));
#21870=CARTESIAN_POINT('Ctrl Pts',(-7.96370537758291,0.90344314254615,4.65427189954256));
#21871=CARTESIAN_POINT('Ctrl Pts',(-8.22699388814835,1.01453885915661,4.66675283279075));
#21872=CARTESIAN_POINT('Ctrl Pts',(-8.49269364459166,1.01644874085989,4.67923376603894));
#21873=CARTESIAN_POINT('Ctrl Pts',(-8.75839340103497,1.01835862256316,4.69171469928713));
#21874=CARTESIAN_POINT('Ctrl Pts',(-9.02325176140395,0.911059288978945,
4.70419563253532));
#21875=CARTESIAN_POINT('Ctrl Pts',(-9.21270367535847,0.72475850926742,4.71667656578351));
#21876=CARTESIAN_POINT('Ctrl Pts',(-9.40215558931299,0.538457729555895,
4.7291574990317));
#21877=CARTESIAN_POINT('Ctrl Pts',(-9.51388182535845,0.275436159672215,
4.74163843227989));
#21878=CARTESIAN_POINT('Ctrl Pts',(-9.51642831724057,0.00974174196411321,
4.75411936552808));
#21879=CARTESIAN_POINT('Ctrl Pts',(-9.51645943884197,0.00649459406651192,
4.75427189954256));
#21880=CARTESIAN_POINT('Ctrl Pts',(-9.516475,0.00324729703359293,4.75442443355703));
#21881=CARTESIAN_POINT('Ctrl Pts',(-9.516475,2.17342662681664E-13,4.75457696757151));
#21882=CARTESIAN_POINT('Origin',(-8.5,0.,1.24542303242842));
#21883=CARTESIAN_POINT('',(-9.51670427207195,7.39794657305722E-5,4.09542303242849));
#21884=CARTESIAN_POINT('',(-9.51599658147032,0.000173149125154374,4.15457696757151));
#21885=CARTESIAN_POINT('',(-9.516475,1.78524650477582E-12,1.24542303242842));
#21886=CARTESIAN_POINT('Ctrl Pts',(-9.51784765822069,0.000442917101461892,
4.09542303242849));
#21887=CARTESIAN_POINT('Ctrl Pts',(-9.51577594300805,-0.303314166886826,
4.10974173804841));
#21888=CARTESIAN_POINT('Ctrl Pts',(-9.20951320363247,-0.947629617697905,
4.13996778481995));
#21889=CARTESIAN_POINT('Ctrl Pts',(-8.11269623164964,-1.13845943309904,
4.18610117274311));
#21890=CARTESIAN_POINT('Ctrl Pts',(-7.3324614462396,-0.288404622204439,
4.23382319619797));
#21891=CARTESIAN_POINT('Ctrl Pts',(-7.57791048256601,0.638296068450016,
4.27359154907703));
#21892=CARTESIAN_POINT('Ctrl Pts',(-8.17310957881519,1.0048619996478,4.30540623138027));
#21893=CARTESIAN_POINT('Ctrl Pts',(-8.87006013423126,1.05864368236586,4.33722091368351));
#21894=CARTESIAN_POINT('Ctrl Pts',(-9.43118836112104,0.602224246389519,
4.36722651403292));
#21895=CARTESIAN_POINT('Ctrl Pts',(-9.51585152810173,0.132104578598546,
4.38927844380651));
#21896=CARTESIAN_POINT('Ctrl Pts',(-9.5151537803744,0.000825055327915034,
4.39542303242849));
#21897=CARTESIAN_POINT('Ctrl Pts',(-9.516475,2.38512201359551E-13,4.15457696757151));
#21898=CARTESIAN_POINT('Ctrl Pts',(-9.51647500000006,-0.26570662058373,
4.1670579008197));
#21899=CARTESIAN_POINT('Ctrl Pts',(-9.40727465387208,-0.529786878176927,
4.17953883406789));
#21900=CARTESIAN_POINT('Ctrl Pts',(-9.21961691907772,-0.717894780174703,
4.19201976731608));
#21901=CARTESIAN_POINT('Ctrl Pts',(-9.03195918428337,-0.906002682172479,
4.20450070056427));
#21902=CARTESIAN_POINT('Ctrl Pts',(-8.76814132834376,-1.01583545019909,
4.21698163381246));
#21903=CARTESIAN_POINT('Ctrl Pts',(-8.502435470445,-1.0164720823066,4.22946256706065));
#21904=CARTESIAN_POINT('Ctrl Pts',(-8.23672961254625,-1.0171087144141,4.24194350030884));
#21905=CARTESIAN_POINT('Ctrl Pts',(-7.97238846933331,-0.908541417082736,
4.25442443355703));
#21906=CARTESIAN_POINT('Ctrl Pts',(-7.78383148002336,-0.721334926798554,
4.26690536680522));
#21907=CARTESIAN_POINT('Ctrl Pts',(-7.59527449071342,-0.534128436514371,
4.27938630005341));
#21908=CARTESIAN_POINT('Ctrl Pts',(-7.48480993131702,-0.270574496755694,
4.2918672333016));
#21909=CARTESIAN_POINT('Ctrl Pts',(-7.48353667075686,-0.00487092690820534,
4.30434816654979));
#21910=CARTESIAN_POINT('Ctrl Pts',(-7.48226341019669,0.260832642939283,
4.31682909979798));
#21911=CARTESIAN_POINT('Ctrl Pts',(-7.59019703546754,0.525433154240478,
4.32931003304617));
#21912=CARTESIAN_POINT('Ctrl Pts',(-7.77695120652522,0.714438148393311,
4.34179096629437));
#21913=CARTESIAN_POINT('Ctrl Pts',(-7.9637053775829,0.903443142546145,4.35427189954256));
#21914=CARTESIAN_POINT('Ctrl Pts',(-8.22699388814834,1.01453885915661,4.36675283279075));
#21915=CARTESIAN_POINT('Ctrl Pts',(-8.49269364459165,1.01644874085989,4.37923376603894));
#21916=CARTESIAN_POINT('Ctrl Pts',(-8.75839340103496,1.01835862256316,4.39171469928713));
#21917=CARTESIAN_POINT('Ctrl Pts',(-9.02325176140394,0.911059288978948,
4.40419563253532));
#21918=CARTESIAN_POINT('Ctrl Pts',(-9.21270367535846,0.724758509267425,
4.41667656578351));
#21919=CARTESIAN_POINT('Ctrl Pts',(-9.40215558931298,0.538457729555901,
4.4291574990317));
#21920=CARTESIAN_POINT('Ctrl Pts',(-9.51388182535844,0.275436159672222,
4.44163843227989));
#21921=CARTESIAN_POINT('Ctrl Pts',(-9.51642831724057,0.00974174196412018,
4.45411936552808));
#21922=CARTESIAN_POINT('Ctrl Pts',(-9.51645943884197,0.00649459406651889,
4.45427189954256));
#21923=CARTESIAN_POINT('Ctrl Pts',(-9.516475,0.00324729703359991,4.45442443355703));
#21924=CARTESIAN_POINT('Ctrl Pts',(-9.516475,2.24316187383949E-13,4.45457696757151));
#21925=CARTESIAN_POINT('Origin',(-8.5,0.,1.24542303242842));
#21926=CARTESIAN_POINT('',(-9.516475,2.11319423208952E-13,3.79542303242848));
#21927=CARTESIAN_POINT('',(-9.51647837596764,1.62386119748113E-6,3.85457696757151));
#21928=CARTESIAN_POINT('',(-9.516475,1.78524650477582E-12,1.24542303242842));
#21929=CARTESIAN_POINT('Ctrl Pts',(-9.516475,2.25764401755587E-13,3.79542303242848));
#21930=CARTESIAN_POINT('Ctrl Pts',(-9.51647500000006,-0.265706620583743,
3.80790396567667));
#21931=CARTESIAN_POINT('Ctrl Pts',(-9.40727465387207,-0.529786878176939,
3.82038489892486));
#21932=CARTESIAN_POINT('Ctrl Pts',(-9.21961691907771,-0.717894780174712,
3.83286583217305));
#21933=CARTESIAN_POINT('Ctrl Pts',(-9.03195918428336,-0.906002682172486,
3.84534676542125));
#21934=CARTESIAN_POINT('Ctrl Pts',(-8.76814132834375,-1.0158354501991,3.85782769866944));
#21935=CARTESIAN_POINT('Ctrl Pts',(-8.50243547044499,-1.0164720823066,3.87030863191763));
#21936=CARTESIAN_POINT('Ctrl Pts',(-8.23672961254624,-1.0171087144141,3.88278956516582));
#21937=CARTESIAN_POINT('Ctrl Pts',(-7.9723884693333,-0.908541417082729,
3.89527049841401));
#21938=CARTESIAN_POINT('Ctrl Pts',(-7.78383148002336,-0.721334926798544,
3.9077514316622));
#21939=CARTESIAN_POINT('Ctrl Pts',(-7.59527449071341,-0.53412843651436,
3.92023236491039));
#21940=CARTESIAN_POINT('Ctrl Pts',(-7.48480993131702,-0.270574496755681,
3.93271329815858));
#21941=CARTESIAN_POINT('Ctrl Pts',(-7.48353667075686,-0.0048709269081926,
3.94519423140677));
#21942=CARTESIAN_POINT('Ctrl Pts',(-7.4822634101967,0.260832642939296,3.95767516465496));
#21943=CARTESIAN_POINT('Ctrl Pts',(-7.59019703546755,0.52543315424049,3.97015609790315));
#21944=CARTESIAN_POINT('Ctrl Pts',(-7.77695120652523,0.71443814839332,3.98263703115134));
#21945=CARTESIAN_POINT('Ctrl Pts',(-7.96370537758291,0.90344314254615,3.99511796439953));
#21946=CARTESIAN_POINT('Ctrl Pts',(-8.22699388814835,1.01453885915661,4.00759889764772));
#21947=CARTESIAN_POINT('Ctrl Pts',(-8.49269364459166,1.01644874085989,4.02007983089591));
#21948=CARTESIAN_POINT('Ctrl Pts',(-8.75839340103497,1.01835862256316,4.0325607641441));
#21949=CARTESIAN_POINT('Ctrl Pts',(-9.02325176140394,0.911059288978945,
4.04504169739229));
#21950=CARTESIAN_POINT('Ctrl Pts',(-9.21270367535847,0.724758509267421,
4.05752263064048));
#21951=CARTESIAN_POINT('Ctrl Pts',(-9.40215558931299,0.538457729555896,
4.07000356388867));
#21952=CARTESIAN_POINT('Ctrl Pts',(-9.51388182535845,0.275436159672217,
4.08248449713686));
#21953=CARTESIAN_POINT('Ctrl Pts',(-9.51642831724057,0.00974174196411465,
4.09496543038505));
#21954=CARTESIAN_POINT('Ctrl Pts',(-9.51645943884197,0.00649459406651096,
4.09511796439953));
#21955=CARTESIAN_POINT('Ctrl Pts',(-9.516475,0.00324729703358956,4.09527049841401));
#21956=CARTESIAN_POINT('Ctrl Pts',(-9.516475,2.11568387779985E-13,4.09542303242848));
#21957=CARTESIAN_POINT('Ctrl Pts',(-9.5174412885927,0.000464791732992929,
3.85457696757151));
#21958=CARTESIAN_POINT('Ctrl Pts',(-9.51678187338335,-0.124250478191715,
3.86044869786864));
#21959=CARTESIAN_POINT('Ctrl Pts',(-9.45952256246098,-0.418651775766005,
3.87427409874159));
#21960=CARTESIAN_POINT('Ctrl Pts',(-9.08719526120723,-0.955443705498223,
3.90400684076614));
#21961=CARTESIAN_POINT('Ctrl Pts',(-8.14851560934884,-1.15012269943444,
3.9437751936452));
#21962=CARTESIAN_POINT('Ctrl Pts',(-7.34215909770885,-0.324805379838734,
3.99149721710006));
#21963=CARTESIAN_POINT('Ctrl Pts',(-7.60098238778599,0.797364195232309,
4.03921924055492));
#21964=CARTESIAN_POINT('Ctrl Pts',(-8.68421342859387,1.18834317539854,4.08694126400978));
#21965=CARTESIAN_POINT('Ctrl Pts',(-9.42205359078049,0.622675900476843,
4.12539383968198));
#21966=CARTESIAN_POINT('Ctrl Pts',(-9.51547907546729,0.142299165762317,
4.14793907420255));
#21967=CARTESIAN_POINT('Ctrl Pts',(-9.51476624073027,0.000618433764589824,
4.15457696757151));
#21968=CARTESIAN_POINT('Origin',(-8.5,0.,1.24542303242842));
#21969=CARTESIAN_POINT('',(-9.51608842318713,-2.89235217017741E-5,3.49542303242848));
#21970=CARTESIAN_POINT('',(-9.516475,2.45236761490803E-13,3.55457696757151));
#21971=CARTESIAN_POINT('',(-9.516475,1.78524650477582E-12,1.24542303242842));
#21972=CARTESIAN_POINT('Ctrl Pts',(-9.51486126663803,-0.000120738881975849,
3.49542303242848));
#21973=CARTESIAN_POINT('Ctrl Pts',(-9.51514336021873,-0.160856911785796,
3.50294630307734));
#21974=CARTESIAN_POINT('Ctrl Pts',(-9.40340564418365,-0.6611996367537,3.52637691487781));
#21975=CARTESIAN_POINT('Ctrl Pts',(-8.61746895833269,-1.19688117390714,
3.5657148678299));
#21976=CARTESIAN_POINT('Ctrl Pts',(-7.73570976145469,-0.820689576164182,
3.60548322070896));
#21977=CARTESIAN_POINT('Ctrl Pts',(-7.4585680161445,-0.178953649869286,
3.6372979030122));
#21978=CARTESIAN_POINT('Ctrl Pts',(-7.50559368937304,0.518485331080344,
3.66911258531544));
#21979=CARTESIAN_POINT('Ctrl Pts',(-8.21119763983049,1.1674402328969,3.70888093819449));
#21980=CARTESIAN_POINT('Ctrl Pts',(-9.25750654792175,0.891435180077196,
3.75363564409078));
#21981=CARTESIAN_POINT('Ctrl Pts',(-9.51442267342405,0.274180741296169,
3.78248300883544));
#21982=CARTESIAN_POINT('Ctrl Pts',(-9.51684974171157,-0.000865705360034545,
3.79542303242848));
#21983=CARTESIAN_POINT('Ctrl Pts',(-9.516475,2.45236761490803E-13,3.55457696757151));
#21984=CARTESIAN_POINT('Ctrl Pts',(-9.51647500000006,-0.265706620583731,
3.5670579008197));
#21985=CARTESIAN_POINT('Ctrl Pts',(-9.40727465387207,-0.529786878176936,
3.57953883406789));
#21986=CARTESIAN_POINT('Ctrl Pts',(-9.21961691907771,-0.717894780174714,
3.59201976731608));
#21987=CARTESIAN_POINT('Ctrl Pts',(-9.03195918428335,-0.906002682172492,
3.60450070056427));
#21988=CARTESIAN_POINT('Ctrl Pts',(-8.76814132834373,-1.0158354501991,3.61698163381246));
#21989=CARTESIAN_POINT('Ctrl Pts',(-8.50243547044497,-1.0164720823066,3.62946256706065));
#21990=CARTESIAN_POINT('Ctrl Pts',(-8.23672961254621,-1.01710871441409,
3.64194350030884));
#21991=CARTESIAN_POINT('Ctrl Pts',(-7.97238846933326,-0.908541417082711,
3.65442443355703));
#21992=CARTESIAN_POINT('Ctrl Pts',(-7.78383148002332,-0.721334926798513,
3.66690536680522));
#21993=CARTESIAN_POINT('Ctrl Pts',(-7.59527449071338,-0.534128436514314,
3.67938630005342));
#21994=CARTESIAN_POINT('Ctrl Pts',(-7.484809931317,-0.270574496755621,3.69186723330161));
#21995=CARTESIAN_POINT('Ctrl Pts',(-7.48353667075686,-0.0048709269081254,
3.7043481665498));
#21996=CARTESIAN_POINT('Ctrl Pts',(-7.48226341019672,0.26083264293937,3.71682909979799));
#21997=CARTESIAN_POINT('Ctrl Pts',(-7.59019703546759,0.525433154240564,
3.72931003304618));
#21998=CARTESIAN_POINT('Ctrl Pts',(-7.77695120652529,0.714438148393383,
3.74179096629437));
#21999=CARTESIAN_POINT('Ctrl Pts',(-7.96370537758299,0.903443142546202,
3.75427189954256));
#22000=CARTESIAN_POINT('Ctrl Pts',(-8.22699388814845,1.01453885915664,3.76675283279075));
#22001=CARTESIAN_POINT('Ctrl Pts',(-8.49269364459177,1.01644874085989,3.77923376603894));
#22002=CARTESIAN_POINT('Ctrl Pts',(-8.75839340103508,1.01835862256313,3.79171469928713));
#22003=CARTESIAN_POINT('Ctrl Pts',(-9.02325176140406,0.911059288978882,
3.80419563253532));
#22004=CARTESIAN_POINT('Ctrl Pts',(-9.21270367535856,0.724758509267328,
3.81667656578351));
#22005=CARTESIAN_POINT('Ctrl Pts',(-9.40215558931306,0.538457729555774,
3.82915749903171));
#22006=CARTESIAN_POINT('Ctrl Pts',(-9.51388182535849,0.27543615967207,3.8416384322799));
#22007=CARTESIAN_POINT('Ctrl Pts',(-9.51642831724057,0.00974174196396079,
3.85411936552809));
#22008=CARTESIAN_POINT('Ctrl Pts',(-9.51645943884197,0.00649459406641969,
3.85427189954256));
#22009=CARTESIAN_POINT('Ctrl Pts',(-9.516475,0.0032472970335609,3.85442443355703));
#22010=CARTESIAN_POINT('Ctrl Pts',(-9.516475,2.45485726061836E-13,3.85457696757151));
#22011=CARTESIAN_POINT('Origin',(-8.5,0.,1.24542303242842));
#22012=CARTESIAN_POINT('',(-9.516475,2.25266472613521E-13,3.19542303242848));
#22013=CARTESIAN_POINT('',(-9.51601909668223,-0.000125713479535779,3.25457696757151));
#22014=CARTESIAN_POINT('',(-9.516475,1.78524650477582E-12,1.24542303242842));
#22015=CARTESIAN_POINT('Ctrl Pts',(-9.516475,2.32488961886839E-13,3.19542303242848));
#22016=CARTESIAN_POINT('Ctrl Pts',(-9.51647500000006,-0.265706620583743,
3.20790396567667));
#22017=CARTESIAN_POINT('Ctrl Pts',(-9.40727465387207,-0.529786878176947,
3.22038489892487));
#22018=CARTESIAN_POINT('Ctrl Pts',(-9.2196169190777,-0.717894780174723,
3.23286583217306));
#22019=CARTESIAN_POINT('Ctrl Pts',(-9.03195918428334,-0.906002682172499,
3.24534676542125));
#22020=CARTESIAN_POINT('Ctrl Pts',(-8.76814132834372,-1.01583545019911,
3.25782769866944));
#22021=CARTESIAN_POINT('Ctrl Pts',(-8.50243547044496,-1.0164720823066,3.27030863191763));
#22022=CARTESIAN_POINT('Ctrl Pts',(-8.2367296125462,-1.01710871441409,3.28278956516582));
#22023=CARTESIAN_POINT('Ctrl Pts',(-7.97238846933325,-0.908541417082704,
3.29527049841401));
#22024=CARTESIAN_POINT('Ctrl Pts',(-7.78383148002331,-0.721334926798503,
3.3077514316622));
#22025=CARTESIAN_POINT('Ctrl Pts',(-7.59527449071337,-0.534128436514303,
3.32023236491039));
#22026=CARTESIAN_POINT('Ctrl Pts',(-7.48480993131699,-0.270574496755608,
3.33271329815858));
#22027=CARTESIAN_POINT('Ctrl Pts',(-7.48353667075686,-0.00487092690811265,
3.34519423140677));
#22028=CARTESIAN_POINT('Ctrl Pts',(-7.48226341019672,0.260832642939383,
3.35767516465496));
#22029=CARTESIAN_POINT('Ctrl Pts',(-7.59019703546759,0.525433154240575,
3.37015609790315));
#22030=CARTESIAN_POINT('Ctrl Pts',(-7.7769512065253,0.714438148393392,3.38263703115135));
#22031=CARTESIAN_POINT('Ctrl Pts',(-7.963705377583,0.903443142546208,3.39511796439954));
#22032=CARTESIAN_POINT('Ctrl Pts',(-8.22699388814847,1.01453885915664,3.40759889764773));
#22033=CARTESIAN_POINT('Ctrl Pts',(-8.49269364459178,1.01644874085989,3.42007983089592));
#22034=CARTESIAN_POINT('Ctrl Pts',(-8.7583934010351,1.01835862256313,3.43256076414411));
#22035=CARTESIAN_POINT('Ctrl Pts',(-9.02325176140407,0.911059288978876,
3.4450416973923));
#22036=CARTESIAN_POINT('Ctrl Pts',(-9.21270367535857,0.724758509267319,
3.45752263064049));
#22037=CARTESIAN_POINT('Ctrl Pts',(-9.40215558931307,0.538457729555763,
3.47000356388868));
#22038=CARTESIAN_POINT('Ctrl Pts',(-9.51388182535849,0.275436159672058,
3.48248449713687));
#22039=CARTESIAN_POINT('Ctrl Pts',(-9.51642831724057,0.00974174196394805,
3.49496543038506));
#22040=CARTESIAN_POINT('Ctrl Pts',(-9.51645943884197,0.00649459406640212,
3.49511796439954));
#22041=CARTESIAN_POINT('Ctrl Pts',(-9.516475,0.00324729703353853,3.49527049841401));
#22042=CARTESIAN_POINT('Ctrl Pts',(-9.516475,2.18292947911237E-13,3.49542303242848));
#22043=CARTESIAN_POINT('Ctrl Pts',(-9.51464021331442,-0.000505934934279403,
3.25457696757151));
#22044=CARTESIAN_POINT('Ctrl Pts',(-9.51522438392244,-0.150599077304496,
3.26160693347338));
#22045=CARTESIAN_POINT('Ctrl Pts',(-9.41409897557488,-0.639618505323573,
3.28454424052688));
#22046=CARTESIAN_POINT('Ctrl Pts',(-8.65488608504732,-1.19252018450271,
3.32338888873198));
#22047=CARTESIAN_POINT('Ctrl Pts',(-7.58161436923836,-0.774977522330395,
3.37111091218686));
#22048=CARTESIAN_POINT('Ctrl Pts',(-7.35051106244356,0.353226941538064,
3.41883293564171));
#22049=CARTESIAN_POINT('Ctrl Pts',(-8.17695225324716,1.15843154909689,3.46655495909658));
#22050=CARTESIAN_POINT('Ctrl Pts',(-9.11055173066928,0.9406899241179,3.50632331197563));
#22051=CARTESIAN_POINT('Ctrl Pts',(-9.46480985202421,0.402086870851785,
3.53566398146727));
#22052=CARTESIAN_POINT('Ctrl Pts',(-9.51660454730387,0.115906227021547,
3.54909730980729));
#22053=CARTESIAN_POINT('Ctrl Pts',(-9.5172889590067,-0.000538403642920175,
3.55457696757151));
#22054=CARTESIAN_POINT('Origin',(-8.5,0.,1.24542303242842));
#22055=CARTESIAN_POINT('',(-9.516475,2.32239997315806E-13,2.89542303242848));
#22056=CARTESIAN_POINT('',(-9.516475,2.59183810895373E-13,2.95457696757151));
#22057=CARTESIAN_POINT('',(-9.516475,1.78524650477582E-12,1.24542303242842));
#22058=CARTESIAN_POINT('Ctrl Pts',(-9.516475,2.39462486589124E-13,2.89542303242848));
#22059=CARTESIAN_POINT('Ctrl Pts',(-9.51647500000006,-0.265706620583729,
2.90790396567667));
#22060=CARTESIAN_POINT('Ctrl Pts',(-9.40727465387208,-0.529786878176927,
2.92038489892486));
#22061=CARTESIAN_POINT('Ctrl Pts',(-9.21961691907772,-0.717894780174703,
2.93286583217305));
#22062=CARTESIAN_POINT('Ctrl Pts',(-9.03195918428337,-0.906002682172478,
2.94534676542124));
#22063=CARTESIAN_POINT('Ctrl Pts',(-8.76814132834376,-1.01583545019909,
2.95782769866944));
#22064=CARTESIAN_POINT('Ctrl Pts',(-8.50243547044501,-1.0164720823066,2.97030863191763));
#22065=CARTESIAN_POINT('Ctrl Pts',(-8.23672961254625,-1.0171087144141,2.98278956516582));
#22066=CARTESIAN_POINT('Ctrl Pts',(-7.97238846933331,-0.908541417082737,
2.99527049841401));
#22067=CARTESIAN_POINT('Ctrl Pts',(-7.78383148002336,-0.721334926798554,
3.0077514316622));
#22068=CARTESIAN_POINT('Ctrl Pts',(-7.59527449071342,-0.534128436514372,
3.02023236491039));
#22069=CARTESIAN_POINT('Ctrl Pts',(-7.48480993131702,-0.270574496755695,
3.03271329815858));
#22070=CARTESIAN_POINT('Ctrl Pts',(-7.48353667075686,-0.00487092690820629,
3.04519423140677));
#22071=CARTESIAN_POINT('Ctrl Pts',(-7.48226341019669,0.260832642939282,
3.05767516465496));
#22072=CARTESIAN_POINT('Ctrl Pts',(-7.59019703546754,0.525433154240477,
3.07015609790315));
#22073=CARTESIAN_POINT('Ctrl Pts',(-7.77695120652522,0.71443814839331,3.08263703115134));
#22074=CARTESIAN_POINT('Ctrl Pts',(-7.9637053775829,0.903443142546142,3.09511796439953));
#22075=CARTESIAN_POINT('Ctrl Pts',(-8.22699388814834,1.01453885915661,3.10759889764772));
#22076=CARTESIAN_POINT('Ctrl Pts',(-8.49269364459164,1.01644874085989,3.12007983089591));
#22077=CARTESIAN_POINT('Ctrl Pts',(-8.75839340103495,1.01835862256316,3.1325607641441));
#22078=CARTESIAN_POINT('Ctrl Pts',(-9.02325176140393,0.911059288978952,
3.14504169739229));
#22079=CARTESIAN_POINT('Ctrl Pts',(-9.21270367535846,0.72475850926743,3.15752263064048));
#22080=CARTESIAN_POINT('Ctrl Pts',(-9.40215558931298,0.538457729555908,
3.17000356388867));
#22081=CARTESIAN_POINT('Ctrl Pts',(-9.51388182535844,0.27543615967223,3.18248449713686));
#22082=CARTESIAN_POINT('Ctrl Pts',(-9.51642831724057,0.00974174196412835,
3.19496543038505));
#22083=CARTESIAN_POINT('Ctrl Pts',(-9.51645943884197,0.00649459406652706,
3.19511796439953));
#22084=CARTESIAN_POINT('Ctrl Pts',(-9.516475,0.00324729703360808,3.19527049841401));
#22085=CARTESIAN_POINT('Ctrl Pts',(-9.516475,2.32488961886839E-13,3.19542303242848));
#22086=CARTESIAN_POINT('Ctrl Pts',(-9.516475,2.59183810895373E-13,2.95457696757151));
#22087=CARTESIAN_POINT('Ctrl Pts',(-9.51647500000007,-0.26570662058371,
2.9670579008197));
#22088=CARTESIAN_POINT('Ctrl Pts',(-9.40727465387209,-0.529786878176909,
2.97953883406789));
#22089=CARTESIAN_POINT('Ctrl Pts',(-9.21961691907774,-0.717894780174689,
2.99201976731608));
#22090=CARTESIAN_POINT('Ctrl Pts',(-9.03195918428339,-0.906002682172468,
3.00450070056427));
#22091=CARTESIAN_POINT('Ctrl Pts',(-8.76814132834378,-1.01583545019909,
3.01698163381246));
#22092=CARTESIAN_POINT('Ctrl Pts',(-8.50243547044503,-1.0164720823066,3.02946256706065));
#22093=CARTESIAN_POINT('Ctrl Pts',(-8.23672961254627,-1.01710871441411,
3.04194350030884));
#22094=CARTESIAN_POINT('Ctrl Pts',(-7.97238846933333,-0.908541417082747,
3.05442443355703));
#22095=CARTESIAN_POINT('Ctrl Pts',(-7.78383148002338,-0.721334926798568,
3.06690536680522));
#22096=CARTESIAN_POINT('Ctrl Pts',(-7.59527449071343,-0.534128436514389,
3.07938630005341));
#22097=CARTESIAN_POINT('Ctrl Pts',(-7.48480993131702,-0.270574496755714,
3.0918672333016));
#22098=CARTESIAN_POINT('Ctrl Pts',(-7.48353667075686,-0.00487092690822602,
3.10434816654979));
#22099=CARTESIAN_POINT('Ctrl Pts',(-7.48226341019669,0.260832642939262,
3.11682909979798));
#22100=CARTESIAN_POINT('Ctrl Pts',(-7.59019703546753,0.52543315424046,3.12931003304617));
#22101=CARTESIAN_POINT('Ctrl Pts',(-7.7769512065252,0.714438148393296,3.14179096629436));
#22102=CARTESIAN_POINT('Ctrl Pts',(-7.96370537758288,0.903443142546132,
3.15427189954255));
#22103=CARTESIAN_POINT('Ctrl Pts',(-8.22699388814832,1.0145388591566,3.16675283279075));
#22104=CARTESIAN_POINT('Ctrl Pts',(-8.49269364459163,1.01644874085989,3.17923376603894));
#22105=CARTESIAN_POINT('Ctrl Pts',(-8.75839340103493,1.01835862256317,3.19171469928713));
#22106=CARTESIAN_POINT('Ctrl Pts',(-9.02325176140392,0.911059288978963,
3.20419563253532));
#22107=CARTESIAN_POINT('Ctrl Pts',(-9.21270367535844,0.724758509267444,
3.21667656578351));
#22108=CARTESIAN_POINT('Ctrl Pts',(-9.40215558931297,0.538457729555926,
3.2291574990317));
#22109=CARTESIAN_POINT('Ctrl Pts',(-9.51388182535844,0.27543615967225,3.24163843227989));
#22110=CARTESIAN_POINT('Ctrl Pts',(-9.51642831724057,0.00974174196414807,
3.25411936552808));
#22111=CARTESIAN_POINT('Ctrl Pts',(-9.51645943884197,0.00649459406654679,
3.25427189954255));
#22112=CARTESIAN_POINT('Ctrl Pts',(-9.516475,0.0032472970336278,3.25442443355703));
#22113=CARTESIAN_POINT('Ctrl Pts',(-9.516475,2.52210286193088E-13,3.25457696757151));
#22114=CARTESIAN_POINT('Origin',(-8.5,0.,1.24542303242842));
#22115=CARTESIAN_POINT('',(-9.516475,2.31991032744774E-13,2.59542303242848));
#22116=CARTESIAN_POINT('',(-9.51688605890966,-5.38497483190686E-5,2.65457696757151));
#22117=CARTESIAN_POINT('',(-9.516475,1.78524650477582E-12,1.24542303242842));
#22118=CARTESIAN_POINT('Ctrl Pts',(-9.516475,2.35602277381432E-13,2.59542303242848));
#22119=CARTESIAN_POINT('Ctrl Pts',(-9.51647500000006,-0.265706620583739,
2.60790396567667));
#22120=CARTESIAN_POINT('Ctrl Pts',(-9.40727465387207,-0.529786878176942,
2.62038489892486));
#22121=CARTESIAN_POINT('Ctrl Pts',(-9.21961691907771,-0.717894780174718,
2.63286583217306));
#22122=CARTESIAN_POINT('Ctrl Pts',(-9.03195918428335,-0.906002682172494,
2.64534676542125));
#22123=CARTESIAN_POINT('Ctrl Pts',(-8.76814132834373,-1.0158354501991,2.65782769866944));
#22124=CARTESIAN_POINT('Ctrl Pts',(-8.50243547044496,-1.0164720823066,2.67030863191763));
#22125=CARTESIAN_POINT('Ctrl Pts',(-8.2367296125462,-1.01710871441409,2.68278956516582));
#22126=CARTESIAN_POINT('Ctrl Pts',(-7.97238846933326,-0.908541417082711,
2.69527049841401));
#22127=CARTESIAN_POINT('Ctrl Pts',(-7.78383148002332,-0.721334926798513,
2.7077514316622));
#22128=CARTESIAN_POINT('Ctrl Pts',(-7.59527449071338,-0.534128436514316,
2.72023236491039));
#22129=CARTESIAN_POINT('Ctrl Pts',(-7.484809931317,-0.270574496755625,2.73271329815858));
#22130=CARTESIAN_POINT('Ctrl Pts',(-7.48353667075686,-0.00487092690813021,
2.74519423140677));
#22131=CARTESIAN_POINT('Ctrl Pts',(-7.48226341019671,0.260832642939364,
2.75767516465496));
#22132=CARTESIAN_POINT('Ctrl Pts',(-7.59019703546758,0.525433154240557,
2.77015609790315));
#22133=CARTESIAN_POINT('Ctrl Pts',(-7.77695120652528,0.714438148393377,
2.78263703115134));
#22134=CARTESIAN_POINT('Ctrl Pts',(-7.96370537758299,0.903443142546197,
2.79511796439954));
#22135=CARTESIAN_POINT('Ctrl Pts',(-8.22699388814845,1.01453885915664,2.80759889764773));
#22136=CARTESIAN_POINT('Ctrl Pts',(-8.49269364459176,1.01644874085989,2.82007983089592));
#22137=CARTESIAN_POINT('Ctrl Pts',(-8.75839340103507,1.01835862256313,2.83256076414411));
#22138=CARTESIAN_POINT('Ctrl Pts',(-9.02325176140405,0.911059288978889,
2.8450416973923));
#22139=CARTESIAN_POINT('Ctrl Pts',(-9.21270367535855,0.724758509267339,
2.85752263064049));
#22140=CARTESIAN_POINT('Ctrl Pts',(-9.40215558931305,0.53845772955579,2.87000356388868));
#22141=CARTESIAN_POINT('Ctrl Pts',(-9.51388182535848,0.275436159672091,
2.88248449713687));
#22142=CARTESIAN_POINT('Ctrl Pts',(-9.51642831724057,0.00974174196398366,
2.89496543038506));
#22143=CARTESIAN_POINT('Ctrl Pts',(-9.51645943884197,0.00649459406643292,
2.89511796439953));
#22144=CARTESIAN_POINT('Ctrl Pts',(-9.516475,0.0032472970335645,2.89527049841401));
#22145=CARTESIAN_POINT('Ctrl Pts',(-9.516475,2.39462486589124E-13,2.89542303242848));
#22146=CARTESIAN_POINT('Ctrl Pts',(-9.516475,2.62546090960999E-13,2.65457696757151));
#22147=CARTESIAN_POINT('Ctrl Pts',(-9.51647500000007,-0.265706620583709,
2.6670579008197));
#22148=CARTESIAN_POINT('Ctrl Pts',(-9.40727465387209,-0.529786878176911,
2.67953883406789));
#22149=CARTESIAN_POINT('Ctrl Pts',(-9.21961691907774,-0.717894780174691,
2.69201976731608));
#22150=CARTESIAN_POINT('Ctrl Pts',(-9.03195918428338,-0.906002682172472,
2.70450070056427));
#22151=CARTESIAN_POINT('Ctrl Pts',(-8.76814132834377,-1.01583545019909,
2.71698163381246));
#22152=CARTESIAN_POINT('Ctrl Pts',(-8.50243547044501,-1.0164720823066,2.72946256706065));
#22153=CARTESIAN_POINT('Ctrl Pts',(-8.23672961254626,-1.0171087144141,2.74194350030884));
#22154=CARTESIAN_POINT('Ctrl Pts',(-7.97238846933331,-0.908541417082739,
2.75442443355703));
#22155=CARTESIAN_POINT('Ctrl Pts',(-7.78383148002337,-0.721334926798555,
2.76690536680522));
#22156=CARTESIAN_POINT('Ctrl Pts',(-7.59527449071342,-0.534128436514371,
2.77938630005341));
#22157=CARTESIAN_POINT('Ctrl Pts',(-7.48480993131702,-0.270574496755691,
2.7918672333016));
#22158=CARTESIAN_POINT('Ctrl Pts',(-7.48353667075686,-0.00487092690820049,
2.80434816654979));
#22159=CARTESIAN_POINT('Ctrl Pts',(-7.4822634101967,0.260832642939291,2.81682909979798));
#22160=CARTESIAN_POINT('Ctrl Pts',(-7.59019703546754,0.52543315424049,2.82931003304617));
#22161=CARTESIAN_POINT('Ctrl Pts',(-7.77695120652523,0.714438148393322,
2.84179096629437));
#22162=CARTESIAN_POINT('Ctrl Pts',(-7.96370537758291,0.903443142546153,
2.85427189954256));
#22163=CARTESIAN_POINT('Ctrl Pts',(-8.22699388814836,1.01453885915661,2.86675283279075));
#22164=CARTESIAN_POINT('Ctrl Pts',(-8.49269364459167,1.01644874085989,2.87923376603894));
#22165=CARTESIAN_POINT('Ctrl Pts',(-8.75839340103498,1.01835862256316,2.89171469928713));
#22166=CARTESIAN_POINT('Ctrl Pts',(-9.02325176140396,0.911059288978938,
2.90419563253532));
#22167=CARTESIAN_POINT('Ctrl Pts',(-9.21270367535848,0.724758509267409,
2.91667656578351));
#22168=CARTESIAN_POINT('Ctrl Pts',(-9.402155589313,0.538457729555879,2.9291574990317));
#22169=CARTESIAN_POINT('Ctrl Pts',(-9.51388182535845,0.275436159672194,
2.94163843227989));
#22170=CARTESIAN_POINT('Ctrl Pts',(-9.51642831724057,0.00974174196409005,
2.95411936552808));
#22171=CARTESIAN_POINT('Ctrl Pts',(-9.51645943884197,0.00649459406651043,
2.95427189954256));
#22172=CARTESIAN_POINT('Ctrl Pts',(-9.516475,0.00324729703361311,2.95442443355703));
#22173=CARTESIAN_POINT('Ctrl Pts',(-9.516475,2.59183810895373E-13,2.95457696757151));
#22174=CARTESIAN_POINT('Origin',(-8.5,0.,1.24542303242842));
#22175=CARTESIAN_POINT('',(-9.516475,2.31742068173741E-13,2.29542303242848));
#22176=CARTESIAN_POINT('',(-9.51574434509424,-0.000859751719978319,2.3545769675715));
#22177=CARTESIAN_POINT('',(-9.516475,1.78524650477582E-12,1.24542303242842));
#22178=CARTESIAN_POINT('Ctrl Pts',(-9.516475,2.28130823537082E-13,2.29542303242848));
#22179=CARTESIAN_POINT('Ctrl Pts',(-9.51647500000006,-0.265706620583739,
2.30790396567667));
#22180=CARTESIAN_POINT('Ctrl Pts',(-9.40727465387207,-0.529786878176934,
2.32038489892486));
#22181=CARTESIAN_POINT('Ctrl Pts',(-9.21961691907772,-0.717894780174708,
2.33286583217305));
#22182=CARTESIAN_POINT('Ctrl Pts',(-9.03195918428336,-0.906002682172482,
2.34534676542125));
#22183=CARTESIAN_POINT('Ctrl Pts',(-8.76814132834376,-1.0158354501991,2.35782769866944));
#22184=CARTESIAN_POINT('Ctrl Pts',(-8.502435470445,-1.0164720823066,2.37030863191763));
#22185=CARTESIAN_POINT('Ctrl Pts',(-8.23672961254625,-1.0171087144141,2.38278956516582));
#22186=CARTESIAN_POINT('Ctrl Pts',(-7.97238846933331,-0.908541417082736,
2.39527049841401));
#22187=CARTESIAN_POINT('Ctrl Pts',(-7.78383148002336,-0.721334926798554,
2.4077514316622));
#22188=CARTESIAN_POINT('Ctrl Pts',(-7.59527449071342,-0.534128436514372,
2.42023236491039));
#22189=CARTESIAN_POINT('Ctrl Pts',(-7.48480993131702,-0.270574496755696,
2.43271329815858));
#22190=CARTESIAN_POINT('Ctrl Pts',(-7.48353667075686,-0.00487092690820941,
2.44519423140677));
#22191=CARTESIAN_POINT('Ctrl Pts',(-7.48226341019669,0.260832642939278,
2.45767516465496));
#22192=CARTESIAN_POINT('Ctrl Pts',(-7.59019703546754,0.525433154240472,
2.47015609790315));
#22193=CARTESIAN_POINT('Ctrl Pts',(-7.77695120652521,0.714438148393305,
2.48263703115134));
#22194=CARTESIAN_POINT('Ctrl Pts',(-7.96370537758289,0.903443142546138,
2.49511796439953));
#22195=CARTESIAN_POINT('Ctrl Pts',(-8.22699388814833,1.0145388591566,2.50759889764772));
#22196=CARTESIAN_POINT('Ctrl Pts',(-8.49269364459163,1.01644874085989,2.52007983089591));
#22197=CARTESIAN_POINT('Ctrl Pts',(-8.75839340103494,1.01835862256317,2.5325607641441));
#22198=CARTESIAN_POINT('Ctrl Pts',(-9.02325176140392,0.911059288978959,
2.54504169739229));
#22199=CARTESIAN_POINT('Ctrl Pts',(-9.21270367535845,0.72475850926744,2.55752263064048));
#22200=CARTESIAN_POINT('Ctrl Pts',(-9.40215558931297,0.538457729555922,
2.57000356388867));
#22201=CARTESIAN_POINT('Ctrl Pts',(-9.51388182535844,0.275436159672246,
2.58248449713686));
#22202=CARTESIAN_POINT('Ctrl Pts',(-9.51642831724057,0.00974174196414591,
2.59496543038505));
#22203=CARTESIAN_POINT('Ctrl Pts',(-9.51645943884197,0.00649459406653981,
2.59511796439953));
#22204=CARTESIAN_POINT('Ctrl Pts',(-9.516475,0.00324729703361602,2.59527049841401));
#22205=CARTESIAN_POINT('Ctrl Pts',(-9.516475,2.35602277381432E-13,2.59542303242848));
#22206=CARTESIAN_POINT('Ctrl Pts',(-9.51574434509424,-0.000859751719978263,
2.35457696757151));
#22207=CARTESIAN_POINT('Ctrl Pts',(-9.51653441684081,-0.102971653508649,
2.35936745159258));
#22208=CARTESIAN_POINT('Ctrl Pts',(-9.45523207179823,-0.543196375581154,
2.38006527676528));
#22209=CARTESIAN_POINT('Ctrl Pts',(-8.8216302613637,-1.1587255804458,2.41667044308961));
#22210=CARTESIAN_POINT('Ctrl Pts',(-7.69804845902684,-0.896211681489087,
2.46439246654446));
#22211=CARTESIAN_POINT('Ctrl Pts',(-7.3785660134251,0.00764272958311676,
2.50416081942352));
#22212=CARTESIAN_POINT('Ctrl Pts',(-7.66367275817319,0.645880124738109,
2.53597550172676));
#22213=CARTESIAN_POINT('Ctrl Pts',(-8.2091023256041,1.0830742068233,2.56779018403));
#22214=CARTESIAN_POINT('Ctrl Pts',(-9.15872944113482,1.00294500423365,2.60732400597825));
#22215=CARTESIAN_POINT('Ctrl Pts',(-9.51774253405965,0.331986183950199,
2.63890415735069));
#22216=CARTESIAN_POINT('Ctrl Pts',(-9.51822696116145,-0.000229511307854096,
2.65457696757151));
#22217=CARTESIAN_POINT('Origin',(-8.5,0.,1.24542303242842));
#22218=CARTESIAN_POINT('',(-9.51753882530083,0.000269776910017053,1.99542303242848));
#22219=CARTESIAN_POINT('',(-9.51515984464674,0.00043457310919498,2.05457696757151));
#22220=CARTESIAN_POINT('',(-9.516475,1.78524650477582E-12,1.24542303242842));
#22221=CARTESIAN_POINT('Ctrl Pts',(-9.51753882530083,0.000269776910017103,
1.99542303242848));
#22222=CARTESIAN_POINT('Ctrl Pts',(-9.51701027049666,-0.136447844912708,
2.00186505680128));
#22223=CARTESIAN_POINT('Ctrl Pts',(-9.45149622815346,-0.44263766423451,
2.01626075174989));
#22224=CARTESIAN_POINT('Ctrl Pts',(-9.05259577107697,-0.975943072842501,
2.04656378785012));
#22225=CARTESIAN_POINT('Ctrl Pts',(-8.10737674978987,-1.1367365362355,2.08633214072917));
#22226=CARTESIAN_POINT('Ctrl Pts',(-7.33160128421964,-0.283165032011243,
2.13405416418404));
#22227=CARTESIAN_POINT('Ctrl Pts',(-7.62947585871493,0.829120622165689,
2.1817761876389));
#22228=CARTESIAN_POINT('Ctrl Pts',(-8.72792114609409,1.18088449447148,2.22949821109376));
#22229=CARTESIAN_POINT('Ctrl Pts',(-9.43137564348633,0.598121868949659,
2.26738049269029));
#22230=CARTESIAN_POINT('Ctrl Pts',(-9.51633032956077,0.129919845406597,
2.2893554331352));
#22231=CARTESIAN_POINT('Ctrl Pts',(-9.51583204610243,0.000442755438962029,
2.29542303242848));
#22232=CARTESIAN_POINT('Ctrl Pts',(-9.51515984464673,0.000434573109195022,
2.05457696757151));
#22233=CARTESIAN_POINT('Ctrl Pts',(-9.51434573427704,-0.199152432567874,
2.06392340468286));
#22234=CARTESIAN_POINT('Ctrl Pts',(-9.36064838525821,-0.739560899199373,
2.08917718294584));
#22235=CARTESIAN_POINT('Ctrl Pts',(-8.48010907733479,-1.20251427821691,
2.13033830236043));
#22236=CARTESIAN_POINT('Ctrl Pts',(-7.64681002815554,-0.727926671585552,
2.17010665523948));
#22237=CARTESIAN_POINT('Ctrl Pts',(-7.44498060597373,-0.0587522064326047,
2.20192133754272));
#22238=CARTESIAN_POINT('Ctrl Pts',(-7.57134386518546,0.628757665817628,
2.23373601984597));
#22239=CARTESIAN_POINT('Ctrl Pts',(-8.34654981722532,1.19279547618219,2.27350437272501));
#22240=CARTESIAN_POINT('Ctrl Pts',(-9.31336999826338,0.815051089939519,
2.3164359121588));
#22241=CARTESIAN_POINT('Ctrl Pts',(-9.51391089471827,0.236102404612829,
2.34346011044096));
#22242=CARTESIAN_POINT('Ctrl Pts',(-9.51574434509424,-0.000859751719978263,
2.35457696757151));
#22243=CARTESIAN_POINT('Origin',(-6.3,-1.5,1.1));
#22244=CARTESIAN_POINT('',(-6.45,-1.5,1.2));
#22245=CARTESIAN_POINT('Origin',(-6.3,-1.5,1.2));
#22246=CARTESIAN_POINT('',(-6.45,-1.5,1.8));
#22247=CARTESIAN_POINT('',(-6.45,-1.5,1.1));
#22248=CARTESIAN_POINT('Origin',(-6.3,-1.5,1.8));
#22249=CARTESIAN_POINT('Origin',(-10.7,1.5,1.1));
#22250=CARTESIAN_POINT('',(-10.85,1.5,1.2));
#22251=CARTESIAN_POINT('Origin',(-10.7,1.5,1.2));
#22252=CARTESIAN_POINT('',(-10.85,1.5,1.8));
#22253=CARTESIAN_POINT('',(-10.85,1.5,1.1));
#22254=CARTESIAN_POINT('Origin',(-10.7,1.5,1.8));
#22255=CARTESIAN_POINT('Origin',(-11.5,3.67394039744206E-16,1.1));
#22256=CARTESIAN_POINT('',(-11.83,3.26980695372343E-16,1.2));
#22257=CARTESIAN_POINT('Origin',(-11.5,3.67394039744206E-16,1.2));
#22258=CARTESIAN_POINT('',(-11.83,4.07807384116069E-16,1.8));
#22259=CARTESIAN_POINT('',(-11.83,3.26980695372343E-16,1.1));
#22260=CARTESIAN_POINT('Origin',(-11.5,3.67394039744206E-16,1.8));
#22261=CARTESIAN_POINT('Origin',(-8.5,3.,1.1));
#22262=CARTESIAN_POINT('',(-8.83,3.,1.2));
#22263=CARTESIAN_POINT('Origin',(-8.5,3.,1.2));
#22264=CARTESIAN_POINT('',(-8.83,3.,1.8));
#22265=CARTESIAN_POINT('',(-8.83,3.,1.1));
#22266=CARTESIAN_POINT('Origin',(-8.5,3.,1.8));
#22267=CARTESIAN_POINT('Origin',(-5.5,0.,1.1));
#22268=CARTESIAN_POINT('',(-5.83,-4.04133443718627E-17,1.2));
#22269=CARTESIAN_POINT('Origin',(-5.5,0.,1.2));
#22270=CARTESIAN_POINT('',(-5.83,4.04133443718627E-17,1.8));
#22271=CARTESIAN_POINT('',(-5.83,-4.04133443718627E-17,1.1));
#22272=CARTESIAN_POINT('Origin',(-5.5,0.,1.8));
#22273=CARTESIAN_POINT('Origin',(-8.5,-3.,1.1));
#22274=CARTESIAN_POINT('',(-8.83,-3.,1.2));
#22275=CARTESIAN_POINT('Origin',(-8.5,-3.,1.2));
#22276=CARTESIAN_POINT('',(-8.83,-3.,1.8));
#22277=CARTESIAN_POINT('',(-8.83,-3.,1.1));
#22278=CARTESIAN_POINT('Origin',(-8.5,-3.,1.8));
#22279=CARTESIAN_POINT('Origin',(-8.5,0.,1.8));
#22280=CARTESIAN_POINT('',(-12.3,-4.65365783675994E-16,1.8));
#22281=CARTESIAN_POINT('Origin',(-8.5,0.,1.8));
#22282=CARTESIAN_POINT('',(-9.09015970213932,-0.827606761448836,1.8));
#22283=CARTESIAN_POINT('Ctrl Pts',(-9.09015970213932,-0.827606761448836,
1.8));
#22284=CARTESIAN_POINT('Ctrl Pts',(-9.20517234022333,-0.758933651578936,
1.8));
#22285=CARTESIAN_POINT('Ctrl Pts',(-9.30543470625733,-0.668153006100454,
1.8));
#22286=CARTESIAN_POINT('Ctrl Pts',(-9.46867195483753,-0.450356182127565,
1.8));
#22287=CARTESIAN_POINT('Ctrl Pts',(-9.52880163313116,-0.3245091067028,1.8));
#22288=CARTESIAN_POINT('Ctrl Pts',(-9.59924924228391,-0.0529555869675627,
1.8));
#22289=CARTESIAN_POINT('Ctrl Pts',(-9.60735796710477,0.0905106217815908,
1.8));
#22290=CARTESIAN_POINT('Ctrl Pts',(-9.5683236154275,0.376768385137387,1.8));
#22291=CARTESIAN_POINT('Ctrl Pts',(-9.51999775237459,0.516568235234083,
1.8));
#22292=CARTESIAN_POINT('Ctrl Pts',(-9.39534294737136,0.731837239747713,
1.8));
#22293=CARTESIAN_POINT('Ctrl Pts',(-9.33251138248444,0.812979534739196,
1.8));
#22294=CARTESIAN_POINT('Ctrl Pts',(-9.18591685672465,0.958099062268399,
1.8));
#22295=CARTESIAN_POINT('Ctrl Pts',(-9.10245313248508,1.02107277613405,1.8));
#22296=CARTESIAN_POINT('Ctrl Pts',(-9.01183881116721,1.07233375495132,1.8));
#22297=CARTESIAN_POINT('',(-7.9098402978609,-0.827606761448988,1.8));
#22298=CARTESIAN_POINT('Ctrl Pts',(-7.98643053267018,1.07334645743582,1.8));
#22299=CARTESIAN_POINT('Ctrl Pts',(-7.95959869951212,1.05836761542859,1.8));
#22300=CARTESIAN_POINT('Ctrl Pts',(-7.93346058196618,1.04232411727427,1.8));
#22301=CARTESIAN_POINT('Ctrl Pts',(-7.90808767262475,1.02521683657119,1.8));
#22302=CARTESIAN_POINT('Ctrl Pts',(-7.86702659414781,0.997532057264915,
1.8));
#22303=CARTESIAN_POINT('Ctrl Pts',(-7.82796733446846,0.967063261293895,
1.8));
#22304=CARTESIAN_POINT('Ctrl Pts',(-7.79102854878543,0.934112112848264,
1.8));
#22305=CARTESIAN_POINT('Ctrl Pts',(-7.76028338488381,0.906685968729699,
1.8));
#22306=CARTESIAN_POINT('Ctrl Pts',(-7.7310076966407,0.877538967785464,1.8));
#22307=CARTESIAN_POINT('Ctrl Pts',(-7.70329177854206,0.846828311810782,
1.8));
#22308=CARTESIAN_POINT('Ctrl Pts',(-7.69029826921053,0.832430838360168,
1.8));
#22309=CARTESIAN_POINT('Ctrl Pts',(-7.67764787552771,0.817689530032765,
1.8));
#22310=CARTESIAN_POINT('Ctrl Pts',(-7.66535160389364,0.80261988762452,1.8));
#22311=CARTESIAN_POINT('Ctrl Pts',(-7.65904048382196,0.794885321773502,
1.8));
#22312=CARTESIAN_POINT('Ctrl Pts',(-7.65282266864073,0.787064257278584,
1.8));
#22313=CARTESIAN_POINT('Ctrl Pts',(-7.64669976589258,0.779158762650024,
1.8));
#22314=CARTESIAN_POINT('Ctrl Pts',(-7.64099494666391,0.771793070326609,
1.8));
#22315=CARTESIAN_POINT('Ctrl Pts',(-7.63537812199093,0.764361279600661,
1.8));
#22316=CARTESIAN_POINT('Ctrl Pts',(-7.62985175793421,0.75686774204179,1.8));
#22317=CARTESIAN_POINT('Ctrl Pts',(-7.60064975503062,0.717270946878432,
1.8));
#22318=CARTESIAN_POINT('Ctrl Pts',(-7.5739537660649,0.675931375403578,1.8));
#22319=CARTESIAN_POINT('Ctrl Pts',(-7.54988948683275,0.63313208044777,1.8));
#22320=CARTESIAN_POINT('Ctrl Pts',(-7.52509818071933,0.589039738746947,
1.8));
#22321=CARTESIAN_POINT('Ctrl Pts',(-7.5030992363447,0.543396988416792,1.8));
#22322=CARTESIAN_POINT('Ctrl Pts',(-7.48408397360475,0.496493124613758,
1.8));
#22323=CARTESIAN_POINT('Ctrl Pts',(-7.47536611429351,0.47498927839399,1.8));
#22324=CARTESIAN_POINT('Ctrl Pts',(-7.46727620351496,0.453220191275412,
1.8));
#22325=CARTESIAN_POINT('Ctrl Pts',(-7.4598369859861,0.4312134286592,1.8));
#22326=CARTESIAN_POINT('Ctrl Pts',(-7.45507728472205,0.417133236026627,
1.8));
#22327=CARTESIAN_POINT('Ctrl Pts',(-7.45058400712676,0.40295574861723,1.8));
#22328=CARTESIAN_POINT('Ctrl Pts',(-7.44636373622635,0.388688247459145,
1.8));
#22329=CARTESIAN_POINT('Ctrl Pts',(-7.44358828645132,0.379305263803885,
1.8));
#22330=CARTESIAN_POINT('Ctrl Pts',(-7.44093298062382,0.369890069488065,
1.8));
#22331=CARTESIAN_POINT('Ctrl Pts',(-7.43840114103695,0.360452578629106,
1.8));
#22332=CARTESIAN_POINT('Ctrl Pts',(-7.42603564356865,0.314359899642265,
1.8));
#22333=CARTESIAN_POINT('Ctrl Pts',(-7.41659412508323,0.267678796341731,
1.8));
#22334=CARTESIAN_POINT('Ctrl Pts',(-7.41022570586029,0.220657430426334,
1.8));
#22335=CARTESIAN_POINT('Ctrl Pts',(-7.40404692106448,0.175036234549352,
1.8));
#22336=CARTESIAN_POINT('Ctrl Pts',(-7.40076084230852,0.129093821696145,
1.8));
#22337=CARTESIAN_POINT('Ctrl Pts',(-7.40055260530635,0.0830577787951491,
1.8));
#22338=CARTESIAN_POINT('Ctrl Pts',(-7.40050727015443,0.0730352997103088,
1.8));
#22339=CARTESIAN_POINT('Ctrl Pts',(-7.40060800915348,0.0630084152029981,
1.8));
#22340=CARTESIAN_POINT('Ctrl Pts',(-7.40085706028656,0.0529795432811744,
1.8));
#22341=CARTESIAN_POINT('Ctrl Pts',(-7.40145499029249,0.028901903587719,
1.8));
#22342=CARTESIAN_POINT('Ctrl Pts',(-7.40290759789421,0.0048126866985071,
1.8));
#22343=CARTESIAN_POINT('Ctrl Pts',(-7.40520170800736,-0.0192454360660064,
1.8));
#22344=CARTESIAN_POINT('Ctrl Pts',(-7.4064626542103,-0.0324688634750262,
1.8));
#22345=CARTESIAN_POINT('Ctrl Pts',(-7.40797894405252,-0.0456892794148736,
1.8));
#22346=CARTESIAN_POINT('Ctrl Pts',(-7.40974342485787,-0.0588641207172785,
1.8));
#22347=CARTESIAN_POINT('Ctrl Pts',(-7.41592575380453,-0.105025689890607,
1.8));
#22348=CARTESIAN_POINT('Ctrl Pts',(-7.42515413053941,-0.15069465683366,
1.8));
#22349=CARTESIAN_POINT('Ctrl Pts',(-7.43727039345037,-0.195579452638668,
1.8));
#22350=CARTESIAN_POINT('Ctrl Pts',(-7.44982841714008,-0.24210075488916,
1.8));
#22351=CARTESIAN_POINT('Ctrl Pts',(-7.46548913747226,-0.28778107330993,
1.8));
#22352=CARTESIAN_POINT('Ctrl Pts',(-7.4841298525239,-0.332272113546041,
1.8));
#22353=CARTESIAN_POINT('Ctrl Pts',(-7.49345021004971,-0.354517633664097,
1.8));
#22354=CARTESIAN_POINT('Ctrl Pts',(-7.50351634802847,-0.376465335519361,
1.8));
#22355=CARTESIAN_POINT('Ctrl Pts',(-7.51431717419396,-0.398067850985725,
1.8));
#22356=CARTESIAN_POINT('Ctrl Pts',(-7.51944823894934,-0.408330390539524,
1.8));
#22357=CARTESIAN_POINT('Ctrl Pts',(-7.52474514890817,-0.418514983219543,
1.8));
#22358=CARTESIAN_POINT('Ctrl Pts',(-7.53020690911777,-0.428616292379385,
1.8));
#22359=CARTESIAN_POINT('Ctrl Pts',(-7.53477770122808,-0.437069791332064,
1.8));
#22360=CARTESIAN_POINT('Ctrl Pts',(-7.53946374370851,-0.445464327647487,
1.8));
#22361=CARTESIAN_POINT('Ctrl Pts',(-7.5442575312461,-0.453785376671825,
1.8));
#22362=CARTESIAN_POINT('Ctrl Pts',(-7.54579335776759,-0.456451261982339,
1.8));
#22363=CARTESIAN_POINT('Ctrl Pts',(-7.54734041244253,-0.459109920914666,
1.8));
#22364=CARTESIAN_POINT('Ctrl Pts',(-7.54889865802203,-0.46176126431195,
1.8));
#22365=CARTESIAN_POINT('Ctrl Pts',(-7.57089648080573,-0.499190398050156,
1.8));
#22366=CARTESIAN_POINT('Ctrl Pts',(-7.59512201376794,-0.535163961610055,
1.8));
#22367=CARTESIAN_POINT('Ctrl Pts',(-7.62143687104016,-0.569509970333361,
1.8));
#22368=CARTESIAN_POINT('Ctrl Pts',(-7.64356266939663,-0.598388442122134,
1.8));
#22369=CARTESIAN_POINT('Ctrl Pts',(-7.66716630710452,-0.626116038796084,
1.8));
#22370=CARTESIAN_POINT('Ctrl Pts',(-7.69217958561781,-0.652572448486006,
1.8));
#22371=CARTESIAN_POINT('Ctrl Pts',(-7.69935390340502,-0.660160685690626,
1.8));
#22372=CARTESIAN_POINT('Ctrl Pts',(-7.70664357687587,-0.667643328511889,
1.8));
#22373=CARTESIAN_POINT('Ctrl Pts',(-7.71403777996775,-0.675008595727681,
1.8));
#22374=CARTESIAN_POINT('Ctrl Pts',(-7.74554705316012,-0.706394563079876,
1.8));
#22375=CARTESIAN_POINT('Ctrl Pts',(-7.77899495328555,-0.735698182477585,
1.8));
#22376=CARTESIAN_POINT('Ctrl Pts',(-7.81424354574822,-0.762712471628142,
1.8));
#22377=CARTESIAN_POINT('Ctrl Pts',(-7.8447822258534,-0.786117114962801,
1.8));
#22378=CARTESIAN_POINT('Ctrl Pts',(-7.87667330535679,-0.807803020240834,
1.8));
#22379=CARTESIAN_POINT('Ctrl Pts',(-7.90984029786111,-0.827606761449139,
1.8));
#22380=CARTESIAN_POINT('Origin',(-8.5,0.,1.8));
#22381=CARTESIAN_POINT('Origin',(-8.5,0.,1.2));
#22382=CARTESIAN_POINT('',(-12.3,-4.65365783675994E-16,1.2));
#22383=CARTESIAN_POINT('',(-12.3,-4.65365783675994E-16,1.2));
#22384=CARTESIAN_POINT('Origin',(-8.5,0.,1.2));
#22385=CARTESIAN_POINT('Origin',(-8.5,0.,1.2));
#22386=CARTESIAN_POINT('Ctrl Pts',(-8.9378559242407,0.917335061595449,1.70084009126667));
#22387=CARTESIAN_POINT('Ctrl Pts',(-9.09066677941173,0.844396458214744,
1.70879376184248));
#22388=CARTESIAN_POINT('Ctrl Pts',(-9.35678627449763,0.62069223278216,1.7247011029941));
#22389=CARTESIAN_POINT('Ctrl Pts',(-9.62072521198725,-0.0294746800758685,
1.75651578529734));
#22390=CARTESIAN_POINT('Ctrl Pts',(-9.27358190662816,-0.920473928894871,
1.79628413817639));
#22391=CARTESIAN_POINT('Ctrl Pts',(-8.14062118033065,-1.14844262332258,
1.84400616163126));
#22392=CARTESIAN_POINT('Ctrl Pts',(-7.47631525146516,-0.457174338716646,
1.88377451451031));
#22393=CARTESIAN_POINT('Ctrl Pts',(-7.47121748055022,0.241452561832278,
1.91558919681355));
#22394=CARTESIAN_POINT('Ctrl Pts',(-7.78668186971636,0.865450294731047,
1.94740387911679));
#22395=CARTESIAN_POINT('Ctrl Pts',(-8.6897509574811,1.18756791113319,1.98717223199585));
#22396=CARTESIAN_POINT('Ctrl Pts',(-9.60167357547127,0.481303778812772,
2.0348942554507));
#22397=CARTESIAN_POINT('Ctrl Pts',(-9.50100253463832,-0.665768137047856,
2.08261627890557));
#22398=CARTESIAN_POINT('Ctrl Pts',(-8.48010907733479,-1.20251427821691,
2.13033830236043));
#22399=CARTESIAN_POINT('Ctrl Pts',(-7.64681002815554,-0.727926671585552,
2.17010665523948));
#22400=CARTESIAN_POINT('Ctrl Pts',(-7.44498060597373,-0.0587522064326047,
2.20192133754272));
#22401=CARTESIAN_POINT('Ctrl Pts',(-7.57134386518546,0.628757665817628,
2.23373601984597));
#22402=CARTESIAN_POINT('Ctrl Pts',(-8.34654981722532,1.19279547618219,2.27350437272501));
#22403=CARTESIAN_POINT('Ctrl Pts',(-9.42125191187756,0.77290076245968,2.32122639617988));
#22404=CARTESIAN_POINT('Ctrl Pts',(-9.64765465886824,-0.356262373710212,
2.36894841963474));
#22405=CARTESIAN_POINT('Ctrl Pts',(-8.8216302613637,-1.1587255804458,2.41667044308961));
#22406=CARTESIAN_POINT('Ctrl Pts',(-7.69804845902684,-0.896211681489087,
2.46439246654446));
#22407=CARTESIAN_POINT('Ctrl Pts',(-7.3785660134251,0.00764272958311676,
2.50416081942352));
#22408=CARTESIAN_POINT('Ctrl Pts',(-7.66367275817319,0.645880124738109,
2.53597550172676));
#22409=CARTESIAN_POINT('Ctrl Pts',(-8.2091023256041,1.0830742068233,2.56779018403));
#22410=CARTESIAN_POINT('Ctrl Pts',(-9.16436302069646,1.00246964476821,2.60755853690905));
#22411=CARTESIAN_POINT('Ctrl Pts',(-9.70239789912868,-0.0182544462211632,
2.65528056036392));
#22412=CARTESIAN_POINT('Ctrl Pts',(-9.1348198302806,-1.02030689992064,2.70300258381878));
#22413=CARTESIAN_POINT('Ctrl Pts',(-7.98510578295691,-1.08672813752691,
2.75072460727364));
#22414=CARTESIAN_POINT('Ctrl Pts',(-7.30714813663279,-0.153061774256481,
2.7984466307285));
#22415=CARTESIAN_POINT('Ctrl Pts',(-7.65691273858533,0.739509857623706,
2.83821498360756));
#22416=CARTESIAN_POINT('Ctrl Pts',(-8.29011032190256,1.03564052975431,2.87002966591079));
#22417=CARTESIAN_POINT('Ctrl Pts',(-8.98864043310205,1.00940649664784,2.90184434821404));
#22418=CARTESIAN_POINT('Ctrl Pts',(-9.65832142754127,0.323442379935309,
2.94161270109309));
#22419=CARTESIAN_POINT('Ctrl Pts',(-9.39737394317918,-0.800508647597189,
2.98933472454795));
#22420=CARTESIAN_POINT('Ctrl Pts',(-8.31251927971242,-1.18695969033239,
3.03705674800282));
#22421=CARTESIAN_POINT('Ctrl Pts',(-7.39958622938631,-0.484957341940189,
3.08477877145768));
#22422=CARTESIAN_POINT('Ctrl Pts',(-7.49775671720164,0.664704372277363,
3.13250079491254));
#22423=CARTESIAN_POINT('Ctrl Pts',(-8.3462581788356,1.11087101034135,3.17226914779159));
#22424=CARTESIAN_POINT('Ctrl Pts',(-9.01886800794062,0.920532984821174,
3.20408383009483));
#22425=CARTESIAN_POINT('Ctrl Pts',(-9.52996935124643,0.443659874939959,
3.23589851239807));
#22426=CARTESIAN_POINT('Ctrl Pts',(-9.58760595877808,-0.513260926890344,
3.27566686527713));
#22427=CARTESIAN_POINT('Ctrl Pts',(-8.65488608504732,-1.19252018450271,
3.32338888873198));
#22428=CARTESIAN_POINT('Ctrl Pts',(-7.58161436923836,-0.774977522330395,
3.37111091218686));
#22429=CARTESIAN_POINT('Ctrl Pts',(-7.35051106244356,0.353226941538064,
3.41883293564171));
#22430=CARTESIAN_POINT('Ctrl Pts',(-8.17695225324716,1.15843154909689,3.46655495909658));
#22431=CARTESIAN_POINT('Ctrl Pts',(-9.11055173066928,0.9406899241179,3.50632331197563));
#22432=CARTESIAN_POINT('Ctrl Pts',(-9.49468098809675,0.356671722621264,
3.53813799427887));
#22433=CARTESIAN_POINT('Ctrl Pts',(-9.56919504916044,-0.338367989045958,
3.56995267658211));
#22434=CARTESIAN_POINT('Ctrl Pts',(-8.98668980890861,-1.0997529406782,3.60972102946116));
#22435=CARTESIAN_POINT('Ctrl Pts',(-7.8368922886023,-1.00318605097734,3.65744305291603));
#22436=CARTESIAN_POINT('Ctrl Pts',(-7.29841635493286,0.01480104106276,3.70516507637089));
#22437=CARTESIAN_POINT('Ctrl Pts',(-7.86180411857744,1.01921543685616,3.75288709982575));
#22438=CARTESIAN_POINT('Ctrl Pts',(-9.01363142052853,1.08743103894989,3.80060912328061));
#22439=CARTESIAN_POINT('Ctrl Pts',(-9.57720536848709,0.311928747092948,
3.84037747615966));
#22440=CARTESIAN_POINT('Ctrl Pts',(-9.48559359232736,-0.381064635674599,
3.87219215846291));
#22441=CARTESIAN_POINT('Ctrl Pts',(-9.08719526120723,-0.955443705498223,
3.90400684076614));
#22442=CARTESIAN_POINT('Ctrl Pts',(-8.14851560934884,-1.15012269943444,
3.9437751936452));
#22443=CARTESIAN_POINT('Ctrl Pts',(-7.34215909770885,-0.324805379838734,
3.99149721710006));
#22444=CARTESIAN_POINT('Ctrl Pts',(-7.60098238778599,0.797364195232309,
4.03921924055492));
#22445=CARTESIAN_POINT('Ctrl Pts',(-8.68421342859387,1.18834317539854,4.08694126400978));
#22446=CARTESIAN_POINT('Ctrl Pts',(-9.59991868137022,0.486315119031409,
4.13466328746464));
#22447=CARTESIAN_POINT('Ctrl Pts',(-9.51872854297443,-0.468895622595936,
4.1744316403437));
#22448=CARTESIAN_POINT('Ctrl Pts',(-8.99603586570454,-0.933034514759925,
4.20624632264694));
#22449=CARTESIAN_POINT('Ctrl Pts',(-8.31894168302622,-1.10674696069834,
4.23806100495018));
#22450=CARTESIAN_POINT('Ctrl Pts',(-7.48168771599556,-0.639815280273472,
4.27782935782924));
#22451=CARTESIAN_POINT('Ctrl Pts',(-7.41186565736802,0.511915756912677,
4.32555138128409));
#22452=CARTESIAN_POINT('Ctrl Pts',(-8.34181353614544,1.19121759958566,4.37327340473896));
#22453=CARTESIAN_POINT('Ctrl Pts',(-9.41681991554689,0.778161507816451,
4.42099542819382));
#22454=CARTESIAN_POINT('Ctrl Pts',(-9.65000288969214,-0.351876191757177,
4.46871745164868));
#22455=CARTESIAN_POINT('Ctrl Pts',(-8.96362831821964,-1.02113649024273,
4.50848580452775));
#22456=CARTESIAN_POINT('Ctrl Pts',(-8.26466394876474,-1.03015626425681,
4.54030048683097));
#22457=CARTESIAN_POINT('Ctrl Pts',(-7.63895283194712,-0.718518422553337,
4.57211516913423));
#22458=CARTESIAN_POINT('Ctrl Pts',(-7.3112802984009,0.182397838956236,4.61188352201326));
#22459=CARTESIAN_POINT('Ctrl Pts',(-8.01203048267288,1.09908136184276,4.65960554546814));
#22460=CARTESIAN_POINT('Ctrl Pts',(-9.15975953510499,1.0043603351126,4.70732756892299));
#22461=CARTESIAN_POINT('Ctrl Pts',(-9.70248278234539,-0.0113687269931911,
4.75504959237786));
#22462=CARTESIAN_POINT('Ctrl Pts',(-9.13946832655052,-1.01853019590215,
4.80277161583271));
#22463=CARTESIAN_POINT('Ctrl Pts',(-8.18251236732564,-1.0755801003455,4.84253996871177));
#22464=CARTESIAN_POINT('Ctrl Pts',(-7.64801679391654,-0.625083676278862,
4.87435465101502));
#22465=CARTESIAN_POINT('Ctrl Pts',(-7.37871875701052,0.0199830748479729,
4.90616933331825));
#22466=CARTESIAN_POINT('Ctrl Pts',(-7.72036584095294,0.915693223013455,
4.94593768619731));
#22467=CARTESIAN_POINT('Ctrl Pts',(-8.85007720703,1.15045210196194,4.99365970965217));
#22468=CARTESIAN_POINT('Ctrl Pts',(-9.65607714221684,0.327884077309669,
5.04138173310702));
#22469=CARTESIAN_POINT('Ctrl Pts',(-9.40194327853509,-0.795356782894278,
5.0891037565619));
#22470=CARTESIAN_POINT('Ctrl Pts',(-8.31719720097595,-1.18865749368552,
5.13682578001674));
#22471=CARTESIAN_POINT('Ctrl Pts',(-7.55616952889954,-0.605685554543534,
5.17659413289581));
#22472=CARTESIAN_POINT('Ctrl Pts',(-7.44670579394524,0.0847130526542142,
5.20840881519905));
#22473=CARTESIAN_POINT('Ctrl Pts',(-7.66510184151263,0.748742955970089,
5.2402234975023));
#22474=CARTESIAN_POINT('Ctrl Pts',(-8.50951785842748,1.20259424204374,5.27999185038134));
#22475=CARTESIAN_POINT('Ctrl Pts',(-9.51746361785082,0.64098508261933,5.32771387383621));
#22476=CARTESIAN_POINT('Ctrl Pts',(-9.58881482009894,-0.508433490677276,
5.37543589729106));
#22477=CARTESIAN_POINT('Ctrl Pts',(-8.6617124163166,-1.19161368916257,5.42315792074593));
#22478=CARTESIAN_POINT('Ctrl Pts',(-7.58404122591754,-0.779322157266933,
5.47087994420079));
#22479=CARTESIAN_POINT('Ctrl Pts',(-7.38993777708112,0.159476676692078,
5.51064829707985));
#22480=CARTESIAN_POINT('Ctrl Pts',(-7.75886872441434,0.753212731004544,
5.54246297938308));
#22481=CARTESIAN_POINT('Ctrl Pts',(-8.35849223365174,1.1124956185188,5.57427766168633));
#22482=CARTESIAN_POINT('Ctrl Pts',(-9.29402998312747,0.903238554602481,
5.61404601456538));
#22483=CARTESIAN_POINT('Ctrl Pts',(-9.68884327202681,-0.180957907666868,
5.66176803802024));
#22484=CARTESIAN_POINT('Ctrl Pts',(-8.99076250408938,-1.09689310850663,
5.7094900614751));
#22485=CARTESIAN_POINT('Ctrl Pts',(-7.84264782508884,-1.00696683556617,
5.75721208492997));
#22486=CARTESIAN_POINT('Ctrl Pts',(-7.29740907026871,0.00992755527834371,
5.80493410838482));
#22487=CARTESIAN_POINT('Ctrl Pts',(-7.76485398692337,0.84689508713768,5.84470246126389));
#22488=CARTESIAN_POINT('Ctrl Pts',(-8.43232822981923,1.05452620513629,5.87651714356711));
#22489=CARTESIAN_POINT('Ctrl Pts',(-9.12086672212119,0.933914055212202,
5.90833182587037));
#22490=CARTESIAN_POINT('Ctrl Pts',(-9.6914577642696,0.163560070272183,5.94810017874941));
#22491=CARTESIAN_POINT('Ctrl Pts',(-9.28066972629324,-0.914685119721433,
5.99582220220428));
#22492=CARTESIAN_POINT('Ctrl Pts',(-8.15346672652938,-1.15062462049409,
6.04354422565913));
#22493=CARTESIAN_POINT('Ctrl Pts',(-7.34403805360179,-0.331430336978762,
6.091266249114));
#22494=CARTESIAN_POINT('Ctrl Pts',(-7.59703200636107,0.794337650555134,
6.13898827256886));
#22495=CARTESIAN_POINT('Ctrl Pts',(-8.49814899597688,1.12145776690186,6.17875662544791));
#22496=CARTESIAN_POINT('Ctrl Pts',(-9.1387772737736,0.841765157457189,6.21057130775116));
#22497=CARTESIAN_POINT('Ctrl Pts',(-9.58057280678224,0.300055592187788,
6.2423859900544));
#22498=CARTESIAN_POINT('Ctrl Pts',(-9.50805779789687,-0.655852862100263,
6.28215434293345));
#22499=CARTESIAN_POINT('Ctrl Pts',(-8.49192487348196,-1.20250941040904,
6.32987636638831));
#22500=CARTESIAN_POINT('Ctrl Pts',(-7.48510361843104,-0.643434271381045,
6.37759838984317));
#22501=CARTESIAN_POINT('Ctrl Pts',(-7.4089520541479,0.505676249830352,6.42532041329804));
#22502=CARTESIAN_POINT('Ctrl Pts',(-8.33684584266954,1.19151341644632,6.4730424367529));
#22503=CARTESIAN_POINT('Ctrl Pts',(-9.23234635719901,0.849317232992327,
6.51281078963195));
#22504=CARTESIAN_POINT('Ctrl Pts',(-9.53382663893441,0.218649185747603,
6.5446254719352));
#22505=CARTESIAN_POINT('Ctrl Pts',(-9.51350682430763,-0.48007797933493,
6.57644015423843));
#22506=CARTESIAN_POINT('Ctrl Pts',(-8.83323634964205,-1.15554187977027,
6.61620850711749));
#22507=CARTESIAN_POINT('Ctrl Pts',(-7.70711659122067,-0.904118349483649,
6.66393053057235));
#22508=CARTESIAN_POINT('Ctrl Pts',(-7.31149575633931,0.17742601193168,6.71165255402721));
#22509=CARTESIAN_POINT('Ctrl Pts',(-8.00574468256001,1.09626902308369,6.75937457748207));
#22510=CARTESIAN_POINT('Ctrl Pts',(-9.15619624715678,1.00783430475606,6.80709660093694));
#22511=CARTESIAN_POINT('Ctrl Pts',(-9.60952973285748,0.163140188382897,
6.84686495381599));
#22512=CARTESIAN_POINT('Ctrl Pts',(-9.42489238334033,-0.511056811947154,
6.87867963611922));
#22513=CARTESIAN_POINT('Ctrl Pts',(-8.95236299576311,-1.02617672416823,
6.91049431842248));
#22514=CARTESIAN_POINT('Ctrl Pts',(-7.99596439398607,-1.09191190509855,
6.95026267130151));
#22515=CARTESIAN_POINT('Ctrl Pts',(-7.30883370513701,-0.164975597507443,
6.99798469475639));
#22516=CARTESIAN_POINT('Ctrl Pts',(-7.71727582008019,0.911792292728067,
7.04570671821124));
#22517=CARTESIAN_POINT('Ctrl Pts',(-8.84348349583492,1.15243792799422,7.09342874166611));
#22518=CARTESIAN_POINT('Ctrl Pts',(-9.65565533900699,0.332842662605653,
7.14115076512097));
#22519=CARTESIAN_POINT('Ctrl Pts',(-9.44582473222385,-0.602566614636137,
7.18091911800003));
#22520=CARTESIAN_POINT('Ctrl Pts',(-8.86507923315232,-0.991626007786943,
7.21273380030326));
#22521=CARTESIAN_POINT('Ctrl Pts',(-8.17069521096301,-1.07202113089142,
7.24454848260651));
#22522=CARTESIAN_POINT('Ctrl Pts',(-7.40440644892101,-0.495982128165813,
7.28431683548555));
#22523=CARTESIAN_POINT('Ctrl Pts',(-7.49123647716817,0.654591662637485,
7.33203885894042));
#22524=CARTESIAN_POINT('Ctrl Pts',(-8.50462872339795,1.20166588610525,7.37976088239528));
#22525=CARTESIAN_POINT('Ctrl Pts',(-9.51377638599174,0.646800996440254,
7.42748290585015));
#22526=CARTESIAN_POINT('Ctrl Pts',(-9.59174012789106,-0.5044075671302,7.475204929305));
#22527=CARTESIAN_POINT('Ctrl Pts',(-8.82103645592899,-1.07452619471326,
7.51497328218406));
#22528=CARTESIAN_POINT('Ctrl Pts',(-8.12729238132298,-0.98878411029843,
7.5467879644873));
#22529=CARTESIAN_POINT('Ctrl Pts',(-7.54956132387895,-0.595262355683333,
7.57860264679055));
#22530=CARTESIAN_POINT('Ctrl Pts',(-7.34694308408231,0.341735642390682,
7.61837099966959));
#22531=CARTESIAN_POINT('Ctrl Pts',(-8.16540476730042,1.15504983444235,7.66609302312446));
#22532=CARTESIAN_POINT('Ctrl Pts',(-9.28972515479892,0.905735340365632,
7.71381504657931));
#22533=CARTESIAN_POINT('Ctrl Pts',(-9.68986002054785,-0.174147125421056,
7.76153707003418));
#22534=CARTESIAN_POINT('Ctrl Pts',(-8.99560885476197,-1.09576245770118,
7.80925909348904));
#22535=CARTESIAN_POINT('Ctrl Pts',(-8.03974503939758,-1.02266139088228,
7.84902744636809));
#22536=CARTESIAN_POINT('Ctrl Pts',(-7.57119801841753,-0.503916525633981,
7.88084212867134));
#22537=CARTESIAN_POINT('Ctrl Pts',(-7.39175997946444,0.17168286473535,7.91265681097457));
#22538=CARTESIAN_POINT('Ctrl Pts',(-7.85158730821006,1.01285955677552,7.95242516385363));
#22539=CARTESIAN_POINT('Ctrl Pts',(-9.00268601129995,1.09242888273514,8.00014718730849));
#22540=CARTESIAN_POINT('Ctrl Pts',(-9.68983581786349,0.168264831258786,
8.04786921076336));
#22541=CARTESIAN_POINT('Ctrl Pts',(-9.28589479704269,-0.91019968016463,
8.09559123421821));
#22542=CARTESIAN_POINT('Ctrl Pts',(-8.15787155631456,-1.15294042718917,
8.14331325767308));
#22543=CARTESIAN_POINT('Ctrl Pts',(-7.48282485956976,-0.472255950572485,
8.18308161055214));
#22544=CARTESIAN_POINT('Ctrl Pts',(-7.4678884532851,0.226607018726978,8.21489629285537));
#22545=CARTESIAN_POINT('Ctrl Pts',(-7.77421828515018,0.854933828755218,
8.24671097515861));
#22546=CARTESIAN_POINT('Ctrl Pts',(-8.67232841342475,1.19022116371383,8.28647932803768));
#22547=CARTESIAN_POINT('Ctrl Pts',(-9.59491116316883,0.497256105602345,
8.33420135149252));
#22548=CARTESIAN_POINT('Ctrl Pts',(-9.5099094215147,-0.651233665626483,
8.3819233749474));
#22549=CARTESIAN_POINT('Ctrl Pts',(-8.49881107916957,-1.202535935537,8.42964539840226));
#22550=CARTESIAN_POINT('Ctrl Pts',(-7.48691960206137,-0.648067595192266,
8.4773674218571));
#22551=CARTESIAN_POINT('Ctrl Pts',(-7.42177080556001,0.30837112935176,8.51713577473619));
#22552=CARTESIAN_POINT('Ctrl Pts',(-7.86772641284064,0.846661146373908,
8.54895045703939));
#22553=CARTESIAN_POINT('Ctrl Pts',(-8.51049035685063,1.12141022894102,8.58076513934267));
#22554=CARTESIAN_POINT('Ctrl Pts',(-9.40906056154167,0.787357857695821,
8.62053349222169));
#22555=CARTESIAN_POINT('Ctrl Pts',(-9.65337439438576,-0.340325720693924,
8.66825551567658));
#22556=CARTESIAN_POINT('Ctrl Pts',(-8.83765888906691,-1.15326007541383,
8.71597753913143));
#22557=CARTESIAN_POINT('Ctrl Pts',(-7.71230695230558,-0.908643908472651,
8.76369956258628));
#22558=CARTESIAN_POINT('Ctrl Pts',(-7.30983761385512,0.172733885592004,
8.81142158604117));
#22559=CARTESIAN_POINT('Ctrl Pts',(-7.88634632323323,0.938669331634422,
8.85118993892019));
#22560=CARTESIAN_POINT('Ctrl Pts',(-8.57579354715678,1.05397358790813,8.88300462122346));
#22561=CARTESIAN_POINT('Ctrl Pts',(-9.24164844925372,0.841206589893327,
8.91481930352667));
#22562=CARTESIAN_POINT('Ctrl Pts',(-9.70263172305109,0.000662824957779389,
8.95458765640575));
#22563=CARTESIAN_POINT('Ctrl Pts',(-9.14957526799147,-1.01200101828229,
9.00230967986059));
#22564=CARTESIAN_POINT('Ctrl Pts',(-8.00080189061878,-1.09307985732958,
9.05003170331546));
#22565=CARTESIAN_POINT('Ctrl Pts',(-7.30979795505992,-0.171794010404939,
9.09775372677033));
#22566=CARTESIAN_POINT('Ctrl Pts',(-7.71295188493065,0.909328744289747,
9.14547575022519));
#22567=CARTESIAN_POINT('Ctrl Pts',(-8.65007393300695,1.11137246852359,9.18524410310424));
#22568=CARTESIAN_POINT('Ctrl Pts',(-9.246911830585,0.747480904860254,9.21705878540749));
#22569=CARTESIAN_POINT('Ctrl Pts',(-9.61125784799244,0.150920324793055,
9.24887346771071));
#22570=CARTESIAN_POINT('Ctrl Pts',(-9.40992790634683,-0.786355330545322,
9.28864182058978));
#22571=CARTESIAN_POINT('Ctrl Pts',(-8.32911251233276,-1.19033254023796,
9.33636384404463));
#22572=CARTESIAN_POINT('Ctrl Pts',(-7.40730065527932,-0.500030468028132,
9.3840858674995));
#22573=CARTESIAN_POINT('Ctrl Pts',(-7.48750455049532,0.648804326837381,
9.43180789095436));
#22574=CARTESIAN_POINT('Ctrl Pts',(-8.49974688525287,1.20263187907136,9.47952991440923));
#22575=CARTESIAN_POINT('Ctrl Pts',(-9.34064149709282,0.742288907721195,
9.51929826728827));
#22576=CARTESIAN_POINT('Ctrl Pts',(-9.55391555690441,0.0765962447736241,
9.55111294959152));
#22577=CARTESIAN_POINT('Ctrl Pts',(-9.4391364257873,-0.612938596369855,
9.58292763189476));
#22578=CARTESIAN_POINT('Ctrl Pts',(-8.67364027820268,-1.19003048465638,
9.62269598477381));
#22579=CARTESIAN_POINT('Ctrl Pts',(-7.59195627203432,-0.78838485392146,
9.67041800822867));
#22580=CARTESIAN_POINT('Ctrl Pts',(-7.34648309378723,0.336780453694595,
9.71814003168354));
#22581=CARTESIAN_POINT('Ctrl Pts',(-8.1587959535008,1.15311486350804,9.76586205513838));
#22582=CARTESIAN_POINT('Ctrl Pts',(-9.28666527733334,0.909659959580418,
9.81358407859327));
#22583=CARTESIAN_POINT('Ctrl Pts',(-9.62140191411355,0.0113444340048612,
9.85335243147231));
#22584=CARTESIAN_POINT('Ctrl Pts',(-9.34714244837062,-0.63162857595835,
9.88516711377556));
#22585=CARTESIAN_POINT('Ctrl Pts',(-8.80919223289119,-1.07799402237682,
9.91698179607879));
#22586=CARTESIAN_POINT('Ctrl Pts',(-7.85270416759372,-1.01357368058532,
9.95675014895785));
#22587=CARTESIAN_POINT('Ctrl Pts',(-7.29746531872796,-0.00210478704529599,
10.0044721724127));
#22588=CARTESIAN_POINT('Ctrl Pts',(-7.84799736347558,1.00941314082721,10.0521941958676));
#22589=CARTESIAN_POINT('Ctrl Pts',(-8.99642206321121,1.09528956214679,10.0999162193224));
#22590=CARTESIAN_POINT('Ctrl Pts',(-9.69008957102098,0.173234850918763,
10.1476382427773));
#22591=CARTESIAN_POINT('Ctrl Pts',(-9.35548634532394,-0.725130375949533,
10.1874065956563));
#22592=CARTESIAN_POINT('Ctrl Pts',(-8.72739302219708,-1.03193866060664,
10.2192212779596));
#22593=CARTESIAN_POINT('Ctrl Pts',(-8.02851887983101,-1.01753452151983,
10.2510359602628));
#22594=CARTESIAN_POINT('Ctrl Pts',(-7.34732047653931,-0.343006438452994,
10.2908043131419));
#22595=CARTESIAN_POINT('Ctrl Pts',(-7.58920203641245,0.7852013495374,10.3385263365967));
#22596=CARTESIAN_POINT('Ctrl Pts',(-8.66735858846781,1.18996362540016,10.3862483600516));
#22597=CARTESIAN_POINT('Ctrl Pts',(-9.59204571388488,0.503517873144797,
10.4339703835065));
#22598=CARTESIAN_POINT('Ctrl Pts',(-9.51335310231618,-0.647641097099265,
10.4816924069613));
#22599=CARTESIAN_POINT('Ctrl Pts',(-8.67252686454233,-1.10810894327751,
10.5214607598404));
#22600=CARTESIAN_POINT('Ctrl Pts',(-7.99679100783777,-0.929185501396585,
10.5532754421436));
#22601=CARTESIAN_POINT('Ctrl Pts',(-7.47768944170931,-0.461033698950278,
10.5850901244469));
#22602=CARTESIAN_POINT('Ctrl Pts',(-7.40386039813483,0.494774164491896,
10.6248584773259));
#22603=CARTESIAN_POINT('Ctrl Pts',(-8.32494671266358,1.18972704280574,10.6725805007808));
#22604=CARTESIAN_POINT('Ctrl Pts',(-9.40513361302378,0.790414745234386,
10.7203025242356));
#22605=CARTESIAN_POINT('Ctrl Pts',(-9.65530433140282,-0.333715435112715,
10.7680245476905));
#22606=CARTESIAN_POINT('Ctrl Pts',(-8.84261372599144,-1.15279631131785,
10.8157465711454));
#22607=CARTESIAN_POINT('Ctrl Pts',(-7.90546168306107,-0.950891759798041,
10.8555149240244));
#22608=CARTESIAN_POINT('Ctrl Pts',(-7.51150003530626,-0.373460581051111,
10.8873296063277));
#22609=CARTESIAN_POINT('Ctrl Pts',(-7.42522961150793,0.320217990095783,
10.9191442886309));
#22610=CARTESIAN_POINT('Ctrl Pts',(-7.99476109608862,1.09135564808188,10.95891264151));
#22611=CARTESIAN_POINT('Ctrl Pts',(-9.14602870394829,1.01426870377897,11.0066346649648));
#22612=CARTESIAN_POINT('Ctrl Pts',(-9.70166201229556,0.0055439259745542,
11.0543566884197));
#22613=CARTESIAN_POINT('Ctrl Pts',(-9.15535975983058,-1.00826468498374,
11.1020787118745));
#22614=CARTESIAN_POINT('Ctrl Pts',(-8.00485243357111,-1.09597097958172,
11.1498007353294));
#22615=CARTESIAN_POINT('Ctrl Pts',(-7.42822998271092,-0.330121158365471,
11.1895690882084));
#22616=CARTESIAN_POINT('Ctrl Pts',(-7.50809623085543,0.364323892375102,
11.2213837705117));
#22617=CARTESIAN_POINT('Ctrl Pts',(-7.89671320806008,0.945365535563497,
11.2531984528149));
#22618=CARTESIAN_POINT('Ctrl Pts',(-8.83196240436717,1.15590850101232,11.292966805694));
#22619=CARTESIAN_POINT('Ctrl Pts',(-9.65217599238663,0.34436110749974,11.3406888291488));
#22620=CARTESIAN_POINT('Ctrl Pts',(-9.41238816090703,-0.782029520380217,
11.3884108526037));
#22621=CARTESIAN_POINT('Ctrl Pts',(-8.33593165763767,-1.19129159689182,
11.4361328760586));
#22622=CARTESIAN_POINT('Ctrl Pts',(-7.40847229147015,-0.504867073730658,
11.4838548995134));
#22623=CARTESIAN_POINT('Ctrl Pts',(-7.47347904807857,0.451581315409203,
11.5236232523925));
#22624=CARTESIAN_POINT('Ctrl Pts',(-7.9882389265501,0.924502887772644,11.5554379346957));
#22625=CARTESIAN_POINT('Ctrl Pts',(-8.662295109207,1.10965366069233,11.587252616999));
#22626=CARTESIAN_POINT('Ctrl Pts',(-9.50733424510565,0.6569636361803,11.627020969878));
#22627=CARTESIAN_POINT('Ctrl Pts',(-9.59664513622963,-0.493420241755894,
11.6747429933329));
#22628=CARTESIAN_POINT('Ctrl Pts',(-8.67833114031927,-1.18836876907038,
11.7224650167878));
#22629=CARTESIAN_POINT('Ctrl Pts',(-7.59648578275535,-0.793571766778151,
11.7701870402426));
#22630=CARTESIAN_POINT('Ctrl Pts',(-7.34420465835447,0.332356177701384,
11.8179090636975));
#22631=CARTESIAN_POINT('Ctrl Pts',(-8.01915026029997,1.01314089690961,11.8576774165765));
#22632=CARTESIAN_POINT('Ctrl Pts',(-8.71786174690529,1.03399286507883,11.8894920988798));
#22633=CARTESIAN_POINT('Ctrl Pts',(-9.34875922243034,0.732992995532587,
11.921306781183));
#22634=CARTESIAN_POINT('Ctrl Pts',(-9.6916373311426,-0.162246638341423,
11.9610751340621));
#22635=CARTESIAN_POINT('Ctrl Pts',(-9.00650705906901,-1.09066249999891,
12.0087971575169));
#22636=CARTESIAN_POINT('Ctrl Pts',(-7.85733887313724,-1.01538613489102,
12.0565191809718));
#22637=CARTESIAN_POINT('Ctrl Pts',(-7.29749708846947,-0.0089909705338671,
12.1042412044266));
#22638=CARTESIAN_POINT('Ctrl Pts',(-7.84337957856142,1.00755799970802,12.1519632278815));
#22639=CARTESIAN_POINT('Ctrl Pts',(-8.79923252726346,1.08080101951651,12.1917315807606));
#22640=CARTESIAN_POINT('Ctrl Pts',(-9.34127841248145,0.639418187488609,
12.2235462630638));
#22641=CARTESIAN_POINT('Ctrl Pts',(-9.62145885139695,-0.000996887084038987,
12.2553609453671));
#22642=CARTESIAN_POINT('Ctrl Pts',(-9.29502513200662,-0.902362754164655,
12.2951292982461));
#22643=CARTESIAN_POINT('Ctrl Pts',(-8.1694501543662,-1.15621403266957,12.342851321701));
#22644=CARTESIAN_POINT('Ctrl Pts',(-7.34963963733674,-0.347409503213033,
12.3905733451558));
#22645=CARTESIAN_POINT('Ctrl Pts',(-7.58472057763644,0.779972864135922,
12.4382953686107));
#22646=CARTESIAN_POINT('Ctrl Pts',(-8.66265259355083,1.19158198813047,12.4860173920655));
#22647=CARTESIAN_POINT('Ctrl Pts',(-9.43344092441323,0.621577822795351,
12.5257857449446));
#22648=CARTESIAN_POINT('Ctrl Pts',(-9.55457743897031,-0.0668686100748459,
12.5576004272478));
#22649=CARTESIAN_POINT('Ctrl Pts',(-9.34745473800569,-0.73450079386759,
12.5894151095511));
#22650=CARTESIAN_POINT('Ctrl Pts',(-8.51084346084306,-1.20258301999602,
12.6291834624301));
#22651=CARTESIAN_POINT('Ctrl Pts',(-7.49353410420185,-0.658118902923919,
12.676905485885));
#22652=CARTESIAN_POINT('Ctrl Pts',(-7.40273343869918,0.489926954106946,
12.7246275093399));
#22653=CARTESIAN_POINT('Ctrl Pts',(-8.31813670676161,1.18870510740178,12.7723495327947));
#22654=CARTESIAN_POINT('Ctrl Pts',(-9.40263354937312,0.794717670730844,
12.8200715562496));
#22655=CARTESIAN_POINT('Ctrl Pts',(-9.61260306996757,-0.140660434590392,
12.8598399091286));
#22656=CARTESIAN_POINT('Ctrl Pts',(-9.25377696749447,-0.740557404306628,
12.8916545914319));
#22657=CARTESIAN_POINT('Ctrl Pts',(-8.66032206785154,-1.10994044151937,
12.9234692737351));
#22658=CARTESIAN_POINT('Ctrl Pts',(-7.7213756745308,-0.916552050029583,
12.9632376266142));
#22659=CARTESIAN_POINT('Ctrl Pts',(-7.30826349421839,0.160804821376725,
13.010959650069));
#22660=CARTESIAN_POINT('Ctrl Pts',(-7.99073740166053,1.08842727494398,13.0586816735239));
#22661=CARTESIAN_POINT('Ctrl Pts',(-9.1402099835718,1.0179515050952,13.1064036969788));
#22662=CARTESIAN_POINT('Ctrl Pts',(-9.70258664433777,0.010433766633717,
13.1541257204336));
#22663=CARTESIAN_POINT('Ctrl Pts',(-9.24937860779893,-0.83432766425052,
13.1938940733127));
#22664=CARTESIAN_POINT('Ctrl Pts',(-8.58551523025838,-1.05322938204002,
13.2257087556159));
#22665=CARTESIAN_POINT('Ctrl Pts',(-7.89503345433145,-0.944291495133931,
13.2575234379192));
#22666=CARTESIAN_POINT('Ctrl Pts',(-7.31148207597819,-0.183708042569379,
13.2972917907982));
#22667=CARTESIAN_POINT('Ctrl Pts',(-7.70395651638576,0.901337263173938,
13.3450138142531));
#22668=CARTESIAN_POINT('Ctrl Pts',(-8.82700349925863,1.15632652757863,13.3927358377079));
#22669=CARTESIAN_POINT('Ctrl Pts',(-9.65018514507657,0.350953304352284,
13.4404578611628));
#22670=CARTESIAN_POINT('Ctrl Pts',(-9.41628673666211,-0.77893652940587,
13.4881798846177));
#22671=CARTESIAN_POINT('Ctrl Pts',(-8.52083705101177,-1.12126569842545,
13.5279482374967));
#22672=CARTESIAN_POINT('Ctrl Pts',(-7.87556538618484,-0.852459030609716,
13.5597629197999));
#22673=CARTESIAN_POINT('Ctrl Pts',(-7.42466201419345,-0.318306715986269,
13.5915776021032));
#22674=CARTESIAN_POINT('Ctrl Pts',(-7.48098307234338,0.638692415623545,
13.6313459549823));
#22675=CARTESIAN_POINT('Ctrl Pts',(-8.48771545022648,1.2024737750269,13.6790679784371));
#22676=CARTESIAN_POINT('Ctrl Pts',(-9.5038575626246,0.660524277275879,13.726790001892));
#22677=CARTESIAN_POINT('Ctrl Pts',(-9.59945268682829,-0.487132301553321,
13.7745120253468));
#22678=CARTESIAN_POINT('Ctrl Pts',(-8.68330312999737,-1.18858044034005,
13.8222340488017));
#22679=CARTESIAN_POINT('Ctrl Pts',(-7.78213757023688,-0.861594151033408,
13.8620024016807));
#22680=CARTESIAN_POINT('Ctrl Pts',(-7.47002326942581,-0.236120563005943,
13.893817083984));
#22681=CARTESIAN_POINT('Ctrl Pts',(-7.47851070073035,0.462850473304309,
13.9256317662872));
#22682=CARTESIAN_POINT('Ctrl Pts',(-8.14724805356803,1.14973456280755,13.9654001191663));
#22683=CARTESIAN_POINT('Ctrl Pts',(-9.27746302049914,0.917412307278985,
14.0131221426211));
#22684=CARTESIAN_POINT('Ctrl Pts',(-9.69133773090962,-0.157279171604172,
14.060844166076));
#22685=CARTESIAN_POINT('Ctrl Pts',(-9.01274434530469,-1.08774414553638,
14.1085661895309));
#22686=CARTESIAN_POINT('Ctrl Pts',(-7.86096046478965,-1.01879928006645,
14.1562882129857));
#22687=CARTESIAN_POINT('Ctrl Pts',(-7.39339125658958,-0.181901176928426,
14.1960565658648));
#22688=CARTESIAN_POINT('Ctrl Pts',(-7.56658796866361,0.495325110967661,
14.227871248168));
#22689=CARTESIAN_POINT('Ctrl Pts',(-8.03032863686894,1.01837113068607,14.2596859304713));
#22690=CARTESIAN_POINT('Ctrl Pts',(-8.98547726602411,1.10028874610241,14.2994542833503));
#22691=CARTESIAN_POINT('Ctrl Pts',(-9.68820253147304,0.185118432341084,
14.3471763068052));
#22692=CARTESIAN_POINT('Ctrl Pts',(-9.29804866714497,-0.898410068830433,
14.3948983302601));
#22693=CARTESIAN_POINT('Ctrl Pts',(-8.17607654062253,-1.15808794236719,
14.4426203537149));
#22694=CARTESIAN_POINT('Ctrl Pts',(-7.35014532908186,-0.352360236686861,
14.4903423771698));
#22695=CARTESIAN_POINT('Ctrl Pts',(-7.54410935628155,0.586467412906594,
14.5301107300488));
#22696=CARTESIAN_POINT('Ctrl Pts',(-8.11818483430833,0.985303082841334,
14.5619254123521));
#22697=CARTESIAN_POINT('Ctrl Pts',(-8.81110824342201,1.07744262493533,14.5937400946553));
#22698=CARTESIAN_POINT('Ctrl Pts',(-9.58703953535871,0.514459472793815,
14.6335084475343));
#22699=CARTESIAN_POINT('Ctrl Pts',(-9.5197011993494,-0.637419449003044,
14.6812304709892));
#22700=CARTESIAN_POINT('Ctrl Pts',(-8.51571617796591,-1.20157202386707,
14.7289524944441));
#22701=CARTESIAN_POINT('Ctrl Pts',(-7.49731927134888,-0.663871558339892,
14.7766745178989));
#22702=CARTESIAN_POINT('Ctrl Pts',(-7.39987670884486,0.485852082205623,
14.8243965413538));
#22703=CARTESIAN_POINT('Ctrl Pts',(-8.16081779720729,1.06893703341116,14.8641648942329));
#22704=CARTESIAN_POINT('Ctrl Pts',(-8.8559140568051,0.994952345727948,14.8959795765361));
#22705=CARTESIAN_POINT('Ctrl Pts',(-9.44022464924591,0.611267993885705,
14.9277942588393));
#22706=CARTESIAN_POINT('Ctrl Pts',(-9.65867724640615,-0.322165374756826,
14.9675626117184));
#22707=CARTESIAN_POINT('Ctrl Pts',(-8.85410231103244,-1.14921958576719,
15.0152846351732));
#22708=CARTESIAN_POINT('Ctrl Pts',(-7.72572214438401,-0.918975590321003,
15.0630066586281));
#22709=CARTESIAN_POINT('Ctrl Pts',(-7.30736222115706,0.153977788901801,
15.110728682083));
#22710=CARTESIAN_POINT('Ctrl Pts',(-7.98591084190305,1.0872147627098,15.1584507055378));
#22711=CARTESIAN_POINT('Ctrl Pts',(-8.9428753883204,1.03030690516172,15.1982190584169));
#22712=CARTESIAN_POINT('Ctrl Pts',(-9.42013743498128,0.519569006187592,
15.2300337407202));
#22713=CARTESIAN_POINT('Ctrl Pts',(-9.61098803899296,-0.152895867268804,
15.2618484230234));
#22714=CARTESIAN_POINT('Ctrl Pts',(-9.1654669503698,-1.00173643888712,15.3016167759024));
#22715=CARTESIAN_POINT('Ctrl Pts',(-8.01588181111314,-1.10078331455882,
15.3493387993573));
#22716=CARTESIAN_POINT('Ctrl Pts',(-7.31318175323431,-0.188383730563224,
15.3970608228122));
#22717=CARTESIAN_POINT('Ctrl Pts',(-7.69881132927115,0.896762228213724,
15.444782846267));
#22718=CARTESIAN_POINT('Ctrl Pts',(-8.82255375228613,1.15857095575389,15.4925048697219));
#22719=CARTESIAN_POINT('Ctrl Pts',(-9.50904512931535,0.489402906826901,
15.5322732226009));
#22720=CARTESIAN_POINT('Ctrl Pts',(-9.53578529193268,-0.209092634933555,
15.5640879049042));
#22721=CARTESIAN_POINT('Ctrl Pts',(-9.2401877616229,-0.842543822232629,
15.5959025872074));
#22722=CARTESIAN_POINT('Ctrl Pts',(-8.34777029430052,-1.19292557033953,
15.6356709400864));
#22723=CARTESIAN_POINT('Ctrl Pts',(-7.41379258935603,-0.515793056893565,
15.6833929635413));
#22724=CARTESIAN_POINT('Ctrl Pts',(-7.47897580231666,0.634172756274122,
15.7311149869962));
#22725=CARTESIAN_POINT('Ctrl Pts',(-8.48126958185156,1.2021390181908,15.7788370104511));
#22726=CARTESIAN_POINT('Ctrl Pts',(-9.50111792497817,0.665597216139478,
15.8265590339059));
#22727=CARTESIAN_POINT('Ctrl Pts',(-9.60129174604384,-0.482092567813502,
15.8742810573608));
#22728=CARTESIAN_POINT('Ctrl Pts',(-8.68981880352144,-1.18720590861504,
15.9220030808156));
#22729=CARTESIAN_POINT('Ctrl Pts',(-7.60428317324231,-0.801471685911831,
15.9697251042705));
#22730=CARTESIAN_POINT('Ctrl Pts',(-7.34085844261802,0.319812236206833,
16.0174471277253));
#22731=CARTESIAN_POINT('Ctrl Pts',(-8.14340243192267,1.1485135933495,16.0651691511802));
#22732=CARTESIAN_POINT('Ctrl Pts',(-9.08302755349385,0.958038040322845,
16.1049375040593));
#22733=CARTESIAN_POINT('Ctrl Pts',(-9.48389821835483,0.385376694788,16.1367521863625));
#22734=CARTESIAN_POINT('Ctrl Pts',(-9.57857408885389,-0.307189213773236,
16.1685668686657));
#22735=CARTESIAN_POINT('Ctrl Pts',(-9.01839426272804,-1.08517048015552,
16.2083352215448));
#22736=CARTESIAN_POINT('Ctrl Pts',(-7.86628709111648,-1.02200475985657,
16.2560572449997));
#22737=CARTESIAN_POINT('Ctrl Pts',(-7.29849140255546,-0.0200766297914018,
16.3037792684545));
#22738=CARTESIAN_POINT('Ctrl Pts',(-7.83249587692306,1.00026625060406,16.3515012919094));
#22739=CARTESIAN_POINT('Ctrl Pts',(-8.98185711668004,1.10187833907993,16.3992233153643));
#22740=CARTESIAN_POINT('Ctrl Pts',(-9.56769966619584,0.343058292158321,
16.4389916682433));
#22741=CARTESIAN_POINT('Ctrl Pts',(-9.49623696904437,-0.352302076283959,
16.4708063505465));
#22742=CARTESIAN_POINT('Ctrl Pts',(-9.11467520479983,-0.938000704161855,
16.5026210328498));
#22743=CARTESIAN_POINT('Ctrl Pts',(-8.18204041706793,-1.15983848287103,
16.5423893857288));
#22744=CARTESIAN_POINT('Ctrl Pts',(-7.35207269505694,-0.358269358953146,
16.5901114091837));
#22745=CARTESIAN_POINT('Ctrl Pts',(-7.57822133797448,0.770938669115475,
16.6378334326386));
#22746=CARTESIAN_POINT('Ctrl Pts',(-8.64964987006652,1.19318859338267,16.6855554560934));
#22747=CARTESIAN_POINT('Ctrl Pts',(-9.58534244846187,0.518030172478724,
16.7332774795483));
#22748=CARTESIAN_POINT('Ctrl Pts',(-9.53190693470597,-0.439134409383287,
16.7730458324274));
#22749=CARTESIAN_POINT('Ctrl Pts',(-9.02290381225217,-0.918246475208663,
16.8048605147306));
#22750=CARTESIAN_POINT('Ctrl Pts',(-8.35113597915327,-1.11153517775485,
16.8366751970339));
#22751=CARTESIAN_POINT('Ctrl Pts',(-7.50068418268081,-0.669097450885376,
16.8764435499128));
#22752=CARTESIAN_POINT('Ctrl Pts',(-7.39746804575687,0.480122254695365,
16.9241655733678));
#22753=CARTESIAN_POINT('Ctrl Pts',(-8.30731076557255,1.18612528247467,16.9718875968226));
#22754=CARTESIAN_POINT('Ctrl Pts',(-9.39385135696734,0.804440079539564,
17.0196096202775));
#22755=CARTESIAN_POINT('Ctrl Pts',(-9.65973006081727,-0.318354655403303,
17.0673316437323));
#22756=CARTESIAN_POINT('Ctrl Pts',(-8.99306665327201,-1.00725181786075,
17.1070999966114));
#22757=CARTESIAN_POINT('Ctrl Pts',(-8.29465842608819,-1.03655189152894,
17.1389146789146));
#22758=CARTESIAN_POINT('Ctrl Pts',(-7.66016704512213,-0.743203577124704,
17.1707293612179));
#22759=CARTESIAN_POINT('Ctrl Pts',(-7.30648773259623,0.147824112332773,
17.2104977140969));
#22760=CARTESIAN_POINT('Ctrl Pts',(-7.9803404223588,1.08445747411188,17.2582197375518));
#22761=CARTESIAN_POINT('Ctrl Pts',(-9.13033490461218,1.02308368911607,17.3059417610066));
#22762=CARTESIAN_POINT('Ctrl Pts',(-9.7023062493245,0.0235323740106206,
17.3536637844615));
#22763=CARTESIAN_POINT('Ctrl Pts',(-9.16875696690466,-0.99954370581896,
17.4013858079164));
#22764=CARTESIAN_POINT('Ctrl Pts',(-8.21385965450184,-1.08434065304146,
17.4411541607954));
#22765=CARTESIAN_POINT('Ctrl Pts',(-7.66651569284325,-0.649545145099307,
17.4729688430987));
#22766=CARTESIAN_POINT('Ctrl Pts',(-7.37861109970015,-0.0125651679117135,
17.5047835254019));
#22767=CARTESIAN_POINT('Ctrl Pts',(-7.69412058637172,0.892682402266311,
17.544551878281));
#22768=CARTESIAN_POINT('Ctrl Pts',(-8.81654339210534,1.16012687698589,17.5922739017358));
#22769=CARTESIAN_POINT('Ctrl Pts',(-9.64607496368117,0.361295591631848,
17.6399959251907));
#22770=CARTESIAN_POINT('Ctrl Pts',(-9.42464482979018,-0.768847207534023,
17.6877179486456));
#22771=CARTESIAN_POINT('Ctrl Pts',(-8.35176929286965,-1.19346183771808,
17.7354399721004));
#22772=CARTESIAN_POINT('Ctrl Pts',(-7.57414417389279,-0.632820621048115,
17.7752083249795));
#22773=CARTESIAN_POINT('Ctrl Pts',(-7.44469102409625,0.0541105458809273,
17.8070230072827));
#22774=CARTESIAN_POINT('Ctrl Pts',(-7.64372479594433,0.724198677214912,
17.8388376895859));
#22775=CARTESIAN_POINT('Ctrl Pts',(-8.47461430237912,1.20236394946876,17.878606042465));
#22776=CARTESIAN_POINT('Ctrl Pts',(-9.49843356039162,0.670242131825755,
17.9263280659198));
#22777=CARTESIAN_POINT('Ctrl Pts',(-9.60311108913075,-0.476621707380359,
17.9740500893747));
#22778=CARTESIAN_POINT('Ctrl Pts',(-8.69622519637391,-1.18641888138153,
18.0217721128296));
#22779=CARTESIAN_POINT('Ctrl Pts',(-7.60704310414848,-0.80557524960553,
18.0694941362844));
#22780=CARTESIAN_POINT('Ctrl Pts',(-7.38577725982833,0.127195261093777,
18.1092624891635));
#22781=CARTESIAN_POINT('Ctrl Pts',(-7.73732247271078,0.731387705096654,
18.1410771714667));
#22782=CARTESIAN_POINT('Ctrl Pts',(-8.3262669675734,1.10792047666078,18.17289185377));
#22783=CARTESIAN_POINT('Ctrl Pts',(-9.26748337738822,0.92590105630058,18.212660206649));
#22784=CARTESIAN_POINT('Ctrl Pts',(-9.69359399866432,-0.146381201467666,
18.2603822301039));
#22785=CARTESIAN_POINT('Ctrl Pts',(-9.02238788447832,-1.0821890893276,18.3081042535587));
#22786=CARTESIAN_POINT('Ctrl Pts',(-7.87214708287262,-1.02561922965847,
18.3558262770137));
#22787=CARTESIAN_POINT('Ctrl Pts',(-7.2976274719566,-0.0249760772001006,
18.4035483004684));
#22788=CARTESIAN_POINT('Ctrl Pts',(-7.740586531955,0.825204298166379,18.4433166533476));
#22789=CARTESIAN_POINT('Ctrl Pts',(-8.40175415087621,1.05211821528215,18.4751313356508));
#22790=CARTESIAN_POINT('Ctrl Pts',(-9.09350283873543,0.951538401523235,
18.506946017954));
#22791=CARTESIAN_POINT('Ctrl Pts',(-9.68620940283924,0.198067547169027,
18.5467143708331));
#22792=CARTESIAN_POINT('Ctrl Pts',(-9.30688528934162,-0.891644671174926,
18.5944363942879));
#22793=CARTESIAN_POINT('Ctrl Pts',(-8.18700405536254,-1.16019647713218,
18.6421584177428));
#22794=CARTESIAN_POINT('Ctrl Pts',(-7.35414309684935,-0.364837014696453,
18.6898804411976));
#22795=CARTESIAN_POINT('Ctrl Pts',(-7.5743604621335,0.767798766972237,18.7376024646525));
#22796=CARTESIAN_POINT('Ctrl Pts',(-8.46560482642789,1.12093172013077,18.7773708175315));
#22797=CARTESIAN_POINT('Ctrl Pts',(-9.11408002803092,0.859948082719013,
18.8091854998348));
#22798=CARTESIAN_POINT('Ctrl Pts',(-9.57141001751387,0.331287674885919,
18.841000182138));
#22799=CARTESIAN_POINT('Ctrl Pts',(-9.52666622211786,-0.626322575824964,
18.8807685350171));
#22800=CARTESIAN_POINT('Ctrl Pts',(-8.52682536005481,-1.20223728516816,
18.928490558472));
#22801=CARTESIAN_POINT('Ctrl Pts',(-7.50420367062632,-0.672615787292656,
18.9762125819268));
#22802=CARTESIAN_POINT('Ctrl Pts',(-7.39473674138445,0.47380082201821,19.0239346053817));
#22803=CARTESIAN_POINT('Ctrl Pts',(-8.3023365797739,1.18627681125878,19.0716566288366));
#22804=CARTESIAN_POINT('Ctrl Pts',(-9.20739053959603,0.870212372728869,
19.1114249817156));
#22805=CARTESIAN_POINT('Ctrl Pts',(-9.52704596967527,0.248558970814542,
19.1432396640189));
#22806=CARTESIAN_POINT('Ctrl Pts',(-9.52701192807412,-0.450463593150274,
19.175054346322));
#22807=CARTESIAN_POINT('Ctrl Pts',(-8.86663007628672,-1.14538460256273,
19.2148226992012));
#22808=CARTESIAN_POINT('Ctrl Pts',(-7.73368824589063,-0.926747206796109,
19.262544722656));
#22809=CARTESIAN_POINT('Ctrl Pts',(-7.30684738329652,0.142860631956667,
19.3102667461109));
#22810=CARTESIAN_POINT('Ctrl Pts',(-7.97413888435272,1.08146390454826,19.3579887695657));
#22811=CARTESIAN_POINT('Ctrl Pts',(-9.12667230207592,1.02645278821612,19.4057107930206));
#22812=CARTESIAN_POINT('Ctrl Pts',(-9.60432806254847,0.195270272771769,
19.4454791458997));
#22813=CARTESIAN_POINT('Ctrl Pts',(-9.43933382179755,-0.484000988661962,
19.4772938282029));
#22814=CARTESIAN_POINT('Ctrl Pts',(-8.98195234416682,-1.01261685109054,
19.5091085105061));
#22815=CARTESIAN_POINT('Ctrl Pts',(-8.02786420308556,-1.10607924214215,
19.5488768633852));
#22816=CARTESIAN_POINT('Ctrl Pts',(-7.31412302271695,-0.199474019713455,
19.59659888684));
#22817=CARTESIAN_POINT('Ctrl Pts',(-7.6911450727875,0.888693441876024,19.6443209102949));
#22818=CARTESIAN_POINT('Ctrl Pts',(-8.80989482891317,1.16192051569952,19.6920429337498));
#22819=CARTESIAN_POINT('Ctrl Pts',(-9.64550943889695,0.366239847673363,
19.7397649572046));
#22820=CARTESIAN_POINT('Ctrl Pts',(-9.46291298893969,-0.574864788356032,
19.7795333100837));
#22821=CARTESIAN_POINT('Ctrl Pts',(-8.89370267398479,-0.980613680455146,
19.8113479923869));
#22822=CARTESIAN_POINT('Ctrl Pts',(-8.20194419316234,-1.08112611899387,
19.8431626746901));
#22823=CARTESIAN_POINT('Ctrl Pts',(-7.41926139538849,-0.527567596738221,
19.8829310275693));
#22824=CARTESIAN_POINT('Ctrl Pts',(-7.47266495046468,0.625041427256538,
19.930653051024));
#22825=CARTESIAN_POINT('Ctrl Pts',(-8.46975416762413,1.20129410076522,19.978375074479));
#22826=CARTESIAN_POINT('Ctrl Pts',(-9.49457910241488,0.675948591854568,
20.0260970979338));
#22827=CARTESIAN_POINT('Ctrl Pts',(-9.60591833167572,-0.472512586381968,
20.0738191213886));
#22828=CARTESIAN_POINT('Ctrl Pts',(-8.85208422800519,-1.06475708288341,
20.1135874742677));
#22829=CARTESIAN_POINT('Ctrl Pts',(-8.15614408721544,-0.999183715360516,
20.1454021565709));
#22830=CARTESIAN_POINT('Ctrl Pts',(-7.56723626857872,-0.622593583732944,
20.1772168388742));
#22831=CARTESIAN_POINT('Ctrl Pts',(-7.33751148016779,0.308129748456874,
20.2169851917532));
#22832=CARTESIAN_POINT('Ctrl Pts',(-8.13202589224642,1.14485332938919,20.2647072152081));
#22833=CARTESIAN_POINT('Ctrl Pts',(-9.26310790487898,0.928271863421839,
20.312429238663));
#22834=CARTESIAN_POINT('Ctrl Pts',(-9.69441266856891,-0.139543781490679,
20.3601512621178));
#22835=CARTESIAN_POINT('Ctrl Pts',(-9.02719938225488,-1.08091827257006,
20.4078732855727));
#22836=CARTESIAN_POINT('Ctrl Pts',(-8.06961674413775,-1.03558737064229,
20.4476416384518));
#22837=CARTESIAN_POINT('Ctrl Pts',(-7.58621297435389,-0.530658324686794,
20.479456320755));
#22838=CARTESIAN_POINT('Ctrl Pts',(-7.38724446850424,0.13944918890389,20.5112710030583));
#22839=CARTESIAN_POINT('Ctrl Pts',(-7.82246699818582,0.993615887593619,
20.5510393559372));
#22840=CARTESIAN_POINT('Ctrl Pts',(-8.97077176781247,1.10655683650741,20.5987613793922));
#22841=CARTESIAN_POINT('Ctrl Pts',(-9.68445160636614,0.202723257388189,
20.646483402847));
#22842=CARTESIAN_POINT('Ctrl Pts',(-9.31197799098589,-0.887009488080663,
20.6942054263019));
#22843=CARTESIAN_POINT('Ctrl Pts',(-8.19147423515819,-1.16238347934517,
20.7419274497567));
#22844=CARTESIAN_POINT('Ctrl Pts',(-7.49695823929343,-0.501575692631794,
20.7816958026358));
#22845=CARTESIAN_POINT('Ctrl Pts',(-7.46174696796193,0.196559475127261,
20.813510484939));
#22846=CARTESIAN_POINT('Ctrl Pts',(-7.74971360013524,0.833511408043322,
20.8453251672423));
#22847=CARTESIAN_POINT('Ctrl Pts',(-8.63771535503727,1.19472088021124,20.8850935201213));
#22848=CARTESIAN_POINT('Ctrl Pts',(-9.58001953300302,0.528821234560933,
20.9328155435762));
#22849=CARTESIAN_POINT('Ctrl Pts',(-9.52838301578789,-0.621651590320803,
20.9805375670311));
#22850=CARTESIAN_POINT('Ctrl Pts',(-8.53370943520822,-1.20206395993246,
21.0282595904859));
#22851=CARTESIAN_POINT('Ctrl Pts',(-7.50615334947754,-0.677194459421418,
21.0759816139408));
#22852=CARTESIAN_POINT('Ctrl Pts',(-7.41327593151281,0.276950804532245,
21.1157499668198));
#22853=CARTESIAN_POINT('Ctrl Pts',(-7.84342241956686,0.827955836183989,
21.1475646491231));
#22854=CARTESIAN_POINT('Ctrl Pts',(-8.47794236898817,1.12124235117772,21.1793793314263));
#22855=CARTESIAN_POINT('Ctrl Pts',(-9.38582839088678,0.813407377963039,
21.2191476843054));
#22856=CARTESIAN_POINT('Ctrl Pts',(-9.66276494835087,-0.306711207289787,
21.2668697077602));
#22857=CARTESIAN_POINT('Ctrl Pts',(-8.87098453458713,-1.14297541618645,
21.3145917312151));
#22858=CARTESIAN_POINT('Ctrl Pts',(-7.73900775363358,-0.931120234320342,
21.3623137546699));
#22859=CARTESIAN_POINT('Ctrl Pts',(-7.30532610571126,0.138122362167578,
21.4100357781248));
#22860=CARTESIAN_POINT('Ctrl Pts',(-7.85936439009799,0.920465623739351,
21.4498041310038));
#22861=CARTESIAN_POINT('Ctrl Pts',(-8.54517508124857,1.05572922562215,21.4816188133071));
#22862=CARTESIAN_POINT('Ctrl Pts',(-9.21692408647285,0.862375094373378,
21.5134334956103));
#22863=CARTESIAN_POINT('Ctrl Pts',(-9.70210596903635,0.0355631808614804,
21.5532018484894));
#22864=CARTESIAN_POINT('Ctrl Pts',(-9.17867017339294,-0.992723972480452,
21.6009238719442));
#22865=CARTESIAN_POINT('Ctrl Pts',(-8.03273355651315,-1.10710631725258,
21.6486458953991));
#22866=CARTESIAN_POINT('Ctrl Pts',(-7.31528473835207,-0.206261578121178,
21.696367918854));
#22867=CARTESIAN_POINT('Ctrl Pts',(-7.68689445148562,0.886105449481559,
21.7440899423088));
#22868=CARTESIAN_POINT('Ctrl Pts',(-8.61775845399796,1.11525956425955,21.7838582951879));
#22869=CARTESIAN_POINT('Ctrl Pts',(-9.22490519083297,0.768841628751961,
21.8156729774911));
#22870=CARTESIAN_POINT('Ctrl Pts',(-9.60641007295241,0.183105706164161,
21.8474876597944));
#22871=CARTESIAN_POINT('Ctrl Pts',(-9.43236487056282,-0.759617830732116,
21.8872560126734));
#22872=CARTESIAN_POINT('Ctrl Pts',(-8.36372819600901,-1.1947903938464,21.9349780361283));
#22873=CARTESIAN_POINT('Ctrl Pts',(-7.4222718664851,-0.531530241039888,
21.9827000595831));
#22874=CARTESIAN_POINT('Ctrl Pts',(-7.46910254533488,0.619148227612382,
22.030422083038));
#22875=CARTESIAN_POINT('Ctrl Pts',(-8.46484635226162,1.20211801487061,22.0781441064929));
#22876=CARTESIAN_POINT('Ctrl Pts',(-9.31874605361725,0.766371873731396,
22.1179124593719));
#22877=CARTESIAN_POINT('Ctrl Pts',(-9.55124883403978,0.107148843804094,
22.1497271416752));
#22878=CARTESIAN_POINT('Ctrl Pts',(-9.45652849662567,-0.585426497780417,
22.1815418239783));
#22879=CARTESIAN_POINT('Ctrl Pts',(-8.7081020895998,-1.18449019452673,22.2213101768575));
#22880=CARTESIAN_POINT('Ctrl Pts',(-7.61521781807871,-0.814404432911052,
22.2690322003123));
#22881=CARTESIAN_POINT('Ctrl Pts',(-7.33719548426661,0.30316329774476,22.3167542237672));
#22882=CARTESIAN_POINT('Ctrl Pts',(-8.12547601519426,1.14272738419793,22.364476247222));
#22883=CARTESIAN_POINT('Ctrl Pts',(-9.25993542285189,0.932106031372354,
22.4121982706769));
#22884=CARTESIAN_POINT('Ctrl Pts',(-9.62060038945631,0.043882984296242,
22.4519666235559));
#22885=CARTESIAN_POINT('Ctrl Pts',(-9.36511565208,-0.606778290914208,22.4837813058592));
#22886=CARTESIAN_POINT('Ctrl Pts',(-8.84034563057633,-1.06856717192135,
22.5155959881624));
#22887=CARTESIAN_POINT('Ctrl Pts',(-7.88239092197955,-1.03193145478393,
22.5553643410415));
#22888=CARTESIAN_POINT('Ctrl Pts',(-7.29803287792558,-0.0370017194567047,
22.6030863644964));
#22889=CARTESIAN_POINT('Ctrl Pts',(-7.81897858119011,0.990066742210633,
22.6508083879512));
#22890=CARTESIAN_POINT('Ctrl Pts',(-8.96442744040265,1.10923452993118,22.6985304114061));
#22891=CARTESIAN_POINT('Ctrl Pts',(-9.68456102159392,0.207698547770979,
22.7462524348609));
#22892=CARTESIAN_POINT('Ctrl Pts',(-9.37616947743245,-0.699998568552913,
22.78602078774));
#22893=CARTESIAN_POINT('Ctrl Pts',(-8.75724433503361,-1.02490503847511,
22.8178354700433));
#22894=CARTESIAN_POINT('Ctrl Pts',(-8.05824652988369,-1.03078844619088,
22.8496501523464));
#22895=CARTESIAN_POINT('Ctrl Pts',(-7.35776007830284,-0.376312983973493,
22.8894185052256));
#22896=CARTESIAN_POINT('Ctrl Pts',(-7.56679892742373,0.758439086501402,
22.9371405286804));
#22897=CARTESIAN_POINT('Ctrl Pts',(-8.63275509706559,1.19431922496145,22.9848625521353));
#22898=CARTESIAN_POINT('Ctrl Pts',(-9.57697357271459,0.534997208838448,
23.0325845755901));
#22899=CARTESIAN_POINT('Ctrl Pts',(-9.53172098907367,-0.617960598526017,
23.080306599045));
#22900=CARTESIAN_POINT('Ctrl Pts',(-8.70461176387205,-1.10263546797914,
23.120074951924));
#22901=CARTESIAN_POINT('Ctrl Pts',(-8.02396811303862,-0.94339738625594,
23.1518896342273));
#22902=CARTESIAN_POINT('Ctrl Pts',(-7.49149931215251,-0.490507198491067,
23.1837043165305));
#22903=CARTESIAN_POINT('Ctrl Pts',(-7.38996361074661,0.462755567399329,
23.2234726694096));
#22904=CARTESIAN_POINT('Ctrl Pts',(-8.29049430233965,1.18414587464485,23.2711946928644));
#22905=CARTESIAN_POINT('Ctrl Pts',(-9.38181438475884,0.816349017113292,
23.3189167163193));
#22906=CARTESIAN_POINT('Ctrl Pts',(-9.66450224059603,-0.300047698603672,
23.3666387397741));
#22907=CARTESIAN_POINT('Ctrl Pts',(-8.87592382612184,-1.1423680569675,23.414360763229));
#22908=CARTESIAN_POINT('Ctrl Pts',(-7.93330717426711,-0.967744899456104,
23.4541291161081));
#22909=CARTESIAN_POINT('Ctrl Pts',(-7.52275427457137,-0.40198977341469,
23.4859437984113));
#22910=CARTESIAN_POINT('Ctrl Pts',(-7.41638948221304,0.288893050975484,
23.5177584807145));
#22911=CARTESIAN_POINT('Ctrl Pts',(-7.96330251111076,1.0762338528618,23.5575268335936));
#22912=CARTESIAN_POINT('Ctrl Pts',(-9.11632231352085,1.03258941290663,23.6052488570485));
#22913=CARTESIAN_POINT('Ctrl Pts',(-9.70099501608219,0.0404140848616688,
23.6529708805033));
#22914=CARTESIAN_POINT('Ctrl Pts',(-9.18434379973964,-0.988821345617322,
23.7006929039582));
#22915=CARTESIAN_POINT('Ctrl Pts',(-8.03686629447588,-1.10987867419518,
23.7484149274131));
#22916=CARTESIAN_POINT('Ctrl Pts',(-7.43826157375447,-0.361085119319684,
23.7881832802921));
#22917=CARTESIAN_POINT('Ctrl Pts',(-7.49794123728335,0.335385184319912,
23.8199979625954));
#22918=CARTESIAN_POINT('Ctrl Pts',(-7.86953258335037,0.927459856653405,
23.8518126448985));
#22919=CARTESIAN_POINT('Ctrl Pts',(-8.79827787305733,1.16505528240947,23.8915809977777));
#22920=CARTESIAN_POINT('Ctrl Pts',(-9.64169728990653,0.377652469885521,
23.9393030212325));
#22921=CARTESIAN_POINT('Ctrl Pts',(-9.43469855296966,-0.755222445366839,
23.9870250446874));
#22922=CARTESIAN_POINT('Ctrl Pts',(-8.37057230129222,-1.19555115348436,
24.0347470681422));
#22923=CARTESIAN_POINT('Ctrl Pts',(-7.42358336856485,-0.53633080854597,
24.0824690915971));
#22924=CARTESIAN_POINT('Ctrl Pts',(-7.46080640494651,0.421601258489856,
24.1222374444762));
#22925=CARTESIAN_POINT('Ctrl Pts',(-7.96162519206712,0.909262092018453,
24.1540521267794));
#22926=CARTESIAN_POINT('Ctrl Pts',(-8.63002436311974,1.11389614154808,24.1858668090826));
#22927=CARTESIAN_POINT('Ctrl Pts',(-9.48784475277574,0.685919999008078,
24.2256351619617));
#22928=CARTESIAN_POINT('Ctrl Pts',(-9.61050241956603,-0.461387544184418,
24.2733571854165));
#22929=CARTESIAN_POINT('Ctrl Pts',(-8.7127427526925,-1.18269304897183,24.3210792088714));
#22930=CARTESIAN_POINT('Ctrl Pts',(-7.61989594642513,-0.819457713778855,
24.3688012323262));
#22931=CARTESIAN_POINT('Ctrl Pts',(-7.33504640190931,0.298674764453505,
24.4165232557811));
#22932=CARTESIAN_POINT('Ctrl Pts',(-7.98995121235915,0.998759822673351,
24.4562916086602));
#22933=CARTESIAN_POINT('Ctrl Pts',(-8.68776329032791,1.03987976834045,24.4881062909634));
#22934=CARTESIAN_POINT('Ctrl Pts',(-9.32713012937044,0.757315454911642,
24.5199209732667));
#22935=CARTESIAN_POINT('Ctrl Pts',(-9.6958438758722,-0.127596728660042,
24.5596893261457));
#22936=CARTESIAN_POINT('Ctrl Pts',(-9.03794499462271,-1.07550419457617,
24.6074113496006));
#22937=CARTESIAN_POINT('Ctrl Pts',(-7.88707627331942,-1.03360864556243,
24.6551333730554));
#22938=CARTESIAN_POINT('Ctrl Pts',(-7.29826447283417,-0.0438840806905483,
24.7028553965103));
#22939=CARTESIAN_POINT('Ctrl Pts',(-7.81441657777274,0.988078373304951,
24.7505774199651));
#22940=CARTESIAN_POINT('Ctrl Pts',(-8.76774141647179,1.08902960614764,24.7903457728442));
#22941=CARTESIAN_POINT('Ctrl Pts',(-9.32236803150491,0.663562963521387,
24.8221604551474));
#22942=CARTESIAN_POINT('Ctrl Pts',(-9.62101545059055,0.0315485133984316,
24.8539751374507));
#22943=CARTESIAN_POINT('Ctrl Pts',(-9.32087705117602,-0.878910898486496,
24.8937434903297));
#22944=CARTESIAN_POINT('Ctrl Pts',(-8.20314295733665,-1.16531969262162,
24.9414655137846));
#22945=CARTESIAN_POINT('Ctrl Pts',(-7.36020604022749,-0.380646891719252,
24.9891875372395));
#22946=CARTESIAN_POINT('Ctrl Pts',(-7.56247108791455,0.753082750296701,
25.0369095606943));
#22947=CARTESIAN_POINT('Ctrl Pts',(-8.62800411895744,1.19580033707794,25.0846315841492));
#22948=CARTESIAN_POINT('Ctrl Pts',(-9.41500945814661,0.648404688957932,
25.1243999370283));
#22949=CARTESIAN_POINT('Ctrl Pts',(-9.55607381873532,-0.03623637923947,
25.1562146193315));
#22950=CARTESIAN_POINT('Ctrl Pts',(-9.36841318440126,-0.709598118880296,
25.1880293016347));
#22951=CARTESIAN_POINT('Ctrl Pts',(-8.54573811554186,-1.20176184221852,
25.2277976545138));
#22952=CARTESIAN_POINT('Ctrl Pts',(-7.51305675689754,-0.687049579495533,
25.2755196779686));
#22953=CARTESIAN_POINT('Ctrl Pts',(-7.38897779306161,0.457877693930538,
25.3232417014235));
#22954=CARTESIAN_POINT('Ctrl Pts',(-8.2837168214319,1.18292674179725,25.3709637248784));
#22955=CARTESIAN_POINT('Ctrl Pts',(-9.37919050223605,0.820577577931373,
25.4186857483332));
#22956=CARTESIAN_POINT('Ctrl Pts',(-9.61621646562617,-0.108313207991237,
25.4584541012123));
#22957=CARTESIAN_POINT('Ctrl Pts',(-9.2749506328032,-0.718370727769788,
25.4902687835155));
#22958=CARTESIAN_POINT('Ctrl Pts',(-8.69246525801796,-1.1048203807029,25.5220834658188));
#22959=CARTESIAN_POINT('Ctrl Pts',(-7.74830215233154,-0.938761868865786,
25.5618518186978));
#22960=CARTESIAN_POINT('Ctrl Pts',(-7.30409883310168,0.126152640883285,
25.6095738421527));
#22961=CARTESIAN_POINT('Ctrl Pts',(-7.95936549339064,1.07318994459167,25.6572958656076));
#22962=CARTESIAN_POINT('Ctrl Pts',(-9.11039916814726,1.03610180258297,25.7050178890624));
#22963=CARTESIAN_POINT('Ctrl Pts',(-9.70177735444918,0.0453286990647764,
25.7527399125173));
#22964=CARTESIAN_POINT('Ctrl Pts',(-9.27327535899608,-0.812229135361383,
25.7925082653963));
#22965=CARTESIAN_POINT('Ctrl Pts',(-8.61604415988881,-1.05030411726996,
25.8243229476996));
#22966=CARTESIAN_POINT('Ctrl Pts',(-7.92269179652815,-0.961450044133608,
25.8561376300028));
#22967=CARTESIAN_POINT('Ctrl Pts',(-7.31731389777389,-0.218121718833848,
25.8959059828819));
#22968=CARTESIAN_POINT('Ctrl Pts',(-7.67813478609319,0.877856286621276,
25.9436280063367));
#22969=CARTESIAN_POINT('Ctrl Pts',(-8.7933089252946,1.16532922440482,25.9913500297916));
#22970=CARTESIAN_POINT('Ctrl Pts',(-9.63951597410066,0.384184115444669,
26.0390720532464));
#22971=CARTESIAN_POINT('Ctrl Pts',(-9.43850572746812,-0.752017619564397,
26.0867940767013));
#22972=CARTESIAN_POINT('Ctrl Pts',(-8.55336765023902,-1.12018875332168,
26.1265624295803));
#22973=CARTESIAN_POINT('Ctrl Pts',(-7.9005669296872,-0.870221224754899,
26.1583771118836));
#22974=CARTESIAN_POINT('Ctrl Pts',(-7.43435225028074,-0.34937919611602,
26.1901917941868));
#22975=CARTESIAN_POINT('Ctrl Pts',(-7.46287726373823,0.608851320565757,
26.2299601470659));
#22976=CARTESIAN_POINT('Ctrl Pts',(-8.45282457279144,1.20161082254541,26.2776821705207));
#22977=CARTESIAN_POINT('Ctrl Pts',(-9.48426620400552,0.689378246365516,
26.3254041939756));
#22978=CARTESIAN_POINT('Ctrl Pts',(-9.61312631029696,-0.455020776575367,
26.3731262174304));
#22979=CARTESIAN_POINT('Ctrl Pts',(-8.71771879103822,-1.18276034286521,
26.4208482408854));
#22980=CARTESIAN_POINT('Ctrl Pts',(-7.80744356640935,-0.882063793301015,
26.4606165937644));
#22981=CARTESIAN_POINT('Ctrl Pts',(-7.47730934038002,-0.265911264380824,
26.4924312760676));
#22982=CARTESIAN_POINT('Ctrl Pts',(-7.4655089049693,0.433011689752842,26.5242459583709));
#22983=CARTESIAN_POINT('Ctrl Pts',(-8.11403107601491,1.13901338462003,26.5640143112499));
#22984=CARTESIAN_POINT('Ctrl Pts',(-9.25051206695811,0.939588062472506,
26.6117363347048));
#22985=CARTESIAN_POINT('Ctrl Pts',(-9.69540024485459,-0.122640048560796,
26.6594583581596));
#22986=CARTESIAN_POINT('Ctrl Pts',(-9.04409496258458,-1.07240606184442,
26.7071803816145));
#22987=CARTESIAN_POINT('Ctrl Pts',(-7.89079538986508,-1.03691525382556,
26.7549024050694));
#22988=CARTESIAN_POINT('Ctrl Pts',(-7.39913614463224,-0.213938591902498,
26.7946707579484));
#22989=CARTESIAN_POINT('Ctrl Pts',(-7.55260665586685,0.468028671440933,
26.8264854402517));
#22990=CARTESIAN_POINT('Ctrl Pts',(-8.00097309834699,1.00431225253255,26.8583001225549));
#22991=CARTESIAN_POINT('Ctrl Pts',(-8.95334217548371,1.11391398795126,26.8980684754339));
#22992=CARTESIAN_POINT('Ctrl Pts',(-9.68232991269352,0.219522361823951,
26.9457904988889));
#22993=CARTESIAN_POINT('Ctrl Pts',(-9.32378460508592,-0.874872134276119,
26.9935125223437));
#22994=CARTESIAN_POINT('Ctrl Pts',(-8.20982093399049,-1.16700051389895,
27.0412345457986));
#22995=CARTESIAN_POINT('Ctrl Pts',(-7.36085519035604,-0.385580864783285,
27.0889565692533));
#22996=CARTESIAN_POINT('Ctrl Pts',(-7.52749254142181,0.558480252265147,
27.1287249221325));
#22997=CARTESIAN_POINT('Ctrl Pts',(-8.08975193490343,0.973807738151165,
27.1605396044356));
#22998=CARTESIAN_POINT('Ctrl Pts',(-8.77970959220288,1.08601726192087,27.192354286739));
#22999=CARTESIAN_POINT('Ctrl Pts',(-9.57165197508597,0.545788919748368,
27.232122639618));
#23000=CARTESIAN_POINT('Ctrl Pts',(-9.53776977793861,-0.607559032348173,
27.2798446630729));
#23001=CARTESIAN_POINT('Ctrl Pts',(-8.55057944115751,-1.20060986462781,
27.3275666865277));
#23002=CARTESIAN_POINT('Ctrl Pts',(-7.5170072729736,-0.692689965571765,
27.3752887099826));
#23003=CARTESIAN_POINT('Ctrl Pts',(-7.38624052039643,0.453721635167412,
27.4230107334374));
#23004=CARTESIAN_POINT('Ctrl Pts',(-8.12993986576823,1.05864368236566,27.4627790863165));
#23005=CARTESIAN_POINT('Ctrl Pts',(-8.8268904211843,1.00486199964796,27.4945937686197));
#23006=CARTESIAN_POINT('Ctrl Pts',(-9.42208951743369,0.638296068450471,
27.526408450923));
#23007=CARTESIAN_POINT('Ctrl Pts',(-9.66753855376051,-0.288404622203879,
27.566176803802));
#23008=CARTESIAN_POINT('Ctrl Pts',(-8.88730376835095,-1.13845943309884,
27.6138988272569));
#23009=CARTESIAN_POINT('Ctrl Pts',(-7.75271713556691,-0.941058259319852,
27.6616208507118));
#23010=CARTESIAN_POINT('Ctrl Pts',(-7.30339603824854,0.119302340762093,
27.7093428741666));
#23011=CARTESIAN_POINT('Ctrl Pts',(-7.95457620017757,1.07183785117575,27.7570648976215));
#23012=CARTESIAN_POINT('Ctrl Pts',(-8.91278904795361,1.04272534785048,27.7968332505005));
#23013=CARTESIAN_POINT('Ctrl Pts',(-9.40467199804332,0.546052709685484,
27.8286479328038));
#23014=CARTESIAN_POINT('Ctrl Pts',(-9.61495692658599,-0.12059021941417,
27.860462615107));
#23015=CARTESIAN_POINT('Ctrl Pts',(-9.19425784119395,-0.98200282614995,
27.9002309679861));
#23016=CARTESIAN_POINT('Ctrl Pts',(-8.04802974380756,-1.1143684208142,27.9479529914409));
#23017=CARTESIAN_POINT('Ctrl Pts',(-7.31915026362204,-0.222747002236805,
27.9956750148958));
#23018=CARTESIAN_POINT('Ctrl Pts',(-7.67312128813442,0.873135548270785,
28.0433970383507));
#23019=CARTESIAN_POINT('Ctrl Pts',(-8.78880236016895,1.16744023289704,28.0911190618055));
#23020=CARTESIAN_POINT('Ctrl Pts',(-9.4944063106267,0.518485331080839,28.1308874146846));
#23021=CARTESIAN_POINT('Ctrl Pts',(-9.54143198385559,-0.178953649868804,
28.1627020969878));
#23022=CARTESIAN_POINT('Ctrl Pts',(-9.2642902385457,-0.820689576163826,
28.1945167792911));
#23023=CARTESIAN_POINT('Ctrl Pts',(-8.38253104166786,-1.19688117390719,
28.2342851321701));
#23024=CARTESIAN_POINT('Ctrl Pts',(-7.42908821758638,-0.547030203993041,
28.282007155625));
#23025=CARTESIAN_POINT('Ctrl Pts',(-7.4612397960453,0.604151939156692,28.3297291790798));
#23026=CARTESIAN_POINT('Ctrl Pts',(-8.44594441868381,1.20132097455935,28.3774512025347));
#23027=CARTESIAN_POINT('Ctrl Pts',(-9.48223928754388,0.693923254147899,
28.4251732259896));
#23028=CARTESIAN_POINT('Ctrl Pts',(-9.59125710079042,-0.258512841292752,
28.4649415788686));
#23029=CARTESIAN_POINT('Ctrl Pts',(-9.17050079378615,-0.816721293551335,
28.4967562611719));
#23030=CARTESIAN_POINT('Ctrl Pts',(-8.5410371348917,-1.12070821481403,28.5285709434751));
#23031=CARTESIAN_POINT('Ctrl Pts',(-7.62806957928328,-0.828287897936413,
28.5683392963542));
#23032=CARTESIAN_POINT('Ctrl Pts',(-7.33220907315438,0.286981604349355,
28.616061319809));
#23033=CARTESIAN_POINT('Ctrl Pts',(-8.10971802963793,1.13653082253137,28.6637833432638));
#23034=CARTESIAN_POINT('Ctrl Pts',(-9.24511928569963,0.94387040363248,28.7115053667187));
#23035=CARTESIAN_POINT('Ctrl Pts',(-9.69684108623964,-0.117876702228018,
28.7592273901736));
#23036=CARTESIAN_POINT('Ctrl Pts',(-9.15612729992706,-0.909487720987729,
28.7989957430526));
#23037=CARTESIAN_POINT('Ctrl Pts',(-8.47270492162156,-1.05634272967534,
28.8308104253559));
#23038=CARTESIAN_POINT('Ctrl Pts',(-7.79777869557615,-0.874389043558764,
28.8626251076591));
#23039=CARTESIAN_POINT('Ctrl Pts',(-7.29866841691336,-0.0559097679814885,
28.9023934605382));
#23040=CARTESIAN_POINT('Ctrl Pts',(-7.80462023258882,0.981091778944407,
28.950115483993));
#23041=CARTESIAN_POINT('Ctrl Pts',(-8.94845616402851,1.11485849141853,28.9978375074479));
#23042=CARTESIAN_POINT('Ctrl Pts',(-9.68105338849322,0.226289253312137,
29.0455595309028));
#23043=CARTESIAN_POINT('Ctrl Pts',(-9.32799092443192,-0.872212497622574,
29.0932815543577));
#23044=CARTESIAN_POINT('Ctrl Pts',(-8.40113958681821,-1.1170934666179,29.1330499072367));
#23045=CARTESIAN_POINT('Ctrl Pts',(-7.78821550048514,-0.781003980273933,
29.1648645895399));
#23046=CARTESIAN_POINT('Ctrl Pts',(-7.39684779309566,-0.201811312772201,
29.1966792718432));
#23047=CARTESIAN_POINT('Ctrl Pts',(-7.55490987902498,0.743724623326478,
29.2364476247223));
#23048=CARTESIAN_POINT('Ctrl Pts',(-8.61602196756742,1.1969251851499,29.284169648177));
#23049=CARTESIAN_POINT('Ctrl Pts',(-9.56857936365253,0.549701954262166,
29.331891671632));
#23050=CARTESIAN_POINT('Ctrl Pts',(-9.54122335203833,-0.601610010653767,
29.3796136950868));
#23051=CARTESIAN_POINT('Ctrl Pts',(-8.55551746389829,-1.20134333884888,
29.4273357185417));
#23052=CARTESIAN_POINT('Ctrl Pts',(-7.6943163535033,-0.780136065581471,
29.4671040714207));
#23053=CARTESIAN_POINT('Ctrl Pts',(-7.45075543190132,-0.124914290005815,
29.498918753724));
#23054=CARTESIAN_POINT('Ctrl Pts',(-7.53360098225563,0.569107464161486,
29.5307334360272));
#23055=CARTESIAN_POINT('Ctrl Pts',(-8.27207885390538,1.18088449447138,29.5705017889063));
#23056=CARTESIAN_POINT('Ctrl Pts',(-9.37052414128468,0.829120622166084,
29.6182238123611));
#23057=CARTESIAN_POINT('Ctrl Pts',(-9.66839871578049,-0.283165032010691,
29.665945835816));
#23058=CARTESIAN_POINT('Ctrl Pts',(-8.89262325021065,-1.13673653623531,
29.7136678592708));
#23059=CARTESIAN_POINT('Ctrl Pts',(-7.94740422892346,-0.975943072842761,
29.7534362121499));
#23060=CARTESIAN_POINT('Ctrl Pts',(-7.52860489572998,-0.416034089157435,
29.7852508944531));
#23061=CARTESIAN_POINT('Ctrl Pts',(-7.41259114042627,0.272911730206623,
29.8170655767564));
#23062=CARTESIAN_POINT('Ctrl Pts',(-7.94709221312467,1.06881550059101,29.8568339296354));
#23063=CARTESIAN_POINT('Ctrl Pts',(-9.10241563751445,1.0405751389091,29.9045559530903));
#23064=CARTESIAN_POINT('Ctrl Pts',(-9.5986718480284,0.223190340067093,29.9443243059693));
#23065=CARTESIAN_POINT('Ctrl Pts',(-9.45136298239413,-0.462871519683194,
29.9761389882726));
#23066=CARTESIAN_POINT('Ctrl Pts',(-9.22802350159151,-0.72929719873085,
29.9920463294242));
#23067=CARTESIAN_POINT('Ctrl Pts',(-9.09015970213924,-0.82760676144889,
30.));
#23068=CARTESIAN_POINT('Ctrl Pts',(-8.96251688654953,0.969001292714065,
1.73389339417778));
#23069=CARTESIAN_POINT('Ctrl Pts',(-9.12393436899475,0.89195463449329,1.74184706475359));
#23070=CARTESIAN_POINT('Ctrl Pts',(-9.40504227116756,0.655650918757411,
1.75775440590521));
#23071=CARTESIAN_POINT('Ctrl Pts',(-9.68384680217516,-0.0311347557633745,
1.78956908820845));
#23072=CARTESIAN_POINT('Ctrl Pts',(-9.3171516591104,-0.972316947591156,
1.8293374410875));
#23073=CARTESIAN_POINT('Ctrl Pts',(-8.1203802128438,-1.21312531614354,1.87705946454236));
#23074=CARTESIAN_POINT('Ctrl Pts',(-7.41865918333397,-0.482923354571855,
1.91682781742141));
#23075=CARTESIAN_POINT('Ctrl Pts',(-7.41327429528892,0.255051675597989,
1.94864249972466));
#23076=CARTESIAN_POINT('Ctrl Pts',(-7.74650629928063,0.914194267158726,
1.9804571820279));
#23077=CARTESIAN_POINT('Ctrl Pts',(-8.70043812865199,1.25445422207282,2.02022553490695));
#23078=CARTESIAN_POINT('Ctrl Pts',(-9.66372213760587,0.5084118152494,2.06794755836181));
#23079=CARTESIAN_POINT('Ctrl Pts',(-9.55738109299735,-0.703265592318366,
2.11566958181668));
#23080=CARTESIAN_POINT('Ctrl Pts',(-8.47898877892832,-1.27024239984107,
2.16339160527153));
#23081=CARTESIAN_POINT('Ctrl Pts',(-7.59875658277994,-0.76892502565052,
2.20315995815059));
#23082=CARTESIAN_POINT('Ctrl Pts',(-7.3855597050091,-0.0620612536970827,
2.23497464045383));
#23083=CARTESIAN_POINT('Ctrl Pts',(-7.51904000752238,0.664170613866673,
2.26678932275707));
#23084=CARTESIAN_POINT('Ctrl Pts',(-8.33790718168219,1.25997621452937,2.30655767563613));
#23085=CARTESIAN_POINT('Ctrl Pts',(-9.47313874820412,0.816432151476354,
2.35427969909098));
#23086=CARTESIAN_POINT('Ctrl Pts',(-9.71229297188154,-0.376327816436324,
2.40200172254585));
#23087=CARTESIAN_POINT('Ctrl Pts',(-8.83974515101956,-1.22398743093948,
2.44972374600071));
#23088=CARTESIAN_POINT('Ctrl Pts',(-7.65288086934604,-0.946688199618081,
2.49744576945557));
#23089=CARTESIAN_POINT('Ctrl Pts',(-7.31540450356857,0.00807318411347469,
2.53721412233462));
#23090=CARTESIAN_POINT('Ctrl Pts',(-7.6165690570546,0.682257445519576,2.56902880463787));
#23091=CARTESIAN_POINT('Ctrl Pts',(-8.19271835958521,1.14407521357768,2.60084348694111));
#23092=CARTESIAN_POINT('Ctrl Pts',(-9.20178133687243,1.05893083384115,2.64061183982016));
#23093=CARTESIAN_POINT('Ctrl Pts',(-9.77011946603895,-0.0192825748483143,
2.68833386327502));
#23094=CARTESIAN_POINT('Ctrl Pts',(-9.17057421212321,-1.07777272054635,
2.73605588672988));
#23095=CARTESIAN_POINT('Ctrl Pts',(-7.95610586271703,-1.14793494130798,
2.78377791018475));
#23096=CARTESIAN_POINT('Ctrl Pts',(-7.23996422244131,-0.161682533818757,
2.83149993363961));
#23097=CARTESIAN_POINT('Ctrl Pts',(-7.60942829901139,0.781160600976021,
2.87126828651866));
#23098=CARTESIAN_POINT('Ctrl Pts',(-8.27828889582619,1.09396997251331,2.9030829688219));
#23099=CARTESIAN_POINT('Ctrl Pts',(-9.01616168526782,1.06625838374102,2.93489765112514));
#23100=CARTESIAN_POINT('Ctrl Pts',(-9.72356051529724,0.341659331902824,
2.9746660040042));
#23101=CARTESIAN_POINT('Ctrl Pts',(-9.44791592231979,-0.845594970502356,
3.02238802745905));
#23102=CARTESIAN_POINT('Ctrl Pts',(-8.30195997305303,-1.2538117450032,3.07011005091392));
#23103=CARTESIAN_POINT('Ctrl Pts',(-7.3376086220987,-0.512271154700922,
3.11783207436878));
#23104=CARTESIAN_POINT('Ctrl Pts',(-7.44130827730874,0.702141914088998,
3.16555409782365));
#23105=CARTESIAN_POINT('Ctrl Pts',(-8.33759911760778,1.17343759126272,3.2053224507027));
#23106=CARTESIAN_POINT('Ctrl Pts',(-9.048091740403,0.972379329670738,3.23713713300594));
#23107=CARTESIAN_POINT('Ctrl Pts',(-9.58797938135923,0.468647727902608,
3.26895181530918));
#23108=CARTESIAN_POINT('Ctrl Pts',(-9.64886220328975,-0.542168856809507,
3.30872016818823));
#23109=CARTESIAN_POINT('Ctrl Pts',(-8.66360959361254,-1.25968541784617,
3.3564421916431));
#23110=CARTESIAN_POINT('Ctrl Pts',(-7.52988896786481,-0.818625878810704,
3.40416421509795));
#23111=CARTESIAN_POINT('Ctrl Pts',(-7.28576943901448,0.373121422369535,
3.45188623855282));
#23112=CARTESIAN_POINT('Ctrl Pts',(-8.15875752784666,1.22367683912943,3.49960826200768));
#23113=CARTESIAN_POINT('Ctrl Pts',(-9.14493928233647,0.993671549987388,
3.53937661488673));
#23114=CARTESIAN_POINT('Ctrl Pts',(-9.55070350372043,0.376760220734811,
3.57119129718998));
#23115=CARTESIAN_POINT('Ctrl Pts',(-9.62941435269904,-0.357425582565709,
3.60300597949321));
#23116=CARTESIAN_POINT('Ctrl Pts',(-9.01410119783594,-1.1616933286404,3.64277433237227));
#23117=CARTESIAN_POINT('Ctrl Pts',(-7.79954467407403,-1.05968758954777,
3.69049635582713));
#23118=CARTESIAN_POINT('Ctrl Pts',(-7.23074064851598,0.0156346666816528,
3.73821837928199));
#23119=CARTESIAN_POINT('Ctrl Pts',(-7.82585959046674,1.07661978399709,3.78594040273685));
#23120=CARTESIAN_POINT('Ctrl Pts',(-9.04256021742503,1.14867743161063,3.83366242619172));
#23121=CARTESIAN_POINT('Ctrl Pts',(-9.63787582997991,0.32949722715489,3.87343077907076));
#23122=CARTESIAN_POINT('Ctrl Pts',(-9.54110428679668,-0.402526993718299,
3.90524546137401));
#23123=CARTESIAN_POINT('Ctrl Pts',(-9.12026732761714,-1.00925629522235,
3.93706014367725));
#23124=CARTESIAN_POINT('Ctrl Pts',(-8.12871927263138,-1.21490001765928,
3.97682849655631));
#23125=CARTESIAN_POINT('Ctrl Pts',(-7.27694707414092,-0.343099098814263,
4.02455052001116));
#23126=CARTESIAN_POINT('Ctrl Pts',(-7.55034783376434,0.842273415997345,
4.07227254346603));
#23127=CARTESIAN_POINT('Ctrl Pts',(-8.69458871454493,1.25527315084461,4.11999456692089));
#23128=CARTESIAN_POINT('Ctrl Pts',(-9.66186840419519,0.513705404640438,
4.16771659037575));
#23129=CARTESIAN_POINT('Ctrl Pts',(-9.57610546723251,-0.49530480569805,
4.2074849432548));
#23130=CARTESIAN_POINT('Ctrl Pts',(-9.0239736441167,-0.98558497194781,4.23929962555805));
#23131=CARTESIAN_POINT('Ctrl Pts',(-8.30874409956685,-1.16908126651006,
4.27111430786129));
#23132=CARTESIAN_POINT('Ctrl Pts',(-7.42433423631398,-0.675851016317698,
4.31088266074034));
#23133=CARTESIAN_POINT('Ctrl Pts',(-7.35057965317154,0.540747924042572,
4.3586046841952));
#23134=CARTESIAN_POINT('Ctrl Pts',(-8.33290414333639,1.25830946861962,4.40632670765007));
#23135=CARTESIAN_POINT('Ctrl Pts',(-9.46845713256172,0.82198919302504,4.45404873110492));
#23136=CARTESIAN_POINT('Ctrl Pts',(-9.71477345998143,-0.371694595533183,
4.50177075455979));
#23137=CARTESIAN_POINT('Ctrl Pts',(-8.98974083571195,-1.07864903513211,
4.54153910743884));
#23138=CARTESIAN_POINT('Ctrl Pts',(-8.25140932968082,-1.08817682170158,
4.57335378974208));
#23139=CARTESIAN_POINT('Ctrl Pts',(-7.59045685283196,-0.758986884336549,
4.60516847204533));
#23140=CARTESIAN_POINT('Ctrl Pts',(-7.24432911621094,0.192670867097964,
4.64493682492437));
#23141=CARTESIAN_POINT('Ctrl Pts',(-7.98454701788834,1.16098392507899,4.69265884837925));
#23142=CARTESIAN_POINT('Ctrl Pts',(-9.19691857333501,1.06092801182391,4.74038087183409));
#23143=CARTESIAN_POINT('Ctrl Pts',(-9.77020913005612,-0.0120090374981049,
4.78810289528898));
#23144=CARTESIAN_POINT('Ctrl Pts',(-9.17548452143473,-1.07589594883799,
4.83582491874381));
#23145=CARTESIAN_POINT('Ctrl Pts',(-8.16463079918994,-1.13615902333401,
4.87559327162288));
#23146=CARTESIAN_POINT('Ctrl Pts',(-7.60003131611499,-0.660289697545374,
4.90740795392612));
#23147=CARTESIAN_POINT('Ctrl Pts',(-7.31556584999249,0.0211085634582759,
4.93922263622936));
#23148=CARTESIAN_POINT('Ctrl Pts',(-7.67645521294405,0.96726698234605,4.97899098910842));
#23149=CARTESIAN_POINT('Ctrl Pts',(-8.86979428821997,1.21524797282673,5.02671301256327));
#23150=CARTESIAN_POINT('Ctrl Pts',(-9.72118982712491,0.346351194972045,
5.07443503601814));
#23151=CARTESIAN_POINT('Ctrl Pts',(-9.45274261220889,-0.840152941993902,
5.122157059473));
#23152=CARTESIAN_POINT('Ctrl Pts',(-8.3069013646354,-1.25560517219555,5.16987908292785));
#23153=CARTESIAN_POINT('Ctrl Pts',(-7.50301102084912,-0.639799032983755,
5.20964743580691));
#23154=CARTESIAN_POINT('Ctrl Pts',(-7.38738205917888,0.0894842691273791,
5.24146211811015));
#23155=CARTESIAN_POINT('Ctrl Pts',(-7.61807862935953,0.790913726750847,
5.2732768004134));
#23156=CARTESIAN_POINT('Ctrl Pts',(-8.51005392413996,1.27032686739803,5.31304515329244));
#23157=CARTESIAN_POINT('Ctrl Pts',(-9.5747692988779,0.677086704380666,5.36076717674732));
#23158=CARTESIAN_POINT('Ctrl Pts',(-9.65013915021099,-0.537069529282636,
5.40848920020216));
#23159=CARTESIAN_POINT('Ctrl Pts',(-8.67082039814986,-1.25872786679072,
5.45621122365704));
#23160=CARTESIAN_POINT('Ctrl Pts',(-7.53245251019283,-0.823215212682402,
5.50393324711189));
#23161=CARTESIAN_POINT('Ctrl Pts',(-7.32741674876059,0.168458736989412,
5.54370159999096));
#23162=CARTESIAN_POINT('Ctrl Pts',(-7.71712665940812,0.795635248872751,
5.57551628229418));
#23163=CARTESIAN_POINT('Ctrl Pts',(-8.35052222000327,1.17515370077386,5.60733096459744));
#23164=CARTESIAN_POINT('Ctrl Pts',(-9.33875141408655,0.954110840936048,
5.64709931747647));
#23165=CARTESIAN_POINT('Ctrl Pts',(-9.75580141396196,-0.191149835863871,
5.69482134093136));
#23166=CARTESIAN_POINT('Ctrl Pts',(-9.01840327573551,-1.15867242473384,
5.7425433643862));
#23167=CARTESIAN_POINT('Ctrl Pts',(-7.80562437442478,-1.06368131583976,
5.79026538784108));
#23168=CARTESIAN_POINT('Ctrl Pts',(-7.22967663147079,0.0104866959751704,
5.83798741129593));
#23169=CARTESIAN_POINT('Ctrl Pts',(-7.72344902443187,0.894593991428199,
5.87775576417499));
#23170=CARTESIAN_POINT('Ctrl Pts',(-8.42851681405126,1.11391932867013,5.90957044647822));
#23171=CARTESIAN_POINT('Ctrl Pts',(-9.15583523570149,0.986514049959575,
5.94138512878147));
#23172=CARTESIAN_POINT('Ctrl Pts',(-9.75856315988134,0.172772115844345,
5.98115348166051));
#23173=CARTESIAN_POINT('Ctrl Pts',(-9.32463867961743,-0.966202100566147,
6.02887550511538));
#23174=CARTESIAN_POINT('Ctrl Pts',(-8.13394924709671,-1.21543020796378,
6.07659752857024));
#23175=CARTESIAN_POINT('Ctrl Pts',(-7.27893185676339,-0.350097187409828,
6.12431955202511));
#23176=CARTESIAN_POINT('Ctrl Pts',(-7.54617495858737,0.839076409987852,
6.17204157547996));
#23177=CARTESIAN_POINT('Ctrl Pts',(-8.49804474355533,1.18462061611618,6.21180992835903));
#23178=CARTESIAN_POINT('Ctrl Pts',(-9.17475454711885,0.889175133368411,
6.24362461066226));
#23179=CARTESIAN_POINT('Ctrl Pts',(-9.64143292944961,0.31695535130891,6.27543929296551));
#23180=CARTESIAN_POINT('Ctrl Pts',(-9.56483372345286,-0.692791868328002,
6.31520764584455));
#23181=CARTESIAN_POINT('Ctrl Pts',(-8.49147006545099,-1.27023725786807,
6.36292966929943));
#23182=CARTESIAN_POINT('Ctrl Pts',(-7.42794252952587,-0.67967383658084,
6.41065169275427));
#23183=CARTESIAN_POINT('Ctrl Pts',(-7.34750194971839,0.534156994858903,
6.45837371620915));
#23184=CARTESIAN_POINT('Ctrl Pts',(-8.32765665896405,1.25862194650517,6.506095739664));
#23185=CARTESIAN_POINT('Ctrl Pts',(-9.27359363721055,0.89715255760802,6.54586409254306));
#23186=CARTESIAN_POINT('Ctrl Pts',(-9.59205391956505,0.230963965632939,
6.5776787748463));
#23187=CARTESIAN_POINT('Ctrl Pts',(-9.57058965043867,-0.507116976178952,
6.60949345714954));
#23188=CARTESIAN_POINT('Ctrl Pts',(-8.85200491848723,-1.22062441757679,
6.64926181002859));
#23189=CARTESIAN_POINT('Ctrl Pts',(-7.66245973772922,-0.955040187706783,
6.69698383348346));
#23190=CARTESIAN_POINT('Ctrl Pts',(-7.24455670919153,0.18741901636682,6.74470585693831));
#23191=CARTESIAN_POINT('Ctrl Pts',(-7.97790718835371,1.15801318951335,6.79242788039319));
#23192=CARTESIAN_POINT('Ctrl Pts',(-9.19315459354979,1.06459764271049,6.84014990384804));
#23193=CARTESIAN_POINT('Ctrl Pts',(-9.67202077022298,0.172328585328035,
6.87991825672709));
#23194=CARTESIAN_POINT('Ctrl Pts',(-9.47698425864094,-0.539840601498366,
6.91173293903033));
#23195=CARTESIAN_POINT('Ctrl Pts',(-8.97784102671058,-1.08397314558408,
6.94354762133358));
#23196=CARTESIAN_POINT('Ctrl Pts',(-7.96757605345196,-1.15341066952153,
6.98331597421262));
#23197=CARTESIAN_POINT('Ctrl Pts',(-7.24174472569243,-0.174267368536913,
7.03103799766749));
#23198=CARTESIAN_POINT('Ctrl Pts',(-7.67319115562676,0.963146343500352,
7.07876002112235));
#23199=CARTESIAN_POINT('Ctrl Pts',(-8.86282920540638,1.21734564473849,7.12648204457721));
#23200=CARTESIAN_POINT('Ctrl Pts',(-9.72074426707527,0.351589058172741,
7.17420406803208));
#23201=CARTESIAN_POINT('Ctrl Pts',(-9.49909556123563,-0.636504427851428,
7.21397242091113));
#23202=CARTESIAN_POINT('Ctrl Pts',(-8.88564125986018,-1.04747646052394,
7.24578710321437));
#23203=CARTESIAN_POINT('Ctrl Pts',(-8.15214807584167,-1.13239960526954,
7.27760178551761));
#23204=CARTESIAN_POINT('Ctrl Pts',(-7.34270032648874,-0.523916879967266,
7.31737013839667));
#23205=CARTESIAN_POINT('Ctrl Pts',(-7.43442080370642,0.691459635471147,
7.36509216185152));
#23206=CARTESIAN_POINT('Ctrl Pts',(-8.50488942279009,1.26934622450957,7.41281418530639));
#23207=CARTESIAN_POINT('Ctrl Pts',(-9.5708743944013,0.683230182643655,7.46053620876125));
#23208=CARTESIAN_POINT('Ctrl Pts',(-9.65322921746207,-0.53281685729308,
7.50825823221611));
#23209=CARTESIAN_POINT('Ctrl Pts',(-8.83911790121967,-1.13504575953026,
7.54802658509517));
#23210=CARTESIAN_POINT('Ctrl Pts',(-8.10630070797208,-1.04447450141926,
7.57984126739841));
#23211=CARTESIAN_POINT('Ctrl Pts',(-7.49603062788743,-0.628788777742681,
7.61165594970165));
#23212=CARTESIAN_POINT('Ctrl Pts',(-7.28200050464232,0.360982909197031,
7.65142430258071));
#23213=CARTESIAN_POINT('Ctrl Pts',(-8.14655966331663,1.2201046592259,7.69914632603555));
#23214=CARTESIAN_POINT('Ctrl Pts',(-9.33420412881433,0.956748250900423,
7.74686834949043));
#23215=CARTESIAN_POINT('Ctrl Pts',(-9.75687542788829,-0.183955456103537,
7.79459037294528));
#23216=CARTESIAN_POINT('Ctrl Pts',(-9.02352258302385,-1.157478093308,7.84231239640016));
#23217=CARTESIAN_POINT('Ctrl Pts',(-8.01382251646826,-1.08025982136799,
7.88208074927919));
#23218=CARTESIAN_POINT('Ctrl Pts',(-7.51888594635904,-0.532298159311594,
7.91389543158245));
#23219=CARTESIAN_POINT('Ctrl Pts',(-7.32934158139695,0.181352403097051,
7.94571011388567));
#23220=CARTESIAN_POINT('Ctrl Pts',(-7.81506734795048,1.06990592744422,7.98547846676475));
#23221=CARTESIAN_POINT('Ctrl Pts',(-9.03099833983435,1.1539567644209,8.03320049021958));
#23222=CARTESIAN_POINT('Ctrl Pts',(-9.7568498620581,0.177741858819174,8.08092251367447));
#23223=CARTESIAN_POINT('Ctrl Pts',(-9.33015803729021,-0.961464031663194,
8.12864453712933));
#23224=CARTESIAN_POINT('Ctrl Pts',(-8.13860216611695,-1.21787644574009,
8.17636656058419));
#23225=CARTESIAN_POINT('Ctrl Pts',(-7.42553542619493,-0.498854394380912,
8.21613491346323));
#23226=CARTESIAN_POINT('Ctrl Pts',(-7.40975777023888,0.239370000425714,
8.24794959576648));
#23227=CARTESIAN_POINT('Ctrl Pts',(-7.73334073953907,0.903085491802819,
8.27976427806972));
#23228=CARTESIAN_POINT('Ctrl Pts',(-8.68203431044009,1.2572569113934,8.31953263094878));
#23229=CARTESIAN_POINT('Ctrl Pts',(-9.65657885208541,0.525262610480109,
8.36725465440363));
#23230=CARTESIAN_POINT('Ctrl Pts',(-9.56678963438923,-0.687912509038488,
8.4149766778585));
#23231=CARTESIAN_POINT('Ctrl Pts',(-8.49874411665927,-1.27026527694677,
8.46269870131337));
#23232=CARTESIAN_POINT('Ctrl Pts',(-7.42986079315603,-0.684568118889016,
8.5104207247682));
#23233=CARTESIAN_POINT('Ctrl Pts',(-7.36104268004619,0.325739236934825,
8.5501890776473));
#23234=CARTESIAN_POINT('Ctrl Pts',(-7.83211544074118,0.894346874630846,
8.5820037599505));
#23235=CARTESIAN_POINT('Ctrl Pts',(-8.51108119571025,1.18457040071787,8.61381844225378));
#23236=CARTESIAN_POINT('Ctrl Pts',(-9.4602607554946,0.831703500582261,8.65358679513279));
#23237=CARTESIAN_POINT('Ctrl Pts',(-9.71833485487774,-0.359493577758626,
8.70130881858769));
#23238=CARTESIAN_POINT('Ctrl Pts',(-8.8566765445911,-1.21821409722202,8.74903084204253));
#23239=CARTESIAN_POINT('Ctrl Pts',(-7.66794243081652,-0.959820635652346,
8.7967528654974));
#23240=CARTESIAN_POINT('Ctrl Pts',(-7.24280517665126,0.182462619648683,
8.84447488895226));
#23241=CARTESIAN_POINT('Ctrl Pts',(-7.85178406346805,0.991537153505232,
8.88424324183131));
#23242=CARTESIAN_POINT('Ctrl Pts',(-8.58006239840726,1.11333558688276,8.91605792413455));
#23243=CARTESIAN_POINT('Ctrl Pts',(-9.28341964256379,0.888585106109975,
8.9478726064378));
#23244=CARTESIAN_POINT('Ctrl Pts',(-9.7703664594142,0.000700156646912752,
8.98764095931684));
#23245=CARTESIAN_POINT('Ctrl Pts',(-9.18616070697658,-1.06899903426569,
9.03536298277171));
#23246=CARTESIAN_POINT('Ctrl Pts',(-7.97268600802238,-1.15464440326732,
9.08308500622657));
#23247=CARTESIAN_POINT('Ctrl Pts',(-7.24276328418966,-0.181469808723208,
9.13080702968144));
#23248=CARTESIAN_POINT('Ctrl Pts',(-7.66862368739739,0.960544042856526,
9.17852905313629));
#23249=CARTESIAN_POINT('Ctrl Pts',(-8.65852641109519,1.17396729261957,9.21829740601534));
#23250=CARTESIAN_POINT('Ctrl Pts',(-9.2889794685506,0.789580594280234,9.2501120883186));
#23251=CARTESIAN_POINT('Ctrl Pts',(-9.67384621642015,0.159420473438413,
9.28192677062181));
#23252=CARTESIAN_POINT('Ctrl Pts',(-9.46117695097487,-0.830644509004026,
9.3216951235009));
#23253=CARTESIAN_POINT('Ctrl Pts',(-8.31948777127265,-1.25737456087654,
9.36941714695573));
#23254=CARTESIAN_POINT('Ctrl Pts',(-7.34575754060823,-0.528193230805871,
9.41713917041061));
#23255=CARTESIAN_POINT('Ctrl Pts',(-7.4304786871105,0.685346344802941,9.46486119386546));
#23256=CARTESIAN_POINT('Ctrl Pts',(-8.49973262930053,1.27036662422184,9.51258321732033));
#23257=CARTESIAN_POINT('Ctrl Pts',(-9.38798818610006,0.7840961729928,9.55235157019938));
#23258=CARTESIAN_POINT('Ctrl Pts',(-9.61327428745144,0.0809103056341308,
9.58416625250263));
#23259=CARTESIAN_POINT('Ctrl Pts',(-9.49203055537855,-0.64746058131023,
9.61598093480587));
#23260=CARTESIAN_POINT('Ctrl Pts',(-8.6834200621885,-1.25705549289229,9.65574928768491));
#23261=CARTESIAN_POINT('Ctrl Pts',(-7.5408133482771,-0.832788339385354,
9.70347131113979));
#23262=CARTESIAN_POINT('Ctrl Pts',(-7.28151460673084,0.355748633899845,
9.75119333459464));
#23263=CARTESIAN_POINT('Ctrl Pts',(-8.13957862728818,1.21806070667769,9.79891535804951));
#23264=CARTESIAN_POINT('Ctrl Pts',(-9.33097191264403,0.960893912885614,
9.84663738150436));
#23265=CARTESIAN_POINT('Ctrl Pts',(-9.6845616175819,0.0119833762775842,
9.88640573438342));
#23266=CARTESIAN_POINT('Ctrl Pts',(-9.3948552845635,-0.66720321967679,9.91822041668666));
#23267=CARTESIAN_POINT('Ctrl Pts',(-8.82660658674435,-1.13870890250777,
9.9500350989899));
#23268=CARTESIAN_POINT('Ctrl Pts',(-7.81624711119259,-1.07066027220188,
9.98980345186896));
#23269=CARTESIAN_POINT('Ctrl Pts',(-7.22973604796101,-0.002223333057961,
10.0375254753238));
#23270=CARTESIAN_POINT('Ctrl Pts',(-7.81127521001297,1.06626540213459,10.0852474987787));
#23271=CARTESIAN_POINT('Ctrl Pts',(-9.02438159307564,1.15697856328588,10.1329695222335));
#23272=CARTESIAN_POINT('Ctrl Pts',(-9.75711790712465,0.182991800391184,
10.1806915456884));
#23273=CARTESIAN_POINT('Ctrl Pts',(-9.40366912726124,-0.765971236790376,
10.2204598985675));
#23274=CARTESIAN_POINT('Ctrl Pts',(-8.74020027325655,-1.09005960634535,
10.2522745808707));
#23275=CARTESIAN_POINT('Ctrl Pts',(-8.00196407609283,-1.0748441959899,10.2840892631739));
#23276=CARTESIAN_POINT('Ctrl Pts',(-7.28239915263251,-0.362325279153768,
10.323857616053));
#23277=CARTESIAN_POINT('Ctrl Pts',(-7.53790398833915,0.829425533369869,
10.3715796395079));
#23278=CARTESIAN_POINT('Ctrl Pts',(-8.67678457453722,1.25698486798276,10.4193016629627));
#23279=CARTESIAN_POINT('Ctrl Pts',(-9.65355201469891,0.531877053879621,
10.4670236864176));
#23280=CARTESIAN_POINT('Ctrl Pts',(-9.57042727050285,-0.684117599530743,
10.5147457098724));
#23281=CARTESIAN_POINT('Ctrl Pts',(-8.68224393873985,-1.17051995879944,
10.5545140627515));
#23282=CARTESIAN_POINT('Ctrl Pts',(-7.96844922392633,-0.981519174093803,
10.5863287450547));
#23283=CARTESIAN_POINT('Ctrl Pts',(-7.42011077084954,-0.487000082053453,
10.618143427358));
#23284=CARTESIAN_POINT('Ctrl Pts',(-7.34212352097922,0.522640881250568,
10.657911780237));
#23285=CARTESIAN_POINT('Ctrl Pts',(-8.31508734504523,1.25673496056136,10.7056338036919));
#23286=CARTESIAN_POINT('Ctrl Pts',(-9.45611263301509,0.834932558426621,
10.7533558271467));
#23287=CARTESIAN_POINT('Ctrl Pts',(-9.72037348998793,-0.352510987054788,
10.8010778506016));
#23288=CARTESIAN_POINT('Ctrl Pts',(-8.86191044830422,-1.21772421296126,
10.8487998740565));
#23289=CARTESIAN_POINT('Ctrl Pts',(-7.87197604037941,-1.00444797441067,
10.8885682269355));
#23290=CARTESIAN_POINT('Ctrl Pts',(-7.45582564786067,-0.394494662819061,
10.9203829092388));
#23291=CARTESIAN_POINT('Ctrl Pts',(-7.36469629318614,0.338253337677466,
10.952197591542));
#23292=CARTESIAN_POINT('Ctrl Pts',(-7.96630498329803,1.15282308294524,10.9919659444211));
#23293=CARTESIAN_POINT('Ctrl Pts',(-9.18241439302195,1.07139444055684,11.0396879678759));
#23294=CARTESIAN_POINT('Ctrl Pts',(-9.76934213251881,0.00585617149158359,
11.0874099913308));
#23295=CARTESIAN_POINT('Ctrl Pts',(-9.19227099350598,-1.06505226285372,
11.1351320147856));
#23296=CARTESIAN_POINT('Ctrl Pts',(-7.97696468603363,-1.1576983595773,11.1828540382405));
#23297=CARTESIAN_POINT('Ctrl Pts',(-7.36786565157653,-0.348714273116267,
11.2226223911196));
#23298=CARTESIAN_POINT('Ctrl Pts',(-7.45223013401734,0.38484337670927,11.2544370734228));
#23299=CARTESIAN_POINT('Ctrl Pts',(-7.86273483295154,0.99861050165816,11.286251755726));
#23300=CARTESIAN_POINT('Ctrl Pts',(-8.85065922194766,1.22101168769465,11.3260201086051));
#23301=CARTESIAN_POINT('Ctrl Pts',(-9.71706895636918,0.363756245997238,
11.3737421320599));
#23302=CARTESIAN_POINT('Ctrl Pts',(-9.46377577222247,-0.826075060154299,
11.4214641555148));
#23303=CARTESIAN_POINT('Ctrl Pts',(-8.32669098511707,-1.25838763360895,
11.4691861789697));
#23304=CARTESIAN_POINT('Ctrl Pts',(-7.34699516580216,-0.533302244267042,
11.5169082024245));
#23305=CARTESIAN_POINT('Ctrl Pts',(-7.41566323903509,0.477015320482895,
11.5566765553036));
#23306=CARTESIAN_POINT('Ctrl Pts',(-7.95941547151687,0.976572825867565,
11.5884912376068));
#23307=CARTESIAN_POINT('Ctrl Pts',(-8.67143590952399,1.17215167793291,11.6203059199101));
#23308=CARTESIAN_POINT('Ctrl Pts',(-9.56406941865381,0.693965203529443,
11.6600742727891));
#23309=CARTESIAN_POINT('Ctrl Pts',(-9.65841048613898,-0.521210702751624,
11.707796296244));
#23310=CARTESIAN_POINT('Ctrl Pts',(-8.68837512347985,-1.25530018600567,
11.7555183196989));
#23311=CARTESIAN_POINT('Ctrl Pts',(-7.54559797052453,-0.838267390032985,
11.8032403431537));
#23312=CARTESIAN_POINT('Ctrl Pts',(-7.27910784504458,0.351075173420432,
11.8509623666086));
#23313=CARTESIAN_POINT('Ctrl Pts',(-7.99206779629669,1.07020311324363,11.8907307194876));
#23314=CARTESIAN_POINT('Ctrl Pts',(-8.73013217658673,1.09222950791386,11.9225454017909));
#23315=CARTESIAN_POINT('Ctrl Pts',(-9.39656311872312,0.77427669556865,11.9543600840941));
#23316=CARTESIAN_POINT('Ctrl Pts',(-9.75875284033654,-0.171384708677798,
11.9941284369732));
#23317=CARTESIAN_POINT('Ctrl Pts',(-9.03503459701296,-1.15209089531113,
12.041850460428));
#23318=CARTESIAN_POINT('Ctrl Pts',(-7.8211428530551,-1.07257480772847,12.0895724838829));
#23319=CARTESIAN_POINT('Ctrl Pts',(-7.22976960704087,-0.00949736081689754,
12.1372945073378));
#23320=CARTESIAN_POINT('Ctrl Pts',(-7.80639734178506,1.06430577558381,12.1850165307926));
#23321=CARTESIAN_POINT('Ctrl Pts',(-8.81608592964515,1.14167399560278,12.2247848836717));
#23322=CARTESIAN_POINT('Ctrl Pts',(-9.38866097389678,0.67543155843589,12.2565995659749));
#23323=CARTESIAN_POINT('Ctrl Pts',(-9.68462176169229,-0.00105303385171488,
12.2884142482782));
#23324=CARTESIAN_POINT('Ctrl Pts',(-9.33980261183377,-0.953185713584225,
12.3281826011572));
#23325=CARTESIAN_POINT('Ctrl Pts',(-8.15083289505076,-1.22133442753447,
12.3759046246121));
#23326=CARTESIAN_POINT('Ctrl Pts',(-7.28484893342126,-0.366976333738949,
12.4236266480669));
#23327=CARTESIAN_POINT('Ctrl Pts',(-7.53317012442289,0.823902568724695,
12.4713486715218));
#23328=CARTESIAN_POINT('Ctrl Pts',(-8.67181352813447,1.25869438029009,12.5190706949767));
#23329=CARTESIAN_POINT('Ctrl Pts',(-9.48601427144361,0.656586387054127,
12.5588390478557));
#23330=CARTESIAN_POINT('Ctrl Pts',(-9.61397344810094,-0.0706347901844313,
12.590653730159));
#23331=CARTESIAN_POINT('Ctrl Pts',(-9.39518516300458,-0.775869416262637,
12.6224684124622));
#23332=CARTESIAN_POINT('Ctrl Pts',(-8.51145418725852,-1.27031501330109,
12.6622367653413));
#23333=CARTESIAN_POINT('Ctrl Pts',(-7.43684783790457,-0.695185537314625,
12.7099587887961));
#23334=CARTESIAN_POINT('Ctrl Pts',(-7.34093308882888,0.517520665829057,
12.757680812251));
#23335=CARTESIAN_POINT('Ctrl Pts',(-8.30789378535402,1.25565546761602,12.8054028357058));
#23336=CARTESIAN_POINT('Ctrl Pts',(-9.45347176054575,0.839477833695256,
12.8531248591607));
#23337=CARTESIAN_POINT('Ctrl Pts',(-9.67526720411315,-0.148582724740579,
12.8928932120397));
#23338=CARTESIAN_POINT('Ctrl Pts',(-9.29623126434288,-0.782267147681163,
12.924707894343));
#23339=CARTESIAN_POINT('Ctrl Pts',(-8.66935174234859,-1.17245461085654,
12.9565225766462));
#23340=CARTESIAN_POINT('Ctrl Pts',(-7.67752192246292,-0.968174180297535,
12.9962909295253));
#23341=CARTESIAN_POINT('Ctrl Pts',(-7.24114239930117,0.169861685563191,
13.0440129529802));
#23342=CARTESIAN_POINT('Ctrl Pts',(-7.96205466597611,1.14972977770164,13.091734976435));
#23343=CARTESIAN_POINT('Ctrl Pts',(-9.1762679501323,1.07528466495317,13.1394569998899));
#23344=CARTESIAN_POINT('Ctrl Pts',(-9.77031884177337,0.0110214182135979,
13.1871790233447));
#23345=CARTESIAN_POINT('Ctrl Pts',(-9.29158517982126,-0.881318744974018,
13.2269473762238));
#23346=CARTESIAN_POINT('Ctrl Pts',(-8.59033162705337,-1.11254946578217,
13.258762058527));
#23347=CARTESIAN_POINT('Ctrl Pts',(-7.86096047197614,-0.997475969022965,
13.2905767408303));
#23348=CARTESIAN_POINT('Ctrl Pts',(-7.24454225832378,-0.194054864121289,
13.3303450937093));
#23349=CARTESIAN_POINT('Ctrl Pts',(-7.65912168086415,0.952102464794035,
13.3780671171642));
#23350=CARTESIAN_POINT('Ctrl Pts',(-8.84542102092192,1.22145325839232,13.425789140619));
#23351=CARTESIAN_POINT('Ctrl Pts',(-9.71496598037074,0.370719729177345,
13.4735111640739));
#23352=CARTESIAN_POINT('Ctrl Pts',(-9.46789392392579,-0.822807865453071,
13.5212331875287));
#23353=CARTESIAN_POINT('Ctrl Pts',(-8.52201063734719,-1.18441772994109,
13.5610015404078));
#23354=CARTESIAN_POINT('Ctrl Pts',(-7.84039592147494,-0.900471307844614,
13.592816222711));
#23355=CARTESIAN_POINT('Ctrl Pts',(-7.36409672760257,-0.336234416608623,
13.6246309050143));
#23356=CARTESIAN_POINT('Ctrl Pts',(-7.42358990565628,0.674664909580162,
13.6643992578934));
#23357=CARTESIAN_POINT('Ctrl Pts',(-8.48702355866553,1.2701996154266,13.7121212813482));
#23358=CARTESIAN_POINT('Ctrl Pts',(-9.56039692213696,0.697726387385763,
13.7598433048031));
#23359=CARTESIAN_POINT('Ctrl Pts',(-9.66137616386497,-0.514568612592982,
13.8075653282579));
#23360=CARTESIAN_POINT('Ctrl Pts',(-8.69362714602554,-1.25552377904438,
13.8552873517128));
#23361=CARTESIAN_POINT('Ctrl Pts',(-7.74170605534076,-0.910120937375022,
13.8950557045919));
#23362=CARTESIAN_POINT('Ctrl Pts',(-7.41201282369385,-0.249419367434961,
13.9268703868951));
#23363=CARTESIAN_POINT('Ctrl Pts',(-7.42097828489804,0.48891918094274,13.9586850691983));
#23364=CARTESIAN_POINT('Ctrl Pts',(-8.12738032545558,1.21449002036506,13.9984534220774));
#23365=CARTESIAN_POINT('Ctrl Pts',(-9.3212513654399,0.969082889036178,14.0461754455323));
#23366=CARTESIAN_POINT('Ctrl Pts',(-9.75843636599122,-0.166137463814466,
14.0938974689871));
#23367=CARTESIAN_POINT('Ctrl Pts',(-9.04162318026726,-1.14900817301567,
14.141619492442));
#23368=CARTESIAN_POINT('Ctrl Pts',(-7.8249684203312,-1.07618018838563,14.1893415158968));
#23369=CARTESIAN_POINT('Ctrl Pts',(-7.33106473546485,-0.192146232024756,
14.2291098687759));
#23370=CARTESIAN_POINT('Ctrl Pts',(-7.51401624895191,0.523222858185244,
14.2609245510791));
#23371=CARTESIAN_POINT('Ctrl Pts',(-8.00387576243607,1.07572792473592,14.2927392333824));
#23372=CARTESIAN_POINT('Ctrl Pts',(-9.01282036199793,1.16225931174772,14.3325075862614));
#23373=CARTESIAN_POINT('Ctrl Pts',(-9.75512458555882,0.195544689997601,
14.3802296097163));
#23374=CARTESIAN_POINT('Ctrl Pts',(-9.34299643880091,-0.949010404736995,
14.4279516331711));
#23375=CARTESIAN_POINT('Ctrl Pts',(-8.15783249325345,-1.2233138797493,14.475673656626));
#23376=CARTESIAN_POINT('Ctrl Pts',(-7.28538310678412,-0.372205902886431,
14.5233956800809));
#23377=CARTESIAN_POINT('Ctrl Pts',(-7.49027159406131,0.619498485376649,
14.5631640329599));
#23378=CARTESIAN_POINT('Ctrl Pts',(-8.09668020484303,1.04079741520829,14.5949787152632));
#23379=CARTESIAN_POINT('Ctrl Pts',(-8.82863051099968,1.13812644920796,14.6267933975664));
#23380=CARTESIAN_POINT('Ctrl Pts',(-9.64826387771769,0.543434907327214,
14.6665617504455));
#23381=CARTESIAN_POINT('Ctrl Pts',(-9.57713290565078,-0.673320246814625,
14.7142837739003));
#23382=CARTESIAN_POINT('Ctrl Pts',(-8.51660134601078,-1.26924707575363,
14.7620057973552));
#23383=CARTESIAN_POINT('Ctrl Pts',(-7.44084619358963,-0.701262194326865,
14.8097278208101));
#23384=CARTESIAN_POINT('Ctrl Pts',(-7.33791546196855,0.51321628861147,14.8574498442649));
#23385=CARTESIAN_POINT('Ctrl Pts',(-8.14171434546497,1.12914180496267,14.897218197144));
#23386=CARTESIAN_POINT('Ctrl Pts',(-8.87595988159389,1.05099014478143,14.9290328794472));
#23387=CARTESIAN_POINT('Ctrl Pts',(-9.49318006986067,0.645695886996565,
14.9608475617504));
#23388=CARTESIAN_POINT('Ctrl Pts',(-9.72393637462547,-0.340310403119495,
15.0006159146295));
#23389=CARTESIAN_POINT('Ctrl Pts',(-8.87404609450619,-1.21394603873967,
15.0483379380843));
#23390=CARTESIAN_POINT('Ctrl Pts',(-7.68211319459765,-0.970734219451872,
15.0960599615392));
#23391=CARTESIAN_POINT('Ctrl Pts',(-7.24019036465419,0.162650140326822,
15.1437819849941));
#23392=CARTESIAN_POINT('Ctrl Pts',(-7.95695626426865,1.14844897424003,15.1915040084489));
#23393=CARTESIAN_POINT('Ctrl Pts',(-8.9678190573545,1.08833594701761,15.231272361328));
#23394=CARTESIAN_POINT('Ctrl Pts',(-9.47196150163588,0.548832220338601,
15.2630870436313));
#23395=CARTESIAN_POINT('Ctrl Pts',(-9.67356121121295,-0.161507282602432,
15.2949017259345));
#23396=CARTESIAN_POINT('Ctrl Pts',(-9.20294744217587,-1.05815633227,15.3346700788135));
#23397=CARTESIAN_POINT('Ctrl Pts',(-7.98861526120894,-1.16278173533498,
15.3823921022684));
#23398=CARTESIAN_POINT('Ctrl Pts',(-7.24633766496125,-0.198993896651544,
15.4301141257232));
#23399=CARTESIAN_POINT('Ctrl Pts',(-7.65368670603976,0.947269754286983,
15.4778361491781));
#23400=CARTESIAN_POINT('Ctrl Pts',(-8.84072065488431,1.22382409746114,15.525558172633));
#23401=CARTESIAN_POINT('Ctrl Pts',(-9.56587666344393,0.516967103108893,
15.565326525512));
#23402=CARTESIAN_POINT('Ctrl Pts',(-9.59412288800059,-0.220869169870519,
15.5971412078153));
#23403=CARTESIAN_POINT('Ctrl Pts',(-9.28187668594746,-0.889997654174282,
15.6289558901185));
#23404=CARTESIAN_POINT('Ctrl Pts',(-8.3391963985811,-1.26011363586197,15.6687242429976));
#23405=CARTESIAN_POINT('Ctrl Pts',(-7.35261511400304,-0.544843601675332,
15.7164462664524));
#23406=CARTESIAN_POINT('Ctrl Pts',(-7.42146958197941,0.669890693554228,
15.7641682899073));
#23407=CARTESIAN_POINT('Ctrl Pts',(-8.48021464548925,1.26984600438468,15.8118903133622));
#23408=CARTESIAN_POINT('Ctrl Pts',(-9.55750298236283,0.703085044786402,
15.859612336817));
#23409=CARTESIAN_POINT('Ctrl Pts',(-9.66331880274563,-0.509245030498203,
15.9073343602719));
#23410=CARTESIAN_POINT('Ctrl Pts',(-8.70050979592311,-1.25407183081503,
15.9550563837268));
#23411=CARTESIAN_POINT('Ctrl Pts',(-7.55383452636763,-0.846612249150831,
16.0027784071816));
#23412=CARTESIAN_POINT('Ctrl Pts',(-7.27557316343251,0.33782473088005,16.0505004306365));
#23413=CARTESIAN_POINT('Ctrl Pts',(-8.1233181103483,1.21320028335102,16.0982224540913));
#23414=CARTESIAN_POINT('Ctrl Pts',(-9.1158648858804,1.01199674841544,16.1379908069704));
#23415=CARTESIAN_POINT('Ctrl Pts',(-9.53931342581282,0.407081917028108,
16.1698054892736));
#23416=CARTESIAN_POINT('Ctrl Pts',(-9.63932163954313,-0.324490753396568,
16.2016201715769));
#23417=CARTESIAN_POINT('Ctrl Pts',(-9.04759131286806,-1.14628955341257,
16.2413885244559));
#23418=CARTESIAN_POINT('Ctrl Pts',(-7.8305950534041,-1.07956620750823,16.2891105479108));
#23419=CARTESIAN_POINT('Ctrl Pts',(-7.2308199229778,-0.0212073876117485,
16.3368325713657));
#23420=CARTESIAN_POINT('Ctrl Pts',(-7.79490064728529,1.05660333990498,16.3845545948205));
#23421=CARTESIAN_POINT('Ctrl Pts',(-9.00899631826399,1.16393843392956,16.4322766182754));
#23422=CARTESIAN_POINT('Ctrl Pts',(-9.62783474663535,0.362380053368341,
16.4720449711544));
#23423=CARTESIAN_POINT('Ctrl Pts',(-9.55234712077239,-0.372144466768089,
16.5038596534577));
#23424=CARTESIAN_POINT('Ctrl Pts',(-9.14929499916242,-0.990830867533636,
16.5356743357609));
#23425=CARTESIAN_POINT('Ctrl Pts',(-8.16413226770568,-1.22516301435909,
16.5754426886399));
#23426=CARTESIAN_POINT('Ctrl Pts',(-7.28741902604588,-0.378447839289557,
16.6231647120948));
#23427=CARTESIAN_POINT('Ctrl Pts',(-7.52630483397695,0.814359548927526,
16.6708867355497));
#23428=CARTESIAN_POINT('Ctrl Pts',(-8.65807846404219,1.26039147291354,16.7186087590046));
#23429=CARTESIAN_POINT('Ctrl Pts',(-9.64647120733396,0.54720671629367,16.7663307824594));
#23430=CARTESIAN_POINT('Ctrl Pts',(-9.59002609357546,-0.463867378651884,
16.8060991353385));
#23431=CARTESIAN_POINT('Ctrl Pts',(-9.0523548496622,-0.969964039050123,
16.8379138176417));
#23432=CARTESIAN_POINT('Ctrl Pts',(-8.34275164585083,-1.17413916597537,
16.869728499945));
#23433=CARTESIAN_POINT('Ctrl Pts',(-7.44440062377225,-0.706782420080965,
16.909496852824));
#23434=CARTESIAN_POINT('Ctrl Pts',(-7.33537113793291,0.507163745220385,
16.9572188762789));
#23435=CARTESIAN_POINT('Ctrl Pts',(-8.29645810449297,1.25293034154812,17.0049408997337));
#23436=CARTESIAN_POINT('Ctrl Pts',(-9.44419493667808,0.849747828922038,
17.0526629231886));
#23437=CARTESIAN_POINT('Ctrl Pts',(-9.72504848574826,-0.336285056074205,
17.1003849466434));
#23438=CARTESIAN_POINT('Ctrl Pts',(-9.02083719942392,-1.0639823489339,17.1401532995225));
#23439=CARTESIAN_POINT('Ctrl Pts',(-8.28309315876083,-1.09493266409099,
17.1719679818257));
#23440=CARTESIAN_POINT('Ctrl Pts',(-7.61286589490514,-0.785062358491983,
17.203782664129));
#23441=CARTESIAN_POINT('Ctrl Pts',(-7.23926662306685,0.156149875810646,
17.243551017008));
#23442=CARTESIAN_POINT('Ctrl Pts',(-7.95107210703395,1.14553638937586,17.2912730404629));
#23443=CARTESIAN_POINT('Ctrl Pts',(-9.16583668605209,1.08070590432238,17.3389950639178));
#23444=CARTESIAN_POINT('Ctrl Pts',(-9.77002265432594,0.024857766580027,
17.3867170873726));
#23445=CARTESIAN_POINT('Ctrl Pts',(-9.20642275932966,-1.05584009988493,
17.4344391108275));
#23446=CARTESIAN_POINT('Ctrl Pts',(-8.19774363120575,-1.14541298869811,
17.4742074637065));
#23447=CARTESIAN_POINT('Ctrl Pts',(-7.61957211175687,-0.686128887500105,
17.5060221460098));
#23448=CARTESIAN_POINT('Ctrl Pts',(-7.31545212919699,-0.013272864473688,
17.537836828313));
#23449=CARTESIAN_POINT('Ctrl Pts',(-7.64873177068013,0.942960144001058,
17.5776051811921));
#23450=CARTESIAN_POINT('Ctrl Pts',(-8.83437177863538,1.22546765143426,17.6253272046469));
#23451=CARTESIAN_POINT('Ctrl Pts',(-9.7106243049545,0.38164451572817,17.6730492281018));
#23452=CARTESIAN_POINT('Ctrl Pts',(-9.47672276235654,-0.812150291851311,
17.7207712515566));
#23453=CARTESIAN_POINT('Ctrl Pts',(-8.34342062912157,-1.26068010694196,
17.7684932750115));
#23454=CARTESIAN_POINT('Ctrl Pts',(-7.52199803547846,-0.668462403241392,
17.8082616278906));
#23455=CARTESIAN_POINT('Ctrl Pts',(-7.38525381327406,0.0571581651059841,
17.8400763101938));
#23456=CARTESIAN_POINT('Ctrl Pts',(-7.59549758383178,0.764987062832501,
17.8718909924971));
#23457=CARTESIAN_POINT('Ctrl Pts',(-8.47318452674403,1.27008360426311,17.9116593453761));
#23458=CARTESIAN_POINT('Ctrl Pts',(-9.55466742874301,0.707991571848307,
17.959381368831));
#23459=CARTESIAN_POINT('Ctrl Pts',(-9.66524061504402,-0.50346603975217,
18.0071033922858));
#23460=CARTESIAN_POINT('Ctrl Pts',(-8.70727701023286,-1.25324047656007,
18.0548254157407));
#23461=CARTESIAN_POINT('Ctrl Pts',(-7.55674990236037,-0.850946934142607,
18.1025474391955));
#23462=CARTESIAN_POINT('Ctrl Pts',(-7.32302190246604,0.134359164483167,
18.1423157920746));
#23463=CARTESIAN_POINT('Ctrl Pts',(-7.69436687770133,0.772580991814832,
18.1741304743778));
#23464=CARTESIAN_POINT('Ctrl Pts',(-8.31648195947549,1.17032087734831,18.2059451566811));
#23465=CARTESIAN_POINT('Ctrl Pts',(-9.31070964793652,0.978049742173947,
18.2457135095601));
#23466=CARTESIAN_POINT('Ctrl Pts',(-9.76081971146936,-0.154625697184869,
18.293435533015));
#23467=CARTESIAN_POINT('Ctrl Pts',(-9.05180986375601,-1.14314024441165,
18.3411575564698));
#23468=CARTESIAN_POINT('Ctrl Pts',(-7.83678509216389,-1.0833842518163,18.3888795799247));
#23469=CARTESIAN_POINT('Ctrl Pts',(-7.22990733399897,-0.0263827821555435,
18.4366016033796));
#23470=CARTESIAN_POINT('Ctrl Pts',(-7.69781477559553,0.871681531812165,
18.4763699562586));
#23471=CARTESIAN_POINT('Ctrl Pts',(-8.39622073897505,1.11137571578626,18.5081846385619));
#23472=CARTESIAN_POINT('Ctrl Pts',(-9.12693016111688,1.00513103635158,18.5399993208651));
#23473=CARTESIAN_POINT('Ctrl Pts',(-9.75301919974774,0.209223126081749,
18.5797676737442));
#23474=CARTESIAN_POINT('Ctrl Pts',(-9.35233075805922,-0.941863965722109,
18.627489697199));
#23475=CARTESIAN_POINT('Ctrl Pts',(-8.16937546850047,-1.2255411716065,18.6752117206539));
#23476=CARTESIAN_POINT('Ctrl Pts',(-7.28960603720165,-0.385385399153776,
18.7229337441087));
#23477=CARTESIAN_POINT('Ctrl Pts',(-7.52222650552583,0.811042800922165,
18.7706557675636));
#23478=CARTESIAN_POINT('Ctrl Pts',(-8.4636676182458,1.18406494128967,18.8104241204426));
#23479=CARTESIAN_POINT('Ctrl Pts',(-9.14866630079203,0.90838215904711,18.8422388027459));
#23480=CARTESIAN_POINT('Ctrl Pts',(-9.63175407270726,0.34994649028926,18.8740534850491));
#23481=CARTESIAN_POINT('Ctrl Pts',(-9.5844902130829,-0.661598374507747,
18.9138218379282));
#23482=CARTESIAN_POINT('Ctrl Pts',(-8.52833622049212,-1.26994980596393,
18.9615438613831));
#23483=CARTESIAN_POINT('Ctrl Pts',(-7.44811833664692,-0.710498916560375,
19.0092658848379));
#23484=CARTESIAN_POINT('Ctrl Pts',(-7.33248600078022,0.500486276220874,
19.0569879082928));
#23485=CARTESIAN_POINT('Ctrl Pts',(-8.29120376213664,1.25309040475059,19.1047099317477));
#23486=CARTESIAN_POINT('Ctrl Pts',(-9.24723225571495,0.9192245553587,19.1444782846267));
#23487=CARTESIAN_POINT('Ctrl Pts',(-9.58489134881782,0.262558332411264,
19.17629296693));
#23488=CARTESIAN_POINT('Ctrl Pts',(-9.58485538992238,-0.475834645766379,
19.2081076492332));
#23489=CARTESIAN_POINT('Ctrl Pts',(-8.8872794497266,-1.20989506125256,19.2478760021122));
#23490=CARTESIAN_POINT('Ctrl Pts',(-7.6905279636182,-0.978943549636808,
19.2955980255671));
#23491=CARTESIAN_POINT('Ctrl Pts',(-7.23964653004754,0.150906841828665,
19.343320049022));
#23492=CARTESIAN_POINT('Ctrl Pts',(-7.94452128542435,1.14237421570735,19.3910420724768));
#23493=CARTESIAN_POINT('Ctrl Pts',(-9.16196779807331,1.08426475813698,19.4387640959317));
#23494=CARTESIAN_POINT('Ctrl Pts',(-9.66652613095242,0.206268303334325,
19.4785324488107));
#23495=CARTESIAN_POINT('Ctrl Pts',(-9.49223906914536,-0.511260937604133,
19.510347131114));
#23496=CARTESIAN_POINT('Ctrl Pts',(-9.00909690916197,-1.06964955206693,
19.5421618134172));
#23497=CARTESIAN_POINT('Ctrl Pts',(-8.00127252658247,-1.16837594064688,
19.5819301662963));
#23498=CARTESIAN_POINT('Ctrl Pts',(-7.24733194871174,-0.210708814104341,
19.6296521897511));
#23499=CARTESIAN_POINT('Ctrl Pts',(-7.64558866994153,0.938746517010665,
19.677374213206));
#23500=CARTESIAN_POINT('Ctrl Pts',(-8.82734875444545,1.22736231163525,19.7250962366608));
#23501=CARTESIAN_POINT('Ctrl Pts',(-9.71002692863045,0.386867242620788,
19.7728182601158));
#23502=CARTESIAN_POINT('Ctrl Pts',(-9.51714626434415,-0.607242376721195,
19.8125866129947));
#23503=CARTESIAN_POINT('Ctrl Pts',(-8.91587683280376,-1.03584389586241,
19.8444012952981));
#23504=CARTESIAN_POINT('Ctrl Pts',(-8.18515706613851,-1.1420174053633,19.8762159776012));
#23505=CARTESIAN_POINT('Ctrl Pts',(-7.35839193464024,-0.557281308254152,
19.9159843304804));
#23506=CARTESIAN_POINT('Ctrl Pts',(-7.41480328973932,0.660245068969852,
19.9637063539351));
#23507=CARTESIAN_POINT('Ctrl Pts',(-8.46805065902489,1.26895349944085,20.0114283773901));
#23508=CARTESIAN_POINT('Ctrl Pts',(-9.5505958796237,0.714019431652471,20.0591504008449));
#23509=CARTESIAN_POINT('Ctrl Pts',(-9.6682059673661,-0.499125484456667,
20.1068724242998));
#23510=CARTESIAN_POINT('Ctrl Pts',(-8.87191434881798,-1.12472643087044,
20.1466407771788));
#23511=CARTESIAN_POINT('Ctrl Pts',(-8.13677740234172,-1.05545983401012,
20.1784554594821));
#23512=CARTESIAN_POINT('Ctrl Pts',(-7.51470106247534,-0.657659357774231,
20.2102701417853));
#23513=CARTESIAN_POINT('Ctrl Pts',(-7.27203769305019,0.325484260962615,
20.2500384946644));
#23514=CARTESIAN_POINT('Ctrl Pts',(-8.11130082014058,1.20933386566167,20.2977605181192));
#23515=CARTESIAN_POINT('Ctrl Pts',(-9.30608773965546,0.980554078115584,
20.3454825415741));
#23516=CARTESIAN_POINT('Ctrl Pts',(-9.76168449057688,-0.147403179400575,
20.3932045650289));
#23517=CARTESIAN_POINT('Ctrl Pts',(-9.05689235516024,-1.14179785259385,
20.4409265884838));
#23518=CARTESIAN_POINT('Ctrl Pts',(-8.04537665815608,-1.09391381936874,
20.4806949413629));
#23519=CARTESIAN_POINT('Ctrl Pts',(-7.53474657604769,-0.560546112471273,
20.5125096236661));
#23520=CARTESIAN_POINT('Ctrl Pts',(-7.32457174740621,0.147303259161259,
20.5443243059694));
#23521=CARTESIAN_POINT('Ctrl Pts',(-7.78430692110201,1.04957841452719,20.5840926588484));
#23522=CARTESIAN_POINT('Ctrl Pts',(-8.99728661934093,1.16888043412664,20.6318146823032));
#23523=CARTESIAN_POINT('Ctrl Pts',(-9.7511624004973,0.214141055647227,20.6795367057581));
#23524=CARTESIAN_POINT('Ctrl Pts',(-9.35771029132173,-0.936967719412176,
20.727258729213));
#23525=CARTESIAN_POINT('Ctrl Pts',(-8.17409741818057,-1.22785135036264,
20.7749807526679));
#23526=CARTESIAN_POINT('Ctrl Pts',(-7.440464827453,-0.529825485694162,20.8147491055469));
#23527=CARTESIAN_POINT('Ctrl Pts',(-7.40327038360504,0.207630116265646,
20.8465637878501));
#23528=CARTESIAN_POINT('Ctrl Pts',(-7.70745589936328,0.880456515508389,
20.8783784701534));
#23529=CARTESIAN_POINT('Ctrl Pts',(-8.6454717721415,1.26201006134416,20.9181468230324));
#23530=CARTESIAN_POINT('Ctrl Pts',(-9.64084849413286,0.55860555358354,20.9658688464873));
#23531=CARTESIAN_POINT('Ctrl Pts',(-9.58630370016657,-0.65666430932124,
21.0135908699422));
#23532=CARTESIAN_POINT('Ctrl Pts',(-8.53560802117004,-1.2697667186881,21.061312893397));
#23533=CARTESIAN_POINT('Ctrl Pts',(-7.45017782549272,-0.715335469088922,
21.1090349168518));
#23534=CARTESIAN_POINT('Ctrl Pts',(-7.35206935690855,0.29254925364273,21.1488032697309));
#23535=CARTESIAN_POINT('Ctrl Pts',(-7.8064425956856,0.87458804221129,21.1806179520342));
#23536=CARTESIAN_POINT('Ctrl Pts',(-8.47670003703183,1.18439306772749,21.2124326343374));
#23537=CARTESIAN_POINT('Ctrl Pts',(-9.43572010035171,0.859220184365848,
21.2522009872165));
#23538=CARTESIAN_POINT('Ctrl Pts',(-9.72825430450134,-0.323985824587268,
21.2999230106713));
#23539=CARTESIAN_POINT('Ctrl Pts',(-8.89187916023458,-1.20735018445592,
21.3476450341262));
#23540=CARTESIAN_POINT('Ctrl Pts',(-7.69614707717368,-0.983562875226182,
21.395367057581));
#23541=CARTESIAN_POINT('Ctrl Pts',(-7.23803957092387,0.145901702765443,
21.4430890810359));
#23542=CARTESIAN_POINT('Ctrl Pts',(-7.8232824513717,0.97230817467188,21.4828574339149));
#23543=CARTESIAN_POINT('Ctrl Pts',(-8.54771943639906,1.11519010578827,21.5146721162182));
#23544=CARTESIAN_POINT('Ctrl Pts',(-9.25730275191042,0.910945865078809,
21.5464867985214));
#23545=CARTESIAN_POINT('Ctrl Pts',(-9.76981109383267,0.0375661736593354,
21.5862551514005));
#23546=CARTESIAN_POINT('Ctrl Pts',(-9.21689429836074,-1.04863626488762,
21.6339771748553));
#23547=CARTESIAN_POINT('Ctrl Pts',(-8.00641613218915,-1.16946086277772,
21.6816991983102));
#23548=CARTESIAN_POINT('Ctrl Pts',(-7.24855909460346,-0.217878662011405,
21.7294212217651));
#23549=CARTESIAN_POINT('Ctrl Pts',(-7.64109864474925,0.936012763466559,
21.7771432452199));
#23550=CARTESIAN_POINT('Ctrl Pts',(-8.62439085665566,1.17807331772505,21.816911598099));
#23551=CARTESIAN_POINT('Ctrl Pts',(-9.26573336877662,0.812144398860403,
21.8487262804022));
#23552=CARTESIAN_POINT('Ctrl Pts',(-9.66872540454101,0.193418602868739,
21.8805409627055));
#23553=CARTESIAN_POINT('Ctrl Pts',(-9.48487761198751,-0.802401097226132,
21.9203093155845));
#23554=CARTESIAN_POINT('Ctrl Pts',(-8.3560530827218,-1.26208349013278,21.9680313390394));
#23555=CARTESIAN_POINT('Ctrl Pts',(-7.36157196177148,-0.561467136978719,
22.0157533624943));
#23556=CARTESIAN_POINT('Ctrl Pts',(-7.41104024249466,0.654019951984267,
22.0634753859491));
#23557=CARTESIAN_POINT('Ctrl Pts',(-8.46286642522661,1.26982381811353,22.111197409404));
#23558=CARTESIAN_POINT('Ctrl Pts',(-9.36485954540964,0.809535542066614,
22.150965762283));
#23559=CARTESIAN_POINT('Ctrl Pts',(-9.61045736917226,0.113183691004152,
22.1827804445863));
#23560=CARTESIAN_POINT('Ctrl Pts',(-9.510402184057,-0.6183989437314,22.2145951268895));
#23561=CARTESIAN_POINT('Ctrl Pts',(-8.71982283494963,-1.25120316202389,
22.2543634797686));
#23562=CARTESIAN_POINT('Ctrl Pts',(-7.56538503329298,-0.860273395535878,
22.3020855032234));
#23563=CARTESIAN_POINT('Ctrl Pts',(-7.27170389959832,0.320238089349084,
22.3498075266783));
#23564=CARTESIAN_POINT('Ctrl Pts',(-8.10438204030062,1.20708818278655,22.3975295501332));
#23565=CARTESIAN_POINT('Ctrl Pts',(-9.30273657679897,0.984604194431938,
22.445251573588));
#23566=CARTESIAN_POINT('Ctrl Pts',(-9.68371494937798,0.0463545658411376,
22.485019926467));
#23567=CARTESIAN_POINT('Ctrl Pts',(-9.41384077673285,-0.640953314554658,
22.5168346087703));
#23568=CARTESIAN_POINT('Ctrl Pts',(-8.85951460900709,-1.12875111209944,
22.5486492910735));
#23569=CARTESIAN_POINT('Ctrl Pts',(-7.8476058857349,-1.09005199467554,22.5884176439526));
#23570=CARTESIAN_POINT('Ctrl Pts',(-7.23033557328084,-0.0390857337598358,
22.6361396674074));
#23571=CARTESIAN_POINT('Ctrl Pts',(-7.78062202915808,1.04582937384607,22.6838616908624));
#23572=CARTESIAN_POINT('Ctrl Pts',(-8.99058496612945,1.17170894084981,22.7315837143172));
#23573=CARTESIAN_POINT('Ctrl Pts',(-9.75127797821979,0.219396564800193,
22.7793057377721));
#23574=CARTESIAN_POINT('Ctrl Pts',(-9.42551717667043,-0.739423953387505,
22.8190740906511));
#23575=CARTESIAN_POINT('Ctrl Pts',(-8.77173287452605,-1.08262983589042,
22.8508887729544));
#23576=CARTESIAN_POINT('Ctrl Pts',(-8.03336604963158,-1.08884460944564,
22.8827034552576));
#23577=CARTESIAN_POINT('Ctrl Pts',(-7.29342673462276,-0.397507719045549,
22.9224718081366));
#23578=CARTESIAN_POINT('Ctrl Pts',(-7.51423908935107,0.801155963652635,
22.9701938315915));
#23579=CARTESIAN_POINT('Ctrl Pts',(-8.64023214205648,1.26158578402983,23.0179158550463));
#23580=CARTESIAN_POINT('Ctrl Pts',(-9.63763097898426,0.565129371661826,
23.0656378785012));
#23581=CARTESIAN_POINT('Ctrl Pts',(-9.58982967509586,-0.652765433141446,
23.1133599019561));
#23582=CARTESIAN_POINT('Ctrl Pts',(-8.71613592676988,-1.16473820591349,
23.1531282548351));
#23583=CARTESIAN_POINT('Ctrl Pts',(-7.99715700058761,-0.996531502061154,
23.1849429371384));
#23584=CARTESIAN_POINT('Ctrl Pts',(-7.43469844210718,-0.518133590791431,
23.2167576194416));
#23585=CARTESIAN_POINT('Ctrl Pts',(-7.32744403743226,0.488818929738514,
23.2565259723207));
#23586=CARTESIAN_POINT('Ctrl Pts',(-8.27869450284539,1.25083944932543,23.3042479957755));
#23587=CARTESIAN_POINT('Ctrl Pts',(-9.43148001699525,0.862327502791391,
23.3519700192304));
#23588=CARTESIAN_POINT('Ctrl Pts',(-9.73008944468282,-0.316947013141832,
23.3996920426852));
#23589=CARTESIAN_POINT('Ctrl Pts',(-8.89709664300896,-1.20670861749425,
23.4474140661402));
#23590=CARTESIAN_POINT('Ctrl Pts',(-7.90138984794499,-1.02225031817649,
23.4871824190191));
#23591=CARTESIAN_POINT('Ctrl Pts',(-7.46771374944203,-0.424630679022691,
23.5189971013225));
#23592=CARTESIAN_POINT('Ctrl Pts',(-7.35535826930249,0.305164112406859,
23.5508117836256));
#23593=CARTESIAN_POINT('Ctrl Pts',(-7.93307458495534,1.13684959656076,23.5905801365048));
#23594=CARTESIAN_POINT('Ctrl Pts',(-9.15103487649505,1.09074701037714,23.6383021599595));
#23595=CARTESIAN_POINT('Ctrl Pts',(-9.76863756968231,0.0426902907282275,
23.6860241834145));
#23596=CARTESIAN_POINT('Ctrl Pts',(-9.22288747522111,-1.04451383390937,
23.7337462068693));
#23597=CARTESIAN_POINT('Ctrl Pts',(-8.01078163460585,-1.17238936466728,
23.7814682303242));
#23598=CARTESIAN_POINT('Ctrl Pts',(-7.3784622428289,-0.381422189174766,
23.8212365832032));
#23599=CARTESIAN_POINT('Ctrl Pts',(-7.44150318994769,0.354274780032955,
23.8530512655065));
#23600=CARTESIAN_POINT('Ctrl Pts',(-7.83402333855529,0.979696337426145,
23.8848659478097));
#23601=CARTESIAN_POINT('Ctrl Pts',(-8.81507750731556,1.23067363496897,23.9246343006888));
#23602=CARTESIAN_POINT('Ctrl Pts',(-9.70600007142817,0.398922647608368,
23.9723563241436));
#23603=CARTESIAN_POINT('Ctrl Pts',(-9.48734273227305,-0.797758154555304,
24.0200783475985));
#23604=CARTESIAN_POINT('Ctrl Pts',(-8.3632826623428,-1.2628870973462,24.0678003710533));
#23605=CARTESIAN_POINT('Ctrl Pts',(-7.36295733039398,-0.566538082496778,
24.1155223945082));
#23606=CARTESIAN_POINT('Ctrl Pts',(-7.40227684611156,0.445346723994319,
24.1552907473872));
#23607=CARTESIAN_POINT('Ctrl Pts',(-7.93130279579168,0.960473636589752,
24.1871054296905));
#23608=CARTESIAN_POINT('Ctrl Pts',(-8.63734760745799,1.17663310419213,24.2189201119937));
#23609=CARTESIAN_POINT('Ctrl Pts',(-9.54348223731444,0.724552449332103,
24.2586884648728));
#23610=CARTESIAN_POINT('Ctrl Pts',(-9.67304824068325,-0.487373856592171,
24.3064104883276));
#23611=CARTESIAN_POINT('Ctrl Pts',(-8.72472486990299,-1.24930479746899,
24.3541325117826));
#23612=CARTESIAN_POINT('Ctrl Pts',(-7.57032664362157,-0.865611287761247,
24.4018545352373));
#23613=CARTESIAN_POINT('Ctrl Pts',(-7.26943377642353,0.315496752466079,
24.4495765586923));
#23614=CARTESIAN_POINT('Ctrl Pts',(-7.96122419684737,1.05501206679947,24.4893449115713));
#23615=CARTESIAN_POINT('Ctrl Pts',(-8.69833851192349,1.09844797389147,24.5211595938745));
#23616=CARTESIAN_POINT('Ctrl Pts',(-9.37371582986139,0.79996904677923,24.5529742761777));
#23617=CARTESIAN_POINT('Ctrl Pts',(-9.76319630647174,-0.134783243543247,
24.5927426290568));
#23618=CARTESIAN_POINT('Ctrl Pts',(-9.06824318291268,-1.13607884239293,
24.6404646525116));
#23619=CARTESIAN_POINT('Ctrl Pts',(-7.85255512587106,-1.09182364834989,
24.6881866759666));
#23620=CARTESIAN_POINT('Ctrl Pts',(-7.23058021209953,-0.0463557239866595,
24.7359086994214));
#23621=CARTESIAN_POINT('Ctrl Pts',(-7.77580308415762,1.04372901584095,24.7836307228763));
#23622=CARTESIAN_POINT('Ctrl Pts',(-8.78282117356678,1.1503660334596,24.8233990757553));
#23623=CARTESIAN_POINT('Ctrl Pts',(-9.36868552067456,0.700936218802155,
24.8552137580586));
#23624=CARTESIAN_POINT('Ctrl Pts',(-9.68415338762423,0.0333253917200288,
24.8870284403618));
#23625=CARTESIAN_POINT('Ctrl Pts',(-9.36711056521203,-0.92841300029759,
24.9267967932409));
#23626=CARTESIAN_POINT('Ctrl Pts',(-8.18642334722071,-1.23095293731781,
24.9745188166957));
#23627=CARTESIAN_POINT('Ctrl Pts',(-7.29601045824367,-0.402085721548624,
25.0222408401506));
#23628=CARTESIAN_POINT('Ctrl Pts',(-7.50966749686034,0.795497947379344,
25.0699628636054));
#23629=CARTESIAN_POINT('Ctrl Pts',(-8.63521357891507,1.26315031548144,25.1176848870603));
#23630=CARTESIAN_POINT('Ctrl Pts',(-9.46654470641044,0.684924198481284,
25.1574532399394));
#23631=CARTESIAN_POINT('Ctrl Pts',(-9.61555410710697,-0.0382772879795426,
25.1892679222426));
#23632=CARTESIAN_POINT('Ctrl Pts',(-9.41732403297787,-0.749564170486076,
25.2210826045458));
#23633=CARTESIAN_POINT('Ctrl Pts',(-8.54831418196222,-1.26944758507203,
25.2608509574249));
#23634=CARTESIAN_POINT('Ctrl Pts',(-7.45747004727097,-0.725745650157399,
25.3085729808797));
#23635=CARTESIAN_POINT('Ctrl Pts',(-7.3264026964314,0.483666324224087,25.3562950043346));
#23636=CARTESIAN_POINT('Ctrl Pts',(-8.2715353000242,1.24955165236358,25.4040170277895));
#23637=CARTESIAN_POINT('Ctrl Pts',(-9.42870835191566,0.86679422500728,25.4517390512443));
#23638=CARTESIAN_POINT('Ctrl Pts',(-9.67908411377995,-0.114413634620136,
25.4915074041234));
#23639=CARTESIAN_POINT('Ctrl Pts',(-9.31859747480905,-0.758830871073753,
25.5233220864267));
#23640=CARTESIAN_POINT('Ctrl Pts',(-8.70330530427728,-1.16704617749599,
25.5551367687298));
#23641=CARTESIAN_POINT('Ctrl Pts',(-7.70596495586421,-0.991634902627059,
25.5949051216089));
#23642=CARTESIAN_POINT('Ctrl Pts',(-7.2367431757516,0.133257821719693,25.6426271450638));
#23643=CARTESIAN_POINT('Ctrl Pts',(-7.92891582615506,1.13363424900439,25.6903491685186));
#23644=CARTESIAN_POINT('Ctrl Pts',(-9.14477812717384,1.09445722519328,25.7380711919735));
#23645=CARTESIAN_POINT('Ctrl Pts',(-9.76946397098398,0.0478817062920451,
25.7857932154284));
#23646=CARTESIAN_POINT('Ctrl Pts',(-9.31682784607392,-0.857975580674369,
25.8255615683074));
#23647=CARTESIAN_POINT('Ctrl Pts',(-8.62258000991318,-1.1094594439762,25.8573762506107));
#23648=CARTESIAN_POINT('Ctrl Pts',(-7.89017658990837,-1.01560092342389,
25.8891909329139));
#23649=CARTESIAN_POINT('Ctrl Pts',(-7.25070254053196,-0.23040679067833,
25.928959285793));
#23650=CARTESIAN_POINT('Ctrl Pts',(-7.63184561666349,0.927298990484284,
25.9766813092478));
#23651=CARTESIAN_POINT('Ctrl Pts',(-8.80982869801229,1.230963005951,26.0244033327027));
#23652=CARTESIAN_POINT('Ctrl Pts',(-9.7036958993495,0.405822169119469,26.0721253561575));
#23653=CARTESIAN_POINT('Ctrl Pts',(-9.49136433480964,-0.794372826254335,
26.1198473796125));
#23654=CARTESIAN_POINT('Ctrl Pts',(-8.55637342802605,-1.18328012903448,
26.1596157324914));
#23655=CARTESIAN_POINT('Ctrl Pts',(-7.86680560424831,-0.919233905949376,
26.1914304147947));
#23656=CARTESIAN_POINT('Ctrl Pts',(-7.3743327380729,-0.369056963869812,
26.2232450970979));
#23657=CARTESIAN_POINT('Ctrl Pts',(-7.40446434000579,0.643143101576107,
26.263013449977));
#23658=CARTESIAN_POINT('Ctrl Pts',(-8.45016755396898,1.26928805965477,26.3107354734318));
#23659=CARTESIAN_POINT('Ctrl Pts',(-9.53970213718575,0.728205472420586,
26.3584574968867));
#23660=CARTESIAN_POINT('Ctrl Pts',(-9.67581991443327,-0.48064849930249,
26.4061795203416));
#23661=CARTESIAN_POINT('Ctrl Pts',(-8.72998116914571,-1.24937588149534,
26.4539015437965));
#23662=CARTESIAN_POINT('Ctrl Pts',(-7.76843733819602,-0.931743472748531,
26.4936698966755));
#23663=CARTESIAN_POINT('Ctrl Pts',(-7.41970926141765,-0.280887943478391,
26.5254845789787));
#23664=CARTESIAN_POINT('Ctrl Pts',(-7.40724420078035,0.457399814633881,
26.557299261282));
#23665=CARTESIAN_POINT('Ctrl Pts',(-8.09229249818659,1.20316500297713,26.597067614161));
#23666=CARTESIAN_POINT('Ctrl Pts',(-9.29278247777338,0.992507629187354,
26.6447896376159));
#23667=CARTESIAN_POINT('Ctrl Pts',(-9.76272768922647,-0.129547392843957,
26.6925116610708));
#23668=CARTESIAN_POINT('Ctrl Pts',(-9.07473952994518,-1.13280621633976,
26.7402336845256));
#23669=CARTESIAN_POINT('Ctrl Pts',(-7.85648371084657,-1.09531649171282,
26.7879557079805));
#23670=CARTESIAN_POINT('Ctrl Pts',(-7.33713318762905,-0.225988061280798,
26.8277240608595));
#23671=CARTESIAN_POINT('Ctrl Pts',(-7.49924747934842,0.494389026039019,
26.8595387431628));
#23672=CARTESIAN_POINT('Ctrl Pts',(-7.97286685852847,1.06087722113241,26.8913534254661));
#23673=CARTESIAN_POINT('Ctrl Pts',(-8.97887535588318,1.17665195574207,26.931121778345));
#23674=CARTESIAN_POINT('Ctrl Pts',(-9.74892120859526,0.231886320813893,
26.9788438018));
#23675=CARTESIAN_POINT('Ctrl Pts',(-9.37018187864511,-0.924146764431696,
27.0265658252548));
#23676=CARTESIAN_POINT('Ctrl Pts',(-8.19347744150011,-1.23272842596829,
27.0742878487097));
#23677=CARTESIAN_POINT('Ctrl Pts',(-7.29669616986645,-0.407297586304945,
27.1220098721645));
#23678=CARTESIAN_POINT('Ctrl Pts',(-7.47271888540121,0.589935029256493,
27.1617782250436));
#23679=CARTESIAN_POINT('Ctrl Pts',(-8.06664590501909,1.02865462863956,27.1935929073468));
#23680=CARTESIAN_POINT('Ctrl Pts',(-8.79546342201053,1.14718402769961,27.2254075896501));
#23681=CARTESIAN_POINT('Ctrl Pts',(-9.63200965783638,0.576528894322741,
27.265175942529));
#23682=CARTESIAN_POINT('Ctrl Pts',(-9.59621914441288,-0.64177802898069,
27.312897965984));
#23683=CARTESIAN_POINT('Ctrl Pts',(-8.55342818117192,-1.26823072569173,
27.3606199894388));
#23684=CARTESIAN_POINT('Ctrl Pts',(-7.46164306468287,-0.731703714585647,
27.4083420128937));
#23685=CARTESIAN_POINT('Ctrl Pts',(-7.32351125483922,0.479276187530674,
27.4560640363485));
#23686=CARTESIAN_POINT('Ctrl Pts',(-8.10909730428403,1.11826871083707,27.4958323892276));
#23687=CARTESIAN_POINT('Ctrl Pts',(-8.84530157405367,1.06145793115618,27.5276470715308));
#23688=CARTESIAN_POINT('Ctrl Pts',(-9.47402352945873,0.674246239304349,
27.5594617538341));
#23689=CARTESIAN_POINT('Ctrl Pts',(-9.73329676936124,-0.304648174304312,
27.5992301067131));
#23690=CARTESIAN_POINT('Ctrl Pts',(-8.90911752740845,-1.20257985174657,
27.646952130168));
#23691=CARTESIAN_POINT('Ctrl Pts',(-7.71062860019822,-0.994060630599014,
27.6946741536228));
#23692=CARTESIAN_POINT('Ctrl Pts',(-7.23600079802103,0.126021698354508,
27.7423961770777));
#23693=CARTESIAN_POINT('Ctrl Pts',(-7.92385678992181,1.13220600285667,27.7901182005326));
#23694=CARTESIAN_POINT('Ctrl Pts',(-8.93603819131223,1.10145382239673,27.8298865534116));
#23695=CARTESIAN_POINT('Ctrl Pts',(-9.45562501891254,0.57680754146138,27.8617012357149));
#23696=CARTESIAN_POINT('Ctrl Pts',(-9.67775363486414,-0.127382113028449,
27.8935159180181));
#23697=CARTESIAN_POINT('Ctrl Pts',(-9.23335989624522,-1.03731128115096,
27.9332842708971));
#23698=CARTESIAN_POINT('Ctrl Pts',(-8.02257383277471,-1.17713198321521,
27.9810062943521));
#23699=CARTESIAN_POINT('Ctrl Pts',(-7.25264233434914,-0.235292579725615,
28.0287283178069));
#23700=CARTESIAN_POINT('Ctrl Pts',(-7.62654974800387,0.922312370266984,
28.0764503412618));
#23701=CARTESIAN_POINT('Ctrl Pts',(-8.80506831370423,1.23319291086091,28.1241723647166));
#23702=CARTESIAN_POINT('Ctrl Pts',(-9.55041335584025,0.547687510381144,
28.1639407175957));
#23703=CARTESIAN_POINT('Ctrl Pts',(-9.60008761343399,-0.189032694070671,
28.1957553998989));
#23704=CARTESIAN_POINT('Ctrl Pts',(-9.30733666482934,-0.866912531214819,
28.2275700822022));
#23705=CARTESIAN_POINT('Ctrl Pts',(-8.37591494401209,-1.26429202730366,
28.2673384350812));
#23706=CARTESIAN_POINT('Ctrl Pts',(-7.36877222403689,-0.577840090294717,
28.3150604585361));
#23707=CARTESIAN_POINT('Ctrl Pts',(-7.40273464670435,0.638179041167884,
28.3627824819909));
#23708=CARTESIAN_POINT('Ctrl Pts',(-8.44289989517833,1.26898188682333,28.4105045054458));
#23709=CARTESIAN_POINT('Ctrl Pts',(-9.53756106054564,0.73300646455629,28.4582265289006));
#23710=CARTESIAN_POINT('Ctrl Pts',(-9.65271898526393,-0.273072825713538,
28.4979948817797));
#23711=CARTESIAN_POINT('Ctrl Pts',(-9.20826480219185,-0.862720746617945,
28.5298095640829));
#23712=CARTESIAN_POINT('Ctrl Pts',(-8.54334843224031,-1.18382884768557,
28.5616242463862));
#23713=CARTESIAN_POINT('Ctrl Pts',(-7.57896063259388,-0.874938806376633,
28.6013925992652));
#23714=CARTESIAN_POINT('Ctrl Pts',(-7.26643664337314,0.303145009105122,
28.6491146227201));
#23715=CARTESIAN_POINT('Ctrl Pts',(-8.08773653200828,1.20054261779437,28.696836646175));
#23716=CARTESIAN_POINT('Ctrl Pts',(-9.28708596378458,0.997031160766581,
28.7445586696298));
#23717=CARTESIAN_POINT('Ctrl Pts',(-9.76424968181474,-0.124515764873607,
28.7922806930847));
#23718=CARTESIAN_POINT('Ctrl Pts',(-9.19308176306757,-0.960711973454944,
28.8320490459637));
#23719=CARTESIAN_POINT('Ctrl Pts',(-8.47116760566466,-1.11583816367412,
28.863863728267));
#23720=CARTESIAN_POINT('Ctrl Pts',(-7.758228121604,-0.923636465033635,28.8956784105702));
#23721=CARTESIAN_POINT('Ctrl Pts',(-7.23100690715492,-0.0590587231617129,
28.9354467634493));
#23722=CARTESIAN_POINT('Ctrl Pts',(-7.76545498830421,1.03634892185952,28.9831687869041));
#23723=CARTESIAN_POINT('Ctrl Pts',(-8.97371415403392,1.17764965562194,29.030890810359));
#23724=CARTESIAN_POINT('Ctrl Pts',(-9.74757278787959,0.239034337797246,
29.0786128338138));
#23725=CARTESIAN_POINT('Ctrl Pts',(-9.37462510670265,-0.921337331473851,
29.1263348572688));
#23726=CARTESIAN_POINT('Ctrl Pts',(-8.39557156138249,-1.18001050930352,
29.1661032101478));
#23727=CARTESIAN_POINT('Ctrl Pts',(-7.74812630734483,-0.824991759482091,
29.197917892451));
#23728=CARTESIAN_POINT('Ctrl Pts',(-7.33471595134323,-0.213177748401308,
29.2297325747542));
#23729=CARTESIAN_POINT('Ctrl Pts',(-7.50168042485667,0.785612751106832,
29.2695009276334));
#23730=CARTESIAN_POINT('Ctrl Pts',(-8.62255656767401,1.2643385173517,29.3172229510881));
#23731=CARTESIAN_POINT('Ctrl Pts',(-9.62876399049447,0.580662319132331,
29.3649449745431));
#23732=CARTESIAN_POINT('Ctrl Pts',(-9.59986723103598,-0.635493945930121,
29.4126669979978));
#23733=CARTESIAN_POINT('Ctrl Pts',(-8.55864432369126,-1.26900551071647,
29.4603890214528));
#23734=CARTESIAN_POINT('Ctrl Pts',(-7.64893856382622,-0.824074962017151,
29.5001573743318));
#23735=CARTESIAN_POINT('Ctrl Pts',(-7.39165978122259,-0.131949724328084,
29.5319720566351));
#23736=CARTESIAN_POINT('Ctrl Pts',(-7.47917136641087,0.601160787975001,
29.5637867389383));
#23737=CARTESIAN_POINT('Ctrl Pts',(-8.25924185780237,1.24739438139286,29.6035550918174));
#23738=CARTESIAN_POINT('Ctrl Pts',(-9.41955388337242,0.875818431378234,
29.6512771152722));
#23739=CARTESIAN_POINT('Ctrl Pts',(-9.73420537750695,-0.299113479422314,
29.6989991387271));
#23740=CARTESIAN_POINT('Ctrl Pts',(-8.91473661362289,-1.20075991772479,
29.746721162182));
#23741=CARTESIAN_POINT('Ctrl Pts',(-7.91628087823187,-1.03091022985124,
29.786489515061));
#23742=CARTESIAN_POINT('Ctrl Pts',(-7.47389388983263,-0.439466000029977,
29.8183041973642));
#23743=CARTESIAN_POINT('Ctrl Pts',(-7.35134599695441,0.288282690195251,
29.8501188796675));
#23744=CARTESIAN_POINT('Ctrl Pts',(-7.91595128905028,1.12901342715968,29.8898872325466));
#23745=CARTESIAN_POINT('Ctrl Pts',(-9.13634494738218,1.09918250918627,29.9376092560014));
#23746=CARTESIAN_POINT('Ctrl Pts',(-9.66055134658927,0.235760887270644,
29.9773776088804));
#23747=CARTESIAN_POINT('Ctrl Pts',(-9.50494573724989,-0.488941412697737,
30.0091922911837));
#23748=CARTESIAN_POINT('Ctrl Pts',(-9.26902730932514,-0.770372743754008,
30.0250996323353));
#23749=CARTESIAN_POINT('Ctrl Pts',(-9.12339873206855,-0.874219306856311,
30.0330533029111));
#23750=CARTESIAN_POINT('Ctrl Pts',(-8.98717784885836,1.02066752383268,1.76694669708888));
#23751=CARTESIAN_POINT('Ctrl Pts',(-9.15720195857778,0.939512810771836,
1.77490036766469));
#23752=CARTESIAN_POINT('Ctrl Pts',(-9.45329826783746,0.690609604732661,
1.79080770881631));
#23753=CARTESIAN_POINT('Ctrl Pts',(-9.7469683923631,-0.032794831450878,
1.82262239111956));
#23754=CARTESIAN_POINT('Ctrl Pts',(-9.3607214115926,-1.02415996628745,1.86239074399861));
#23755=CARTESIAN_POINT('Ctrl Pts',(-8.10013924535698,-1.2778080089645,1.91011276745347));
#23756=CARTESIAN_POINT('Ctrl Pts',(-7.36100311520275,-0.508672370427067,
1.94988112033252));
#23757=CARTESIAN_POINT('Ctrl Pts',(-7.35533111002763,0.268650789363701,
1.98169580263576));
#23758=CARTESIAN_POINT('Ctrl Pts',(-7.7063307288449,0.962938239586403,2.013510484939));
#23759=CARTESIAN_POINT('Ctrl Pts',(-8.71112529982286,1.32134053301244,2.05327883781806));
#23760=CARTESIAN_POINT('Ctrl Pts',(-9.72577069974048,0.535519851686026,
2.10100086127292));
#23761=CARTESIAN_POINT('Ctrl Pts',(-9.61375965135636,-0.740763047588873,
2.14872288472778));
#23762=CARTESIAN_POINT('Ctrl Pts',(-8.47786848052187,-1.33797052146523,
2.19644490818264));
#23763=CARTESIAN_POINT('Ctrl Pts',(-7.55070313740433,-0.809923379715486,
2.2362132610617));
#23764=CARTESIAN_POINT('Ctrl Pts',(-7.32613880404449,-0.065370300961561,
2.26802794336494));
#23765=CARTESIAN_POINT('Ctrl Pts',(-7.46673614985931,0.699583561915718,
2.29984262566818));
#23766=CARTESIAN_POINT('Ctrl Pts',(-8.32926454613903,1.32715695287655,2.33961097854723));
#23767=CARTESIAN_POINT('Ctrl Pts',(-9.52502558453072,0.859963540493027,
2.38733300200209));
#23768=CARTESIAN_POINT('Ctrl Pts',(-9.77693128489481,-0.396393259162436,
2.43505502545695));
#23769=CARTESIAN_POINT('Ctrl Pts',(-8.85786004067544,-1.28924928143315,
2.48277704891182));
#23770=CARTESIAN_POINT('Ctrl Pts',(-7.60771327966523,-0.997164717747076,
2.53049907236667));
#23771=CARTESIAN_POINT('Ctrl Pts',(-7.25224299371205,0.00850363864383403,
2.57026742524573));
#23772=CARTESIAN_POINT('Ctrl Pts',(-7.56946535593601,0.718634766301041,
2.60208210754897));
#23773=CARTESIAN_POINT('Ctrl Pts',(-8.17633439356632,1.20507622033207,2.63389678985222));
#23774=CARTESIAN_POINT('Ctrl Pts',(-9.2391996530484,1.11539202291409,2.67366514273126));
#23775=CARTESIAN_POINT('Ctrl Pts',(-9.83784103294923,-0.0203107034754631,
2.72138716618613));
#23776=CARTESIAN_POINT('Ctrl Pts',(-9.2063285939658,-1.13523854117206,2.76910918964099));
#23777=CARTESIAN_POINT('Ctrl Pts',(-7.92710594247716,-1.20914174508905,
2.81683121309585));
#23778=CARTESIAN_POINT('Ctrl Pts',(-7.17278030824983,-0.170303293381034,
2.86455323655072));
#23779=CARTESIAN_POINT('Ctrl Pts',(-7.56194385943746,0.822811344328335,
2.90432158942976));
#23780=CARTESIAN_POINT('Ctrl Pts',(-8.26646746974983,1.15229941527231,2.93613627173301));
#23781=CARTESIAN_POINT('Ctrl Pts',(-9.04368293743357,1.1231102708342,2.96795095403625));
#23782=CARTESIAN_POINT('Ctrl Pts',(-9.78879960305325,0.359876283870339,
3.0077193069153));
#23783=CARTESIAN_POINT('Ctrl Pts',(-9.49845790146036,-0.890681293407522,
3.05544133037016));
#23784=CARTESIAN_POINT('Ctrl Pts',(-8.29140066639367,-1.32066379967401,
3.10316335382503));
#23785=CARTESIAN_POINT('Ctrl Pts',(-7.27563101481108,-0.539584967461653,
3.15088537727989));
#23786=CARTESIAN_POINT('Ctrl Pts',(-7.38485983741583,0.73957945590063,3.19860740073475));
#23787=CARTESIAN_POINT('Ctrl Pts',(-8.32894005637996,1.2360041721841,3.23837575361381));
#23788=CARTESIAN_POINT('Ctrl Pts',(-9.07731547286537,1.0242256745203,3.27019043591704));
#23789=CARTESIAN_POINT('Ctrl Pts',(-9.64598941147203,0.493635580865258,
3.30200511822029));
#23790=CARTESIAN_POINT('Ctrl Pts',(-9.7101184478014,-0.571076786728671,
3.34177347109933));
#23791=CARTESIAN_POINT('Ctrl Pts',(-8.67233310217777,-1.32685065118963,
3.3894954945542));
#23792=CARTESIAN_POINT('Ctrl Pts',(-7.47816356649126,-0.862274235291014,
3.43721751800906));
#23793=CARTESIAN_POINT('Ctrl Pts',(-7.22102781558539,0.393015903201006,
3.48493954146392));
#23794=CARTESIAN_POINT('Ctrl Pts',(-8.14056280244616,1.28892212916197,3.53266156491878));
#23795=CARTESIAN_POINT('Ctrl Pts',(-9.17932683400365,1.04665317585688,3.57242991779784));
#23796=CARTESIAN_POINT('Ctrl Pts',(-9.60672601934412,0.396848718848358,
3.60424460010108));
#23797=CARTESIAN_POINT('Ctrl Pts',(-9.68963365623764,-0.376483176085459,
3.63605928240432));
#23798=CARTESIAN_POINT('Ctrl Pts',(-9.04151258676327,-1.2236337166026,3.67582763528338));
#23799=CARTESIAN_POINT('Ctrl Pts',(-7.76219705954577,-1.11618912811821,
3.72354965873823));
#23800=CARTESIAN_POINT('Ctrl Pts',(-7.1630649420991,0.0164682923005445,
3.7712716821931));
#23801=CARTESIAN_POINT('Ctrl Pts',(-7.78991506235602,1.13402413113802,3.81899370564796));
#23802=CARTESIAN_POINT('Ctrl Pts',(-9.07148901432152,1.20992382427138,3.86671572910283));
#23803=CARTESIAN_POINT('Ctrl Pts',(-9.69854629147273,0.347065707216833,
3.90648408198187));
#23804=CARTESIAN_POINT('Ctrl Pts',(-9.596614981266,-0.423989351762,3.93829876428512));
#23805=CARTESIAN_POINT('Ctrl Pts',(-9.15333939402706,-1.06306888494648,
3.97011344658835));
#23806=CARTESIAN_POINT('Ctrl Pts',(-8.1089229359139,-1.27967733588411,4.00988179946741));
#23807=CARTESIAN_POINT('Ctrl Pts',(-7.211735050573,-0.361392817789792,4.05760382292227));
#23808=CARTESIAN_POINT('Ctrl Pts',(-7.49971327974267,0.88718263676238,4.10532584637714));
#23809=CARTESIAN_POINT('Ctrl Pts',(-8.70496400049602,1.32220312629068,4.15304786983199));
#23810=CARTESIAN_POINT('Ctrl Pts',(-9.72381812702013,0.541095690249467,
4.20076989328686));
#23811=CARTESIAN_POINT('Ctrl Pts',(-9.63348239149061,-0.521713988800163,
4.24053824616591));
#23812=CARTESIAN_POINT('Ctrl Pts',(-9.05191142252884,-1.03813542913569,
4.27235292846915));
#23813=CARTESIAN_POINT('Ctrl Pts',(-8.2985465161075,-1.23141557232177,4.30416761077239));
#23814=CARTESIAN_POINT('Ctrl Pts',(-7.36698075663241,-0.711886752361923,
4.34393596365145));
#23815=CARTESIAN_POINT('Ctrl Pts',(-7.28929364897506,0.569580091172468,
4.39165798710631));
#23816=CARTESIAN_POINT('Ctrl Pts',(-8.32399475052738,1.32540133765357,4.43938001056117));
#23817=CARTESIAN_POINT('Ctrl Pts',(-9.52009434957654,0.865816878233629,
4.48710203401603));
#23818=CARTESIAN_POINT('Ctrl Pts',(-9.77954403027077,-0.391512999309189,
4.5348240574709));
#23819=CARTESIAN_POINT('Ctrl Pts',(-9.01585335320423,-1.1361615800215,4.57459241034995));
#23820=CARTESIAN_POINT('Ctrl Pts',(-8.2381547105969,-1.14619737914636,4.60640709265319));
#23821=CARTESIAN_POINT('Ctrl Pts',(-7.54196087371678,-0.799455346119763,
4.63822177495643));
#23822=CARTESIAN_POINT('Ctrl Pts',(-7.17737793402098,0.202943895239693,
4.67799012783549));
#23823=CARTESIAN_POINT('Ctrl Pts',(-7.95706355310381,1.22288648831522,4.72571215129034));
#23824=CARTESIAN_POINT('Ctrl Pts',(-9.23407761156503,1.11749568853522,4.77343417474522));
#23825=CARTESIAN_POINT('Ctrl Pts',(-9.83793547776687,-0.0126493480030172,
4.82115619820006));
#23826=CARTESIAN_POINT('Ctrl Pts',(-9.21150071631891,-1.13326170177383,
4.86887822165494));
#23827=CARTESIAN_POINT('Ctrl Pts',(-8.14674923105428,-1.19673794632252,
4.90864657453397));
#23828=CARTESIAN_POINT('Ctrl Pts',(-7.55204583831342,-0.695495718811888,
4.94046125683723));
#23829=CARTESIAN_POINT('Ctrl Pts',(-7.25241294297447,0.0222340520685815,
4.97227593914046));
#23830=CARTESIAN_POINT('Ctrl Pts',(-7.63254458493515,1.01884074167864,5.01204429201953));
#23831=CARTESIAN_POINT('Ctrl Pts',(-8.88951136940995,1.28004384369151,5.05976631547437));
#23832=CARTESIAN_POINT('Ctrl Pts',(-9.78630251203301,0.364818312634419,
5.10748833892925));
#23833=CARTESIAN_POINT('Ctrl Pts',(-9.50354194588265,-0.884949101093522,
5.15521036238411));
#23834=CARTESIAN_POINT('Ctrl Pts',(-8.29660552829489,-1.32255285070557,
5.20293238583896));
#23835=CARTESIAN_POINT('Ctrl Pts',(-7.44985251279868,-0.673912511423973,
5.24270073871802));
#23836=CARTESIAN_POINT('Ctrl Pts',(-7.32805832441254,0.0942554856005425,
5.27451542102126));
#23837=CARTESIAN_POINT('Ctrl Pts',(-7.57105541720643,0.833084497531607,
5.3063301033245));
#23838=CARTESIAN_POINT('Ctrl Pts',(-8.51058998985244,1.33805949275232,5.34609845620355));
#23839=CARTESIAN_POINT('Ctrl Pts',(-9.632074979905,0.713188326142003,5.39382047965842));
#23840=CARTESIAN_POINT('Ctrl Pts',(-9.711463480323,-0.565705567887997,5.44154250311327));
#23841=CARTESIAN_POINT('Ctrl Pts',(-8.67992837998318,-1.32584204441887,
5.48926452656815));
#23842=CARTESIAN_POINT('Ctrl Pts',(-7.4808637944681,-0.867108268097873,
5.53698655002299));
#23843=CARTESIAN_POINT('Ctrl Pts',(-7.26489572044008,0.177440797286747,
5.57675490290206));
#23844=CARTESIAN_POINT('Ctrl Pts',(-7.67538459440189,0.838057766740956,
5.60856958520529));
#23845=CARTESIAN_POINT('Ctrl Pts',(-8.3425522063548,1.23781178302893,5.64038426750854));
#23846=CARTESIAN_POINT('Ctrl Pts',(-9.38347284504564,1.00498312726961,5.6801526203876));
#23847=CARTESIAN_POINT('Ctrl Pts',(-9.82275955589709,-0.201341764060873,
5.72787464384245));
#23848=CARTESIAN_POINT('Ctrl Pts',(-9.04604404738165,-1.22045174096105,
5.77559666729732));
#23849=CARTESIAN_POINT('Ctrl Pts',(-7.76860092376069,-1.12039579611335,
5.82331869075218));
#23850=CARTESIAN_POINT('Ctrl Pts',(-7.16194419267288,0.0110458366719952,
5.87104071420704));
#23851=CARTESIAN_POINT('Ctrl Pts',(-7.68204406194035,0.94229289571872,5.9108090670861));
#23852=CARTESIAN_POINT('Ctrl Pts',(-8.42470539828331,1.17331245220397,5.94262374938933));
#23853=CARTESIAN_POINT('Ctrl Pts',(-9.19080374928177,1.03911404470695,5.97443843169258));
#23854=CARTESIAN_POINT('Ctrl Pts',(-9.82566855549311,0.181984161416506,
6.01420678457162));
#23855=CARTESIAN_POINT('Ctrl Pts',(-9.36860763294159,-1.01771908141086,
6.06192880802649));
#23856=CARTESIAN_POINT('Ctrl Pts',(-8.11443176766407,-1.28023579543347,
6.10965083148135));
#23857=CARTESIAN_POINT('Ctrl Pts',(-7.21382565992496,-0.368764037840895,
6.15737285493622));
#23858=CARTESIAN_POINT('Ctrl Pts',(-7.4953179108137,0.883815169420571,6.20509487839108));
#23859=CARTESIAN_POINT('Ctrl Pts',(-8.49794049113376,1.24778346533051,6.24486323127012));
#23860=CARTESIAN_POINT('Ctrl Pts',(-9.2107318204641,0.936585109279635,6.27667791357337));
#23861=CARTESIAN_POINT('Ctrl Pts',(-9.70229305211699,0.33385511043003,6.30849259587662));
#23862=CARTESIAN_POINT('Ctrl Pts',(-9.62160964900884,-0.729730874555741,
6.34826094875566));
#23863=CARTESIAN_POINT('Ctrl Pts',(-8.49101525742003,-1.33796510532709,
6.39598297221054));
#23864=CARTESIAN_POINT('Ctrl Pts',(-7.37078144062068,-0.715913401780636,
6.44370499566537));
#23865=CARTESIAN_POINT('Ctrl Pts',(-7.2860518452889,0.562637739887455,6.49142701912026));
#23866=CARTESIAN_POINT('Ctrl Pts',(-8.31846747525854,1.32573047656402,6.5391490425751));
#23867=CARTESIAN_POINT('Ctrl Pts',(-9.31484091722209,0.944987882223714,
6.57891739545418));
#23868=CARTESIAN_POINT('Ctrl Pts',(-9.65028120019568,0.243278745518274,
6.6107320777574));
#23869=CARTESIAN_POINT('Ctrl Pts',(-9.62767247656973,-0.534155973022973,
6.64254676006066));
#23870=CARTESIAN_POINT('Ctrl Pts',(-8.87077348733239,-1.28570695538331,
6.68231511293969));
#23871=CARTESIAN_POINT('Ctrl Pts',(-7.6178028842378,-1.00596202592991,6.73003713639457));
#23872=CARTESIAN_POINT('Ctrl Pts',(-7.17761766204372,0.197412020801958,
6.77775915984942));
#23873=CARTESIAN_POINT('Ctrl Pts',(-7.95006969414746,1.21975735594301,6.82548118330428));
#23874=CARTESIAN_POINT('Ctrl Pts',(-9.23011293994277,1.1213609806649,6.87320320675915));
#23875=CARTESIAN_POINT('Ctrl Pts',(-9.73451180758851,0.181516982273174,
6.9129715596382));
#23876=CARTESIAN_POINT('Ctrl Pts',(-9.52907613394154,-0.568624391049578,
6.94478624194144));
#23877=CARTESIAN_POINT('Ctrl Pts',(-9.00331905765805,-1.14176956699993,
6.97660092424469));
#23878=CARTESIAN_POINT('Ctrl Pts',(-7.93918771291786,-1.2149094339445,7.01636927712373));
#23879=CARTESIAN_POINT('Ctrl Pts',(-7.17465574624786,-0.183559139566383,
7.0640913005786));
#23880=CARTESIAN_POINT('Ctrl Pts',(-7.6291064911733,1.01450039427264,7.11181332403346));
#23881=CARTESIAN_POINT('Ctrl Pts',(-8.88217491497787,1.28225336148277,7.15953534748833));
#23882=CARTESIAN_POINT('Ctrl Pts',(-9.7858331951435,0.37033545373983,7.20725737094318));
#23883=CARTESIAN_POINT('Ctrl Pts',(-9.55236639024744,-0.670442241066719,
7.24702572382224));
#23884=CARTESIAN_POINT('Ctrl Pts',(-8.90620328656803,-1.10332691326094,
7.27884040612548));
#23885=CARTESIAN_POINT('Ctrl Pts',(-8.13360094072032,-1.19277807964766,
7.31065508842873));
#23886=CARTESIAN_POINT('Ctrl Pts',(-7.2809942040565,-0.551851631768721,
7.35042344130776));
#23887=CARTESIAN_POINT('Ctrl Pts',(-7.37760513024462,0.72832760830481,7.39814546476264));
#23888=CARTESIAN_POINT('Ctrl Pts',(-8.50515012218228,1.33702656291388,7.44586748821749));
#23889=CARTESIAN_POINT('Ctrl Pts',(-9.62797240281083,0.719659368847056,
7.49358951167236));
#23890=CARTESIAN_POINT('Ctrl Pts',(-9.71471830703312,-0.56122614745596,
7.54131153512722));
#23891=CARTESIAN_POINT('Ctrl Pts',(-8.85719934651032,-1.19556532434727,
7.58107988800627));
#23892=CARTESIAN_POINT('Ctrl Pts',(-8.08530903462118,-1.10016489254009,
7.61289457030952));
#23893=CARTESIAN_POINT('Ctrl Pts',(-7.4424999318959,-0.662315199802028,
7.64470925261275));
#23894=CARTESIAN_POINT('Ctrl Pts',(-7.21705792520234,0.380230176003379,
7.68447760549182));
#23895=CARTESIAN_POINT('Ctrl Pts',(-8.12771455933282,1.28515948400945,7.73219962894666));
#23896=CARTESIAN_POINT('Ctrl Pts',(-9.37868310282978,1.00776116143522,7.77992165240154));
#23897=CARTESIAN_POINT('Ctrl Pts',(-9.82389083522868,-0.193763786786019,
7.82764367585639));
#23898=CARTESIAN_POINT('Ctrl Pts',(-9.05143631128576,-1.21919372891482,
7.87536569931126));
#23899=CARTESIAN_POINT('Ctrl Pts',(-7.98789999353893,-1.1378582518537,7.91513405219031));
#23900=CARTESIAN_POINT('Ctrl Pts',(-7.46657387430056,-0.560679792989207,
7.94694873449354));
#23901=CARTESIAN_POINT('Ctrl Pts',(-7.26692318332948,0.191021941458752,
7.97876341679679));
#23902=CARTESIAN_POINT('Ctrl Pts',(-7.77854738769087,1.12695229811292,8.01853176967584));
#23903=CARTESIAN_POINT('Ctrl Pts',(-9.0593106683688,1.21548464610666,8.06625379313071));
#23904=CARTESIAN_POINT('Ctrl Pts',(-9.82386390625267,0.187218886379563,
8.11397581658557));
#23905=CARTESIAN_POINT('Ctrl Pts',(-9.37442127753776,-1.01272838316176,
8.16169784004043));
#23906=CARTESIAN_POINT('Ctrl Pts',(-8.11933277591933,-1.28281246429101,
8.20941986349528));
#23907=CARTESIAN_POINT('Ctrl Pts',(-7.36824599282011,-0.525452838189341,
8.24918821637434));
#23908=CARTESIAN_POINT('Ctrl Pts',(-7.35162708719266,0.252132982124451,
8.28100289867758));
#23909=CARTESIAN_POINT('Ctrl Pts',(-7.69246319392794,0.951237154850419,
8.31281758098083));
#23910=CARTESIAN_POINT('Ctrl Pts',(-8.69174020745547,1.32429265907298,8.35258593385989));
#23911=CARTESIAN_POINT('Ctrl Pts',(-9.71824654100196,0.553269115357872,
8.40030795731473));
#23912=CARTESIAN_POINT('Ctrl Pts',(-9.62366984726379,-0.724591352450493,
8.44802998076961));
#23913=CARTESIAN_POINT('Ctrl Pts',(-8.49867715414896,-1.33799461835653,
8.49575200422446));
#23914=CARTESIAN_POINT('Ctrl Pts',(-7.3728019842507,-0.721068642585769,
8.54347402767932));
#23915=CARTESIAN_POINT('Ctrl Pts',(-7.30031455453236,0.343107344517893,
8.58324238055838));
#23916=CARTESIAN_POINT('Ctrl Pts',(-7.79650446864174,0.942032602887781,
8.61505706286162));
#23917=CARTESIAN_POINT('Ctrl Pts',(-8.51167203456982,1.24773057249472,8.64687174516487));
#23918=CARTESIAN_POINT('Ctrl Pts',(-9.5114609494476,0.8760491434687,8.6866400980439));
#23919=CARTESIAN_POINT('Ctrl Pts',(-9.78329531536966,-0.378661434823328,
8.73436212149879));
#23920=CARTESIAN_POINT('Ctrl Pts',(-8.87569420011532,-1.2831681190302,8.78208414495363));
#23921=CARTESIAN_POINT('Ctrl Pts',(-7.62357790932744,-1.01099736283204,
8.82980616840852));
#23922=CARTESIAN_POINT('Ctrl Pts',(-7.17577273944743,0.192191353705361,
8.87752819186336));
#23923=CARTESIAN_POINT('Ctrl Pts',(-7.81722180370288,1.04440497537604,8.91729654474242));
#23924=CARTESIAN_POINT('Ctrl Pts',(-8.58433124965774,1.17269758585738,8.94911122704566));
#23925=CARTESIAN_POINT('Ctrl Pts',(-9.32519083587387,0.935963622326625,
8.9809259093489));
#23926=CARTESIAN_POINT('Ctrl Pts',(-9.83810119577728,0.00073748833604553,
9.02069426222796));
#23927=CARTESIAN_POINT('Ctrl Pts',(-9.22274614596173,-1.12599705024909,
9.06841628568281));
#23928=CARTESIAN_POINT('Ctrl Pts',(-7.94457012542596,-1.21620894920507,
9.11613830913767));
#23929=CARTESIAN_POINT('Ctrl Pts',(-7.17572861331942,-0.191145607041478,
9.16386033259254));
#23930=CARTESIAN_POINT('Ctrl Pts',(-7.62429548986411,1.01175934142331,9.2115823560474));
#23931=CARTESIAN_POINT('Ctrl Pts',(-8.66697888918347,1.23656211671555,9.25135070892645));
#23932=CARTESIAN_POINT('Ctrl Pts',(-9.33104710651617,0.831680283700215,
9.28316539122969));
#23933=CARTESIAN_POINT('Ctrl Pts',(-9.7364345848479,0.167920622083772,9.31498007353294));
#23934=CARTESIAN_POINT('Ctrl Pts',(-9.5124259956029,-0.87493368746273,9.35474842641199));
#23935=CARTESIAN_POINT('Ctrl Pts',(-8.30986303021255,-1.32441658151513,
9.40247044986685));
#23936=CARTESIAN_POINT('Ctrl Pts',(-7.28421442593712,-0.556355993583608,
9.45019247332171));
#23937=CARTESIAN_POINT('Ctrl Pts',(-7.37345282372569,0.721888362768501,
9.49791449677658));
#23938=CARTESIAN_POINT('Ctrl Pts',(-8.49971837334819,1.33810136937232,9.54563652023143));
#23939=CARTESIAN_POINT('Ctrl Pts',(-9.43533487510731,0.825903438264406,
9.58540487311049));
#23940=CARTESIAN_POINT('Ctrl Pts',(-9.67263301799846,0.0852243664946371,
9.61721955541373));
#23941=CARTESIAN_POINT('Ctrl Pts',(-9.54492468496979,-0.681982566250605,
9.64903423771696));
#23942=CARTESIAN_POINT('Ctrl Pts',(-8.69319984617433,-1.32408050112819,
9.68880259059603));
#23943=CARTESIAN_POINT('Ctrl Pts',(-7.48967042451988,-0.877191824849249,
9.73652461405088));
#23944=CARTESIAN_POINT('Ctrl Pts',(-7.21654611967445,0.374716814105095,
9.78424663750576));
#23945=CARTESIAN_POINT('Ctrl Pts',(-8.12036130107557,1.28300654984733,9.83196866096061));
#23946=CARTESIAN_POINT('Ctrl Pts',(-9.3752785479547,1.01212786619081,9.87969068441547));
#23947=CARTESIAN_POINT('Ctrl Pts',(-9.74772132105027,0.0126223185503058,
9.91945903729454));
#23948=CARTESIAN_POINT('Ctrl Pts',(-9.44256812075637,-0.702777863395229,
9.95127371959776));
#23949=CARTESIAN_POINT('Ctrl Pts',(-8.84402094059755,-1.19942378263872,
9.98308840190103));
#23950=CARTESIAN_POINT('Ctrl Pts',(-7.77979005479142,-1.12774686381844,
10.02285675478));
#23951=CARTESIAN_POINT('Ctrl Pts',(-7.16200677719407,-0.00234187907062422,
10.0705787782349));
#23952=CARTESIAN_POINT('Ctrl Pts',(-7.77455305655034,1.12311766344198,10.1183008016898));
#23953=CARTESIAN_POINT('Ctrl Pts',(-9.05234112294006,1.21866756442496,10.1660228251446));
#23954=CARTESIAN_POINT('Ctrl Pts',(-9.82414624322832,0.192748749863605,
10.2137448485995));
#23955=CARTESIAN_POINT('Ctrl Pts',(-9.45185190919853,-0.806812097631219,
10.2535132014786));
#23956=CARTESIAN_POINT('Ctrl Pts',(-8.75300752431604,-1.14818055208406,
10.2853278837818));
#23957=CARTESIAN_POINT('Ctrl Pts',(-7.97540927235462,-1.13215387045997,
10.3171425660851));
#23958=CARTESIAN_POINT('Ctrl Pts',(-7.21747782872572,-0.38164411985454,
10.3569109189641));
#23959=CARTESIAN_POINT('Ctrl Pts',(-7.48660594026586,0.873649717202334,
10.4046329424189));
#23960=CARTESIAN_POINT('Ctrl Pts',(-8.68621056060662,1.32400611056535,10.4523549658738));
#23961=CARTESIAN_POINT('Ctrl Pts',(-9.71505831551299,0.560236234614444,
10.5000769893287));
#23962=CARTESIAN_POINT('Ctrl Pts',(-9.62750143868948,-0.720594101962218,
10.5477990127836));
#23963=CARTESIAN_POINT('Ctrl Pts',(-8.6919610129374,-1.23293097432137,10.5875673656626));
#23964=CARTESIAN_POINT('Ctrl Pts',(-7.94010744001488,-1.03385284679102,
10.6193820479658));
#23965=CARTESIAN_POINT('Ctrl Pts',(-7.36253209998977,-0.51296646515663,
10.6511967302691));
#23966=CARTESIAN_POINT('Ctrl Pts',(-7.28038664382364,0.550507598009241,
10.6909650831481));
#23967=CARTESIAN_POINT('Ctrl Pts',(-8.30522797742683,1.32374287831698,10.738687106603));
#23968=CARTESIAN_POINT('Ctrl Pts',(-9.50709165300646,0.879450371618857,
10.7864091300578));
#23969=CARTESIAN_POINT('Ctrl Pts',(-9.78544264857298,-0.371306538996862,
10.8341311535127));
#23970=CARTESIAN_POINT('Ctrl Pts',(-8.88120717061705,-1.28265211460467,
10.8818531769676));
#23971=CARTESIAN_POINT('Ctrl Pts',(-7.83849039769771,-1.05800418902331,
10.9216215298466));
#23972=CARTESIAN_POINT('Ctrl Pts',(-7.4001512604151,-0.415528744587011,
10.9534362121499));
#23973=CARTESIAN_POINT('Ctrl Pts',(-7.30416297486433,0.356288685259149,
10.9852508944531));
#23974=CARTESIAN_POINT('Ctrl Pts',(-7.93784887050746,1.21429051780861,11.0250192473322));
#23975=CARTESIAN_POINT('Ctrl Pts',(-9.21880008209559,1.1285201773347,11.072741270787));
#23976=CARTESIAN_POINT('Ctrl Pts',(-9.83702225274205,0.00616841700861393,
11.1204632942419));
#23977=CARTESIAN_POINT('Ctrl Pts',(-9.22918222718139,-1.1218398407237,11.1681853176968));
#23978=CARTESIAN_POINT('Ctrl Pts',(-7.94907693849614,-1.21942573957288,
11.2159073411516));
#23979=CARTESIAN_POINT('Ctrl Pts',(-7.30750132044213,-0.367307387867063,
11.2556756940307));
#23980=CARTESIAN_POINT('Ctrl Pts',(-7.39636403717926,0.40536286104344,11.2874903763339));
#23981=CARTESIAN_POINT('Ctrl Pts',(-7.82875645784298,1.05185546775282,11.3193050586371));
#23982=CARTESIAN_POINT('Ctrl Pts',(-8.86935603952817,1.28611487437698,11.3590734115162));
#23983=CARTESIAN_POINT('Ctrl Pts',(-9.78196192035174,0.383151384494735,
11.4067954349711));
#23984=CARTESIAN_POINT('Ctrl Pts',(-9.51516338353789,-0.870120599928379,
11.4545174584259));
#23985=CARTESIAN_POINT('Ctrl Pts',(-8.31745031259649,-1.32548367032607,
11.5022394818808));
#23986=CARTESIAN_POINT('Ctrl Pts',(-7.28551804013416,-0.561737414803424,
11.5499615053357));
#23987=CARTESIAN_POINT('Ctrl Pts',(-7.35784742999161,0.502449325556585,
11.5897298582147));
#23988=CARTESIAN_POINT('Ctrl Pts',(-7.93059201648363,1.02864276396249,11.621544540518));
#23989=CARTESIAN_POINT('Ctrl Pts',(-8.68057670984098,1.23464969517349,11.6533592228212));
#23990=CARTESIAN_POINT('Ctrl Pts',(-9.62080459220198,0.730966770878588,
11.6931275757003));
#23991=CARTESIAN_POINT('Ctrl Pts',(-9.7201758360483,-0.549001163747355,
11.7408495991551));
#23992=CARTESIAN_POINT('Ctrl Pts',(-8.69841910664045,-1.32223160294096,
11.78857162261));
#23993=CARTESIAN_POINT('Ctrl Pts',(-7.49471015829369,-0.88296301328782,
11.8362936460648));
#23994=CARTESIAN_POINT('Ctrl Pts',(-7.21401103173468,0.369794169139481,
11.8840156695197));
#23995=CARTESIAN_POINT('Ctrl Pts',(-7.96498533229343,1.12726532957765,11.9237840223988));
#23996=CARTESIAN_POINT('Ctrl Pts',(-8.74240260626814,1.1504661507489,11.955598704702));
#23997=CARTESIAN_POINT('Ctrl Pts',(-9.44436701501593,0.815560395604711,
11.9874133870052));
#23998=CARTESIAN_POINT('Ctrl Pts',(-9.82586834953045,-0.180522779014172,
12.0271817398843));
#23999=CARTESIAN_POINT('Ctrl Pts',(-9.06356213495693,-1.21351929062335,
12.0749037633391));
#24000=CARTESIAN_POINT('Ctrl Pts',(-7.78494683297297,-1.12976348056592,
12.122625786794));
#24001=CARTESIAN_POINT('Ctrl Pts',(-7.16204212561228,-0.0100037510999278,
12.1703478102489));
#24002=CARTESIAN_POINT('Ctrl Pts',(-7.7694151050087,1.12105355145961,12.2180698337037));
#24003=CARTESIAN_POINT('Ctrl Pts',(-8.83293933202686,1.20254697168905,12.2578381865828));
#24004=CARTESIAN_POINT('Ctrl Pts',(-9.43604353531208,0.711444929383173,
12.289652868886));
#24005=CARTESIAN_POINT('Ctrl Pts',(-9.74778467198765,-0.00110918061939206,
12.3214675511893));
#24006=CARTESIAN_POINT('Ctrl Pts',(-9.38458009166091,-1.00400867300379,
12.3612359040683));
#24007=CARTESIAN_POINT('Ctrl Pts',(-8.13221563573533,-1.28645482239937,
12.4089579275232));
#24008=CARTESIAN_POINT('Ctrl Pts',(-7.22005822950576,-0.386543164264866,
12.456679950978));
#24009=CARTESIAN_POINT('Ctrl Pts',(-7.48161967120934,0.86783227331347,12.5044019744329));
#24010=CARTESIAN_POINT('Ctrl Pts',(-8.68097446271812,1.32580677244971,12.5521239978878));
#24011=CARTESIAN_POINT('Ctrl Pts',(-9.53858761847399,0.691594951312903,
12.5918923507668));
#24012=CARTESIAN_POINT('Ctrl Pts',(-9.67336945723156,-0.0744009702940164,
12.62370703307));
#24013=CARTESIAN_POINT('Ctrl Pts',(-9.44291558800347,-0.817238038657684,
12.6555217153733));
#24014=CARTESIAN_POINT('Ctrl Pts',(-8.51206491367397,-1.33804700660616,
12.6952900682523));
#24015=CARTESIAN_POINT('Ctrl Pts',(-7.38016157160731,-0.732252171705333,
12.7430120917072));
#24016=CARTESIAN_POINT('Ctrl Pts',(-7.27913273895857,0.545114377551169,
12.7907341151621));
#24017=CARTESIAN_POINT('Ctrl Pts',(-8.29765086394642,1.32260582783026,12.8384561386169));
#24018=CARTESIAN_POINT('Ctrl Pts',(-9.50430997171838,0.884237996659668,
12.8861781620718));
#24019=CARTESIAN_POINT('Ctrl Pts',(-9.73793133825872,-0.156505014890767,
12.9259465149508));
#24020=CARTESIAN_POINT('Ctrl Pts',(-9.3386855611913,-0.823976891055697,
12.9577611972541));
#24021=CARTESIAN_POINT('Ctrl Pts',(-8.67838141684562,-1.23496878019371,
12.9895758795573));
#24022=CARTESIAN_POINT('Ctrl Pts',(-7.63366817039504,-1.01979631056548,
13.0293442324364));
#24023=CARTESIAN_POINT('Ctrl Pts',(-7.17402130438394,0.178918549749654,
13.0770662558912));
#24024=CARTESIAN_POINT('Ctrl Pts',(-7.93337193029169,1.2110322804593,13.1247882793461));
#24025=CARTESIAN_POINT('Ctrl Pts',(-9.2123259166928,1.13261782481115,13.172510302801));
#24026=CARTESIAN_POINT('Ctrl Pts',(-9.83805103920895,0.01160906979348,13.2202323262558));
#24027=CARTESIAN_POINT('Ctrl Pts',(-9.33379175184362,-0.928309825697517,
13.2600006791349));
#24028=CARTESIAN_POINT('Ctrl Pts',(-8.59514802384834,-1.17186954952432,
13.2918153614381));
#24029=CARTESIAN_POINT('Ctrl Pts',(-7.82688748962083,-1.050660442912,13.3236300437414));
#24030=CARTESIAN_POINT('Ctrl Pts',(-7.17760244066937,-0.204401685673198,
13.3633983966204));
#24031=CARTESIAN_POINT('Ctrl Pts',(-7.61428684534256,1.00286766641413,13.4111204200753));
#24032=CARTESIAN_POINT('Ctrl Pts',(-8.86383854258517,1.286579989206,13.4588424435302));
#24033=CARTESIAN_POINT('Ctrl Pts',(-9.77974681566496,0.390486154002405,
13.506564466985));
#24034=CARTESIAN_POINT('Ctrl Pts',(-9.51950111118942,-0.866679201500273,
13.5542864904399));
#24035=CARTESIAN_POINT('Ctrl Pts',(-8.52318422368264,-1.24756976145673,
13.5940548433189));
#24036=CARTESIAN_POINT('Ctrl Pts',(-7.80522645676502,-0.948483585079513,
13.6258695256222));
#24037=CARTESIAN_POINT('Ctrl Pts',(-7.30353144101171,-0.354162117230974,
13.6576842079254));
#24038=CARTESIAN_POINT('Ctrl Pts',(-7.36619673896916,0.710637403536776,
13.6974525608045));
#24039=CARTESIAN_POINT('Ctrl Pts',(-8.48633166710459,1.33792545582631,13.7451745842593));
#24040=CARTESIAN_POINT('Ctrl Pts',(-9.61693628164932,0.734928497495645,
13.7928966077142));
#24041=CARTESIAN_POINT('Ctrl Pts',(-9.72329964090166,-0.542004923632641,
13.840618631169));
#24042=CARTESIAN_POINT('Ctrl Pts',(-8.70395116205371,-1.32246711774871,
13.8883406546239));
#24043=CARTESIAN_POINT('Ctrl Pts',(-7.70127454044465,-0.958647723716633,
13.9281090075029));
#24044=CARTESIAN_POINT('Ctrl Pts',(-7.35400237796188,-0.26271817186398,
13.9599236898062));
#24045=CARTESIAN_POINT('Ctrl Pts',(-7.36344586906573,0.514987888581172,
13.9917383721094));
#24046=CARTESIAN_POINT('Ctrl Pts',(-8.10751259734313,1.27924547792257,14.0315067249885));
#24047=CARTESIAN_POINT('Ctrl Pts',(-9.36503971038065,1.02075347079337,14.0792287484434));
#24048=CARTESIAN_POINT('Ctrl Pts',(-9.82553500107283,-0.174995756024761,
14.1269507718982));
#24049=CARTESIAN_POINT('Ctrl Pts',(-9.07050201522982,-1.21027220049496,
14.1746727953531));
#24050=CARTESIAN_POINT('Ctrl Pts',(-7.78897637587278,-1.13356109670482,
14.2223948188079));
#24051=CARTESIAN_POINT('Ctrl Pts',(-7.2687382143401,-0.202391287121085,
14.262163171687));
#24052=CARTESIAN_POINT('Ctrl Pts',(-7.4614445292402,0.551120605402827,14.2939778539902));
#24053=CARTESIAN_POINT('Ctrl Pts',(-7.97742288800319,1.13308471878577,14.3257925362935));
#24054=CARTESIAN_POINT('Ctrl Pts',(-9.04016345797176,1.22422987739303,14.3655608891725));
#24055=CARTESIAN_POINT('Ctrl Pts',(-9.82204663964461,0.205970947654117,
14.4132829126274));
#24056=CARTESIAN_POINT('Ctrl Pts',(-9.38794421045684,-0.999610740643557,
14.4610049360823));
#24057=CARTESIAN_POINT('Ctrl Pts',(-8.13958844588438,-1.28853981713142,
14.5087269595371));
#24058=CARTESIAN_POINT('Ctrl Pts',(-7.22062088448637,-0.392051569086001,
14.556448982992));
#24059=CARTESIAN_POINT('Ctrl Pts',(-7.43643383184107,0.652529557846704,
14.596217335871));
#24060=CARTESIAN_POINT('Ctrl Pts',(-8.07517557537772,1.09629174757525,14.6280320181743));
#24061=CARTESIAN_POINT('Ctrl Pts',(-8.84615277857736,1.19881027348058,14.6598467004775));
#24062=CARTESIAN_POINT('Ctrl Pts',(-9.70948822007665,0.572410341860612,
14.6996150533566));
#24063=CARTESIAN_POINT('Ctrl Pts',(-9.63456461195216,-0.709221044626205,
14.7473370768114));
#24064=CARTESIAN_POINT('Ctrl Pts',(-8.51748651405567,-1.33692212764019,
14.7950591002663));
#24065=CARTESIAN_POINT('Ctrl Pts',(-7.38437311583038,-0.738652830313837,
14.8427811237211));
#24066=CARTESIAN_POINT('Ctrl Pts',(-7.27595421509225,0.540580495017316,
14.890503147176));
#24067=CARTESIAN_POINT('Ctrl Pts',(-8.12261089372266,1.18934657651418,14.930271500055));
#24068=CARTESIAN_POINT('Ctrl Pts',(-8.89600570638269,1.10702794383491,14.9620861823583));
#24069=CARTESIAN_POINT('Ctrl Pts',(-9.54613549047543,0.680123780107426,
14.9939008646615));
#24070=CARTESIAN_POINT('Ctrl Pts',(-9.78919550284478,-0.358455431482166,
15.0336692175406));
#24071=CARTESIAN_POINT('Ctrl Pts',(-8.89398987797994,-1.27867249171216,
15.0813912409954));
#24072=CARTESIAN_POINT('Ctrl Pts',(-7.63850424481128,-1.02249284858274,
15.1291132644503));
#24073=CARTESIAN_POINT('Ctrl Pts',(-7.17301850815132,0.171322491751843,
15.1768352879052));
#24074=CARTESIAN_POINT('Ctrl Pts',(-7.92800168663425,1.20968318577025,15.22455731136));
#24075=CARTESIAN_POINT('Ctrl Pts',(-8.99276272638861,1.1463649888735,15.2643256642391));
#24076=CARTESIAN_POINT('Ctrl Pts',(-9.52378556829048,0.57809543448961,15.2961403465423));
#24077=CARTESIAN_POINT('Ctrl Pts',(-9.73613438343296,-0.170118697936061,
15.3279550288456));
#24078=CARTESIAN_POINT('Ctrl Pts',(-9.24042793398194,-1.11457622565287,
15.3677233817246));
#24079=CARTESIAN_POINT('Ctrl Pts',(-7.96134871130471,-1.22478015611113,
15.4154454051795));
#24080=CARTESIAN_POINT('Ctrl Pts',(-7.17949357668821,-0.209604062739865,
15.4631674286343));
#24081=CARTESIAN_POINT('Ctrl Pts',(-7.60856208280836,0.997777280360243,
15.5108894520892));
#24082=CARTESIAN_POINT('Ctrl Pts',(-8.85888755748251,1.28907723916839,15.5586114755441));
#24083=CARTESIAN_POINT('Ctrl Pts',(-9.6227081975725,0.544531299390886,15.5983798284232));
#24084=CARTESIAN_POINT('Ctrl Pts',(-9.6524604840685,-0.232645704807483,
15.6301945107264));
#24085=CARTESIAN_POINT('Ctrl Pts',(-9.32356561027203,-0.937451486115936,
15.6620091930296));
#24086=CARTESIAN_POINT('Ctrl Pts',(-8.33062250286166,-1.32730170138441,
15.7017775459087));
#24087=CARTESIAN_POINT('Ctrl Pts',(-7.29143763865007,-0.5738941464571,15.7494995693635));
#24088=CARTESIAN_POINT('Ctrl Pts',(-7.36396336164215,0.705608630834335,
15.7972215928184));
#24089=CARTESIAN_POINT('Ctrl Pts',(-8.47915970912695,1.33755299057857,15.8449436162733));
#24090=CARTESIAN_POINT('Ctrl Pts',(-9.61388803974747,0.74057287343333,15.8926656397281));
#24091=CARTESIAN_POINT('Ctrl Pts',(-9.72534585944743,-0.536397493182908,
15.940387663183));
#24092=CARTESIAN_POINT('Ctrl Pts',(-8.71120078832479,-1.32093775301502,
15.9881096866378));
#24093=CARTESIAN_POINT('Ctrl Pts',(-7.50338587949291,-0.891752812389831,
16.0358317100927));
#24094=CARTESIAN_POINT('Ctrl Pts',(-7.21028788424701,0.355837225553266,
16.0835537335475));
#24095=CARTESIAN_POINT('Ctrl Pts',(-8.10323378877393,1.27788697335254,16.1312757570025));
#24096=CARTESIAN_POINT('Ctrl Pts',(-9.14870221826696,1.06595545650804,16.1710441098815));
#24097=CARTESIAN_POINT('Ctrl Pts',(-9.59472863327079,0.428787139268216,
16.2028587921847));
#24098=CARTESIAN_POINT('Ctrl Pts',(-9.70006919023239,-0.3417922930199,16.234673474488));
#24099=CARTESIAN_POINT('Ctrl Pts',(-9.07678836300807,-1.20740862666961,
16.274441827367));
#24100=CARTESIAN_POINT('Ctrl Pts',(-7.79490301569173,-1.13712765515989,
16.3221638508219));
#24101=CARTESIAN_POINT('Ctrl Pts',(-7.16314844340014,-0.0223381454320956,
16.3698858742767));
#24102=CARTESIAN_POINT('Ctrl Pts',(-7.75730541764752,1.1129404292059,16.4176078977316));
#24103=CARTESIAN_POINT('Ctrl Pts',(-9.03613551984794,1.22599852877919,16.4653299211865));
#24104=CARTESIAN_POINT('Ctrl Pts',(-9.68796982707485,0.381701814578363,
16.5050982740655));
#24105=CARTESIAN_POINT('Ctrl Pts',(-9.60845727250044,-0.39198685725222,
16.5369129563688));
#24106=CARTESIAN_POINT('Ctrl Pts',(-9.18391479352499,-1.04366103090541,
16.568727638672));
#24107=CARTESIAN_POINT('Ctrl Pts',(-8.14622411834344,-1.29048754584716,
16.6084959915511));
#24108=CARTESIAN_POINT('Ctrl Pts',(-7.22276535703482,-0.398626319625968,
16.6562180150059));
#24109=CARTESIAN_POINT('Ctrl Pts',(-7.47438832997941,0.857780428739577,
16.7039400384608));
#24110=CARTESIAN_POINT('Ctrl Pts',(-8.6665070580179,1.32759435244441,16.7516620619156));
#24111=CARTESIAN_POINT('Ctrl Pts',(-9.70759996620601,0.576383260108618,
16.7993840853705));
#24112=CARTESIAN_POINT('Ctrl Pts',(-9.64814525244498,-0.488600347920483,
16.8391524382496));
#24113=CARTESIAN_POINT('Ctrl Pts',(-9.08180588707221,-1.02168160289158,
16.8709671205528));
#24114=CARTESIAN_POINT('Ctrl Pts',(-8.33436731254839,-1.23674315419589,
16.9027818028561));
#24115=CARTESIAN_POINT('Ctrl Pts',(-7.38811706486369,-0.744467389276554,
16.9425501557351));
#24116=CARTESIAN_POINT('Ctrl Pts',(-7.27327423010892,0.534205235745406,
16.9902721791899));
#24117=CARTESIAN_POINT('Ctrl Pts',(-8.28560544341343,1.31973540062158,17.0379942026448));
#24118=CARTESIAN_POINT('Ctrl Pts',(-9.49453851638878,0.895055578304513,
17.0857162260997));
#24119=CARTESIAN_POINT('Ctrl Pts',(-9.79036691067929,-0.354215456745108,
17.1334382495546));
#24120=CARTESIAN_POINT('Ctrl Pts',(-9.04860774557578,-1.12071288000705,
17.1732066024336));
#24121=CARTESIAN_POINT('Ctrl Pts',(-8.2715278914335,-1.15331343665304,17.2050212847369));
#24122=CARTESIAN_POINT('Ctrl Pts',(-7.56556474468814,-0.826921139859261,
17.2368359670401));
#24123=CARTESIAN_POINT('Ctrl Pts',(-7.1720455135375,0.164475639288519,17.2766043199192));
#24124=CARTESIAN_POINT('Ctrl Pts',(-7.92180379170907,1.20661530463984,17.324326343374));
#24125=CARTESIAN_POINT('Ctrl Pts',(-9.20133846749202,1.13832811952868,17.3720483668289));
#24126=CARTESIAN_POINT('Ctrl Pts',(-9.83773905932737,0.0261831591494336,
17.4197703902837));
#24127=CARTESIAN_POINT('Ctrl Pts',(-9.24408855175464,-1.11213649395089,
17.4674924137386));
#24128=CARTESIAN_POINT('Ctrl Pts',(-8.18162760790967,-1.20648532435476,
17.5072607666176));
#24129=CARTESIAN_POINT('Ctrl Pts',(-7.57262853067048,-0.722712629900904,
17.5390754489209));
#24130=CARTESIAN_POINT('Ctrl Pts',(-7.25229315869388,-0.0139805610356614,
17.5708901312241));
#24131=CARTESIAN_POINT('Ctrl Pts',(-7.60334295498851,0.993237885735805,
17.6106584841032));
#24132=CARTESIAN_POINT('Ctrl Pts',(-8.85220016516547,1.29080842588264,17.658380507558));
#24133=CARTESIAN_POINT('Ctrl Pts',(-9.77517364622778,0.401993439824491,
17.7061025310129));
#24134=CARTESIAN_POINT('Ctrl Pts',(-9.52880069492294,-0.8554533761686,17.7538245544678));
#24135=CARTESIAN_POINT('Ctrl Pts',(-8.33507196537348,-1.32789837616584,
17.8015465779226));
#24136=CARTESIAN_POINT('Ctrl Pts',(-7.46985189706413,-0.70410418543467,
17.8413149308017));
#24137=CARTESIAN_POINT('Ctrl Pts',(-7.32581660245188,0.0602057843310409,
17.8731296131049));
#24138=CARTESIAN_POINT('Ctrl Pts',(-7.54727037171921,0.805775448450091,
17.9049442954082));
#24139=CARTESIAN_POINT('Ctrl Pts',(-8.47175475110896,1.33780325905746,17.9447126482872));
#24140=CARTESIAN_POINT('Ctrl Pts',(-9.61090129709441,0.74574101187086,17.9924346717421));
#24141=CARTESIAN_POINT('Ctrl Pts',(-9.72737014095729,-0.53031037212398,
18.0401566951969));
#24142=CARTESIAN_POINT('Ctrl Pts',(-8.71832882409182,-1.32006207173862,
18.0878787186518));
#24143=CARTESIAN_POINT('Ctrl Pts',(-7.50645670057225,-0.896318618679687,
18.1356007421067));
#24144=CARTESIAN_POINT('Ctrl Pts',(-7.26026654510378,0.141523067872558,
18.1753690949857));
#24145=CARTESIAN_POINT('Ctrl Pts',(-7.65141128269188,0.81377427853301,18.207183777289));
#24146=CARTESIAN_POINT('Ctrl Pts',(-8.30669695137759,1.23272127803583,18.2389984595922));
#24147=CARTESIAN_POINT('Ctrl Pts',(-9.3539359184848,1.03019842804731,18.2787668124713));
#24148=CARTESIAN_POINT('Ctrl Pts',(-9.82804542427443,-0.162870192902072,
18.3264888359261));
#24149=CARTESIAN_POINT('Ctrl Pts',(-9.08123184303367,-1.2040913994957,18.374210859381));
#24150=CARTESIAN_POINT('Ctrl Pts',(-7.80142310145517,-1.14114927397414,
18.4219328828358));
#24151=CARTESIAN_POINT('Ctrl Pts',(-7.16218719604133,-0.0277894871109879,
18.4696549062907));
#24152=CARTESIAN_POINT('Ctrl Pts',(-7.65504301923606,0.918158765457952,
18.5094232591697));
#24153=CARTESIAN_POINT('Ctrl Pts',(-8.39068732707389,1.17063321629036,18.541237941473));
#24154=CARTESIAN_POINT('Ctrl Pts',(-9.16035748349834,1.05872367117993,18.5730526237762));
#24155=CARTESIAN_POINT('Ctrl Pts',(-9.81982899665625,0.220378704994469,
18.6128209766553));
#24156=CARTESIAN_POINT('Ctrl Pts',(-9.39777622677681,-0.992083260269288,
18.6605430001101));
#24157=CARTESIAN_POINT('Ctrl Pts',(-8.15174688163843,-1.29088586608082,
18.708265023565));
#24158=CARTESIAN_POINT('Ctrl Pts',(-7.22506897755392,-0.405933783611097,
18.7559870470198));
#24159=CARTESIAN_POINT('Ctrl Pts',(-7.47009254891817,0.854286834872094,
18.8037090704747));
#24160=CARTESIAN_POINT('Ctrl Pts',(-8.4617304100637,1.24719816244857,18.8434774233538));
#24161=CARTESIAN_POINT('Ctrl Pts',(-9.18325257355315,0.956816235375206,
18.875292105657));
#24162=CARTESIAN_POINT('Ctrl Pts',(-9.69209812790066,0.368605305692601,
18.9071067879602));
#24163=CARTESIAN_POINT('Ctrl Pts',(-9.64231420404793,-0.696874173190531,
18.9468751408393));
#24164=CARTESIAN_POINT('Ctrl Pts',(-8.52984708092943,-1.3376623267597,18.9945971642942));
#24165=CARTESIAN_POINT('Ctrl Pts',(-7.39203300266752,-0.748382045828093,
19.042319187749));
#24166=CARTESIAN_POINT('Ctrl Pts',(-7.27023526017598,0.527171730423539,
19.0900412112039));
#24167=CARTESIAN_POINT('Ctrl Pts',(-8.28007094449939,1.31990399824239,19.1377632346588));
#24168=CARTESIAN_POINT('Ctrl Pts',(-9.28707397183385,0.96823673798853,19.1775315875378));
#24169=CARTESIAN_POINT('Ctrl Pts',(-9.64273672796038,0.276557694007988,
19.2093462698411));
#24170=CARTESIAN_POINT('Ctrl Pts',(-9.64269885177062,-0.501205698382487,
19.2411609521443));
#24171=CARTESIAN_POINT('Ctrl Pts',(-8.90792882316648,-1.2744055199424,19.2809293050234));
#24172=CARTESIAN_POINT('Ctrl Pts',(-7.64736768134579,-1.03113989247751,
19.3286513284782));
#24173=CARTESIAN_POINT('Ctrl Pts',(-7.17244567679856,0.158953051700663,
19.3763733519331));
#24174=CARTESIAN_POINT('Ctrl Pts',(-7.914903686496,1.20328452686644,19.4240953753879));
#24175=CARTESIAN_POINT('Ctrl Pts',(-9.1972632940707,1.14207672805785,19.4718173988428));
#24176=CARTESIAN_POINT('Ctrl Pts',(-9.72872419935639,0.217266333896879,
19.5115857517218));
#24177=CARTESIAN_POINT('Ctrl Pts',(-9.54514431649316,-0.538520886546302,
19.5434004340251));
#24178=CARTESIAN_POINT('Ctrl Pts',(-9.03624147415713,-1.12668225304333,
19.5752151163283));
#24179=CARTESIAN_POINT('Ctrl Pts',(-7.97468085007939,-1.2306726391516,19.6149834692074));
#24180=CARTESIAN_POINT('Ctrl Pts',(-7.18054087470649,-0.221943608495227,
19.6627054926623));
#24181=CARTESIAN_POINT('Ctrl Pts',(-7.60003226709561,0.988799592145305,
19.7104275161171));
#24182=CARTESIAN_POINT('Ctrl Pts',(-8.84480267997769,1.29280410757097,19.7581495395719));
#24183=CARTESIAN_POINT('Ctrl Pts',(-9.77454441836398,0.407494637568213,
19.8058715630269));
#24184=CARTESIAN_POINT('Ctrl Pts',(-9.57137953974861,-0.639619965086357,
19.8456399159058));
#24185=CARTESIAN_POINT('Ctrl Pts',(-8.93805099162274,-1.09107411126967,
19.8774545982092));
#24186=CARTESIAN_POINT('Ctrl Pts',(-8.16836993911467,-1.20290869173274,
19.9092692805123));
#24187=CARTESIAN_POINT('Ctrl Pts',(-7.29752247389199,-0.586995019770082,
19.9490376333915));
#24188=CARTESIAN_POINT('Ctrl Pts',(-7.35694162901394,0.695448710683165,
19.9967596568463));
#24189=CARTESIAN_POINT('Ctrl Pts',(-8.46634715042567,1.33661289811648,20.0444816803011));
#24190=CARTESIAN_POINT('Ctrl Pts',(-9.60661265683251,0.752090271450374,
20.092203703756));
#24191=CARTESIAN_POINT('Ctrl Pts',(-9.73049360305648,-0.525738382531365,
20.1399257272109));
#24192=CARTESIAN_POINT('Ctrl Pts',(-8.8917444696308,-1.18469577885746,20.1796940800899));
#24193=CARTESIAN_POINT('Ctrl Pts',(-8.11741071746799,-1.11173595265972,
20.2115087623932));
#24194=CARTESIAN_POINT('Ctrl Pts',(-7.46216585637197,-0.692725131815518,
20.2433234446964));
#24195=CARTESIAN_POINT('Ctrl Pts',(-7.20656390593258,0.342838773468356,
20.2830917975755));
#24196=CARTESIAN_POINT('Ctrl Pts',(-8.09057574803475,1.27381440193415,20.3308138210303));
#24197=CARTESIAN_POINT('Ctrl Pts',(-9.34906757443192,1.03283629280933,20.3785358444852));
#24198=CARTESIAN_POINT('Ctrl Pts',(-9.82895631258486,-0.155262577310471,
20.42625786794));
#24199=CARTESIAN_POINT('Ctrl Pts',(-9.08658532806561,-1.20267743261765,
20.4739798913949));
#24200=CARTESIAN_POINT('Ctrl Pts',(-8.0211365721744,-1.1522402680952,20.5137482442739));
#24201=CARTESIAN_POINT('Ctrl Pts',(-7.48328017774149,-0.59043390025575,
20.5455629265772));
#24202=CARTESIAN_POINT('Ctrl Pts',(-7.26189902630817,0.155157329418629,
20.5773776088804));
#24203=CARTESIAN_POINT('Ctrl Pts',(-7.74614684401822,1.10554094146076,20.6171459617595));
#24204=CARTESIAN_POINT('Ctrl Pts',(-9.02380147086936,1.23120403174586,20.6648679852144));
#24205=CARTESIAN_POINT('Ctrl Pts',(-9.81787319462849,0.225558853906263,
20.7125900086692));
#24206=CARTESIAN_POINT('Ctrl Pts',(-9.40344259165754,-0.986925950743689,
20.7603120321241));
#24207=CARTESIAN_POINT('Ctrl Pts',(-8.15672060120297,-1.2933192213801,20.8080340555789));
#24208=CARTESIAN_POINT('Ctrl Pts',(-7.38397141561257,-0.558075278756529,
20.847802408458));
#24209=CARTESIAN_POINT('Ctrl Pts',(-7.34479379924817,0.218700757404031,
20.8796170907612));
#24210=CARTESIAN_POINT('Ctrl Pts',(-7.66519819859131,0.927401622973458,
20.9114317730645));
#24211=CARTESIAN_POINT('Ctrl Pts',(-8.65322818924572,1.32929924247707,20.9512001259435));
#24212=CARTESIAN_POINT('Ctrl Pts',(-9.70167745526272,0.588389872606148,
20.9989221493984));
#24213=CARTESIAN_POINT('Ctrl Pts',(-9.64422438454522,-0.691677028321677,
21.0466441728533));
#24214=CARTESIAN_POINT('Ctrl Pts',(-8.53750660713187,-1.33746947744374,
21.0943661963081));
#24215=CARTESIAN_POINT('Ctrl Pts',(-7.39420230150788,-0.753476478756427,
21.142088219763));
#24216=CARTESIAN_POINT('Ctrl Pts',(-7.29086278230429,0.308147702753215,
21.181856572642));
#24217=CARTESIAN_POINT('Ctrl Pts',(-7.76946277180434,0.921220248238589,
21.2136712549453));
#24218=CARTESIAN_POINT('Ctrl Pts',(-8.47545770507547,1.24754378427726,21.2454859372485));
#24219=CARTESIAN_POINT('Ctrl Pts',(-9.48561180981664,0.905032990768657,
21.2852542901276));
#24220=CARTESIAN_POINT('Ctrl Pts',(-9.79374366065181,-0.34126044188475,
21.3329763135824));
#24221=CARTESIAN_POINT('Ctrl Pts',(-8.91277378588204,-1.2717249527254,21.3806983370373));
#24222=CARTESIAN_POINT('Ctrl Pts',(-7.65328640071379,-1.03600551613202,
21.4284203604922));
#24223=CARTESIAN_POINT('Ctrl Pts',(-7.17075303613647,0.153681043363308,
21.476142383947));
#24224=CARTESIAN_POINT('Ctrl Pts',(-7.78720051264544,1.02415072560441,21.5159107368261));
#24225=CARTESIAN_POINT('Ctrl Pts',(-8.55026379154953,1.1746509859544,21.5477254191293));
#24226=CARTESIAN_POINT('Ctrl Pts',(-9.29768141734801,0.95951663578424,21.5795401014325));
#24227=CARTESIAN_POINT('Ctrl Pts',(-9.83751621862897,0.0395691664571907,
21.6193084543116));
#24228=CARTESIAN_POINT('Ctrl Pts',(-9.25511842332855,-1.10454855729479,
21.6670304777665));
#24229=CARTESIAN_POINT('Ctrl Pts',(-7.98009870786515,-1.23181540830285,
21.7147525012213));
#24230=CARTESIAN_POINT('Ctrl Pts',(-7.18183345085486,-0.229495745901632,
21.7624745246762));
#24231=CARTESIAN_POINT('Ctrl Pts',(-7.59530283801286,0.985920077451556,
21.810196548131));
#24232=CARTESIAN_POINT('Ctrl Pts',(-8.63102325931338,1.24088707119056,21.8499649010101));
#24233=CARTESIAN_POINT('Ctrl Pts',(-9.30656154672025,0.855447168968843,
21.8817795833133));
#24234=CARTESIAN_POINT('Ctrl Pts',(-9.73104073612964,0.203731499573318,
21.9135942656166));
#24235=CARTESIAN_POINT('Ctrl Pts',(-9.53739035341218,-0.845184363720151,
21.9533626184956));
#24236=CARTESIAN_POINT('Ctrl Pts',(-8.3483779694346,-1.32937658641915,22.0010846419505));
#24237=CARTESIAN_POINT('Ctrl Pts',(-7.30087205705786,-0.591404032917553,
22.0488066654053));
#24238=CARTESIAN_POINT('Ctrl Pts',(-7.35297793965443,0.688891676356153,
22.0965286888602));
#24239=CARTESIAN_POINT('Ctrl Pts',(-8.46088649819163,1.33752962135645,22.1442507123151));
#24240=CARTESIAN_POINT('Ctrl Pts',(-9.410973037202,0.85269921040183,22.1840190651941));
#24241=CARTESIAN_POINT('Ctrl Pts',(-9.66966590430475,0.11921853820421,22.2158337474974));
#24242=CARTESIAN_POINT('Ctrl Pts',(-9.56427587148831,-0.651371389682384,
22.2476484298006));
#24243=CARTESIAN_POINT('Ctrl Pts',(-8.73154358029947,-1.31791612952105,
22.2874167826797));
#24244=CARTESIAN_POINT('Ctrl Pts',(-7.51555224850724,-0.906142358160704,
22.3351388061345));
#24245=CARTESIAN_POINT('Ctrl Pts',(-7.20621231493002,0.337312880953408,
22.3828608295894));
#24246=CARTESIAN_POINT('Ctrl Pts',(-8.08328806540698,1.27144898137517,22.4305828530443));
#24247=CARTESIAN_POINT('Ctrl Pts',(-9.34553773074606,1.03710235749152,22.4783048764991));
#24248=CARTESIAN_POINT('Ctrl Pts',(-9.74682950929964,0.0488261473860323,
22.5180732293782));
#24249=CARTESIAN_POINT('Ctrl Pts',(-9.46256590138573,-0.675128338195107,
22.5498879116814));
#24250=CARTESIAN_POINT('Ctrl Pts',(-8.87868358743782,-1.18893505227754,
22.5817025939847));
#24251=CARTESIAN_POINT('Ctrl Pts',(-7.81282084949026,-1.14817253456714,
22.6214709468637));
#24252=CARTESIAN_POINT('Ctrl Pts',(-7.1626382686361,-0.0411697480629679,
22.6691929703186));
#24253=CARTESIAN_POINT('Ctrl Pts',(-7.74226547712604,1.1015920054815,22.7169149937735));
#24254=CARTESIAN_POINT('Ctrl Pts',(-9.01674249185626,1.23418335176844,22.7646370172283));
#24255=CARTESIAN_POINT('Ctrl Pts',(-9.81799493484566,0.231094581829405,
22.8123590406832));
#24256=CARTESIAN_POINT('Ctrl Pts',(-9.47486487590842,-0.778849338222097,
22.8521273935622));
#24257=CARTESIAN_POINT('Ctrl Pts',(-8.78622141401848,-1.14035463330573,
22.8839420758655));
#24258=CARTESIAN_POINT('Ctrl Pts',(-8.00848556937946,-1.1469007727004,22.9157567581687));
#24259=CARTESIAN_POINT('Ctrl Pts',(-7.2290933909427,-0.418702454117604,
22.9555251110478));
#24260=CARTESIAN_POINT('Ctrl Pts',(-7.46167925127839,0.843872840803867,
23.0032471345026));
#24261=CARTESIAN_POINT('Ctrl Pts',(-8.64770918704739,1.32885234309821,23.0509691579575));
#24262=CARTESIAN_POINT('Ctrl Pts',(-9.69828838525392,0.595261534485202,
23.0986911814123));
#24263=CARTESIAN_POINT('Ctrl Pts',(-9.64793836111807,-0.687570267756874,
23.1464132048672));
#24264=CARTESIAN_POINT('Ctrl Pts',(-8.72766008966769,-1.22684094384785,
23.1861815577462));
#24265=CARTESIAN_POINT('Ctrl Pts',(-7.97034588813662,-1.04966561786637,
23.2179962400495));
#24266=CARTESIAN_POINT('Ctrl Pts',(-7.37789757206185,-0.545759983091795,
23.2498109223527));
#24267=CARTESIAN_POINT('Ctrl Pts',(-7.26492446411792,0.514882292077699,
23.2895792752318));
#24268=CARTESIAN_POINT('Ctrl Pts',(-8.26689470335111,1.31753302400601,23.3373012986866));
#24269=CARTESIAN_POINT('Ctrl Pts',(-9.48114564923169,0.908305988469492,
23.3850233221415));
#24270=CARTESIAN_POINT('Ctrl Pts',(-9.79567664876958,-0.333846327679993,
23.4327453455963));
#24271=CARTESIAN_POINT('Ctrl Pts',(-8.9182694598961,-1.271049178021,23.4804673690513));
#24272=CARTESIAN_POINT('Ctrl Pts',(-7.86947252162285,-1.07675573689688,
23.5202357219303));
#24273=CARTESIAN_POINT('Ctrl Pts',(-7.4126732243127,-0.447271584630692,
23.5520504042335));
#24274=CARTESIAN_POINT('Ctrl Pts',(-7.29432705639192,0.321435173838232,
23.5838650865367));
#24275=CARTESIAN_POINT('Ctrl Pts',(-7.90284665879995,1.19746534025971,23.6236334394159));
#24276=CARTESIAN_POINT('Ctrl Pts',(-9.18574743946922,1.14890460784766,23.6713554628707));
#24277=CARTESIAN_POINT('Ctrl Pts',(-9.83628012328246,0.0449664965947858,
23.7190774863255));
#24278=CARTESIAN_POINT('Ctrl Pts',(-9.26143115070254,-1.10020632220142,
23.7667995097804));
#24279=CARTESIAN_POINT('Ctrl Pts',(-7.98469697473584,-1.23490005513938,
23.8145215332353));
#24280=CARTESIAN_POINT('Ctrl Pts',(-7.31866291190331,-0.40175925902985,
23.8542898861143));
#24281=CARTESIAN_POINT('Ctrl Pts',(-7.38506514261205,0.373164375745999,
23.8861045684176));
#24282=CARTESIAN_POINT('Ctrl Pts',(-7.79851409376019,1.03193281819888,23.9179192507208));
#24283=CARTESIAN_POINT('Ctrl Pts',(-8.83187714157381,1.29629198752846,23.9576876035999));
#24284=CARTESIAN_POINT('Ctrl Pts',(-9.77030285294977,0.420192825331216,
24.0054096270547));
#24285=CARTESIAN_POINT('Ctrl Pts',(-9.5399869115765,-0.840293863743771,
24.0531316505096));
#24286=CARTESIAN_POINT('Ctrl Pts',(-8.35599302339332,-1.33022304120804,
24.1008536739645));
#24287=CARTESIAN_POINT('Ctrl Pts',(-7.30233129222316,-0.596745356447589,
24.1485756974192));
#24288=CARTESIAN_POINT('Ctrl Pts',(-7.34374728727658,0.469092189498782,
24.1883440502984));
#24289=CARTESIAN_POINT('Ctrl Pts',(-7.90098039951627,1.01168518116105,24.2201587326016));
#24290=CARTESIAN_POINT('Ctrl Pts',(-8.64467085179622,1.23937006683619,24.2519734149049));
#24291=CARTESIAN_POINT('Ctrl Pts',(-9.59911972185314,0.763184899656127,
24.2917417677839));
#24292=CARTESIAN_POINT('Ctrl Pts',(-9.73559406180045,-0.513360168999922,
24.3394637912387));
#24293=CARTESIAN_POINT('Ctrl Pts',(-8.73670698711347,-1.31591654596616,
24.3871858146937));
#24294=CARTESIAN_POINT('Ctrl Pts',(-7.52075734081801,-0.911764861743639,
24.4349078381485));
#24295=CARTESIAN_POINT('Ctrl Pts',(-7.20382115093774,0.332318740478653,
24.4826298616033));
#24296=CARTESIAN_POINT('Ctrl Pts',(-7.9324971813356,1.11126431092559,24.5223982144824));
#24297=CARTESIAN_POINT('Ctrl Pts',(-8.70891373351908,1.15701617944249,24.5542128967856));
#24298=CARTESIAN_POINT('Ctrl Pts',(-9.42030153035235,0.842622638646819,
24.5860275790888));
#24299=CARTESIAN_POINT('Ctrl Pts',(-9.83054873707127,-0.141969758426454,
24.625795931968));
#24300=CARTESIAN_POINT('Ctrl Pts',(-9.09854137120265,-1.19665349020969,
24.6735179554228));
#24301=CARTESIAN_POINT('Ctrl Pts',(-7.81803397842269,-1.15003865113736,
24.7212399788777));
#24302=CARTESIAN_POINT('Ctrl Pts',(-7.16289595136489,-0.0488273672827691,
24.7689620023325));
#24303=CARTESIAN_POINT('Ctrl Pts',(-7.73718959054251,1.09937965837695,24.8166840257874));
#24304=CARTESIAN_POINT('Ctrl Pts',(-8.79790093066177,1.21170246077156,24.8564523786664));
#24305=CARTESIAN_POINT('Ctrl Pts',(-9.41500300984422,0.738309474082921,
24.8882670609697));
#24306=CARTESIAN_POINT('Ctrl Pts',(-9.74729132465791,0.0351022700416287,
24.9200817432729));
#24307=CARTESIAN_POINT('Ctrl Pts',(-9.41334407924803,-0.977915102108688,
24.9598500961519));
#24308=CARTESIAN_POINT('Ctrl Pts',(-8.16970373710478,-1.29658618201399,
25.0075721196068));
#24309=CARTESIAN_POINT('Ctrl Pts',(-7.23181487625983,-0.423524551377999,
25.0552941430617));
#24310=CARTESIAN_POINT('Ctrl Pts',(-7.45686390580615,0.837913144461989,
25.1030161665166));
#24311=CARTESIAN_POINT('Ctrl Pts',(-8.64242303887271,1.33050029388494,25.1507381899714));
#24312=CARTESIAN_POINT('Ctrl Pts',(-9.51807995467424,0.721443708004637,
25.1905065428505));
#24313=CARTESIAN_POINT('Ctrl Pts',(-9.67503439547865,-0.040318196719616,
25.2223212251537));
#24314=CARTESIAN_POINT('Ctrl Pts',(-9.46623488155447,-0.789530222091854,
25.2541359074569));
#24315=CARTESIAN_POINT('Ctrl Pts',(-8.55089024838259,-1.33713332792553,
25.293904260336));
#24316=CARTESIAN_POINT('Ctrl Pts',(-7.40188333764438,-0.764441720819265,
25.3416262837908));
#24317=CARTESIAN_POINT('Ctrl Pts',(-7.26382759980121,0.509454954517635,
25.3893483072458));
#24318=CARTESIAN_POINT('Ctrl Pts',(-8.25935377861649,1.31617656292992,25.4370703307005));
#24319=CARTESIAN_POINT('Ctrl Pts',(-9.47822620159528,0.913010872083186,
25.4847923541555));
#24320=CARTESIAN_POINT('Ctrl Pts',(-9.7419517619337,-0.120514061249036,
25.5245607070345));
#24321=CARTESIAN_POINT('Ctrl Pts',(-9.36224431681492,-0.799291014377719,
25.5563753893377));
#24322=CARTESIAN_POINT('Ctrl Pts',(-8.71414535053657,-1.22927197428909,
25.588190071641));
#24323=CARTESIAN_POINT('Ctrl Pts',(-7.66362775939689,-1.04450793638833,
25.62795842452));
#24324=CARTESIAN_POINT('Ctrl Pts',(-7.16938751840154,0.140363002556102,
25.6756804479749));
#24325=CARTESIAN_POINT('Ctrl Pts',(-7.89846615891949,1.19407855341712,25.7234024714298));
#24326=CARTESIAN_POINT('Ctrl Pts',(-9.17915708620039,1.15281264780359,25.7711244948846));
#24327=CARTESIAN_POINT('Ctrl Pts',(-9.83715058751881,0.050434713519313,
25.8188465183394));
#24328=CARTESIAN_POINT('Ctrl Pts',(-9.36038033315174,-0.903722025987354,
25.8586148712185));
#24329=CARTESIAN_POINT('Ctrl Pts',(-8.62911585993756,-1.16861477068243,
25.8904295535218));
#24330=CARTESIAN_POINT('Ctrl Pts',(-7.85766138328856,-1.06975180271418,
25.922244235825));
#24331=CARTESIAN_POINT('Ctrl Pts',(-7.18409118329007,-0.24269186252281,
25.9620125887041));
#24332=CARTESIAN_POINT('Ctrl Pts',(-7.58555644723375,0.976741694347291,
26.0097346121589));
#24333=CARTESIAN_POINT('Ctrl Pts',(-8.82634847073002,1.29659678749717,26.0574566356138));
#24334=CARTESIAN_POINT('Ctrl Pts',(-9.76787582459831,0.427460222794269,
26.1051786590687));
#24335=CARTESIAN_POINT('Ctrl Pts',(-9.54422294215118,-0.836728032944274,
26.1529006825235));
#24336=CARTESIAN_POINT('Ctrl Pts',(-8.55937920581306,-1.24637150474729,
26.1926690354026));
#24337=CARTESIAN_POINT('Ctrl Pts',(-7.83304427880943,-0.968246587143855,
26.2244837177057));
#24338=CARTESIAN_POINT('Ctrl Pts',(-7.31431322586505,-0.388734731623603,
26.2562984000091));
#24339=CARTESIAN_POINT('Ctrl Pts',(-7.34605141627337,0.677434882586455,
26.2960667528881));
#24340=CARTESIAN_POINT('Ctrl Pts',(-8.4475105351465,1.33696529676412,26.343788776343));
#24341=CARTESIAN_POINT('Ctrl Pts',(-9.595138070366,0.767032698475656,26.3915107997978));
#24342=CARTESIAN_POINT('Ctrl Pts',(-9.73851351856959,-0.506276222029613,
26.4392328232527));
#24343=CARTESIAN_POINT('Ctrl Pts',(-8.74224354725321,-1.31599142012546,
26.4869548467075));
#24344=CARTESIAN_POINT('Ctrl Pts',(-7.72943110998268,-0.981423152196046,
26.5267231995866));
#24345=CARTESIAN_POINT('Ctrl Pts',(-7.36210918245529,-0.295864622575958,
26.5585378818898));
#24346=CARTESIAN_POINT('Ctrl Pts',(-7.34897949659139,0.48178793951492,26.5903525641931));
#24347=CARTESIAN_POINT('Ctrl Pts',(-8.07055392035829,1.26731662133423,26.6301209170721));
#24348=CARTESIAN_POINT('Ctrl Pts',(-9.33505288858864,1.0454271959022,26.677842940527));
#24349=CARTESIAN_POINT('Ctrl Pts',(-9.83005513359837,-0.136454737127118,
26.7255649639818));
#24350=CARTESIAN_POINT('Ctrl Pts',(-9.10538409730576,-1.1932063708351,26.7732869874367));
#24351=CARTESIAN_POINT('Ctrl Pts',(-7.82217203182808,-1.15371772960008,
26.8210090108916));
#24352=CARTESIAN_POINT('Ctrl Pts',(-7.27513023062585,-0.238037530659098,
26.8607773637706));
#24353=CARTESIAN_POINT('Ctrl Pts',(-7.44588830282998,0.520749380637105,
26.8925920460739));
#24354=CARTESIAN_POINT('Ctrl Pts',(-7.94476061870995,1.11744218973226,26.9244067283771));
#24355=CARTESIAN_POINT('Ctrl Pts',(-9.00440853628265,1.23938992353288,26.9641750812562));
#24356=CARTESIAN_POINT('Ctrl Pts',(-9.81551250449702,0.244250279803835,
27.011897104711));
#24357=CARTESIAN_POINT('Ctrl Pts',(-9.41657915220431,-0.973421394587272,
27.0596191281659));
#24358=CARTESIAN_POINT('Ctrl Pts',(-8.17713394900972,-1.29845633803764,
27.1073411516208));
#24359=CARTESIAN_POINT('Ctrl Pts',(-7.23253714937687,-0.429014307826603,
27.1550631750756));
#24360=CARTESIAN_POINT('Ctrl Pts',(-7.4179452293806,0.621389806247837,27.1948315279547));
#24361=CARTESIAN_POINT('Ctrl Pts',(-8.04353987513476,1.08350151912796,27.2266462102579));
#24362=CARTESIAN_POINT('Ctrl Pts',(-8.81121725181817,1.20835079347835,27.2584608925612));
#24363=CARTESIAN_POINT('Ctrl Pts',(-9.69236734058681,0.607268868897116,
27.2982292454402));
#24364=CARTESIAN_POINT('Ctrl Pts',(-9.65466851088711,-0.675997025613207,
27.3459512688951));
#24365=CARTESIAN_POINT('Ctrl Pts',(-8.55627692118636,-1.33585158675565,
27.3936732923499));
#24366=CARTESIAN_POINT('Ctrl Pts',(-7.40627885639209,-0.770717463599528,
27.4413953158048));
#24367=CARTESIAN_POINT('Ctrl Pts',(-7.26078198928205,0.504830739893935,
27.4891173392597));
#24368=CARTESIAN_POINT('Ctrl Pts',(-8.08825474279979,1.17789373930847,27.5288856921387));
#24369=CARTESIAN_POINT('Ctrl Pts',(-8.86371272692307,1.11805386266439,27.5607003744419));
#24370=CARTESIAN_POINT('Ctrl Pts',(-9.52595754148374,0.71019641015823,27.5925150567452));
#24371=CARTESIAN_POINT('Ctrl Pts',(-9.79905498496199,-0.320891726404749,
27.6322834096242));
#24372=CARTESIAN_POINT('Ctrl Pts',(-8.93093128646595,-1.26670027039429,
27.6800054330791));
#24373=CARTESIAN_POINT('Ctrl Pts',(-7.66854006482953,-1.04706300187818,
27.727727456534));
#24374=CARTESIAN_POINT('Ctrl Pts',(-7.16860555779351,0.132741055946924,
27.7754494799888));
#24375=CARTESIAN_POINT('Ctrl Pts',(-7.89313737966605,1.19257415453759,27.8231715034437));
#24376=CARTESIAN_POINT('Ctrl Pts',(-8.95928733467085,1.16018229694298,27.8629398563227));
#24377=CARTESIAN_POINT('Ctrl Pts',(-9.50657803978175,0.607562373237274,
27.894754538626));
#24378=CARTESIAN_POINT('Ctrl Pts',(-9.74055034314229,-0.134174006642727,
27.9265692209292));
#24379=CARTESIAN_POINT('Ctrl Pts',(-9.27246195129652,-1.09261973615198,
27.9663375738083));
#24380=CARTESIAN_POINT('Ctrl Pts',(-7.99711792174184,-1.23989554561622,
28.0140595972632));
#24381=CARTESIAN_POINT('Ctrl Pts',(-7.18613440507626,-0.247838157214425,
28.061781620718));
#24382=CARTESIAN_POINT('Ctrl Pts',(-7.5799782078733,0.971489192263182,28.1095036441729));
#24383=CARTESIAN_POINT('Ctrl Pts',(-8.82133426723954,1.29894558882478,28.1572256676277));
#24384=CARTESIAN_POINT('Ctrl Pts',(-9.60642040105378,0.57688968968145,28.1969940205068));
#24385=CARTESIAN_POINT('Ctrl Pts',(-9.65874324301241,-0.19911173827254,
28.22880870281));
#24386=CARTESIAN_POINT('Ctrl Pts',(-9.35038309111296,-0.913135486265807,
28.2606233851133));
#24387=CARTESIAN_POINT('Ctrl Pts',(-8.36929884635634,-1.33170288070013,
28.3003917379923));
#24388=CARTESIAN_POINT('Ctrl Pts',(-7.30845623048737,-0.608649976596389,
28.3481137614472));
#24389=CARTESIAN_POINT('Ctrl Pts',(-7.3442294973634,0.672206143179074,28.395835784902));
#24390=CARTESIAN_POINT('Ctrl Pts',(-8.43985537167285,1.33664279908731,28.4435578083569));
#24391=CARTESIAN_POINT('Ctrl Pts',(-9.59288283354739,0.77208967496468,28.4912798318118));
#24392=CARTESIAN_POINT('Ctrl Pts',(-9.71418086973746,-0.287632810134326,
28.5310481846908));
#24393=CARTESIAN_POINT('Ctrl Pts',(-9.24602881059754,-0.908720199684553,
28.5628628669941));
#24394=CARTESIAN_POINT('Ctrl Pts',(-8.54565972958893,-1.24694948055712,
28.5946775492973));
#24395=CARTESIAN_POINT('Ctrl Pts',(-7.52985168590447,-0.921589714816851,
28.6344459021763));
#24396=CARTESIAN_POINT('Ctrl Pts',(-7.20066421359191,0.319308413860887,
28.6821679256312));
#24397=CARTESIAN_POINT('Ctrl Pts',(-8.0657550343786,1.26455441305737,28.7298899490861));
#24398=CARTESIAN_POINT('Ctrl Pts',(-9.32905264186954,1.05019191790068,28.7776119725409));
#24399=CARTESIAN_POINT('Ctrl Pts',(-9.83165827738984,-0.131154827519194,
28.8253339959958));
#24400=CARTESIAN_POINT('Ctrl Pts',(-9.23003622620806,-1.01193622592216,
28.8651023488749));
#24401=CARTESIAN_POINT('Ctrl Pts',(-8.46963028970779,-1.1753335976729,28.8969170311781));
#24402=CARTESIAN_POINT('Ctrl Pts',(-7.71867754763184,-0.972883886508505,
28.9287317134813));
#24403=CARTESIAN_POINT('Ctrl Pts',(-7.16334539739647,-0.0622076783419375,
28.9685000663604));
#24404=CARTESIAN_POINT('Ctrl Pts',(-7.72628974401962,1.09160606477463,29.0162220898152));
#24405=CARTESIAN_POINT('Ctrl Pts',(-8.99897214403931,1.24044081982536,29.0639441132701));
#24406=CARTESIAN_POINT('Ctrl Pts',(-9.81409218726597,0.251779422282355,
29.111666136725));
#24407=CARTESIAN_POINT('Ctrl Pts',(-9.42125928897337,-0.970462165325127,
29.1593881601799));
#24408=CARTESIAN_POINT('Ctrl Pts',(-8.39000353594678,-1.24292755198914,
29.1991565130589));
#24409=CARTESIAN_POINT('Ctrl Pts',(-7.70803711420451,-0.868979538690246,
29.2309711953621));
#24410=CARTESIAN_POINT('Ctrl Pts',(-7.2725841095908,-0.224544184030418,
29.2627858776653));
#24411=CARTESIAN_POINT('Ctrl Pts',(-7.44845097068834,0.827500878887188,
29.3025542305445));
#24412=CARTESIAN_POINT('Ctrl Pts',(-8.62909116778061,1.33175184955349,29.3502762539992));
#24413=CARTESIAN_POINT('Ctrl Pts',(-9.68894861733642,0.611622684002498,
29.3979982774542));
#24414=CARTESIAN_POINT('Ctrl Pts',(-9.65851111003362,-0.669377881206477,
29.445720300909));
#24415=CARTESIAN_POINT('Ctrl Pts',(-8.56177118348423,-1.33666768258405,
29.4934423243639));
#24416=CARTESIAN_POINT('Ctrl Pts',(-7.60356077414914,-0.868013858452832,
29.533210677243));
#24417=CARTESIAN_POINT('Ctrl Pts',(-7.33256413054386,-0.138985158650351,
29.5650253595461));
#24418=CARTESIAN_POINT('Ctrl Pts',(-7.42474175056611,0.633214111788515,
29.5968400418494));
#24419=CARTESIAN_POINT('Ctrl Pts',(-8.24640486169936,1.31390426831433,29.6366083947285));
#24420=CARTESIAN_POINT('Ctrl Pts',(-9.46858362546016,0.922516240590384,
29.6843304181833));
#24421=CARTESIAN_POINT('Ctrl Pts',(-9.8000120392334,-0.315061926833937,
29.7320524416382));
#24422=CARTESIAN_POINT('Ctrl Pts',(-8.93684997703512,-1.26478329921426,
29.7797744650931));
#24423=CARTESIAN_POINT('Ctrl Pts',(-7.88515752754028,-1.08587738685972,
29.8195428179721));
#24424=CARTESIAN_POINT('Ctrl Pts',(-7.41918288393529,-0.462897910902516,
29.8513575002754));
#24425=CARTESIAN_POINT('Ctrl Pts',(-7.29010085348255,0.303653650183876,
29.8831721825785));
#24426=CARTESIAN_POINT('Ctrl Pts',(-7.8848103649759,1.18921135372836,29.9229405354577));
#24427=CARTESIAN_POINT('Ctrl Pts',(-9.17027425724991,1.15778987946344,29.9706625589125));
#24428=CARTESIAN_POINT('Ctrl Pts',(-9.72243084515013,0.248331434474197,
30.0104309117915));
#24429=CARTESIAN_POINT('Ctrl Pts',(-9.55852849210566,-0.515011305712282,
30.0422455940948));
#24430=CARTESIAN_POINT('Ctrl Pts',(-9.31003111705877,-0.811448288777166,
30.0581529352464));
#24431=CARTESIAN_POINT('Ctrl Pts',(-9.15663776199785,-0.920831852263732,
30.0661066058222));
#24432=CARTESIAN_POINT('Ctrl Pts',(-9.0118388111672,1.0723337549513,1.79999999999999));
#24433=CARTESIAN_POINT('Ctrl Pts',(-9.19046954816081,0.987070987050382,
1.8079536705758));
#24434=CARTESIAN_POINT('Ctrl Pts',(-9.50155426450738,0.725568290707912,
1.82386101172742));
#24435=CARTESIAN_POINT('Ctrl Pts',(-9.81008998255101,-0.0344549071383838,
1.85567569403066));
#24436=CARTESIAN_POINT('Ctrl Pts',(-9.40429116407483,-1.07600298498373,
1.89544404690971));
#24437=CARTESIAN_POINT('Ctrl Pts',(-8.07989827787013,-1.34249070178545,
1.94316607036458));
#24438=CARTESIAN_POINT('Ctrl Pts',(-7.30334704707155,-0.534421386282276,
1.98293442324363));
#24439=CARTESIAN_POINT('Ctrl Pts',(-7.29738792476634,0.282249903129412,
2.01474910554687));
#24440=CARTESIAN_POINT('Ctrl Pts',(-7.66615515840917,1.01168221201408,2.04656378785011));
#24441=CARTESIAN_POINT('Ctrl Pts',(-8.72181247099373,1.38822684395207,2.08633214072916));
#24442=CARTESIAN_POINT('Ctrl Pts',(-9.78781926187509,0.562627888122653,
2.13405416418403));
#24443=CARTESIAN_POINT('Ctrl Pts',(-9.67013820971537,-0.778260502859383,
2.18177618763889));
#24444=CARTESIAN_POINT('Ctrl Pts',(-8.4767481821154,-1.40569864308939,2.22949821109375));
#24445=CARTESIAN_POINT('Ctrl Pts',(-7.50264969202872,-0.850921733780454,
2.2692665639728));
#24446=CARTESIAN_POINT('Ctrl Pts',(-7.26671790307987,-0.0686793482260387,
2.30108124627604));
#24447=CARTESIAN_POINT('Ctrl Pts',(-7.41443229219623,0.734996509964761,
2.33289592857928));
#24448=CARTESIAN_POINT('Ctrl Pts',(-8.32062191059588,1.39433769122372,2.37266428145833));
#24449=CARTESIAN_POINT('Ctrl Pts',(-9.57691242085731,0.903494929509702,
2.4203863049132));
#24450=CARTESIAN_POINT('Ctrl Pts',(-9.84156959790808,-0.416458701888548,
2.46810832836806));
#24451=CARTESIAN_POINT('Ctrl Pts',(-8.87597493033133,-1.35451113192682,
2.51583035182292));
#24452=CARTESIAN_POINT('Ctrl Pts',(-7.5625456899844,-1.04764123587607,2.56355237527778));
#24453=CARTESIAN_POINT('Ctrl Pts',(-7.18908148385554,0.00893409317419132,
2.60332072815684));
#24454=CARTESIAN_POINT('Ctrl Pts',(-7.52236165481741,0.755012087082508,
2.63513541046008));
#24455=CARTESIAN_POINT('Ctrl Pts',(-8.15995042754744,1.26607722708645,2.66695009276332));
#24456=CARTESIAN_POINT('Ctrl Pts',(-9.27661796922437,1.17185321198702,2.70671844564237));
#24457=CARTESIAN_POINT('Ctrl Pts',(-9.90556259985949,-0.0213388321026141,
2.75444046909723));
#24458=CARTESIAN_POINT('Ctrl Pts',(-9.24208297580843,-1.19270436179778,
2.8021624925521));
#24459=CARTESIAN_POINT('Ctrl Pts',(-7.89810602223727,-1.27034854887012,
2.84988451600696));
#24460=CARTESIAN_POINT('Ctrl Pts',(-7.10559639405835,-0.178924052943307,
2.89760653946182));
#24461=CARTESIAN_POINT('Ctrl Pts',(-7.51445941986352,0.864462087680646,
2.93737489234087));
#24462=CARTESIAN_POINT('Ctrl Pts',(-8.25464604367347,1.21062885803132,2.96918957464412));
#24463=CARTESIAN_POINT('Ctrl Pts',(-9.07120418959933,1.17996215792738,3.00100425694735));
#24464=CARTESIAN_POINT('Ctrl Pts',(-9.85403869080924,0.378093235837854,
3.04077260982641));
#24465=CARTESIAN_POINT('Ctrl Pts',(-9.54899988060095,-0.935767616312688,
3.08849463328127));
#24466=CARTESIAN_POINT('Ctrl Pts',(-8.2808413597343,-1.38751585434482,3.13621665673613));
#24467=CARTESIAN_POINT('Ctrl Pts',(-7.21365340752345,-0.566898780222384,
3.183938680191));
#24468=CARTESIAN_POINT('Ctrl Pts',(-7.32841139752292,0.777016997712263,
3.23166070364585));
#24469=CARTESIAN_POINT('Ctrl Pts',(-8.32028099515215,1.29857075310548,3.27142905652491));
#24470=CARTESIAN_POINT('Ctrl Pts',(-9.10653920532774,1.07607201936986,3.30324373882815));
#24471=CARTESIAN_POINT('Ctrl Pts',(-9.70399944158484,0.518623433827907,
3.33505842113139));
#24472=CARTESIAN_POINT('Ctrl Pts',(-9.77137469231307,-0.599984716647835,
3.37482677401044));
#24473=CARTESIAN_POINT('Ctrl Pts',(-8.681056610743,-1.3940158845331,3.4225487974653));
#24474=CARTESIAN_POINT('Ctrl Pts',(-7.42643816511771,-0.905922591771324,
3.47027082092017));
#24475=CARTESIAN_POINT('Ctrl Pts',(-7.15628619215633,0.412910384032477,
3.51799284437503));
#24476=CARTESIAN_POINT('Ctrl Pts',(-8.12236807704563,1.35416741919452,3.56571486782989));
#24477=CARTESIAN_POINT('Ctrl Pts',(-9.21371438567086,1.09963480172637,3.60548322070895));
#24478=CARTESIAN_POINT('Ctrl Pts',(-9.66274853496778,0.416937216961904,
3.63729790301218));
#24479=CARTESIAN_POINT('Ctrl Pts',(-9.74985295977625,-0.39554076960521,
3.66911258531543));
#24480=CARTESIAN_POINT('Ctrl Pts',(-9.0689239756906,-1.2855741045648,3.70888093819448));
#24481=CARTESIAN_POINT('Ctrl Pts',(-7.7248494450175,-1.17269066668865,3.75660296164935));
#24482=CARTESIAN_POINT('Ctrl Pts',(-7.09538923568223,0.0173019179194368,
3.8043249851042));
#24483=CARTESIAN_POINT('Ctrl Pts',(-7.7539705342453,1.19142847827895,3.85204700855907));
#24484=CARTESIAN_POINT('Ctrl Pts',(-9.10041781121801,1.27117021693212,3.89976903201393));
#24485=CARTESIAN_POINT('Ctrl Pts',(-9.75921675296556,0.364634187278776,
3.93953738489298));
#24486=CARTESIAN_POINT('Ctrl Pts',(-9.65212567573532,-0.4454517098057,3.97135206719623));
#24487=CARTESIAN_POINT('Ctrl Pts',(-9.18641146043698,-1.1168814746706,4.00316674949946));
#24488=CARTESIAN_POINT('Ctrl Pts',(-8.08912659919642,-1.34445465410894,
4.04293510237852));
#24489=CARTESIAN_POINT('Ctrl Pts',(-7.14652302700508,-0.379686536765321,
4.09065712583338));
#24490=CARTESIAN_POINT('Ctrl Pts',(-7.449078725721,0.932091857527417,4.13837914928824));
#24491=CARTESIAN_POINT('Ctrl Pts',(-8.71533928644708,1.38913310173676,4.1861011727431));
#24492=CARTESIAN_POINT('Ctrl Pts',(-9.7857678498451,0.568485975858496,4.23382319619797));
#24493=CARTESIAN_POINT('Ctrl Pts',(-9.69085931574868,-0.548123171902275,
4.27359154907701));
#24494=CARTESIAN_POINT('Ctrl Pts',(-9.07984920094099,-1.09068588632358,
4.30540623138026));
#24495=CARTESIAN_POINT('Ctrl Pts',(-8.28834893264812,-1.29374987813349,
4.33722091368349));
#24496=CARTESIAN_POINT('Ctrl Pts',(-7.30962727695085,-0.747922488406148,
4.37698926656256));
#24497=CARTESIAN_POINT('Ctrl Pts',(-7.22800764477856,0.598412258302363,
4.42471129001741));
#24498=CARTESIAN_POINT('Ctrl Pts',(-8.31508535771834,1.39249320668754,4.47243331347228));
#24499=CARTESIAN_POINT('Ctrl Pts',(-9.57173156659136,0.909644563442217,
4.52015533692714));
#24500=CARTESIAN_POINT('Ctrl Pts',(-9.84431460056008,-0.411331403085193,
4.567877360382));
#24501=CARTESIAN_POINT('Ctrl Pts',(-9.04196587069652,-1.19367412491089,
4.60764571326105));
#24502=CARTESIAN_POINT('Ctrl Pts',(-8.22490009151298,-1.20421793659114,
4.63946039556429));
#24503=CARTESIAN_POINT('Ctrl Pts',(-7.49346489460161,-0.839923807902976,
4.67127507786754));
#24504=CARTESIAN_POINT('Ctrl Pts',(-7.11042675183102,0.213216923381422,
4.71104343074659));
#24505=CARTESIAN_POINT('Ctrl Pts',(-7.92958008831927,1.28478905155145,4.75876545420144));
#24506=CARTESIAN_POINT('Ctrl Pts',(-9.27123664979505,1.17406336524653,4.80648747765632));
#24507=CARTESIAN_POINT('Ctrl Pts',(-9.90566182547761,-0.0132896585079293,
4.85420950111116));
#24508=CARTESIAN_POINT('Ctrl Pts',(-9.24751691120311,-1.19062745470968,
4.90193152456605));
#24509=CARTESIAN_POINT('Ctrl Pts',(-8.1288676629186,-1.25731686931103,4.94169987744508));
#24510=CARTESIAN_POINT('Ctrl Pts',(-7.50406036051186,-0.730701740078402,
4.97351455974834));
#24511=CARTESIAN_POINT('Ctrl Pts',(-7.18926003595645,0.0233595406788859,
5.00532924205156));
#24512=CARTESIAN_POINT('Ctrl Pts',(-7.58863395692623,1.07041450101124,5.04509759493063));
#24513=CARTESIAN_POINT('Ctrl Pts',(-8.90922845059994,1.3448397145563,5.09281961838548));
#24514=CARTESIAN_POINT('Ctrl Pts',(-9.85141519694107,0.383285430296794,
5.14054164184035));
#24515=CARTESIAN_POINT('Ctrl Pts',(-9.55434127955645,-0.929745260193144,
5.18826366529521));
#24516=CARTESIAN_POINT('Ctrl Pts',(-8.28630969195433,-1.3895005292156,5.23598568875008));
#24517=CARTESIAN_POINT('Ctrl Pts',(-7.39669400474826,-0.708025989864192,
5.27575404162911));
#24518=CARTESIAN_POINT('Ctrl Pts',(-7.26873458964617,0.0990267020737063,
5.30756872393238));
#24519=CARTESIAN_POINT('Ctrl Pts',(-7.52403220505333,0.875255268312366,
5.3393834062356));
#24520=CARTESIAN_POINT('Ctrl Pts',(-8.51112605556492,1.40579211810661,5.37915175911467));
#24521=CARTESIAN_POINT('Ctrl Pts',(-9.68938066093212,0.749289947903339,
5.42687378256952));
#24522=CARTESIAN_POINT('Ctrl Pts',(-9.77278781043502,-0.594341606493356,
5.47459580602438));
#24523=CARTESIAN_POINT('Ctrl Pts',(-8.68903636181648,-1.39295622204702,
5.52231782947925));
#24524=CARTESIAN_POINT('Ctrl Pts',(-7.42927507874336,-0.911001323513343,
5.5700398529341));
#24525=CARTESIAN_POINT('Ctrl Pts',(-7.20237469211957,0.186422857584081,
5.60980820581317));
#24526=CARTESIAN_POINT('Ctrl Pts',(-7.63364252939566,0.880480284609163,
5.6416228881164));
#24527=CARTESIAN_POINT('Ctrl Pts',(-8.33458219270634,1.30046986528399,5.67343757041965));
#24528=CARTESIAN_POINT('Ctrl Pts',(-9.42819427600473,1.05585541360318,5.7132059232987));
#24529=CARTESIAN_POINT('Ctrl Pts',(-9.88971769783222,-0.211533692257875,
5.76092794675356));
#24530=CARTESIAN_POINT('Ctrl Pts',(-9.07368481902778,-1.28223105718826,
5.80864997020842));
#24531=CARTESIAN_POINT('Ctrl Pts',(-7.73157747309663,-1.17711027638694,
5.85637199366328));
#24532=CARTESIAN_POINT('Ctrl Pts',(-7.09421175387495,0.0116049773688213,
5.90409401711815));
#24533=CARTESIAN_POINT('Ctrl Pts',(-7.64063909944886,0.98999180000924,5.94386236999719));
#24534=CARTESIAN_POINT('Ctrl Pts',(-8.42089398251533,1.23270557573781,5.97567705230044));
#24535=CARTESIAN_POINT('Ctrl Pts',(-9.22577226286207,1.09171403945432,6.00749173460368));
#24536=CARTESIAN_POINT('Ctrl Pts',(-9.89277395110486,0.191196206988666,
6.04726008748273));
#24537=CARTESIAN_POINT('Ctrl Pts',(-9.41257658626577,-1.06923606225557,
6.0949821109376));
#24538=CARTESIAN_POINT('Ctrl Pts',(-8.09491428823142,-1.34504138290316,
6.14270413439245));
#24539=CARTESIAN_POINT('Ctrl Pts',(-7.14871946308653,-0.38743088827196,
6.19042615784733));
#24540=CARTESIAN_POINT('Ctrl Pts',(-7.44446086304004,0.928553928853288,
6.23814818130217));
#24541=CARTESIAN_POINT('Ctrl Pts',(-8.49783623871218,1.31094631454484,6.27791653418124));
#24542=CARTESIAN_POINT('Ctrl Pts',(-9.24670909380938,0.983995085190856,
6.30973121648447));
#24543=CARTESIAN_POINT('Ctrl Pts',(-9.76315317478435,0.350754869551153,
6.34154589878773));
#24544=CARTESIAN_POINT('Ctrl Pts',(-9.67838557456485,-0.766669880783481,
6.38131425166676));
#24545=CARTESIAN_POINT('Ctrl Pts',(-8.49056044938906,-1.40569295278612,
6.42903627512164));
#24546=CARTESIAN_POINT('Ctrl Pts',(-7.3136203517155,-0.752152966980432,
6.47675829857649));
#24547=CARTESIAN_POINT('Ctrl Pts',(-7.22460174085939,0.591118484916007,
6.52448032203136));
#24548=CARTESIAN_POINT('Ctrl Pts',(-8.30927829155303,1.39283900662287,6.57220234548622));
#24549=CARTESIAN_POINT('Ctrl Pts',(-9.35608819723364,0.992823206839408,
6.61197069836527));
#24550=CARTESIAN_POINT('Ctrl Pts',(-9.70850848082631,0.25559352540361,6.6437853806685));
#24551=CARTESIAN_POINT('Ctrl Pts',(-9.68475530270078,-0.561194969866995,
6.67560006297176));
#24552=CARTESIAN_POINT('Ctrl Pts',(-8.88954205617756,-1.35078949318983,
6.7153684158508));
#24553=CARTESIAN_POINT('Ctrl Pts',(-7.57314603074635,-1.05688386415305,
6.76309043930567));
#24554=CARTESIAN_POINT('Ctrl Pts',(-7.11067861489593,0.207405025237098,
6.81081246276052));
#24555=CARTESIAN_POINT('Ctrl Pts',(-7.92223219994117,1.28150152237267,6.8585344862154));
#24556=CARTESIAN_POINT('Ctrl Pts',(-9.26707128633578,1.17812431861932,6.90625650967024));
#24557=CARTESIAN_POINT('Ctrl Pts',(-9.79700284495402,0.190705379218312,
6.94602486254932));
#24558=CARTESIAN_POINT('Ctrl Pts',(-9.58116800924214,-0.597408180600789,
6.97783954485253));
#24559=CARTESIAN_POINT('Ctrl Pts',(-9.02879708860554,-1.19956598841578,
7.0096542271558));
#24560=CARTESIAN_POINT('Ctrl Pts',(-7.91079937238375,-1.27640819836747,
7.04942258003484));
#24561=CARTESIAN_POINT('Ctrl Pts',(-7.10756676680328,-0.192850910595855,
7.09714460348971));
#24562=CARTESIAN_POINT('Ctrl Pts',(-7.58502182671985,1.06585444504493,7.14486662694456));
#24563=CARTESIAN_POINT('Ctrl Pts',(-8.90152062454935,1.34716107822704,7.19258865039943));
#24564=CARTESIAN_POINT('Ctrl Pts',(-9.85092212321177,0.389081849306921,
7.24031067385429));
#24565=CARTESIAN_POINT('Ctrl Pts',(-9.60563721925922,-0.704380054282014,
7.28007902673334));
#24566=CARTESIAN_POINT('Ctrl Pts',(-8.92676531327588,-1.15917736599793,
7.31189370903659));
#24567=CARTESIAN_POINT('Ctrl Pts',(-8.11505380559897,-1.25315655402578,
7.34370839133982));
#24568=CARTESIAN_POINT('Ctrl Pts',(-7.21928808162424,-0.579786383570173,
7.38347674421888));
#24569=CARTESIAN_POINT('Ctrl Pts',(-7.32078945678287,0.765195581138472,
7.43119876767373));
#24570=CARTESIAN_POINT('Ctrl Pts',(-8.50541082157443,1.4047069013182,7.47892079112861));
#24571=CARTESIAN_POINT('Ctrl Pts',(-9.68507041122039,0.756088555050457,
7.52664281458347));
#24572=CARTESIAN_POINT('Ctrl Pts',(-9.77620739660413,-0.58963543761884,
7.57436483803832));
#24573=CARTESIAN_POINT('Ctrl Pts',(-8.875280791801,-1.25608488916428,7.61413319091738));
#24574=CARTESIAN_POINT('Ctrl Pts',(-8.06431736127027,-1.15585528366093,
7.64594787322062));
#24575=CARTESIAN_POINT('Ctrl Pts',(-7.38896923590437,-0.695841621861376,
7.67776255552386));
#24576=CARTESIAN_POINT('Ctrl Pts',(-7.15211534576237,0.399477442809727,
7.71753090840292));
#24577=CARTESIAN_POINT('Ctrl Pts',(-8.10886945534902,1.350214308793,7.76525293185777));
#24578=CARTESIAN_POINT('Ctrl Pts',(-9.42316207684519,1.05877407197001,7.81297495531264));
#24579=CARTESIAN_POINT('Ctrl Pts',(-9.8909062425691,-0.203572117468501,
7.8606969787675));
#24580=CARTESIAN_POINT('Ctrl Pts',(-9.07935003954765,-1.28090936452164,
7.90841900222236));
#24581=CARTESIAN_POINT('Ctrl Pts',(-7.9619774706096,-1.19545668233942,7.94818735510142));
#24582=CARTESIAN_POINT('Ctrl Pts',(-7.41426180224206,-0.589061426666821,
7.98000203740465));
#24583=CARTESIAN_POINT('Ctrl Pts',(-7.204504785262,0.200691479820453,8.01181671970791));
#24584=CARTESIAN_POINT('Ctrl Pts',(-7.74202742743127,1.18399866878161,8.05158507258693));
#24585=CARTESIAN_POINT('Ctrl Pts',(-9.08762299690323,1.27701252779242,8.09930709604183));
#24586=CARTESIAN_POINT('Ctrl Pts',(-9.89087795044728,0.196695913939951,
8.14702911949667));
#24587=CARTESIAN_POINT('Ctrl Pts',(-9.41868451778527,-1.06399273466032,
8.19475114295154));
#24588=CARTESIAN_POINT('Ctrl Pts',(-8.10006338572175,-1.34774848284193,
8.24247316640639));
#24589=CARTESIAN_POINT('Ctrl Pts',(-7.31095655944527,-0.55205128199777,
8.28224151928546));
#24590=CARTESIAN_POINT('Ctrl Pts',(-7.29349640414644,0.264895963823187,
8.31405620158869));
#24591=CARTESIAN_POINT('Ctrl Pts',(-7.65158564831681,0.999388817898019,
8.34587088389193));
#24592=CARTESIAN_POINT('Ctrl Pts',(-8.70144610447083,1.39132840675256,8.385639236771));
#24593=CARTESIAN_POINT('Ctrl Pts',(-9.77991422991853,0.581275620235635,
8.43336126022583));
#24594=CARTESIAN_POINT('Ctrl Pts',(-9.68055006013832,-0.761270195862498,
8.48108328368072));
#24595=CARTESIAN_POINT('Ctrl Pts',(-8.49861019163866,-1.4057239597663,8.52880530713557));
#24596=CARTESIAN_POINT('Ctrl Pts',(-7.31574317534535,-0.75756916628252,
8.57652733059043));
#24597=CARTESIAN_POINT('Ctrl Pts',(-7.23958642901857,0.360475452100957,
8.61629568346948));
#24598=CARTESIAN_POINT('Ctrl Pts',(-7.76089349654227,0.989718331144719,
8.64811036577273));
#24599=CARTESIAN_POINT('Ctrl Pts',(-8.51226287342945,1.31089074427157,8.67992504807597));
#24600=CARTESIAN_POINT('Ctrl Pts',(-9.56266114340054,0.920394786355142,
8.71969340095502));
#24601=CARTESIAN_POINT('Ctrl Pts',(-9.84825577586161,-0.397829291888031,
8.76741542440989));
#24602=CARTESIAN_POINT('Ctrl Pts',(-8.89471185563952,-1.34812214083839,
8.81513744786473));
#24603=CARTESIAN_POINT('Ctrl Pts',(-7.57921338783839,-1.06217409001174,
8.86285947131962));
#24604=CARTESIAN_POINT('Ctrl Pts',(-7.10874030224357,0.20192008776204,8.91058149477447));
#24605=CARTESIAN_POINT('Ctrl Pts',(-7.78265954393772,1.09727279724685,8.95034984765352));
#24606=CARTESIAN_POINT('Ctrl Pts',(-8.58860010090821,1.23205958483201,8.98216452995677));
#24607=CARTESIAN_POINT('Ctrl Pts',(-9.36696202918395,0.983342138543273,
9.01397921226));
#24608=CARTESIAN_POINT('Ctrl Pts',(-9.90583593214038,0.000774820025180653,
9.05374756513906));
#24609=CARTESIAN_POINT('Ctrl Pts',(-9.25933158494685,-1.18299506623249,
9.10146958859392));
#24610=CARTESIAN_POINT('Ctrl Pts',(-7.91645424282956,-1.27777349514281,
9.14919161204877));
#24611=CARTESIAN_POINT('Ctrl Pts',(-7.10869394244917,-0.200821405359748,
9.19691363550366));
#24612=CARTESIAN_POINT('Ctrl Pts',(-7.57996729233084,1.06297463999009,9.24463565895849));
#24613=CARTESIAN_POINT('Ctrl Pts',(-8.67543136727172,1.29915694081153,9.28440401183757));
#24614=CARTESIAN_POINT('Ctrl Pts',(-9.37311474448176,0.873779973120195,
9.3162186941408));
#24615=CARTESIAN_POINT('Ctrl Pts',(-9.79902295327563,0.17642077072913,9.34803337644404));
#24616=CARTESIAN_POINT('Ctrl Pts',(-9.56367504023093,-0.919222865921435,
9.3878017293231));
#24617=CARTESIAN_POINT('Ctrl Pts',(-8.30023828915245,-1.39145860215371,
9.43552375277796));
#24618=CARTESIAN_POINT('Ctrl Pts',(-7.22267131126601,-0.584518756361346,
9.48324577623282));
#24619=CARTESIAN_POINT('Ctrl Pts',(-7.31642696034088,0.758430380734061,
9.53096779968769));
#24620=CARTESIAN_POINT('Ctrl Pts',(-8.49970411739585,1.4058361145228,9.57868982314254));
#24621=CARTESIAN_POINT('Ctrl Pts',(-9.48268156411455,0.867710703536009,
9.6184581760216));
#24622=CARTESIAN_POINT('Ctrl Pts',(-9.73199174854549,0.0895384273551449,
9.65027285832483));
#24623=CARTESIAN_POINT('Ctrl Pts',(-9.59781881456104,-0.716504551190982,
9.68208754062809));
#24624=CARTESIAN_POINT('Ctrl Pts',(-8.70297963016015,-1.3911055093641,9.72185589350711));
#24625=CARTESIAN_POINT('Ctrl Pts',(-7.43852750076266,-0.921595310313144,
9.76957791696201));
#24626=CARTESIAN_POINT('Ctrl Pts',(-7.15157763261807,0.393684994310346,
9.81729994041685));
#24627=CARTESIAN_POINT('Ctrl Pts',(-8.10114397486295,1.34795239301698,9.86502196387172));
#24628=CARTESIAN_POINT('Ctrl Pts',(-9.4195851832654,1.06336181949601,9.91274398732657));
#24629=CARTESIAN_POINT('Ctrl Pts',(-9.81088102451861,0.0132612608230292,
9.95251234020565));
#24630=CARTESIAN_POINT('Ctrl Pts',(-9.49028095694926,-0.738352507113669,
9.98432702250886));
#24631=CARTESIAN_POINT('Ctrl Pts',(-8.86143529445072,-1.26013866276967,
10.0161417048121));
#24632=CARTESIAN_POINT('Ctrl Pts',(-7.74333299839028,-1.184833455435,10.0559100576912));
#24633=CARTESIAN_POINT('Ctrl Pts',(-7.09427750642714,-0.00246042508328673,
10.103632081146));
#24634=CARTESIAN_POINT('Ctrl Pts',(-7.7378309030877,1.17996992474936,10.1513541046009));
#24635=CARTESIAN_POINT('Ctrl Pts',(-9.08030065280452,1.28035656556405,10.1990761280558));
#24636=CARTESIAN_POINT('Ctrl Pts',(-9.89117457933197,0.202505699336026,
10.2467981515106));
#24637=CARTESIAN_POINT('Ctrl Pts',(-9.50003469113584,-0.847652958472063,
10.2865665043897));
#24638=CARTESIAN_POINT('Ctrl Pts',(-8.76581477537552,-1.20630149782277,
10.3183811866929));
#24639=CARTESIAN_POINT('Ctrl Pts',(-7.94885446861643,-1.18946354493003,
10.3501958689961));
#24640=CARTESIAN_POINT('Ctrl Pts',(-7.15255650481893,-0.400962960555315,
10.3899642218752));
#24641=CARTESIAN_POINT('Ctrl Pts',(-7.43530789219255,0.917873901034805,
10.43768624533));
#24642=CARTESIAN_POINT('Ctrl Pts',(-8.69563654667604,1.39102735314794,10.4854082687849));
#24643=CARTESIAN_POINT('Ctrl Pts',(-9.77656461632702,0.588595415349269,
10.5331302922398));
#24644=CARTESIAN_POINT('Ctrl Pts',(-9.68457560687616,-0.757070604393695,
10.5808523156946));
#24645=CARTESIAN_POINT('Ctrl Pts',(-8.70167808713493,-1.2953419898433,10.6206206685737));
#24646=CARTESIAN_POINT('Ctrl Pts',(-7.91176565610344,-1.08618651948824,
10.6524353508769));
#24647=CARTESIAN_POINT('Ctrl Pts',(-7.30495342912999,-0.538932848259806,
10.6842500331802));
#24648=CARTESIAN_POINT('Ctrl Pts',(-7.21864976666804,0.578374314767913,
10.7240183860592));
#24649=CARTESIAN_POINT('Ctrl Pts',(-8.29536860980847,1.39075079607261,10.7717404095141));
#24650=CARTESIAN_POINT('Ctrl Pts',(-9.55807067299778,0.923968184811093,
10.8194624329689));
#24651=CARTESIAN_POINT('Ctrl Pts',(-9.85051180715808,-0.390102090938935,
10.8671844564238));
#24652=CARTESIAN_POINT('Ctrl Pts',(-8.90050389292981,-1.34758001624808,
10.9149064798787));
#24653=CARTESIAN_POINT('Ctrl Pts',(-7.80500475501606,-1.11156040363594,
10.9546748327577));
#24654=CARTESIAN_POINT('Ctrl Pts',(-7.34447687296949,-0.436562826354961,
10.986489515061));
#24655=CARTESIAN_POINT('Ctrl Pts',(-7.24362965654256,0.374324032840834,
11.0183041973642));
#24656=CARTESIAN_POINT('Ctrl Pts',(-7.90939275771686,1.27575795267197,11.0580725502433));
#24657=CARTESIAN_POINT('Ctrl Pts',(-9.25518577116924,1.18564591411257,11.1057945736981));
#24658=CARTESIAN_POINT('Ctrl Pts',(-9.90470237296531,0.00648066252564181,
11.153516597153));
#24659=CARTESIAN_POINT('Ctrl Pts',(-9.26609346085678,-1.17862741859367,
11.2012386206079));
#24660=CARTESIAN_POINT('Ctrl Pts',(-7.92118919095866,-1.28115311956846,
11.2489606440627));
#24661=CARTESIAN_POINT('Ctrl Pts',(-7.24713698930774,-0.385900502617859,
11.2887289969418));
#24662=CARTESIAN_POINT('Ctrl Pts',(-7.34049794034117,0.425882345377609,
11.320543679245));
#24663=CARTESIAN_POINT('Ctrl Pts',(-7.79477808273445,1.10510043384748,11.3523583615483));
#24664=CARTESIAN_POINT('Ctrl Pts',(-8.88805285710864,1.35121806105931,11.3921267144273));
#24665=CARTESIAN_POINT('Ctrl Pts',(-9.84685488433432,0.402546522992234,
11.4398487378822));
#24666=CARTESIAN_POINT('Ctrl Pts',(-9.5665509948533,-0.914166139702461,
11.487570761337));
#24667=CARTESIAN_POINT('Ctrl Pts',(-8.30820964007592,-1.3925797070432,11.5352927847919));
#24668=CARTESIAN_POINT('Ctrl Pts',(-7.22404091446613,-0.590172585339807,
11.5830148082467));
#24669=CARTESIAN_POINT('Ctrl Pts',(-7.30003162094818,0.527883330630275,
11.6227831611258));
#24670=CARTESIAN_POINT('Ctrl Pts',(-7.90176856145037,1.08071270205741,11.6545978434291));
#24671=CARTESIAN_POINT('Ctrl Pts',(-8.68971751015799,1.29714771241407,11.6864125257323));
#24672=CARTESIAN_POINT('Ctrl Pts',(-9.67753976575011,0.767968338227732,
11.7261808786114));
#24673=CARTESIAN_POINT('Ctrl Pts',(-9.78194118595766,-0.576791624743086,
11.7739029020662));
#24674=CARTESIAN_POINT('Ctrl Pts',(-8.70846308980102,-1.38916301987625,
11.8216249255211));
#24675=CARTESIAN_POINT('Ctrl Pts',(-7.44382234606286,-0.927658636542655,
11.8693469489759));
#24676=CARTESIAN_POINT('Ctrl Pts',(-7.14891421842479,0.38851316485853,11.9170689724308));
#24677=CARTESIAN_POINT('Ctrl Pts',(-7.93790286829016,1.18432754591167,11.9568373253098));
#24678=CARTESIAN_POINT('Ctrl Pts',(-8.75467303594958,1.20870279358393,11.9886520076131));
#24679=CARTESIAN_POINT('Ctrl Pts',(-9.49217091130871,0.856844095640773,
12.0204666899163));
#24680=CARTESIAN_POINT('Ctrl Pts',(-9.89298385872439,-0.189660849350548,
12.0602350427954));
#24681=CARTESIAN_POINT('Ctrl Pts',(-9.09208967290089,-1.27494768593557,
12.1079570662503));
#24682=CARTESIAN_POINT('Ctrl Pts',(-7.74875081289082,-1.18695215340337,
12.1556790897051));
#24683=CARTESIAN_POINT('Ctrl Pts',(-7.0943146441837,-0.0105101413829567,
12.20340111316));
#24684=CARTESIAN_POINT('Ctrl Pts',(-7.73243286823234,1.1778013273354,12.2511231366148));
#24685=CARTESIAN_POINT('Ctrl Pts',(-8.84979273440854,1.26341994777532,12.2908914894939));
#24686=CARTESIAN_POINT('Ctrl Pts',(-9.48342609672741,0.747458300330454,
12.3227061717971));
#24687=CARTESIAN_POINT('Ctrl Pts',(-9.810947582283,-0.00116532738706759,
12.3545208541004));
#24688=CARTESIAN_POINT('Ctrl Pts',(-9.42935757148806,-1.05483163242336,
12.3942892069794));
#24689=CARTESIAN_POINT('Ctrl Pts',(-8.11359837641989,-1.35157521726427,
12.4420112304343));
#24690=CARTESIAN_POINT('Ctrl Pts',(-7.15526752559027,-0.406109994790781,
12.4897332538891));
#24691=CARTESIAN_POINT('Ctrl Pts',(-7.43006921799579,0.911761977902243,
12.537455277344));
#24692=CARTESIAN_POINT('Ctrl Pts',(-8.69013539730176,1.39291916460934,12.5851773007989));
#24693=CARTESIAN_POINT('Ctrl Pts',(-9.59116096550439,0.726603515571681,
12.6249456536779));
#24694=CARTESIAN_POINT('Ctrl Pts',(-9.73276546636217,-0.0781671504036021,
12.6567603359812));
#24695=CARTESIAN_POINT('Ctrl Pts',(-9.49064601300238,-0.858606661052731,
12.6885750182844));
#24696=CARTESIAN_POINT('Ctrl Pts',(-8.51267564008941,-1.40577899991123,
12.7283433711635));
#24697=CARTESIAN_POINT('Ctrl Pts',(-7.32347530531005,-0.76931880609604,
12.7760653946183));
#24698=CARTESIAN_POINT('Ctrl Pts',(-7.21733238908827,0.572708089273282,
12.8237874180732));
#24699=CARTESIAN_POINT('Ctrl Pts',(-8.28740794253882,1.3895561880445,12.871509441528));
#24700=CARTESIAN_POINT('Ctrl Pts',(-9.55514818289102,0.928998159624082,
12.9192314649829));
#24701=CARTESIAN_POINT('Ctrl Pts',(-9.80059547240428,-0.164427305040956,
12.958999817862));
#24702=CARTESIAN_POINT('Ctrl Pts',(-9.38113985803971,-0.865686634430231,
12.9908145001652));
#24703=CARTESIAN_POINT('Ctrl Pts',(-8.68741109134266,-1.29748294953088,
13.0226291824684));
#24704=CARTESIAN_POINT('Ctrl Pts',(-7.58981441832717,-1.07141844083344,
13.0623975353475));
#24705=CARTESIAN_POINT('Ctrl Pts',(-7.1069002094667,0.187975413936122,13.1101195588023));
#24706=CARTESIAN_POINT('Ctrl Pts',(-7.90468919460728,1.27233478321696,13.1578415822572));
#24707=CARTESIAN_POINT('Ctrl Pts',(-9.24838388325329,1.18995098466913,13.2055636057121));
#24708=CARTESIAN_POINT('Ctrl Pts',(-9.90578323664456,0.012196721373359,
13.253285629167));
#24709=CARTESIAN_POINT('Ctrl Pts',(-9.37599832386594,-0.975300906421013,
13.293053982046));
#24710=CARTESIAN_POINT('Ctrl Pts',(-8.59996442064334,-1.23118963326647,
13.3248686643492));
#24711=CARTESIAN_POINT('Ctrl Pts',(-7.7928145072655,-1.10384491680104,13.3566833466525));
#24712=CARTESIAN_POINT('Ctrl Pts',(-7.11066262301496,-0.214748507225108,
13.3964516995315));
#24713=CARTESIAN_POINT('Ctrl Pts',(-7.56945200982095,1.05363286803423,13.4441737229864));
#24714=CARTESIAN_POINT('Ctrl Pts',(-8.88225606424844,1.35170672001969,13.4918957464413));
#24715=CARTESIAN_POINT('Ctrl Pts',(-9.84452765095915,0.410252578827465,
13.5396177698961));
#24716=CARTESIAN_POINT('Ctrl Pts',(-9.57110829845308,-0.910550537547473,
13.587339793351));
#24717=CARTESIAN_POINT('Ctrl Pts',(-8.52435781001808,-1.31072179297237,
13.62710814623));
#24718=CARTESIAN_POINT('Ctrl Pts',(-7.77005699205511,-0.996495862314412,
13.6589228285333));
#24719=CARTESIAN_POINT('Ctrl Pts',(-7.24296615442084,-0.372089817853327,
13.6907375108365));
#24720=CARTESIAN_POINT('Ctrl Pts',(-7.30880357228206,0.746609897493391,
13.7305058637156));
#24721=CARTESIAN_POINT('Ctrl Pts',(-8.48563977554364,1.40565129622601,13.7782278871704));
#24722=CARTESIAN_POINT('Ctrl Pts',(-9.67347564116168,0.772130607605528,
13.8259499106253));
#24723=CARTESIAN_POINT('Ctrl Pts',(-9.78522311793835,-0.569441234672302,
13.8736719340801));
#24724=CARTESIAN_POINT('Ctrl Pts',(-8.71427517808187,-1.38941045645305,
13.921393957535));
#24725=CARTESIAN_POINT('Ctrl Pts',(-7.66084302554854,-1.00717451005825,
13.9611623104141));
#24726=CARTESIAN_POINT('Ctrl Pts',(-7.29599193222992,-0.276016976292999,
13.9929769927173));
#24727=CARTESIAN_POINT('Ctrl Pts',(-7.30591345323344,0.541056596219603,
14.0247916750205));
#24728=CARTESIAN_POINT('Ctrl Pts',(-8.08764486923065,1.34400093548008,14.0645600278996));
#24729=CARTESIAN_POINT('Ctrl Pts',(-9.40882805532143,1.07242405255057,14.1122820513545));
#24730=CARTESIAN_POINT('Ctrl Pts',(-9.8926336361544,-0.183854048235054,
14.1600040748093));
#24731=CARTESIAN_POINT('Ctrl Pts',(-9.09938085019241,-1.27153622797425,
14.2077260982642));
#24732=CARTESIAN_POINT('Ctrl Pts',(-7.75298433141432,-1.190942005024,14.2554481217191));
#24733=CARTESIAN_POINT('Ctrl Pts',(-7.20641169321538,-0.212636342217414,
14.2952164745981));
#24734=CARTESIAN_POINT('Ctrl Pts',(-7.40887280952849,0.579018352620409,
14.3270311569013));
#24735=CARTESIAN_POINT('Ctrl Pts',(-7.95097001357033,1.19044151283563,14.3588458392046));
#24736=CARTESIAN_POINT('Ctrl Pts',(-9.06750655394557,1.28620044303833,14.3986141920836));
#24737=CARTESIAN_POINT('Ctrl Pts',(-9.88896869373039,0.216397205310634,
14.4463362155385));
#24738=CARTESIAN_POINT('Ctrl Pts',(-9.43289198211277,-1.05021107655012,
14.4940582389934));
#24739=CARTESIAN_POINT('Ctrl Pts',(-8.1213443985153,-1.35376575451354,14.5417802624482));
#24740=CARTESIAN_POINT('Ctrl Pts',(-7.15585866218863,-0.411897235285569,
14.5895022859031));
#24741=CARTESIAN_POINT('Ctrl Pts',(-7.38259606962084,0.685560630316758,
14.6292706387821));
#24742=CARTESIAN_POINT('Ctrl Pts',(-8.0536709459124,1.15178607994221,14.6610853210854));
#24743=CARTESIAN_POINT('Ctrl Pts',(-8.86367504615505,1.25949409775321,14.6929000033886));
#24744=CARTESIAN_POINT('Ctrl Pts',(-9.77071256243562,0.601385776394011,
14.7326683562677));
#24745=CARTESIAN_POINT('Ctrl Pts',(-9.69199631825355,-0.745121842437787,
14.7803903797225));
#24746=CARTESIAN_POINT('Ctrl Pts',(-8.51837168210054,-1.40459717952675,
14.8281124031774));
#24747=CARTESIAN_POINT('Ctrl Pts',(-7.32790003807112,-0.776043466300811,
14.8758344266323));
#24748=CARTESIAN_POINT('Ctrl Pts',(-7.21399296821595,0.567944701423163,
14.9235564500871));
#24749=CARTESIAN_POINT('Ctrl Pts',(-8.10350744198034,1.2495513480657,14.9633248029662));
#24750=CARTESIAN_POINT('Ctrl Pts',(-8.91605153117148,1.1630657428884,14.9951394852694));
#24751=CARTESIAN_POINT('Ctrl Pts',(-9.5990909110902,0.714551673218286,15.0269541675726));
#24752=CARTESIAN_POINT('Ctrl Pts',(-9.85445463106407,-0.376600459844835,
15.0667225204517));
#24753=CARTESIAN_POINT('Ctrl Pts',(-8.91393366145371,-1.34339894468464,
15.1144445439066));
#24754=CARTESIAN_POINT('Ctrl Pts',(-7.5948952950249,-1.07425147771361,15.1621665673614));
#24755=CARTESIAN_POINT('Ctrl Pts',(-7.10584665164846,0.179994843176864,
15.2098885908163));
#24756=CARTESIAN_POINT('Ctrl Pts',(-7.89904710899984,1.27091739730048,15.2576106142712));
#24757=CARTESIAN_POINT('Ctrl Pts',(-9.0177063954227,1.20439403072938,15.2973789671502));
#24758=CARTESIAN_POINT('Ctrl Pts',(-9.57560963494508,0.607358648640619,
15.3291936494535));
#24759=CARTESIAN_POINT('Ctrl Pts',(-9.79870755565295,-0.178730113269691,
15.3610083317567));
#24760=CARTESIAN_POINT('Ctrl Pts',(-9.27790842578802,-1.17099611903574,
15.4007766846358));
#24761=CARTESIAN_POINT('Ctrl Pts',(-7.93408216140049,-1.28677857688729,
15.4484987080906));
#24762=CARTESIAN_POINT('Ctrl Pts',(-7.11264948841516,-0.220214228828185,
15.4962207315455));
#24763=CARTESIAN_POINT('Ctrl Pts',(-7.56343745957694,1.0482848064335,15.5439427550003));
#24764=CARTESIAN_POINT('Ctrl Pts',(-8.87705446008071,1.35433038087565,15.5916647784552));
#24765=CARTESIAN_POINT('Ctrl Pts',(-9.67953973170108,0.572095495672879,
15.6314331313343));
#24766=CARTESIAN_POINT('Ctrl Pts',(-9.71079808013641,-0.244422239744446,
15.6632478136375));
#24767=CARTESIAN_POINT('Ctrl Pts',(-9.36525453459661,-0.98490531805759,
15.6950624959407));
#24768=CARTESIAN_POINT('Ctrl Pts',(-8.32204860714223,-1.39448976690685,
15.7348308488198));
#24769=CARTESIAN_POINT('Ctrl Pts',(-7.23026016329708,-0.602944691238868,
15.7825528722746));
#24770=CARTESIAN_POINT('Ctrl Pts',(-7.3064571413049,0.741326568114441,15.8302748957295));
#24771=CARTESIAN_POINT('Ctrl Pts',(-8.47810477276462,1.40525997677245,15.8779969191844));
#24772=CARTESIAN_POINT('Ctrl Pts',(-9.67027309713215,0.778060702080256,
15.9257189426392));
#24773=CARTESIAN_POINT('Ctrl Pts',(-9.78737291614922,-0.563549955867611,
15.9734409660941));
#24774=CARTESIAN_POINT('Ctrl Pts',(-8.72189178072646,-1.387803675215,16.021162989549));
#24775=CARTESIAN_POINT('Ctrl Pts',(-7.45293723261821,-0.93689337562883,
16.0688850130038));
#24776=CARTESIAN_POINT('Ctrl Pts',(-7.14500260506151,0.373849720226483,
16.1166070364587));
#24777=CARTESIAN_POINT('Ctrl Pts',(-8.08314946719955,1.34257366335405,16.1643290599135));
#24778=CARTESIAN_POINT('Ctrl Pts',(-9.1815395506535,1.11991416460064,16.2040974127926));
#24779=CARTESIAN_POINT('Ctrl Pts',(-9.65014384072878,0.450492361508324,
16.2359120950958));
#24780=CARTESIAN_POINT('Ctrl Pts',(-9.76081674092163,-0.359093832643231,
16.2677267773991));
#24781=CARTESIAN_POINT('Ctrl Pts',(-9.1059854131481,-1.26852769992666,16.3074951302781));
#24782=CARTESIAN_POINT('Ctrl Pts',(-7.75921097797935,-1.19468910281155,
16.355217153733));
#24783=CARTESIAN_POINT('Ctrl Pts',(-7.09547696382248,-0.0234689032524444,
16.4029391771879));
#24784=CARTESIAN_POINT('Ctrl Pts',(-7.71971018800974,1.16927751850682,16.4506612006427));
#24785=CARTESIAN_POINT('Ctrl Pts',(-9.06327472143189,1.28805862362881,16.4983832240976));
#24786=CARTESIAN_POINT('Ctrl Pts',(-9.74810490751436,0.401023575788387,
16.5381515769766));
#24787=CARTESIAN_POINT('Ctrl Pts',(-9.66456742422846,-0.411829247736352,
16.5699662592799));
#24788=CARTESIAN_POINT('Ctrl Pts',(-9.21853458788756,-1.09649119427719,
16.6017809415831));
#24789=CARTESIAN_POINT('Ctrl Pts',(-8.12831596898121,-1.35581207733523,
16.6415492944622));
#24790=CARTESIAN_POINT('Ctrl Pts',(-7.15811168802375,-0.418804799962375,
16.6892713179171));
#24791=CARTESIAN_POINT('Ctrl Pts',(-7.42247182598189,0.901201308551626,
16.7369933413719));
#24792=CARTESIAN_POINT('Ctrl Pts',(-8.67493565199357,1.39479723197529,16.7847153648268));
#24793=CARTESIAN_POINT('Ctrl Pts',(-9.7687287250781,0.605559803923564,16.8324373882816));
#24794=CARTESIAN_POINT('Ctrl Pts',(-9.70626441131446,-0.513333317189079,
16.8722057411607));
#24795=CARTESIAN_POINT('Ctrl Pts',(-9.11125692448223,-1.07339916673304,
16.9040204234639));
#24796=CARTESIAN_POINT('Ctrl Pts',(-8.32598297924596,-1.2993471424164,16.9358351057672));
#24797=CARTESIAN_POINT('Ctrl Pts',(-7.33183350595512,-0.782152358472143,
16.9756034586462));
#24798=CARTESIAN_POINT('Ctrl Pts',(-7.21117732228494,0.561246726270426,
17.0233254821011));
#24799=CARTESIAN_POINT('Ctrl Pts',(-8.27475278233387,1.38654045969504,17.0710475055559));
#24800=CARTESIAN_POINT('Ctrl Pts',(-9.5448820960995,0.940363327686985,17.1187695290108));
#24801=CARTESIAN_POINT('Ctrl Pts',(-9.85568533561032,-0.37214585741601,
17.1664915524657));
#24802=CARTESIAN_POINT('Ctrl Pts',(-9.07637829172762,-1.17744341108019,
17.2062599053447));
#24803=CARTESIAN_POINT('Ctrl Pts',(-8.25996262410618,-1.21169420921509,
17.2380745876479));
#24804=CARTESIAN_POINT('Ctrl Pts',(-7.51826359447111,-0.86877992122654,
17.2698892699512));
#24805=CARTESIAN_POINT('Ctrl Pts',(-7.10482440400817,0.172801402766392,
17.3096576228303));
#24806=CARTESIAN_POINT('Ctrl Pts',(-7.89253547638418,1.26769421990383,17.3573796462851));
#24807=CARTESIAN_POINT('Ctrl Pts',(-9.23684024893197,1.19595033473499,17.40510166974));
#24808=CARTESIAN_POINT('Ctrl Pts',(-9.90545546432878,0.0275085517188402,
17.4528236931948));
#24809=CARTESIAN_POINT('Ctrl Pts',(-9.28175434417965,-1.16843288801686,
17.5005457166497));
#24810=CARTESIAN_POINT('Ctrl Pts',(-8.16551158461359,-1.26755766001141,
17.5403140695287));
#24811=CARTESIAN_POINT('Ctrl Pts',(-7.52568494958409,-0.759296372301703,
17.572128751832));
#24812=CARTESIAN_POINT('Ctrl Pts',(-7.18913418819074,-0.0146882575976357,
17.6039434341352));
#24813=CARTESIAN_POINT('Ctrl Pts',(-7.55795413929691,1.04351562747055,17.6437117870143));
#24814=CARTESIAN_POINT('Ctrl Pts',(-8.87002855169553,1.35614920033101,17.6914338104691));
#24815=CARTESIAN_POINT('Ctrl Pts',(-9.8397229875011,0.42234236392081,17.739155833924));
#24816=CARTESIAN_POINT('Ctrl Pts',(-9.58087862748931,-0.898756460485886,
17.7868778573788));
#24817=CARTESIAN_POINT('Ctrl Pts',(-8.3267233016254,-1.39511664538973,17.8345998808337));
#24818=CARTESIAN_POINT('Ctrl Pts',(-7.41770575864982,-0.739745967627945,
17.8743682337128));
#24819=CARTESIAN_POINT('Ctrl Pts',(-7.26637939162968,0.063253403556096,
17.906182916016));
#24820=CARTESIAN_POINT('Ctrl Pts',(-7.49904315960666,0.846563834067683,
17.9379975983193));
#24821=CARTESIAN_POINT('Ctrl Pts',(-8.47032497547387,1.40552291385181,17.9777659511983));
#24822=CARTESIAN_POINT('Ctrl Pts',(-9.66713516544579,0.783490451893412,
18.0254879746532));
#24823=CARTESIAN_POINT('Ctrl Pts',(-9.78949966687058,-0.557154704495792,
18.073209998108));
#24824=CARTESIAN_POINT('Ctrl Pts',(-8.72938063795075,-1.38688366691717,
18.1209320215629));
#24825=CARTESIAN_POINT('Ctrl Pts',(-7.45616349878414,-0.941690303216765,
18.1686540450177));
#24826=CARTESIAN_POINT('Ctrl Pts',(-7.1975111877415,0.148686971261949,18.2084223978968));
#24827=CARTESIAN_POINT('Ctrl Pts',(-7.60845568768243,0.854967565251188,
18.2402370802));
#24828=CARTESIAN_POINT('Ctrl Pts',(-8.29691194327969,1.29512167872335,18.2720517625033));
#24829=CARTESIAN_POINT('Ctrl Pts',(-9.39716218903309,1.08234711392068,18.3118201153823));
#24830=CARTESIAN_POINT('Ctrl Pts',(-9.89527113707947,-0.171114688619274,
18.3595421388372));
#24831=CARTESIAN_POINT('Ctrl Pts',(-9.11065382231136,-1.26504255457975,
18.4072641622921));
#24832=CARTESIAN_POINT('Ctrl Pts',(-7.76606111074645,-1.19891429613197,
18.4549861857469));
#24833=CARTESIAN_POINT('Ctrl Pts',(-7.0944670580837,-0.0291961920664319,
18.5027082092018));
#24834=CARTESIAN_POINT('Ctrl Pts',(-7.61227126287659,0.96463599910374,18.5424765620808));
#24835=CARTESIAN_POINT('Ctrl Pts',(-8.38515391517273,1.22989071679447,18.5742912443841));
#24836=CARTESIAN_POINT('Ctrl Pts',(-9.1937848058798,1.11231630600828,18.6061059266873));
#24837=CARTESIAN_POINT('Ctrl Pts',(-9.88663879356476,0.23153428390719,18.6458742795664));
#24838=CARTESIAN_POINT('Ctrl Pts',(-9.4432216954944,-1.04230255481647,18.6935963030212));
#24839=CARTESIAN_POINT('Ctrl Pts',(-8.13411829477636,-1.35623056055514,
18.7413183264762));
#24840=CARTESIAN_POINT('Ctrl Pts',(-7.1605319179062,-0.42648216806842,18.7890403499309));
#24841=CARTESIAN_POINT('Ctrl Pts',(-7.4179585923105,0.897530868822023,18.8367623733859));
#24842=CARTESIAN_POINT('Ctrl Pts',(-8.45979320188161,1.31033138360747,18.8765307262648));
#24843=CARTESIAN_POINT('Ctrl Pts',(-9.21783884631427,1.0052503117033,18.9083454085682));
#24844=CARTESIAN_POINT('Ctrl Pts',(-9.75244218309404,0.387264121095941,
18.9401600908714));
#24845=CARTESIAN_POINT('Ctrl Pts',(-9.70013819501298,-0.732149971873314,
18.9799284437504));
#24846=CARTESIAN_POINT('Ctrl Pts',(-8.53135794136673,-1.40537484755547,
19.0276504672053));
#24847=CARTESIAN_POINT('Ctrl Pts',(-7.33594766868813,-0.786265175095812,
19.0753724906601));
#24848=CARTESIAN_POINT('Ctrl Pts',(-7.20798451957174,0.553857184626204,
19.123094514115));
#24849=CARTESIAN_POINT('Ctrl Pts',(-8.26893812686215,1.3867175917342,19.1708165375699));
#24850=CARTESIAN_POINT('Ctrl Pts',(-9.32691568795275,1.01724892061836,19.2105848904489));
#24851=CARTESIAN_POINT('Ctrl Pts',(-9.70058210710294,0.290557055604711,
19.2423995727522));
#24852=CARTESIAN_POINT('Ctrl Pts',(-9.70054231361888,-0.526576750998593,
19.2742142550554));
#24853=CARTESIAN_POINT('Ctrl Pts',(-8.92857819660635,-1.33891597863224,
19.3139826079344));
#24854=CARTESIAN_POINT('Ctrl Pts',(-7.60420739907338,-1.08333623531821,
19.3617046313893));
#24855=CARTESIAN_POINT('Ctrl Pts',(-7.10524482354957,0.16699926157266,19.4094266548442));
#24856=CARTESIAN_POINT('Ctrl Pts',(-7.88528608756766,1.26419483802554,19.457148678299));
#24857=CARTESIAN_POINT('Ctrl Pts',(-9.23255879006808,1.19988869797871,19.5048707017539));
#24858=CARTESIAN_POINT('Ctrl Pts',(-9.79092226776038,0.228264364459435,
19.5446390546329));
#24859=CARTESIAN_POINT('Ctrl Pts',(-9.59804956384096,-0.565780835488472,
19.5764537369362));
#24860=CARTESIAN_POINT('Ctrl Pts',(-9.06338603915228,-1.18371495401972,
19.6082684192394));
#24861=CARTESIAN_POINT('Ctrl Pts',(-7.94808917357633,-1.29296933765633,
19.6480367721185));
#24862=CARTESIAN_POINT('Ctrl Pts',(-7.11374980070125,-0.233178402886113,
19.6957587955734));
#24863=CARTESIAN_POINT('Ctrl Pts',(-7.55447586424967,1.03885266727995,19.7434808190282));
#24864=CARTESIAN_POINT('Ctrl Pts',(-8.86225660550994,1.3582459035067,19.7912028424831));
#24865=CARTESIAN_POINT('Ctrl Pts',(-9.83906190809751,0.42812203251564,19.8389248659379));
#24866=CARTESIAN_POINT('Ctrl Pts',(-9.62561281515307,-0.671997553451521,
19.878693218817));
#24867=CARTESIAN_POINT('Ctrl Pts',(-8.96022515044173,-1.14630432667693,
19.9105079011202));
#24868=CARTESIAN_POINT('Ctrl Pts',(-8.15158281209082,-1.26379997810217,
19.9423225834235));
#24869=CARTESIAN_POINT('Ctrl Pts',(-7.23665301314377,-0.616708731286011,
19.9820909363026));
#24870=CARTESIAN_POINT('Ctrl Pts',(-7.29907996828855,0.730652352396478,
20.0298129597574));
#24871=CARTESIAN_POINT('Ctrl Pts',(-8.46464364182645,1.40427229679211,20.0775349832123));
#24872=CARTESIAN_POINT('Ctrl Pts',(-9.66262943404131,0.790161111248278,
20.1252570066671));
#24873=CARTESIAN_POINT('Ctrl Pts',(-9.79278123874688,-0.552351280606063,
20.172979030122));
#24874=CARTESIAN_POINT('Ctrl Pts',(-8.91157459044358,-1.24466512684449,
20.212747383001));
#24875=CARTESIAN_POINT('Ctrl Pts',(-8.09804403259428,-1.16801207130933,
20.2445620653043));
#24876=CARTESIAN_POINT('Ctrl Pts',(-7.40963065026857,-0.727790905856804,
20.2763767476075));
#24877=CARTESIAN_POINT('Ctrl Pts',(-7.141090118815,0.360193285974096,20.3161451004866));
#24878=CARTESIAN_POINT('Ctrl Pts',(-8.06985067592889,1.33829493820663,20.3638671239414));
#24879=CARTESIAN_POINT('Ctrl Pts',(-9.39204740920843,1.08511850750307,20.4115891473963));
#24880=CARTESIAN_POINT('Ctrl Pts',(-9.89622813459281,-0.163121975220366,
20.4593111708511));
#24881=CARTESIAN_POINT('Ctrl Pts',(-9.116278300971,-1.26355701264145,20.507033194306));
#24882=CARTESIAN_POINT('Ctrl Pts',(-7.99689648619272,-1.21056671682166,
20.5468015471851));
#24883=CARTESIAN_POINT('Ctrl Pts',(-7.43181377943531,-0.620321688040228,
20.5786162294883));
#24884=CARTESIAN_POINT('Ctrl Pts',(-7.19922630521013,0.163011399675998,
20.6104309117915));
#24885=CARTESIAN_POINT('Ctrl Pts',(-7.70798676693442,1.16150346839434,20.6501992646706));
#24886=CARTESIAN_POINT('Ctrl Pts',(-9.05031632239779,1.29352762936509,20.6979212881254));
#24887=CARTESIAN_POINT('Ctrl Pts',(-9.88458398875966,0.2369766521653,20.7456433115803));
#24888=CARTESIAN_POINT('Ctrl Pts',(-9.44917489199335,-1.0368841820752,20.7933653350352));
#24889=CARTESIAN_POINT('Ctrl Pts',(-8.13934378422536,-1.35878709239757,
20.84108735849));
#24890=CARTESIAN_POINT('Ctrl Pts',(-7.32747800377215,-0.586325071818895,
20.8808557113691));
#24891=CARTESIAN_POINT('Ctrl Pts',(-7.28631721489128,0.229771398542417,
20.9126703936723));
#24892=CARTESIAN_POINT('Ctrl Pts',(-7.62294049781938,0.974346730438525,
20.9444850759756));
#24893=CARTESIAN_POINT('Ctrl Pts',(-8.66098460634993,1.39658842360999,20.9842534288546));
#24894=CARTESIAN_POINT('Ctrl Pts',(-9.76250641639258,0.618174191628754,
21.0319754523095));
#24895=CARTESIAN_POINT('Ctrl Pts',(-9.70214506892388,-0.726689747322114,
21.0796974757644));
#24896=CARTESIAN_POINT('Ctrl Pts',(-8.5394051930937,-1.40517223619938,21.1274194992192));
#24897=CARTESIAN_POINT('Ctrl Pts',(-7.33822677752304,-0.791617488423931,
21.1751415226741));
#24898=CARTESIAN_POINT('Ctrl Pts',(-7.22965620770004,0.3237461518637,21.2149098755531));
#24899=CARTESIAN_POINT('Ctrl Pts',(-7.73248294792305,0.967852454265888,
21.2467245578564));
#24900=CARTESIAN_POINT('Ctrl Pts',(-8.47421537311915,1.31069450082703,21.2785392401596));
#24901=CARTESIAN_POINT('Ctrl Pts',(-9.53550351928153,0.950845797171466,
21.3183075930387));
#24902=CARTESIAN_POINT('Ctrl Pts',(-9.85923301680232,-0.358535059182232,
21.3660296164935));
#24903=CARTESIAN_POINT('Ctrl Pts',(-8.93366841152947,-1.33609972099487,
21.4137516399484));
#24904=CARTESIAN_POINT('Ctrl Pts',(-7.61042572425391,-1.08844815703786,
21.4614736634032));
#24905=CARTESIAN_POINT('Ctrl Pts',(-7.10346650134907,0.161460383961172,
21.5091956868581));
#24906=CARTESIAN_POINT('Ctrl Pts',(-7.75111857391915,1.07599327653694,21.5489640397371));
#24907=CARTESIAN_POINT('Ctrl Pts',(-8.55280814670003,1.23411186612053,21.5807787220404));
#24908=CARTESIAN_POINT('Ctrl Pts',(-9.33806008278557,1.00808740648967,21.6125934043437));
#24909=CARTESIAN_POINT('Ctrl Pts',(-9.9052213434253,0.0415721592550428,
21.6523617572227));
#24910=CARTESIAN_POINT('Ctrl Pts',(-9.29334254829634,-1.16046084970195,
21.7000837806776));
#24911=CARTESIAN_POINT('Ctrl Pts',(-7.95378128354117,-1.29416995382799,
21.7478058041324));
#24912=CARTESIAN_POINT('Ctrl Pts',(-7.11510780710624,-0.241112829791858,
21.7955278275873));
#24913=CARTESIAN_POINT('Ctrl Pts',(-7.5495070312765,1.03582739143655,21.8432498510421));
#24914=CARTESIAN_POINT('Ctrl Pts',(-8.63765566197109,1.30370082465606,21.8830182039212));
#24915=CARTESIAN_POINT('Ctrl Pts',(-9.34738972466389,0.898749939077283,
21.9148328862245));
#24916=CARTESIAN_POINT('Ctrl Pts',(-9.79335606771826,0.214044396277898,
21.9466475685277));
#24917=CARTESIAN_POINT('Ctrl Pts',(-9.58990309483685,-0.887967630214171,
21.9864159214067));
#24918=CARTESIAN_POINT('Ctrl Pts',(-8.34070285614741,-1.39666968270552,
22.0341379448616));
#24919=CARTESIAN_POINT('Ctrl Pts',(-7.24017215234422,-0.621340928856387,
22.0818599683165));
#24920=CARTESIAN_POINT('Ctrl Pts',(-7.29491563681422,0.723763400728039,
22.1295819917713));
#24921=CARTESIAN_POINT('Ctrl Pts',(-8.45890657115661,1.40523542459937,22.1773040152262));
#24922=CARTESIAN_POINT('Ctrl Pts',(-9.45708652899441,0.895862878737048,
22.2170723681053));
#24923=CARTESIAN_POINT('Ctrl Pts',(-9.72887443943722,0.125253385404268,
22.2488870504085));
#24924=CARTESIAN_POINT('Ctrl Pts',(-9.61814955891965,-0.684343835633367,
22.2807017327117));
#24925=CARTESIAN_POINT('Ctrl Pts',(-8.74326432564931,-1.38462909701821,
22.3204700855908));
#24926=CARTESIAN_POINT('Ctrl Pts',(-7.46571946372151,-0.95201132078553,
22.3681921090456));
#24927=CARTESIAN_POINT('Ctrl Pts',(-7.14072073026172,0.354387672557732,
22.4159141325005));
#24928=CARTESIAN_POINT('Ctrl Pts',(-8.06219409051336,1.33580977996379,22.4636361559554));
#24929=CARTESIAN_POINT('Ctrl Pts',(-9.38833888469312,1.08960052055111,22.5113581794102));
#24930=CARTESIAN_POINT('Ctrl Pts',(-9.80994406922133,0.0512977289309273,
22.5511265322893));
#24931=CARTESIAN_POINT('Ctrl Pts',(-9.51129102603857,-0.709303361835555,
22.5829412145925));
#24932=CARTESIAN_POINT('Ctrl Pts',(-8.89785256586858,-1.24911899245564,
22.6147558968957));
#24933=CARTESIAN_POINT('Ctrl Pts',(-7.7780358132456,-1.20629307445875,22.6545242497748));
#24934=CARTESIAN_POINT('Ctrl Pts',(-7.09494096399137,-0.0432537623660983,
22.7022462732296));
#24935=CARTESIAN_POINT('Ctrl Pts',(-7.70390892509399,1.15735463711693,22.7499682966846));
#24936=CARTESIAN_POINT('Ctrl Pts',(-9.04290001758308,1.29665776268707,22.7976903201394));
#24937=CARTESIAN_POINT('Ctrl Pts',(-9.88471189147151,0.24279259885862,22.8454123435943));
#24938=CARTESIAN_POINT('Ctrl Pts',(-9.52421257514643,-0.818274723056693,
22.8851806964733));
#24939=CARTESIAN_POINT('Ctrl Pts',(-8.80070995351091,-1.19807943072104,
22.9169953787766));
#24940=CARTESIAN_POINT('Ctrl Pts',(-7.98360508912736,-1.20495693595516,
22.9488100610798));
#24941=CARTESIAN_POINT('Ctrl Pts',(-7.16476004726262,-0.439897189189659,
22.9885784139589));
#24942=CARTESIAN_POINT('Ctrl Pts',(-7.40911941320573,0.8865897179551,23.0363004374137));
#24943=CARTESIAN_POINT('Ctrl Pts',(-8.65518623203828,1.39611890216659,23.0840224608686));
#24944=CARTESIAN_POINT('Ctrl Pts',(-9.75894579152361,0.625393697308581,
23.1317444843234));
#24945=CARTESIAN_POINT('Ctrl Pts',(-9.70604704714024,-0.722375102372304,
23.1794665077783));
#24946=CARTESIAN_POINT('Ctrl Pts',(-8.73918425256553,-1.28894368178221,
23.2192348606573));
#24947=CARTESIAN_POINT('Ctrl Pts',(-7.9435347756856,-1.10279973367158,23.2510495429606));
#24948=CARTESIAN_POINT('Ctrl Pts',(-7.32109670201655,-0.573386375392157,
23.2828642252638));
#24949=CARTESIAN_POINT('Ctrl Pts',(-7.20240489080355,0.540945654416883,
23.3226325781429));
#24950=CARTESIAN_POINT('Ctrl Pts',(-8.25509490385685,1.38422659868659,23.3703546015978));
#24951=CARTESIAN_POINT('Ctrl Pts',(-9.53081128146812,0.954284474147591,
23.4180766250526));
#24952=CARTESIAN_POINT('Ctrl Pts',(-9.86126385285633,-0.350745642218154,
23.4657986485075));
#24953=CARTESIAN_POINT('Ctrl Pts',(-8.93944227678327,-1.33538973854775,
23.5135206719623));
#24954=CARTESIAN_POINT('Ctrl Pts',(-7.83755519530068,-1.13126115561726,
23.5532890248414));
#24955=CARTESIAN_POINT('Ctrl Pts',(-7.35763269918339,-0.469912490238693,
23.5851037071446));
#24956=CARTESIAN_POINT('Ctrl Pts',(-7.23329584348133,0.337706235269606,
23.6169183894479));
#24957=CARTESIAN_POINT('Ctrl Pts',(-7.87261873264457,1.25808108395866,23.6566867423269));
#24958=CARTESIAN_POINT('Ctrl Pts',(-9.22046000244338,1.20706220531818,23.7044087657818));
#24959=CARTESIAN_POINT('Ctrl Pts',(-9.90392267688262,0.047242702461344,
23.7521307892367));
#24960=CARTESIAN_POINT('Ctrl Pts',(-9.29997482618396,-1.15589881049347,
23.7998528126915));
#24961=CARTESIAN_POINT('Ctrl Pts',(-7.95861231486585,-1.29741074561148,
23.8475748361464));
#24962=CARTESIAN_POINT('Ctrl Pts',(-7.25886358097769,-0.422096328884932,
23.8873431890254));
#24963=CARTESIAN_POINT('Ctrl Pts',(-7.32862709527643,0.392053971459042,
23.9191578713287));
#24964=CARTESIAN_POINT('Ctrl Pts',(-7.76300484896508,1.08416929897163,23.9509725536319));
#24965=CARTESIAN_POINT('Ctrl Pts',(-8.84867677583206,1.36191034008796,23.990740906511));
#24966=CARTESIAN_POINT('Ctrl Pts',(-9.83460563447141,0.441463003054064,
24.0384629299658));
#24967=CARTESIAN_POINT('Ctrl Pts',(-9.59263109087989,-0.882829572932237,
24.0861849534207));
#24968=CARTESIAN_POINT('Ctrl Pts',(-8.34870338444389,-1.39755898506989,
24.1339069768756));
#24969=CARTESIAN_POINT('Ctrl Pts',(-7.24170525405229,-0.626952630398398,
24.1816290003304));
#24970=CARTESIAN_POINT('Ctrl Pts',(-7.28521772844163,0.492837655003246,
24.2213973532095));
#24971=CARTESIAN_POINT('Ctrl Pts',(-7.87065800324083,1.06289672573235,24.2532120355127));
#24972=CARTESIAN_POINT('Ctrl Pts',(-8.65199409613447,1.30210702948024,24.2850267178159));
#24973=CARTESIAN_POINT('Ctrl Pts',(-9.65475720639185,0.801817349980151,
24.324795070695));
#24974=CARTESIAN_POINT('Ctrl Pts',(-9.79813988291764,-0.539346481407673,
24.3725170941499));
#24975=CARTESIAN_POINT('Ctrl Pts',(-8.74868910432396,-1.38252829446333,
24.4202391176047));
#24976=CARTESIAN_POINT('Ctrl Pts',(-7.47118803801445,-0.957918435726028,
24.4679611410596));
#24977=CARTESIAN_POINT('Ctrl Pts',(-7.13820852545198,0.349140728491224,
24.5156831645144));
#24978=CARTESIAN_POINT('Ctrl Pts',(-7.9037701658238,1.16751655505172,24.5554515173935));
#24979=CARTESIAN_POINT('Ctrl Pts',(-8.71948895511468,1.21558438499351,24.5872661996968));
#24980=CARTESIAN_POINT('Ctrl Pts',(-9.46688723084328,0.885276230514411,
24.619080882));
#24981=CARTESIAN_POINT('Ctrl Pts',(-9.89790116767083,-0.149156273309663,
24.658849234879));
#24982=CARTESIAN_POINT('Ctrl Pts',(-9.1288395594926,-1.25722813802644,24.7065712583339));
#24983=CARTESIAN_POINT('Ctrl Pts',(-7.78351283097435,-1.20825365392482,
24.7542932817887));
#24984=CARTESIAN_POINT('Ctrl Pts',(-7.09521169063023,-0.0512990105788772,
24.8020153052436));
#24985=CARTESIAN_POINT('Ctrl Pts',(-7.69857609692742,1.15503030091294,24.8497373286984));
#24986=CARTESIAN_POINT('Ctrl Pts',(-8.81298068775674,1.27303888808352,24.8895056815776));
#24987=CARTESIAN_POINT('Ctrl Pts',(-9.46132049901386,0.775682729363686,
24.9213203638807));
#24988=CARTESIAN_POINT('Ctrl Pts',(-9.8104292616916,0.0368791483632278,
24.9531350461841));
#24989=CARTESIAN_POINT('Ctrl Pts',(-9.45957759328401,-1.02741720391978,
24.992903399063));
#24990=CARTESIAN_POINT('Ctrl Pts',(-8.15298412698885,-1.36221942671018,
25.0406254225179));
#24991=CARTESIAN_POINT('Ctrl Pts',(-7.167619294276,-0.444963381207372,25.0883474459728));
#24992=CARTESIAN_POINT('Ctrl Pts',(-7.40406031475195,0.880328341544631,
25.1360694694276));
#24993=CARTESIAN_POINT('Ctrl Pts',(-8.64963249883034,1.39785027228844,25.1837914928825));
#24994=CARTESIAN_POINT('Ctrl Pts',(-9.56961520293805,0.757963217527989,
25.2235598457616));
#24995=CARTESIAN_POINT('Ctrl Pts',(-9.73451468385032,-0.0423591054596894,
25.2553745280648));
#24996=CARTESIAN_POINT('Ctrl Pts',(-9.51514573013107,-0.829496273697633,
25.2871892103681));
#24997=CARTESIAN_POINT('Ctrl Pts',(-8.55346631480298,-1.40481907077904,
25.3269575632471));
#24998=CARTESIAN_POINT('Ctrl Pts',(-7.34629662801778,-0.80313779148113,
25.374679586702));
#24999=CARTESIAN_POINT('Ctrl Pts',(-7.20125250317102,0.535243584811184,
25.4224016101568));
#25000=CARTESIAN_POINT('Ctrl Pts',(-8.24717225720877,1.38280147349625,25.4701236336117));
#25001=CARTESIAN_POINT('Ctrl Pts',(-9.52774405127491,0.959227519159094,
25.5178456570666));
#25002=CARTESIAN_POINT('Ctrl Pts',(-9.80481941008746,-0.126614487877935,
25.5576140099456));
#25003=CARTESIAN_POINT('Ctrl Pts',(-9.40589115882078,-0.839751157681684,
25.5894286922489));
#25004=CARTESIAN_POINT('Ctrl Pts',(-8.72498539679587,-1.29149777108218,
25.6212433745521));
#25005=CARTESIAN_POINT('Ctrl Pts',(-7.62129056292958,-1.09738097014961,
25.6610117274311));
#25006=CARTESIAN_POINT('Ctrl Pts',(-7.10203186105147,0.147468183392511,
25.708733750886));
#25007=CARTESIAN_POINT('Ctrl Pts',(-7.8680164916839,1.25452285782985,25.7564557743409));
#25008=CARTESIAN_POINT('Ctrl Pts',(-9.21353604522699,1.2111680704139,25.8041777977957));
#25009=CARTESIAN_POINT('Ctrl Pts',(-9.90483720405359,0.0529877207465818,
25.8518998212506));
#25010=CARTESIAN_POINT('Ctrl Pts',(-9.40393282022959,-0.94946847130034,
25.8916681741296));
#25011=CARTESIAN_POINT('Ctrl Pts',(-8.63565170996194,-1.22777009738866,
25.9234828564329));
#25012=CARTESIAN_POINT('Ctrl Pts',(-7.82514617666876,-1.12390268200446,
25.9552975387361));
#25013=CARTESIAN_POINT('Ctrl Pts',(-7.11747982604816,-0.254976934367291,
25.9950658916152));
#25014=CARTESIAN_POINT('Ctrl Pts',(-7.53926727780403,1.0261843982103,26.04278791507));
#25015=CARTESIAN_POINT('Ctrl Pts',(-8.84286824344772,1.36223056904334,26.0905099385249));
#25016=CARTESIAN_POINT('Ctrl Pts',(-9.83205574984714,0.44909827646907,26.1382319619798));
#25017=CARTESIAN_POINT('Ctrl Pts',(-9.59708154949269,-0.879083239634216,
26.1859539854346));
#25018=CARTESIAN_POINT('Ctrl Pts',(-8.56238498360011,-1.30946288046009,
26.2257223383137));
#25019=CARTESIAN_POINT('Ctrl Pts',(-7.79928295337053,-1.01725926833834,
26.2575370206169));
#25020=CARTESIAN_POINT('Ctrl Pts',(-7.25429371365722,-0.408412499377393,
26.2893517029202));
#25021=CARTESIAN_POINT('Ctrl Pts',(-7.28763849254092,0.711726663596802,
26.3291200557992));
#25022=CARTESIAN_POINT('Ctrl Pts',(-8.44485351632405,1.40464253387347,26.3768420792541));
#25023=CARTESIAN_POINT('Ctrl Pts',(-9.65057400354622,0.805859924530725,
26.4245641027089));
#25024=CARTESIAN_POINT('Ctrl Pts',(-9.8012071227059,-0.531903944756735,
26.4722861261638));
#25025=CARTESIAN_POINT('Ctrl Pts',(-8.7545059253607,-1.38260695875558,26.5200081496186));
#25026=CARTESIAN_POINT('Ctrl Pts',(-7.69042488176934,-1.03110283164356,
26.5597765024977));
#25027=CARTESIAN_POINT('Ctrl Pts',(-7.30450910349292,-0.310841301673525,
26.591591184801));
#25028=CARTESIAN_POINT('Ctrl Pts',(-7.29071479240244,0.506176064395959,
26.6234058671042));
#25029=CARTESIAN_POINT('Ctrl Pts',(-8.04881534252997,1.33146823969133,26.6631742199833));
#25030=CARTESIAN_POINT('Ctrl Pts',(-9.3773232994039,1.09834676261705,26.7108962434381));
#25031=CARTESIAN_POINT('Ctrl Pts',(-9.89738257797027,-0.143362081410278,
26.758618266893));
#25032=CARTESIAN_POINT('Ctrl Pts',(-9.13602866466635,-1.25360652533043,
26.8063402903478));
#25033=CARTESIAN_POINT('Ctrl Pts',(-7.78786035280959,-1.21211896748734,
26.8540623138027));
#25034=CARTESIAN_POINT('Ctrl Pts',(-7.21312727362265,-0.250087000037398,
26.8938306666818));
#25035=CARTESIAN_POINT('Ctrl Pts',(-7.39252912631154,0.54710973523519,26.925645348985));
#25036=CARTESIAN_POINT('Ctrl Pts',(-7.91665437889142,1.17400715833212,26.9574600312882));
#25037=CARTESIAN_POINT('Ctrl Pts',(-9.02994171668213,1.30212789132369,26.9972283841673));
#25038=CARTESIAN_POINT('Ctrl Pts',(-9.88210380039875,0.256614238793779,
27.0449504076221));
#25039=CARTESIAN_POINT('Ctrl Pts',(-9.46297642576351,-1.02269602474285,
27.092672431077));
#25040=CARTESIAN_POINT('Ctrl Pts',(-8.16079045651933,-1.36418425010698,
27.1403944545319));
#25041=CARTESIAN_POINT('Ctrl Pts',(-7.16837812888729,-0.450731029348263,
27.1881164779867));
#25042=CARTESIAN_POINT('Ctrl Pts',(-7.36317157335998,0.652844583239182,
27.2278848308658));
#25043=CARTESIAN_POINT('Ctrl Pts',(-8.02043384525043,1.13834840961636,27.259699513169));
#25044=CARTESIAN_POINT('Ctrl Pts',(-8.82697108162581,1.26951755925708,27.2915141954723));
#25045=CARTESIAN_POINT('Ctrl Pts',(-9.75272502333722,0.638008843471489,
27.3312825483513));
#25046=CARTESIAN_POINT('Ctrl Pts',(-9.71311787736138,-0.710216022245723,
27.3790045718062));
#25047=CARTESIAN_POINT('Ctrl Pts',(-8.55912566120076,-1.40347244781957,
27.4267265952611));
#25048=CARTESIAN_POINT('Ctrl Pts',(-7.35091464810136,-0.809731212613409,
27.4744486187159));
#25049=CARTESIAN_POINT('Ctrl Pts',(-7.19805272372483,0.530385292257197,
27.5221706421708));
#25050=CARTESIAN_POINT('Ctrl Pts',(-8.06741218131559,1.23751876777988,27.5619389950498));
#25051=CARTESIAN_POINT('Ctrl Pts',(-8.88212387979244,1.17464979417261,27.593753677353));
#25052=CARTESIAN_POINT('Ctrl Pts',(-9.57789155350878,0.74614658101211,27.6255683596563));
#25053=CARTESIAN_POINT('Ctrl Pts',(-9.86481320056272,-0.337135278505183,
27.6653367125353));
#25054=CARTESIAN_POINT('Ctrl Pts',(-8.95274504552348,-1.33082068904202,
27.7130587359902));
#25055=CARTESIAN_POINT('Ctrl Pts',(-7.62645152946083,-1.10006537315734,
27.7607807594451));
#25056=CARTESIAN_POINT('Ctrl Pts',(-7.10121031756601,0.139460413539338,
27.8085027829));
#25057=CARTESIAN_POINT('Ctrl Pts',(-7.86241796941027,1.25294230621852,27.8562248063548));
#25058=CARTESIAN_POINT('Ctrl Pts',(-8.98253647802948,1.21891077148923,27.8959931592339));
#25059=CARTESIAN_POINT('Ctrl Pts',(-9.55753106065096,0.638317205013169,
27.927807841537));
#25060=CARTESIAN_POINT('Ctrl Pts',(-9.80334705142044,-0.140965900257004,
27.9596225238404));
#25061=CARTESIAN_POINT('Ctrl Pts',(-9.3115640063478,-1.14792819115299,27.9993908767193));
#25062=CARTESIAN_POINT('Ctrl Pts',(-7.97166201070898,-1.30265910801723,
28.0471129001743));
#25063=CARTESIAN_POINT('Ctrl Pts',(-7.11962647580337,-0.260383734703235,
28.0948349236291));
#25064=CARTESIAN_POINT('Ctrl Pts',(-7.53340666774274,1.02066601425938,28.142556947084));
#25065=CARTESIAN_POINT('Ctrl Pts',(-8.83760022077483,1.36469826678866,28.1902789705388));
#25066=CARTESIAN_POINT('Ctrl Pts',(-9.66242744626732,0.606091868981755,
28.2300473234179));
#25067=CARTESIAN_POINT('Ctrl Pts',(-9.71739887259082,-0.209190782474407,
28.2618620057211));
#25068=CARTESIAN_POINT('Ctrl Pts',(-9.3934295173966,-0.959358441316799,
28.2936766880244));
#25069=CARTESIAN_POINT('Ctrl Pts',(-8.36268274870058,-1.39911373409659,
28.3334450409034));
#25070=CARTESIAN_POINT('Ctrl Pts',(-7.24814023693788,-0.639459862898064,
28.3811670643583));
#25071=CARTESIAN_POINT('Ctrl Pts',(-7.28572434802244,0.706233245190266,
28.4288890878131));
#25072=CARTESIAN_POINT('Ctrl Pts',(-8.43681084816737,1.40430371135129,28.4766111112681));
#25073=CARTESIAN_POINT('Ctrl Pts',(-9.64820460654916,0.811172885373071,
28.5243331347228));
#25074=CARTESIAN_POINT('Ctrl Pts',(-9.77564275421098,-0.302192794555114,
28.564101487602));
#25075=CARTESIAN_POINT('Ctrl Pts',(-9.28379281900323,-0.954719652751162,
28.5959161699052));
#25076=CARTESIAN_POINT('Ctrl Pts',(-8.54797102693755,-1.31007011342867,
28.6277308522084));
#25077=CARTESIAN_POINT('Ctrl Pts',(-7.48074273921507,-0.968240623257071,
28.6674992050875));
#25078=CARTESIAN_POINT('Ctrl Pts',(-7.13489178381066,0.335471818616655,
28.7152212285423));
#25079=CARTESIAN_POINT('Ctrl Pts',(-8.04377353674895,1.32856620832038,28.7629432519972));
#25080=CARTESIAN_POINT('Ctrl Pts',(-9.37101931995447,1.10335267503478,28.810665275452));
#25081=CARTESIAN_POINT('Ctrl Pts',(-9.89906687296496,-0.137793890164783,
28.8583872989069));
#25082=CARTESIAN_POINT('Ctrl Pts',(-9.26699068934855,-1.06316047838938,
28.8981556517859));
#25083=CARTESIAN_POINT('Ctrl Pts',(-8.46809297375091,-1.23482903167168,
28.9299703340892));
#25084=CARTESIAN_POINT('Ctrl Pts',(-7.67912697365966,-1.02213130798338,
28.9617850163925));
#25085=CARTESIAN_POINT('Ctrl Pts',(-7.09568388763803,-0.0653566335221624,
29.0015533692715));
#25086=CARTESIAN_POINT('Ctrl Pts',(-7.68712449973501,1.14686320768974,29.0492753927264));
#25087=CARTESIAN_POINT('Ctrl Pts',(-9.02423013404472,1.30323198402877,29.0969974161812));
#25088=CARTESIAN_POINT('Ctrl Pts',(-9.88061158665234,0.264524506767463,
29.1447194396361));
#25089=CARTESIAN_POINT('Ctrl Pts',(-9.4678934712441,-1.0195869991764,29.1924414630909));
#25090=CARTESIAN_POINT('Ctrl Pts',(-8.38443551051107,-1.30584459467476,
29.23220981597));
#25091=CARTESIAN_POINT('Ctrl Pts',(-7.6679479210642,-0.912967317898404,
29.2640244982733));
#25092=CARTESIAN_POINT('Ctrl Pts',(-7.21045226783838,-0.235910619659525,
29.2958391805765));
#25093=CARTESIAN_POINT('Ctrl Pts',(-7.39522151652002,0.869389006667542,
29.3356075334556));
#25094=CARTESIAN_POINT('Ctrl Pts',(-8.63562576788721,1.39916518175529,29.3833295569103));
#25095=CARTESIAN_POINT('Ctrl Pts',(-9.74913324417835,0.642583048872662,
29.4310515803653));
#25096=CARTESIAN_POINT('Ctrl Pts',(-9.71715498903128,-0.703261816482831,
29.4787736038201));
#25097=CARTESIAN_POINT('Ctrl Pts',(-8.56489804327719,-1.40432985445164,
29.526495627275));
#25098=CARTESIAN_POINT('Ctrl Pts',(-7.55818298447205,-0.911952754888512,
29.566263980154));
#25099=CARTESIAN_POINT('Ctrl Pts',(-7.27346847986514,-0.14602059297262,
29.5980786624573));
#25100=CARTESIAN_POINT('Ctrl Pts',(-7.37031213472133,0.66526743560203,29.6298933447605));
#25101=CARTESIAN_POINT('Ctrl Pts',(-8.23356786559638,1.38041415523581,29.6696616976396));
#25102=CARTESIAN_POINT('Ctrl Pts',(-9.51761336754789,0.969214049802536,
29.7173837210944));
#25103=CARTESIAN_POINT('Ctrl Pts',(-9.86581870095987,-0.33101037424556,
29.7651057445493));
#25104=CARTESIAN_POINT('Ctrl Pts',(-8.95896334044735,-1.32880668070373,
29.8128277680042));
#25105=CARTESIAN_POINT('Ctrl Pts',(-7.85403417684868,-1.14084454386819,
29.8525961208832));
#25106=CARTESIAN_POINT('Ctrl Pts',(-7.36447187803796,-0.486329821775057,
29.8844108031865));
#25107=CARTESIAN_POINT('Ctrl Pts',(-7.22885571001066,0.319024610172502,
29.9162254854897));
#25108=CARTESIAN_POINT('Ctrl Pts',(-7.85366944090153,1.24940928029703,29.9559938383688));
#25109=CARTESIAN_POINT('Ctrl Pts',(-9.20420356711764,1.21639724974061,30.0037158618236));
#25110=CARTESIAN_POINT('Ctrl Pts',(-9.78431034371099,0.260901981677749,
30.0434842147027));
#25111=CARTESIAN_POINT('Ctrl Pts',(-9.61211124696142,-0.541081198726826,
30.0752988970059));
#25112=CARTESIAN_POINT('Ctrl Pts',(-9.3510349247924,-0.852523833800324,
30.0912062381575));
#25113=CARTESIAN_POINT('Ctrl Pts',(-9.18987679192715,-0.967444397671153,
30.0991599087333));
#25114=CARTESIAN_POINT('',(-9.01183881116714,1.07233375495133,30.));
#25115=CARTESIAN_POINT('Ctrl Pts',(-9.01356946732976,1.07334645743585,30.));
#25116=CARTESIAN_POINT('Ctrl Pts',(-9.0404013004879,1.05836761542857,30.));
#25117=CARTESIAN_POINT('Ctrl Pts',(-9.06653941803383,1.04232411727425,30.));
#25118=CARTESIAN_POINT('Ctrl Pts',(-9.09191232737533,1.02521683657113,30.));
#25119=CARTESIAN_POINT('Ctrl Pts',(-9.13297340585366,0.9975320572639,30.));
#25120=CARTESIAN_POINT('Ctrl Pts',(-9.17203266553443,0.967063261291628,
30.));
#25121=CARTESIAN_POINT('Ctrl Pts',(-9.20897145121856,0.9341121128447,30.));
#25122=CARTESIAN_POINT('Ctrl Pts',(-9.23971661511987,0.906685968726147,
30.));
#25123=CARTESIAN_POINT('Ctrl Pts',(-9.2689923033626,0.877538967782025,30.));
#25124=CARTESIAN_POINT('Ctrl Pts',(-9.29670822146099,0.846828311807377,
30.));
#25125=CARTESIAN_POINT('Ctrl Pts',(-9.30970173078921,0.832430838360316,
30.));
#25126=CARTESIAN_POINT('Ctrl Pts',(-9.32235212446905,0.817689530036482,
30.));
#25127=CARTESIAN_POINT('Ctrl Pts',(-9.33464839610017,0.802619887632117,
30.));
#25128=CARTESIAN_POINT('Ctrl Pts',(-9.34095951606682,0.794885321909954,
30.));
#25129=CARTESIAN_POINT('Ctrl Pts',(-9.34717733114601,0.78706425754689,30.));
#25130=CARTESIAN_POINT('Ctrl Pts',(-9.35330023379542,0.779158763052844,
30.));
#25131=CARTESIAN_POINT('Ctrl Pts',(-9.35900505310472,0.77179307063187,30.));
#25132=CARTESIAN_POINT('Ctrl Pts',(-9.36462187785631,0.764361279806068,
30.));
#25133=CARTESIAN_POINT('Ctrl Pts',(-9.37014824198907,0.756867742145807,
30.));
#25134=CARTESIAN_POINT('Ctrl Pts',(-9.39935024489035,0.717270946994591,
30.));
#25135=CARTESIAN_POINT('Ctrl Pts',(-9.42604623385499,0.675931375532437,
30.));
#25136=CARTESIAN_POINT('Ctrl Pts',(-9.45011051308741,0.633132080589728,
30.));
#25137=CARTESIAN_POINT('Ctrl Pts',(-9.47490181921347,0.589039738880434,
30.));
#25138=CARTESIAN_POINT('Ctrl Pts',(-9.49690076359938,0.543396988540731,
30.));
#25139=CARTESIAN_POINT('Ctrl Pts',(-9.51591602634924,0.496493124727175,
30.));
#25140=CARTESIAN_POINT('Ctrl Pts',(-9.52463388565747,0.474989278521212,
30.));
#25141=CARTESIAN_POINT('Ctrl Pts',(-9.53272379643383,0.453220191416638,
30.));
#25142=CARTESIAN_POINT('Ctrl Pts',(-9.5401630139613,0.431213428814737,30.));
#25143=CARTESIAN_POINT('Ctrl Pts',(-9.5449227151396,0.41713323644234,30.));
#25144=CARTESIAN_POINT('Ctrl Pts',(-9.54941599265901,0.402955749296612,
30.));
#25145=CARTESIAN_POINT('Ctrl Pts',(-9.55363626349372,0.388688248405426,
30.));
#25146=CARTESIAN_POINT('Ctrl Pts',(-9.55641171336528,0.379305264453263,
30.));
#25147=CARTESIAN_POINT('Ctrl Pts',(-9.55906701928206,0.369890069837169,
30.));
#25148=CARTESIAN_POINT('Ctrl Pts',(-9.56159885895017,0.360452578677009,
30.));
#25149=CARTESIAN_POINT('Ctrl Pts',(-9.57396435642608,0.314359899669795,
30.));
#25150=CARTESIAN_POINT('Ctrl Pts',(-9.58340587491649,0.267678796348387,
30.));
#25151=CARTESIAN_POINT('Ctrl Pts',(-9.58977429414167,0.220657430411709,
30.));
#25152=CARTESIAN_POINT('Ctrl Pts',(-9.59595307893544,0.175036234545199,
30.));
#25153=CARTESIAN_POINT('Ctrl Pts',(-9.59923915769065,0.129093821702756,
30.));
#25154=CARTESIAN_POINT('Ctrl Pts',(-9.59944739469354,0.0830577788125183,
30.));
#25155=CARTESIAN_POINT('Ctrl Pts',(-9.59949272984566,0.0730352997219751,
30.));
#25156=CARTESIAN_POINT('Ctrl Pts',(-9.59939199084664,0.0630084152088303,
30.));
#25157=CARTESIAN_POINT('Ctrl Pts',(-9.59914293971342,0.0529795432812796,
30.));
#25158=CARTESIAN_POINT('Ctrl Pts',(-9.59854500970755,0.0289019035901314,
30.));
#25159=CARTESIAN_POINT('Ctrl Pts',(-9.59709240210605,0.0048126867034857,
30.));
#25160=CARTESIAN_POINT('Ctrl Pts',(-9.59479829199329,-0.0192454360586858,
30.));
#25161=CARTESIAN_POINT('Ctrl Pts',(-9.59353734581922,-0.0324688631660106,
30.));
#25162=CARTESIAN_POINT('Ctrl Pts',(-9.5920210560175,-0.0456892788046415,
30.));
#25163=CARTESIAN_POINT('Ctrl Pts',(-9.59025657526382,-0.0588641198083392,
30.));
#25164=CARTESIAN_POINT('Ctrl Pts',(-9.58407424635836,-0.105025688979562,
30.));
#25165=CARTESIAN_POINT('Ctrl Pts',(-9.57484586966463,-0.150694655922387,
30.));
#25166=CARTESIAN_POINT('Ctrl Pts',(-9.56272960679499,-0.195579451729583,
30.));
#25167=CARTESIAN_POINT('Ctrl Pts',(-9.55017158310486,-0.24210075414254,
30.));
#25168=CARTESIAN_POINT('Ctrl Pts',(-9.53451086275111,-0.287781072722504,
30.));
#25169=CARTESIAN_POINT('Ctrl Pts',(-9.51587014765823,-0.332272113111234,
30.));
#25170=CARTESIAN_POINT('Ctrl Pts',(-9.50654979011179,-0.354517633305599,
30.));
#25171=CARTESIAN_POINT('Ctrl Pts',(-9.49648365210744,-0.376465335235619,
30.));
#25172=CARTESIAN_POINT('Ctrl Pts',(-9.48568282591157,-0.398067850774574,
30.));
#25173=CARTESIAN_POINT('Ctrl Pts',(-9.48055176124769,-0.408330390150984,
30.));
#25174=CARTESIAN_POINT('Ctrl Pts',(-9.47525485138614,-0.418514982656314,
30.));
#25175=CARTESIAN_POINT('Ctrl Pts',(-9.46979309127951,-0.428616291644545,
30.));
#25176=CARTESIAN_POINT('Ctrl Pts',(-9.46522229892417,-0.437069791066159,
30.));
#25177=CARTESIAN_POINT('Ctrl Pts',(-9.46053625618582,-0.44546432784445,
30.));
#25178=CARTESIAN_POINT('Ctrl Pts',(-9.45574246837851,-0.453785377323363,
30.));
#25179=CARTESIAN_POINT('Ctrl Pts',(-9.45420664198032,-0.456451262415496,
30.));
#25180=CARTESIAN_POINT('Ctrl Pts',(-9.45265958743055,-0.459109921130538,
30.));
#25181=CARTESIAN_POINT('Ctrl Pts',(-9.45110134197801,-0.461761264311804,
30.));
#25182=CARTESIAN_POINT('Ctrl Pts',(-9.42910351919434,-0.499190398049958,
30.));
#25183=CARTESIAN_POINT('Ctrl Pts',(-9.40487798623216,-0.53516396160983,
30.));
#25184=CARTESIAN_POINT('Ctrl Pts',(-9.37856312896001,-0.56950997033306,
30.));
#25185=CARTESIAN_POINT('Ctrl Pts',(-9.35643733060892,-0.598388442114831,
30.));
#25186=CARTESIAN_POINT('Ctrl Pts',(-9.332833692907,-0.626116038782497,30.));
#25187=CARTESIAN_POINT('Ctrl Pts',(-9.30782041440045,-0.652572448466639,
30.));
#25188=CARTESIAN_POINT('Ctrl Pts',(-9.30064609642426,-0.660160685871532,
30.));
#25189=CARTESIAN_POINT('Ctrl Pts',(-9.2933564227585,-0.667643328887313,
30.));
#25190=CARTESIAN_POINT('Ctrl Pts',(-9.28596221946619,-0.675008596291465,
30.));
#25191=CARTESIAN_POINT('Ctrl Pts',(-9.25445294625133,-0.706394563617926,
30.));
#25192=CARTESIAN_POINT('Ctrl Pts',(-9.22100504610438,-0.735698182988929,
30.));
#25193=CARTESIAN_POINT('Ctrl Pts',(-9.185756453621,-0.762712472111516,30.));
#25194=CARTESIAN_POINT('Ctrl Pts',(-9.15521777370757,-0.786117115261243,
30.));
#25195=CARTESIAN_POINT('Ctrl Pts',(-9.12332669441508,-0.807803020376991,
30.));
#25196=CARTESIAN_POINT('Ctrl Pts',(-9.09015970213924,-0.82760676144889,
30.));
#25197=CARTESIAN_POINT('Ctrl Pts',(-9.68829027239597,-0.000978575593966811,
29.7537368763048));
#25198=CARTESIAN_POINT('Ctrl Pts',(-9.68913288765981,-0.0952583801369799,
29.757526499053));
#25199=CARTESIAN_POINT('Ctrl Pts',(-9.67882321668234,-0.189362368800223,
29.7613161218011));
#25200=CARTESIAN_POINT('Ctrl Pts',(-9.65664191863911,-0.280605687980609,
29.7651057445493));
#25201=CARTESIAN_POINT('Ctrl Pts',(-9.56353358078901,-0.663609143064989,
29.7810130857009));
#25202=CARTESIAN_POINT('Ctrl Pts',(-9.26124846061824,-0.996207911884316,
29.7969204268525));
#25203=CARTESIAN_POINT('Ctrl Pts',(-8.88912006781309,-1.12491486892692,
29.8128277680042));
#25204=CARTESIAN_POINT('Ctrl Pts',(-8.51699167500794,-1.25362182596952,
29.8287351091558));
#25205=CARTESIAN_POINT('Ctrl Pts',(-8.07502000956843,-1.1784369712353,29.8446424503074));
#25206=CARTESIAN_POINT('Ctrl Pts',(-7.76450868815171,-0.935203778959528,
29.860549791459));
#25207=CARTESIAN_POINT('Ctrl Pts',(-7.60925302744333,-0.81358718282163,
29.8685034620348));
#25208=CARTESIAN_POINT('Ctrl Pts',(-7.48686245274063,-0.649958502298315,
29.8764571326107));
#25209=CARTESIAN_POINT('Ctrl Pts',(-7.40871514438587,-0.467474858043207,
29.8844108031865));
#25210=CARTESIAN_POINT('Ctrl Pts',(-7.33056783603113,-0.284991213788141,
29.8923644737623));
#25211=CARTESIAN_POINT('Ctrl Pts',(-7.29666379402431,-0.0836526058012479,
29.9003181443381));
#25212=CARTESIAN_POINT('Ctrl Pts',(-7.31571534807915,0.11259877753163,29.9082718149139));
#25213=CARTESIAN_POINT('Ctrl Pts',(-7.35381845618883,0.505101544197385,
29.9241791560655));
#25214=CARTESIAN_POINT('Ctrl Pts',(-7.60374394854509,0.877255412247096,
29.9400864972171));
#25215=CARTESIAN_POINT('Ctrl Pts',(-7.95379571575922,1.0578303411793,29.9559938383687));
#25216=CARTESIAN_POINT('Ctrl Pts',(-8.2765908013847,1.2243448544765,29.9706625589125));
#25217=CARTESIAN_POINT('Ctrl Pts',(-8.68452661087086,1.22795338154701,29.9853312794563));
#25218=CARTESIAN_POINT('Ctrl Pts',(-9.01356946732952,1.07334645743597,30.));
#25219=CARTESIAN_POINT('Ctrl Pts',(-9.09176790333495,-0.828203493281094,
1.8));
#25220=CARTESIAN_POINT('Ctrl Pts',(-8.83745586871391,-1.007228726393,1.81466872054375));
#25221=CARTESIAN_POINT('Ctrl Pts',(-8.11993078322208,-1.12691245974044,
1.84524478223913));
#25222=CARTESIAN_POINT('Ctrl Pts',(-7.47631525146516,-0.457174338716646,
1.88377451451031));
#25223=CARTESIAN_POINT('Ctrl Pts',(-7.47121748055022,0.241452561832278,
1.91558919681355));
#25224=CARTESIAN_POINT('Ctrl Pts',(-7.78668186971636,0.865450294731047,
1.94740387911679));
#25225=CARTESIAN_POINT('Ctrl Pts',(-8.6897509574811,1.18756791113319,1.98717223199585));
#25226=CARTESIAN_POINT('Ctrl Pts',(-9.42307202460602,0.619626775593939,
2.02554781833935));
#25227=CARTESIAN_POINT('Ctrl Pts',(-9.51573132444702,0.140538355580566,
2.04801606353124));
#25228=CARTESIAN_POINT('Ctrl Pts',(-9.51515984464673,0.000434573109195022,
2.05457696757151));
#25229=CARTESIAN_POINT('Origin',(-8.5,0.,1.24542303242842));
#25230=CARTESIAN_POINT('Ctrl Pts',(-7.9098402978609,-0.827606761448989,
1.8));
#25231=CARTESIAN_POINT('Ctrl Pts',(-7.69350384516205,-0.673338983038085,
1.81248093324819));
#25232=CARTESIAN_POINT('Ctrl Pts',(-7.54189267616637,-0.43110531180156,
1.82496186649638));
#25233=CARTESIAN_POINT('Ctrl Pts',(-7.49768958341452,-0.169101314096706,
1.83744279974457));
#25234=CARTESIAN_POINT('Ctrl Pts',(-7.45348649066266,0.0929026836081468,
1.84992373299276));
#25235=CARTESIAN_POINT('Ctrl Pts',(-7.51723259935484,0.371469608550013,
1.86240466624095));
#25236=CARTESIAN_POINT('Ctrl Pts',(-7.67098159359225,0.588175065318269,
1.87488559948914));
#25237=CARTESIAN_POINT('Ctrl Pts',(-7.82473058782966,0.804880522086524,
1.88736653273733));
#25238=CARTESIAN_POINT('Ctrl Pts',(-8.06660030394209,0.957071646902186,
1.89984746598552));
#25239=CARTESIAN_POINT('Ctrl Pts',(-8.32849763913847,1.00190237340967,1.91232839923372));
#25240=CARTESIAN_POINT('Ctrl Pts',(-8.59039497433485,1.04673309991714,1.92480933248191));
#25241=CARTESIAN_POINT('Ctrl Pts',(-8.86911383512443,0.983654619552456,
1.9372902657301));
#25242=CARTESIAN_POINT('Ctrl Pts',(-9.0861870518979,0.830425292131839,1.94977119897829));
#25243=CARTESIAN_POINT('Ctrl Pts',(-9.30326026867136,0.677195964711223,
1.96225213222648));
#25244=CARTESIAN_POINT('Ctrl Pts',(-9.45603047560713,0.435691592250255,
1.97473306547467));
#25245=CARTESIAN_POINT('Ctrl Pts',(-9.50148857850568,0.173902423064403,
1.98721399872286));
#25246=CARTESIAN_POINT('Ctrl Pts',(-9.51145490317781,0.11650724620064,1.9899503432914));
#25247=CARTESIAN_POINT('Ctrl Pts',(-9.51647499999999,0.0582540466810683,
1.99268668785994));
#25248=CARTESIAN_POINT('Ctrl Pts',(-9.516475,2.33298725921038E-13,1.99542303242848));
#25249=CARTESIAN_POINT('Ctrl Pts',(-7.81012320807277,-0.967444397671095,
1.70084009126668));
#25250=CARTESIAN_POINT('Ctrl Pts',(-7.64896507520752,-0.852523833800245,
1.70879376184249));
#25251=CARTESIAN_POINT('Ctrl Pts',(-7.38788875303855,-0.541081198726736,
1.72470110299411));
#25252=CARTESIAN_POINT('Ctrl Pts',(-7.21568965628902,0.260901981677851,
1.75651578529735));
#25253=CARTESIAN_POINT('Ctrl Pts',(-7.79579643288244,1.21639724974065,1.79628413817641));
#25254=CARTESIAN_POINT('Ctrl Pts',(-9.14633055909857,1.24940928029698,1.84400616163127));
#25255=CARTESIAN_POINT('Ctrl Pts',(-9.77114428998937,0.319024610172379,
1.88377451451032));
#25256=CARTESIAN_POINT('Ctrl Pts',(-9.63552812196199,-0.486329821775173,
1.91558919681356));
#25257=CARTESIAN_POINT('Ctrl Pts',(-9.14596582315122,-1.14084454386822,
1.9474038791168));
#25258=CARTESIAN_POINT('Ctrl Pts',(-8.0410366595526,-1.32880668070371,1.98717223199586));
#25259=CARTESIAN_POINT('Ctrl Pts',(-7.13418129904012,-0.331010374245513,
2.03489425545072));
#25260=CARTESIAN_POINT('Ctrl Pts',(-7.48238663245215,0.969214049802592,
2.08261627890558));
#25261=CARTESIAN_POINT('Ctrl Pts',(-8.7664321344037,1.3804141552358,2.13033830236044));
#25262=CARTESIAN_POINT('Ctrl Pts',(-9.62968786527869,0.665267435601966,
2.17010665523949));
#25263=CARTESIAN_POINT('Ctrl Pts',(-9.72653152013487,-0.146020592972697,
2.20192133754273));
#25264=CARTESIAN_POINT('Ctrl Pts',(-9.44181701552787,-0.911952754888573,
2.23373601984598));
#25265=CARTESIAN_POINT('Ctrl Pts',(-8.4351019567227,-1.40432985445164,2.27350437272503));
#25266=CARTESIAN_POINT('Ctrl Pts',(-7.28284501096867,-0.703261816482742,
2.32122639617989));
#25267=CARTESIAN_POINT('Ctrl Pts',(-7.25086675582171,0.64258304887272,2.36894841963475));
#25268=CARTESIAN_POINT('Ctrl Pts',(-8.36437423211283,1.3991651817553,2.41667044308961));
#25269=CARTESIAN_POINT('Ctrl Pts',(-9.60477848348003,0.869389006667507,
2.46439246654448));
#25270=CARTESIAN_POINT('Ctrl Pts',(-9.78954773216159,-0.235910619659578,
2.50416081942353));
#25271=CARTESIAN_POINT('Ctrl Pts',(-9.33205207893577,-0.912967317898448,
2.53597550172677));
#25272=CARTESIAN_POINT('Ctrl Pts',(-8.61556448948887,-1.30584459467476,
2.56779018403001));
#25273=CARTESIAN_POINT('Ctrl Pts',(-7.53210652875583,-1.01958699917634,
2.60755853690906));
#25274=CARTESIAN_POINT('Ctrl Pts',(-7.11938841334767,0.264524506767542,
2.65528056036393));
#25275=CARTESIAN_POINT('Ctrl Pts',(-7.97576986595538,1.30323198402881,2.70300258381879));
#25276=CARTESIAN_POINT('Ctrl Pts',(-9.31287550026506,1.14686320768969,2.75072460727365));
#25277=CARTESIAN_POINT('Ctrl Pts',(-9.90431611236195,-0.0653566335222347,
2.79844663072851));
#25278=CARTESIAN_POINT('Ctrl Pts',(-9.32087302634031,-1.02213130798339,
2.83821498360756));
#25279=CARTESIAN_POINT('Ctrl Pts',(-8.53190702624905,-1.23482903167169,
2.87002966591081));
#25280=CARTESIAN_POINT('Ctrl Pts',(-7.73300931065141,-1.06316047838934,
2.90184434821405));
#25281=CARTESIAN_POINT('Ctrl Pts',(-7.10093312703504,-0.137793890164714,
2.9416127010931));
#25282=CARTESIAN_POINT('Ctrl Pts',(-7.62898068004556,1.10335267503482,2.98933472454796));
#25283=CARTESIAN_POINT('Ctrl Pts',(-8.95622646325114,1.32856620832035,3.03705674800283));
#25284=CARTESIAN_POINT('Ctrl Pts',(-9.86510821618935,0.335471818616583,
3.08477877145768));
#25285=CARTESIAN_POINT('Ctrl Pts',(-9.51925726078488,-0.968240623257094,
3.13250079491255));
#25286=CARTESIAN_POINT('Ctrl Pts',(-8.45202897306244,-1.31007011342866,
3.1722691477916));
#25287=CARTESIAN_POINT('Ctrl Pts',(-7.71620718099674,-0.954719652751151,
3.20408383009485));
#25288=CARTESIAN_POINT('Ctrl Pts',(-7.22435724578901,-0.302192794555079,
3.23589851239808));
#25289=CARTESIAN_POINT('Ctrl Pts',(-7.35179539345088,0.811172885373114,
3.27566686527714));
#25290=CARTESIAN_POINT('Ctrl Pts',(-8.56318915183267,1.40430371135129,3.32338888873199));
#25291=CARTESIAN_POINT('Ctrl Pts',(-9.7142756519776,0.706233245190208,3.37111091218687));
#25292=CARTESIAN_POINT('Ctrl Pts',(-9.75185976306211,-0.639459862898116,
3.41883293564172));
#25293=CARTESIAN_POINT('Ctrl Pts',(-8.63731725129933,-1.3991137340966,3.46655495909659));
#25294=CARTESIAN_POINT('Ctrl Pts',(-7.60657048260336,-0.959358441316762,
3.50632331197563));
#25295=CARTESIAN_POINT('Ctrl Pts',(-7.28260112740917,-0.209190782474353,
3.53813799427888));
#25296=CARTESIAN_POINT('Ctrl Pts',(-7.33757255373269,0.606091868981768,
3.56995267658212));
#25297=CARTESIAN_POINT('Ctrl Pts',(-8.1623997792252,1.36469826678867,3.60972102946117));
#25298=CARTESIAN_POINT('Ctrl Pts',(-9.46659333225728,1.02066601425937,3.65744305291603));
#25299=CARTESIAN_POINT('Ctrl Pts',(-9.88037352419663,-0.260383734703279,
3.7051650763709));
#25300=CARTESIAN_POINT('Ctrl Pts',(-9.028337989291,-1.30265910801724,3.75288709982575));
#25301=CARTESIAN_POINT('Ctrl Pts',(-7.68843599365213,-1.14792819115296,
3.80060912328062));
#25302=CARTESIAN_POINT('Ctrl Pts',(-7.19665294857957,-0.140965900256968,
3.84037747615968));
#25303=CARTESIAN_POINT('Ctrl Pts',(-7.44246893934906,0.638317205013197,
3.87219215846291));
#25304=CARTESIAN_POINT('Ctrl Pts',(-8.01746352197057,1.21891077148926,3.90400684076616));
#25305=CARTESIAN_POINT('Ctrl Pts',(-9.13758203058977,1.25294230621849,3.9437751936452));
#25306=CARTESIAN_POINT('Ctrl Pts',(-9.89878968243401,0.139460413539292,
3.99149721710008));
#25307=CARTESIAN_POINT('Ctrl Pts',(-9.37354847053911,-1.10006537315735,
4.03921924055493));
#25308=CARTESIAN_POINT('Ctrl Pts',(-8.04725495447656,-1.33082068904202,
4.0869412640098));
#25309=CARTESIAN_POINT('Ctrl Pts',(-7.13518679943722,-0.337135278505145,
4.13466328746465));
#25310=CARTESIAN_POINT('Ctrl Pts',(-7.42210844649126,0.746146581012124,
4.17443164034372));
#25311=CARTESIAN_POINT('Ctrl Pts',(-8.11787612020756,1.17464979417261,4.20624632264694));
#25312=CARTESIAN_POINT('Ctrl Pts',(-8.93258781868444,1.23751876777989,4.2380610049502));
#25313=CARTESIAN_POINT('Ctrl Pts',(-9.80194727627518,0.530385292257153,
4.27782935782925));
#25314=CARTESIAN_POINT('Ctrl Pts',(-9.64908535189861,-0.809731212613409,
4.3255513812841));
#25315=CARTESIAN_POINT('Ctrl Pts',(-8.44087433879924,-1.40347244781957,
4.37327340473898));
#25316=CARTESIAN_POINT('Ctrl Pts',(-7.28688212263863,-0.710216022245734,
4.42099542819382));
#25317=CARTESIAN_POINT('Ctrl Pts',(-7.24727497666278,0.638008843471503,
4.4687174516487));
#25318=CARTESIAN_POINT('Ctrl Pts',(-8.17302891837419,1.26951755925708,4.50848580452774));
#25319=CARTESIAN_POINT('Ctrl Pts',(-8.97956615474956,1.13834840961636,4.54030048683099));
#25320=CARTESIAN_POINT('Ctrl Pts',(-9.63682842664003,0.652844583239195,
4.57211516913422));
#25321=CARTESIAN_POINT('Ctrl Pts',(-9.83162187111272,-0.450731029348286,
4.61188352201329));
#25322=CARTESIAN_POINT('Ctrl Pts',(-8.83920954348061,-1.364184250107,4.65960554546813));
#25323=CARTESIAN_POINT('Ctrl Pts',(-7.53702357423647,-1.02269602474283,
4.70732756892301));
#25324=CARTESIAN_POINT('Ctrl Pts',(-7.11789619960128,0.256614238793786,
4.75504959237787));
#25325=CARTESIAN_POINT('Ctrl Pts',(-7.97005828331786,1.30212789132369,4.80277161583273));
#25326=CARTESIAN_POINT('Ctrl Pts',(-9.08334562110853,1.17400715833213,4.84253996871178));
#25327=CARTESIAN_POINT('Ctrl Pts',(-9.60747087368845,0.547109735235215,
4.87435465101502));
#25328=CARTESIAN_POINT('Ctrl Pts',(-9.78687272637736,-0.250087000037372,
4.90616933331827));
#25329=CARTESIAN_POINT('Ctrl Pts',(-9.21213964719043,-1.21211896748734,
4.94593768619731));
#25330=CARTESIAN_POINT('Ctrl Pts',(-7.86397133533361,-1.25360652533042,
4.99365970965218));
#25331=CARTESIAN_POINT('Ctrl Pts',(-7.10261742202974,-0.143362081410263,
5.04138173310704));
#25332=CARTESIAN_POINT('Ctrl Pts',(-7.62267670059613,1.09834676261708,5.0891037565619));
#25333=CARTESIAN_POINT('Ctrl Pts',(-8.95118465747005,1.33146823969133,5.13682578001676));
#25334=CARTESIAN_POINT('Ctrl Pts',(-9.70928520759754,0.506176064395958,
5.17659413289582));
#25335=CARTESIAN_POINT('Ctrl Pts',(-9.69549089650709,-0.310841301673474,
5.20840881519905));
#25336=CARTESIAN_POINT('Ctrl Pts',(-9.30957511823071,-1.03110283164355,
5.2402234975023));
#25337=CARTESIAN_POINT('Ctrl Pts',(-8.24549407463932,-1.38260695875559,
5.27999185038136));
#25338=CARTESIAN_POINT('Ctrl Pts',(-7.1987928772941,-0.531903944756733,
5.32771387383621));
#25339=CARTESIAN_POINT('Ctrl Pts',(-7.34942599645375,0.805859924530717,
5.37543589729107));
#25340=CARTESIAN_POINT('Ctrl Pts',(-8.55514648367598,1.40464253387348,5.42315792074594));
#25341=CARTESIAN_POINT('Ctrl Pts',(-9.71236150745908,0.711726663596795,
5.47087994420079));
#25342=CARTESIAN_POINT('Ctrl Pts',(-9.74570628634277,-0.408412499377414,
5.51064829707986));
#25343=CARTESIAN_POINT('Ctrl Pts',(-9.20071704662944,-1.01725926833835,
5.54246297938309));
#25344=CARTESIAN_POINT('Ctrl Pts',(-8.43761501639986,-1.30946288046008,
5.57427766168634));
#25345=CARTESIAN_POINT('Ctrl Pts',(-7.40291845050727,-0.879083239634173,
5.61404601456539));
#25346=CARTESIAN_POINT('Ctrl Pts',(-7.16794425015288,0.44909827646911,5.66176803802024));
#25347=CARTESIAN_POINT('Ctrl Pts',(-8.15713175655234,1.36223056904336,5.70949006147512));
#25348=CARTESIAN_POINT('Ctrl Pts',(-9.46073272219602,1.02618439821026,5.75721208492997));
#25349=CARTESIAN_POINT('Ctrl Pts',(-9.88252017395179,-0.254976934367327,
5.80493410838483));
#25350=CARTESIAN_POINT('Ctrl Pts',(-9.17485382333125,-1.12390268200446,
5.84470246126389));
#25351=CARTESIAN_POINT('Ctrl Pts',(-8.36434829003804,-1.22777009738866,
5.87651714356712));
#25352=CARTESIAN_POINT('Ctrl Pts',(-7.59606717977041,-0.949468471300325,
5.90833182587037));
#25353=CARTESIAN_POINT('Ctrl Pts',(-7.09516279594638,0.0529877207466158,
5.94810017874943));
#25354=CARTESIAN_POINT('Ctrl Pts',(-7.78646395477307,1.21116807041393,5.99582220220428));
#25355=CARTESIAN_POINT('Ctrl Pts',(-9.13198350831614,1.25452285782982,6.04354422565915));
#25356=CARTESIAN_POINT('Ctrl Pts',(-9.89796813894857,0.147468183392425,
6.09126624911401));
#25357=CARTESIAN_POINT('Ctrl Pts',(-9.37870943707034,-1.09738097014965,
6.13898827256887));
#25358=CARTESIAN_POINT('Ctrl Pts',(-8.2750146032041,-1.29149777108216,6.17875662544793));
#25359=CARTESIAN_POINT('Ctrl Pts',(-7.59410884117921,-0.839751157681671,
6.21057130775117));
#25360=CARTESIAN_POINT('Ctrl Pts',(-7.19518058991253,-0.12661448787792,
6.2423859900544));
#25361=CARTESIAN_POINT('Ctrl Pts',(-7.47225594872512,0.959227519159126,
6.28215434293346));
#25362=CARTESIAN_POINT('Ctrl Pts',(-8.75282774279127,1.38280147349625,6.32987636638832));
#25363=CARTESIAN_POINT('Ctrl Pts',(-9.79874749682902,0.535243584811133,
6.37759838984319));
#25364=CARTESIAN_POINT('Ctrl Pts',(-9.65370337198217,-0.803137791481188,
6.42532041329804));
#25365=CARTESIAN_POINT('Ctrl Pts',(-8.44653368519695,-1.40481907077903,
6.47304243675291));
#25366=CARTESIAN_POINT('Ctrl Pts',(-7.48485426986889,-0.82949627369758,
6.51281078963196));
#25367=CARTESIAN_POINT('Ctrl Pts',(-7.26548531614969,-0.0423591054596432,
6.5446254719352));
#25368=CARTESIAN_POINT('Ctrl Pts',(-7.43038479706196,0.757963217528006,
6.57644015423845));
#25369=CARTESIAN_POINT('Ctrl Pts',(-8.35036750116968,1.39785027228845,6.61620850711748));
#25370=CARTESIAN_POINT('Ctrl Pts',(-9.59593968524807,0.880328341544614,
6.66393053057237));
#25371=CARTESIAN_POINT('Ctrl Pts',(-9.83238070572399,-0.444963381207409,
6.7116525540272));
#25372=CARTESIAN_POINT('Ctrl Pts',(-8.84701587301111,-1.3622194267102,6.75937457748209));
#25373=CARTESIAN_POINT('Ctrl Pts',(-7.54042240671594,-1.02741720391975,
6.80709660093693));
#25374=CARTESIAN_POINT('Ctrl Pts',(-7.1895707383084,0.0368791483633014,
6.846864953816));
#25375=CARTESIAN_POINT('Ctrl Pts',(-7.53867950098618,0.775682729363746,
6.87867963611924));
#25376=CARTESIAN_POINT('Ctrl Pts',(-8.18701931224334,1.27303888808354,6.91049431842248));
#25377=CARTESIAN_POINT('Ctrl Pts',(-9.30142390307262,1.1550303009129,6.95026267130153));
#25378=CARTESIAN_POINT('Ctrl Pts',(-9.90478830936975,-0.0512990105789078,
6.9979846947564));
#25379=CARTESIAN_POINT('Ctrl Pts',(-9.21648716902564,-1.20825365392484,
7.04570671821125));
#25380=CARTESIAN_POINT('Ctrl Pts',(-7.87116044050737,-1.25722813802644,
7.09342874166612));
#25381=CARTESIAN_POINT('Ctrl Pts',(-7.10209883232916,-0.149156273309624,
7.14115076512098));
#25382=CARTESIAN_POINT('Ctrl Pts',(-7.53311276915676,0.885276230514455,
7.18091911800003));
#25383=CARTESIAN_POINT('Ctrl Pts',(-8.28051104488537,1.21558438499352,7.21273380030327));
#25384=CARTESIAN_POINT('Ctrl Pts',(-9.09622983417627,1.16751655505169,7.24454848260651));
#25385=CARTESIAN_POINT('Ctrl Pts',(-9.86179147454805,0.349140728491166,
7.28431683548556));
#25386=CARTESIAN_POINT('Ctrl Pts',(-9.52881196198549,-0.957918435726067,
7.33203885894043));
#25387=CARTESIAN_POINT('Ctrl Pts',(-8.25131089567602,-1.38252829446331,
7.37976088239529));
#25388=CARTESIAN_POINT('Ctrl Pts',(-7.20186011708233,-0.539346481407665,
7.42748290585015));
#25389=CARTESIAN_POINT('Ctrl Pts',(-7.34524279360816,0.801817349980164,
7.47520492930502));
#25390=CARTESIAN_POINT('Ctrl Pts',(-8.34800590386557,1.30210702948025,7.51497328218407));
#25391=CARTESIAN_POINT('Ctrl Pts',(-9.12934199675921,1.06289672573233,7.54678796448731));
#25392=CARTESIAN_POINT('Ctrl Pts',(-9.71478227155839,0.492837655003186,
7.57860264679055));
#25393=CARTESIAN_POINT('Ctrl Pts',(-9.75829474594768,-0.626952630398444,
7.61837099966961));
#25394=CARTESIAN_POINT('Ctrl Pts',(-8.65129661555606,-1.39755898506989,
7.66609302312447));
#25395=CARTESIAN_POINT('Ctrl Pts',(-7.40736890912006,-0.882829572932191,
7.71381504657932));
#25396=CARTESIAN_POINT('Ctrl Pts',(-7.16539436552863,0.441463003054117,
7.76153707003419));
#25397=CARTESIAN_POINT('Ctrl Pts',(-8.15132322416797,1.36191034008795,7.80925909348904));
#25398=CARTESIAN_POINT('Ctrl Pts',(-9.23699515103494,1.08416929897162,7.84902744636811));
#25399=CARTESIAN_POINT('Ctrl Pts',(-9.67137290472358,0.392053971459019,
7.88084212867133));
#25400=CARTESIAN_POINT('Ctrl Pts',(-9.74113641902229,-0.422096328884964,
7.9126568109746));
#25401=CARTESIAN_POINT('Ctrl Pts',(-9.04138768513413,-1.2974107456115,7.95242516385363));
#25402=CARTESIAN_POINT('Ctrl Pts',(-7.70002517381599,-1.15589881049344,
8.0001471873085));
#25403=CARTESIAN_POINT('Ctrl Pts',(-7.09607732311738,0.0472427024613963,
8.04786921076337));
#25404=CARTESIAN_POINT('Ctrl Pts',(-7.77953999755666,1.2070622053182,8.09559123421822));
#25405=CARTESIAN_POINT('Ctrl Pts',(-9.12738126735548,1.25808108395864,8.1433132576731));
#25406=CARTESIAN_POINT('Ctrl Pts',(-9.76670415651867,0.337706235269572,
8.18308161055213));
#25407=CARTESIAN_POINT('Ctrl Pts',(-9.64236730081661,-0.469912490238714,
8.21489629285539));
#25408=CARTESIAN_POINT('Ctrl Pts',(-9.16244480469929,-1.13126115561727,
8.24671097515861));
#25409=CARTESIAN_POINT('Ctrl Pts',(-8.06055772321674,-1.33538973854775,
8.28647932803768));
#25410=CARTESIAN_POINT('Ctrl Pts',(-7.13873614714364,-0.350745642218132,
8.33420135149253));
#25411=CARTESIAN_POINT('Ctrl Pts',(-7.46918871853192,0.954284474147625,
8.3819233749474));
#25412=CARTESIAN_POINT('Ctrl Pts',(-8.74490509614319,1.38422659868658,8.42964539840227));
#25413=CARTESIAN_POINT('Ctrl Pts',(-9.79759510919648,0.540945654416837,
8.47736742185711));
#25414=CARTESIAN_POINT('Ctrl Pts',(-9.67890329798344,-0.57338637539219,
8.51713577473619));
#25415=CARTESIAN_POINT('Ctrl Pts',(-9.05646522431439,-1.10279973367158,
8.54895045703941));
#25416=CARTESIAN_POINT('Ctrl Pts',(-8.26081574743447,-1.28894368178221,
8.58076513934267));
#25417=CARTESIAN_POINT('Ctrl Pts',(-7.29395295285977,-0.722375102372306,
8.6205334922217));
#25418=CARTESIAN_POINT('Ctrl Pts',(-7.24105420847638,0.625393697308591,
8.66825551567658));
#25419=CARTESIAN_POINT('Ctrl Pts',(-8.34481376796175,1.39611890216659,8.71597753913143));
#25420=CARTESIAN_POINT('Ctrl Pts',(-9.59088058679426,0.886589717955089,
8.7636995625863));
#25421=CARTESIAN_POINT('Ctrl Pts',(-9.83523995273739,-0.439897189189682,
8.81142158604116));
#25422=CARTESIAN_POINT('Ctrl Pts',(-9.0163949108726,-1.20495693595518,8.85118993892021));
#25423=CARTESIAN_POINT('Ctrl Pts',(-8.19929004648907,-1.19807943072103,
8.88300462122345));
#25424=CARTESIAN_POINT('Ctrl Pts',(-7.47578742485353,-0.818274723056666,
8.91481930352669));
#25425=CARTESIAN_POINT('Ctrl Pts',(-7.11528810852852,0.242792598858646,
8.95458765640575));
#25426=CARTESIAN_POINT('Ctrl Pts',(-7.9570999824169,1.29665776268705,9.0023096798606));
#25427=CARTESIAN_POINT('Ctrl Pts',(-9.29609107490602,1.15735463711695,9.05003170331547));
#25428=CARTESIAN_POINT('Ctrl Pts',(-9.90505903600862,-0.0432537623661014,
9.09775372677034));
#25429=CARTESIAN_POINT('Ctrl Pts',(-9.2219641867544,-1.20629307445875,9.14547575022517));
#25430=CARTESIAN_POINT('Ctrl Pts',(-8.10214743413141,-1.24911899245564,
9.18524410310427));
#25431=CARTESIAN_POINT('Ctrl Pts',(-7.48870897396143,-0.709303361835556,
9.21705878540747));
#25432=CARTESIAN_POINT('Ctrl Pts',(-7.19005593077866,0.0512977289309366,
9.24887346771074));
#25433=CARTESIAN_POINT('Ctrl Pts',(-7.61166111530691,1.08960052055114,9.28864182058977));
#25434=CARTESIAN_POINT('Ctrl Pts',(-8.93780590948666,1.33580977996377,9.33636384404464));
#25435=CARTESIAN_POINT('Ctrl Pts',(-9.85927926973828,0.354387672557732,
9.38408586749951));
#25436=CARTESIAN_POINT('Ctrl Pts',(-9.53428053627848,-0.952011320785507,
9.43180789095435));
#25437=CARTESIAN_POINT('Ctrl Pts',(-8.25673567435074,-1.38462909701822,
9.47952991440924));
#25438=CARTESIAN_POINT('Ctrl Pts',(-7.38185044108033,-0.684343835633376,
9.51929826728827));
#25439=CARTESIAN_POINT('Ctrl Pts',(-7.27112556056279,0.125253385404266,
9.55111294959153));
#25440=CARTESIAN_POINT('Ctrl Pts',(-7.54291347100558,0.89586287873705,9.58292763189476));
#25441=CARTESIAN_POINT('Ctrl Pts',(-8.54109342884341,1.40523542459937,9.62269598477382));
#25442=CARTESIAN_POINT('Ctrl Pts',(-9.70508436318578,0.723763400728029,
9.67041800822868));
#25443=CARTESIAN_POINT('Ctrl Pts',(-9.75982784765577,-0.621340928856411,
9.71814003168354));
#25444=CARTESIAN_POINT('Ctrl Pts',(-8.65929714385257,-1.39666968270552,
9.7658620551384));
#25445=CARTESIAN_POINT('Ctrl Pts',(-7.41009690516316,-0.887967630214163,
9.81358407859327));
#25446=CARTESIAN_POINT('Ctrl Pts',(-7.20664393228174,0.214044396277857,
9.85335243147231));
#25447=CARTESIAN_POINT('Ctrl Pts',(-7.65261027533608,0.898749939077259,
9.88516711377557));
#25448=CARTESIAN_POINT('Ctrl Pts',(-8.36234433802887,1.30370082465606,9.91698179607878));
#25449=CARTESIAN_POINT('Ctrl Pts',(-9.4504929687235,1.03582739143657,9.95675014895787));
#25450=CARTESIAN_POINT('Ctrl Pts',(-9.88489219289376,-0.24111282979186,
10.0044721724127));
#25451=CARTESIAN_POINT('Ctrl Pts',(-9.04621871645882,-1.294169953828,10.0521941958676));
#25452=CARTESIAN_POINT('Ctrl Pts',(-7.70665745170364,-1.16046084970194,
10.0999162193224));
#25453=CARTESIAN_POINT('Ctrl Pts',(-7.09477865657472,0.0415721592550427,
10.1476382427773));
#25454=CARTESIAN_POINT('Ctrl Pts',(-7.6619399172144,1.00808740648965,10.1874065956564));
#25455=CARTESIAN_POINT('Ctrl Pts',(-8.44719185329995,1.23411186612052,10.2192212779596));
#25456=CARTESIAN_POINT('Ctrl Pts',(-9.24888142608082,1.07599327653697,10.2510359602628));
#25457=CARTESIAN_POINT('Ctrl Pts',(-9.89653349865093,0.161460383961197,
10.2908043131419));
#25458=CARTESIAN_POINT('Ctrl Pts',(-9.38957427574612,-1.08844815703784,
10.3385263365968));
#25459=CARTESIAN_POINT('Ctrl Pts',(-8.06633158847052,-1.33609972099488,
10.3862483600516));
#25460=CARTESIAN_POINT('Ctrl Pts',(-7.1407669831977,-0.358535059182231,
10.4339703835065));
#25461=CARTESIAN_POINT('Ctrl Pts',(-7.46449648071845,0.950845797171473,
10.4816924069613));
#25462=CARTESIAN_POINT('Ctrl Pts',(-8.52578462688086,1.31069450082703,10.5214607598404));
#25463=CARTESIAN_POINT('Ctrl Pts',(-9.26751705207691,0.967852454265898,
10.5532754421436));
#25464=CARTESIAN_POINT('Ctrl Pts',(-9.77034379229997,0.32374615186375,10.5850901244469));
#25465=CARTESIAN_POINT('Ctrl Pts',(-9.66177322247695,-0.791617488423889,
10.6248584773259));
#25466=CARTESIAN_POINT('Ctrl Pts',(-8.46059480690637,-1.40517223619938,
10.6725805007808));
#25467=CARTESIAN_POINT('Ctrl Pts',(-7.29785493107611,-0.726689747322139,
10.7203025242356));
#25468=CARTESIAN_POINT('Ctrl Pts',(-7.23749358360742,0.61817419162873,10.7680245476905));
#25469=CARTESIAN_POINT('Ctrl Pts',(-8.33901539365003,1.39658842360999,10.8157465711454));
#25470=CARTESIAN_POINT('Ctrl Pts',(-9.37705950218062,0.974346730438539,
10.8555149240244));
#25471=CARTESIAN_POINT('Ctrl Pts',(-9.71368278510872,0.229771398542418,
10.8873296063277));
#25472=CARTESIAN_POINT('Ctrl Pts',(-9.67252199622786,-0.586325071818906,
10.9191442886309));
#25473=CARTESIAN_POINT('Ctrl Pts',(-8.86065621577464,-1.35878709239755,
10.95891264151));
#25474=CARTESIAN_POINT('Ctrl Pts',(-7.55082510800669,-1.03688418207522,
11.0066346649648));
#25475=CARTESIAN_POINT('Ctrl Pts',(-7.11541601124033,0.236976652165245,
11.0543566884197));
#25476=CARTESIAN_POINT('Ctrl Pts',(-7.94968367760215,1.29352762936508,11.1020787118745));
#25477=CARTESIAN_POINT('Ctrl Pts',(-9.29201323306557,1.16150346839435,11.1498007353294));
#25478=CARTESIAN_POINT('Ctrl Pts',(-9.80077369478986,0.163011399676013,
11.1895690882084));
#25479=CARTESIAN_POINT('Ctrl Pts',(-9.5681862205647,-0.620321688040218,
11.2213837705117));
#25480=CARTESIAN_POINT('Ctrl Pts',(-9.00310351380729,-1.21056671682165,
11.2531984528149));
#25481=CARTESIAN_POINT('Ctrl Pts',(-7.88372169902902,-1.26355701264146,
11.292966805694));
#25482=CARTESIAN_POINT('Ctrl Pts',(-7.10377186540718,-0.163121975220387,
11.3406888291489));
#25483=CARTESIAN_POINT('Ctrl Pts',(-7.60795259079157,1.08511850750303,11.3884108526037));
#25484=CARTESIAN_POINT('Ctrl Pts',(-8.93014932407102,1.33829493820665,11.4361328760586));
#25485=CARTESIAN_POINT('Ctrl Pts',(-9.85890988118501,0.360193285974161,
11.4838548995135));
#25486=CARTESIAN_POINT('Ctrl Pts',(-9.59036934973144,-0.727790905856776,
11.5236232523925));
#25487=CARTESIAN_POINT('Ctrl Pts',(-8.90195596740575,-1.16801207130932,
11.5554379346957));
#25488=CARTESIAN_POINT('Ctrl Pts',(-8.08842540955644,-1.24466512684449,
11.587252616999));
#25489=CARTESIAN_POINT('Ctrl Pts',(-7.20721876125312,-0.55235128060609,
11.627020969878));
#25490=CARTESIAN_POINT('Ctrl Pts',(-7.33737056595869,0.790161111248255,
11.6747429933329));
#25491=CARTESIAN_POINT('Ctrl Pts',(-8.53535635817352,1.40427229679212,11.7224650167878));
#25492=CARTESIAN_POINT('Ctrl Pts',(-9.70092003171144,0.730652352396493,
11.7701870402426));
#25493=CARTESIAN_POINT('Ctrl Pts',(-9.76334698685623,-0.616708731285964,
11.8179090636975));
#25494=CARTESIAN_POINT('Ctrl Pts',(-8.84841718790923,-1.26379997810216,
11.8576774165765));
#25495=CARTESIAN_POINT('Ctrl Pts',(-8.03977484955831,-1.14630432667695,
11.8894920988798));
#25496=CARTESIAN_POINT('Ctrl Pts',(-7.37438718484698,-0.671997553451563,
11.921306781183));
#25497=CARTESIAN_POINT('Ctrl Pts',(-7.16093809190246,0.428122032515589,
11.9610751340621));
#25498=CARTESIAN_POINT('Ctrl Pts',(-8.13774339449002,1.35824590350669,12.0087971575169));
#25499=CARTESIAN_POINT('Ctrl Pts',(-9.44552413575031,1.03885266727997,12.0565191809718));
#25500=CARTESIAN_POINT('Ctrl Pts',(-9.88625019929875,-0.233178402886088,
12.1042412044267));
#25501=CARTESIAN_POINT('Ctrl Pts',(-9.05191082642372,-1.29296933765629,
12.1519632278815));
#25502=CARTESIAN_POINT('Ctrl Pts',(-7.93661396084778,-1.18371495401975,
12.1917315807606));
#25503=CARTESIAN_POINT('Ctrl Pts',(-7.40195043615906,-0.565780835488536,
12.2235462630638));
#25504=CARTESIAN_POINT('Ctrl Pts',(-7.20907773223965,0.228264364459372,
12.2553609453671));
#25505=CARTESIAN_POINT('Ctrl Pts',(-7.76744120993183,1.19988869797868,12.2951292982461));
#25506=CARTESIAN_POINT('Ctrl Pts',(-9.11471391243231,1.26419483802557,12.3428513217009));
#25507=CARTESIAN_POINT('Ctrl Pts',(-9.89475517645041,0.166999261572729,
12.3905733451558));
#25508=CARTESIAN_POINT('Ctrl Pts',(-9.39579260092668,-1.08333623531818,
12.4382953686107));
#25509=CARTESIAN_POINT('Ctrl Pts',(-8.07142180339368,-1.33891597863226,
12.4860173920655));
#25510=CARTESIAN_POINT('Ctrl Pts',(-7.29945768638114,-0.526576750998625,
12.5257857449446));
#25511=CARTESIAN_POINT('Ctrl Pts',(-7.29941789289706,0.290557055604651,
12.5576004272478));
#25512=CARTESIAN_POINT('Ctrl Pts',(-7.67308431204718,1.0172489206183,12.5894151095511));
#25513=CARTESIAN_POINT('Ctrl Pts',(-8.73106187313777,1.38671759173422,12.6291834624301));
#25514=CARTESIAN_POINT('Ctrl Pts',(-9.79201548042824,0.553857184626279,
12.676905485885));
#25515=CARTESIAN_POINT('Ctrl Pts',(-9.66405233131191,-0.786265175095756,
12.7246275093399));
#25516=CARTESIAN_POINT('Ctrl Pts',(-8.46864205863334,-1.40537484755547,
12.7723495327947));
#25517=CARTESIAN_POINT('Ctrl Pts',(-7.29986180498706,-0.732149971873374,
12.8200715562496));
#25518=CARTESIAN_POINT('Ctrl Pts',(-7.24755781690594,0.387264121095883,
12.8598399091287));
#25519=CARTESIAN_POINT('Ctrl Pts',(-7.78216115368569,1.00525031170328,12.8916545914319));
#25520=CARTESIAN_POINT('Ctrl Pts',(-8.54020679811835,1.31033138360747,12.9234692737351));
#25521=CARTESIAN_POINT('Ctrl Pts',(-9.58204140768946,0.897530868822055,
12.9632376266142));
#25522=CARTESIAN_POINT('Ctrl Pts',(-9.8394680820938,-0.426482168068336,
13.010959650069));
#25523=CARTESIAN_POINT('Ctrl Pts',(-8.86588170522376,-1.35623056055511,
13.0586816735239));
#25524=CARTESIAN_POINT('Ctrl Pts',(-7.55677830450565,-1.04230255481654,
13.1064036969788));
#25525=CARTESIAN_POINT('Ctrl Pts',(-7.11336120643524,0.231534283907112,
13.1541257204336));
#25526=CARTESIAN_POINT('Ctrl Pts',(-7.80621519412012,1.11231630600824,13.1938940733127));
#25527=CARTESIAN_POINT('Ctrl Pts',(-8.61484608482721,1.22989071679448,13.2257087556159));
#25528=CARTESIAN_POINT('Ctrl Pts',(-9.38772873712336,0.964635999103795,
13.2575234379192));
#25529=CARTESIAN_POINT('Ctrl Pts',(-9.9055329419163,-0.0291961920663647,
13.2972917907982));
#25530=CARTESIAN_POINT('Ctrl Pts',(-9.23393888925362,-1.19891429613191,
13.345013814253));
#25531=CARTESIAN_POINT('Ctrl Pts',(-7.88934617768876,-1.26504255457979,
13.392735837708));
#25532=CARTESIAN_POINT('Ctrl Pts',(-7.10472886292055,-0.171114688619423,
13.4404578611628));
#25533=CARTESIAN_POINT('Ctrl Pts',(-7.6028378109668,1.08234711392059,13.4881798846177));
#25534=CARTESIAN_POINT('Ctrl Pts',(-8.70308805672016,1.29512167872337,13.5279482374967));
#25535=CARTESIAN_POINT('Ctrl Pts',(-9.39154431231752,0.85496756525127,13.5597629198));
#25536=CARTESIAN_POINT('Ctrl Pts',(-9.80248881225848,0.148686971262036,
13.5915776021032));
#25537=CARTESIAN_POINT('Ctrl Pts',(-9.54383650121592,-0.941690303216714,
13.6313459549822));
#25538=CARTESIAN_POINT('Ctrl Pts',(-8.27061936204929,-1.38688366691718,
13.6790679784371));
#25539=CARTESIAN_POINT('Ctrl Pts',(-7.21050033312947,-0.557154704495852,
13.726790001892));
#25540=CARTESIAN_POINT('Ctrl Pts',(-7.33286483455415,0.783490451893329,
13.7745120253468));
#25541=CARTESIAN_POINT('Ctrl Pts',(-8.52967502452601,1.4055229138518,13.8222340488017));
#25542=CARTESIAN_POINT('Ctrl Pts',(-9.50095684039326,0.846563834067789,
13.8620024016807));
#25543=CARTESIAN_POINT('Ctrl Pts',(-9.73362060837031,0.0632534035562258,
13.893817083984));
#25544=CARTESIAN_POINT('Ctrl Pts',(-9.58229424135026,-0.739745967627832,
13.9256317662872));
#25545=CARTESIAN_POINT('Ctrl Pts',(-8.67327669837474,-1.39511664538971,
13.9654001191663));
#25546=CARTESIAN_POINT('Ctrl Pts',(-7.41912137251077,-0.898756460486,14.0131221426211));
#25547=CARTESIAN_POINT('Ctrl Pts',(-7.16027701249887,0.422342363920669,
14.060844166076));
#25548=CARTESIAN_POINT('Ctrl Pts',(-8.12997144830433,1.35614920033099,14.1085661895309));
#25549=CARTESIAN_POINT('Ctrl Pts',(-9.44204586070303,1.04351562747063,14.1562882129857));
#25550=CARTESIAN_POINT('Ctrl Pts',(-9.81086581180923,-0.0146882575975216,
14.1960565658648));
#25551=CARTESIAN_POINT('Ctrl Pts',(-9.474315050416,-0.759296372301599,14.227871248168));
#25552=CARTESIAN_POINT('Ctrl Pts',(-8.83448841538654,-1.26755766001138,
14.2596859304713));
#25553=CARTESIAN_POINT('Ctrl Pts',(-7.71824565582048,-1.16843288801694,
14.2994542833503));
#25554=CARTESIAN_POINT('Ctrl Pts',(-7.09454453567121,0.0275085517186915,
14.3471763068052));
#25555=CARTESIAN_POINT('Ctrl Pts',(-7.76315975106791,1.19595033473491,14.3948983302601));
#25556=CARTESIAN_POINT('Ctrl Pts',(-9.10746452361569,1.26769421990389,14.4426203537149));
#25557=CARTESIAN_POINT('Ctrl Pts',(-9.89517559599181,0.172801402766538,
14.4903423771698));
#25558=CARTESIAN_POINT('Ctrl Pts',(-9.48173640552899,-0.868779921226412,
14.5301107300488));
#25559=CARTESIAN_POINT('Ctrl Pts',(-8.740037375894,-1.21169420921505,14.561925412352));
#25560=CARTESIAN_POINT('Ctrl Pts',(-7.92362170827253,-1.17744341108029,
14.5937400946553));
#25561=CARTESIAN_POINT('Ctrl Pts',(-7.14431466438971,-0.372145857416179,
14.6335084475344));
#25562=CARTESIAN_POINT('Ctrl Pts',(-7.4551179039004,0.940363327686876,14.6812304709892));
#25563=CARTESIAN_POINT('Ctrl Pts',(-8.72524721766598,1.38654045969507,14.7289524944441));
#25564=CARTESIAN_POINT('Ctrl Pts',(-9.78882267771499,0.561246726270562,
14.7766745178989));
#25565=CARTESIAN_POINT('Ctrl Pts',(-9.66816649404496,-0.782152358472022,
14.8243965413538));
#25566=CARTESIAN_POINT('Ctrl Pts',(-8.67401702075417,-1.29934714241638,
14.8641648942329));
#25567=CARTESIAN_POINT('Ctrl Pts',(-7.88874307551789,-1.07339916673311,
14.8959795765361));
#25568=CARTESIAN_POINT('Ctrl Pts',(-7.2937355886856,-0.513333317189202,
14.9277942588393));
#25569=CARTESIAN_POINT('Ctrl Pts',(-7.23127127492183,0.605559803923401,
14.9675626117184));
#25570=CARTESIAN_POINT('Ctrl Pts',(-8.32506434800626,1.39479723197527,15.0152846351733));
#25571=CARTESIAN_POINT('Ctrl Pts',(-9.577528174018,0.901201308551766,15.0630066586281));
#25572=CARTESIAN_POINT('Ctrl Pts',(-9.84188831197631,-0.418804799962236,
15.110728682083));
#25573=CARTESIAN_POINT('Ctrl Pts',(-8.87168403101893,-1.35581207733519,
15.1584507055378));
#25574=CARTESIAN_POINT('Ctrl Pts',(-7.78146541211255,-1.09649119427727,
15.1982190584169));
#25575=CARTESIAN_POINT('Ctrl Pts',(-7.33543257577158,-0.411829247736474,
15.2300337407201));
#25576=CARTESIAN_POINT('Ctrl Pts',(-7.25189509248559,0.401023575788254,
15.2618484230234));
#25577=CARTESIAN_POINT('Ctrl Pts',(-7.93672527856798,1.28805862362876,15.3016167759024));
#25578=CARTESIAN_POINT('Ctrl Pts',(-9.2802898119901,1.1692775185069,15.3493387993573));
#25579=CARTESIAN_POINT('Ctrl Pts',(-9.90452303617752,-0.023468903252238,
15.3970608228122));
#25580=CARTESIAN_POINT('Ctrl Pts',(-9.24078902202083,-1.19468910281144,
15.444782846267));
#25581=CARTESIAN_POINT('Ctrl Pts',(-7.89401458685209,-1.26852769992676,
15.4925048697219));
#25582=CARTESIAN_POINT('Ctrl Pts',(-7.23918325907841,-0.359093832643389,
15.5322732226009));
#25583=CARTESIAN_POINT('Ctrl Pts',(-7.34985615927118,0.450492361508205,
15.5640879049042));
#25584=CARTESIAN_POINT('Ctrl Pts',(-7.81846044934637,1.11991416460057,15.5959025872074));
#25585=CARTESIAN_POINT('Ctrl Pts',(-8.91685053280032,1.3425736633541,15.6356709400865));
#25586=CARTESIAN_POINT('Ctrl Pts',(-9.85499739493844,0.373849720226626,
15.6833929635413));
#25587=CARTESIAN_POINT('Ctrl Pts',(-9.54706276738189,-0.936893375628721,
15.7311149869962));
#25588=CARTESIAN_POINT('Ctrl Pts',(-8.27810821927371,-1.38780367521502,
15.7788370104511));
#25589=CARTESIAN_POINT('Ctrl Pts',(-7.21262708385088,-0.563549955867792,
15.8265590339059));
#25590=CARTESIAN_POINT('Ctrl Pts',(-7.32972690286773,0.778060702080066,
15.8742810573608));
#25591=CARTESIAN_POINT('Ctrl Pts',(-8.52189522723517,1.40525997677246,15.9220030808156));
#25592=CARTESIAN_POINT('Ctrl Pts',(-9.69354285869501,0.741326568114595,
15.9697251042705));
#25593=CARTESIAN_POINT('Ctrl Pts',(-9.76973983670298,-0.602944691238737,
16.0174471277254));
#25594=CARTESIAN_POINT('Ctrl Pts',(-8.67795139285792,-1.39448976690683,
16.0651691511802));
#25595=CARTESIAN_POINT('Ctrl Pts',(-7.63474546540348,-0.984905318057682,
16.1049375040593));
#25596=CARTESIAN_POINT('Ctrl Pts',(-7.28920191986363,-0.244422239744572,
16.1367521863625));
#25597=CARTESIAN_POINT('Ctrl Pts',(-7.32046026829885,0.572095495672729,
16.1685668686657));
#25598=CARTESIAN_POINT('Ctrl Pts',(-8.1229455399191,1.35433038087558,16.2083352215448));
#25599=CARTESIAN_POINT('Ctrl Pts',(-9.43656254042288,1.04828480643365,16.2560572449997));
#25600=CARTESIAN_POINT('Ctrl Pts',(-9.88735051158488,-0.220214228827959,
16.3037792684545));
#25601=CARTESIAN_POINT('Ctrl Pts',(-9.06591783859971,-1.2867785768872,16.3515012919094));
#25602=CARTESIAN_POINT('Ctrl Pts',(-7.72209157421216,-1.17099611903586,
16.3992233153643));
#25603=CARTESIAN_POINT('Ctrl Pts',(-7.20129244434704,-0.17873011326985,
16.4389916682433));
#25604=CARTESIAN_POINT('Ctrl Pts',(-7.42439036505487,0.607358648640506,
16.4708063505466));
#25605=CARTESIAN_POINT('Ctrl Pts',(-7.98229360457716,1.20439403072933,16.5026210328498));
#25606=CARTESIAN_POINT('Ctrl Pts',(-9.100952891,1.27091739730054,16.5423893857288));
#25607=CARTESIAN_POINT('Ctrl Pts',(-9.8941533483515,0.179994843177065,16.5901114091837));
#25608=CARTESIAN_POINT('Ctrl Pts',(-9.40510470497528,-1.07425147771346,
16.6378334326385));
#25609=CARTESIAN_POINT('Ctrl Pts',(-8.08606633854649,-1.34339894468471,
16.6855554560935));
#25610=CARTESIAN_POINT('Ctrl Pts',(-7.145545368936,-0.376600459845053,16.7332774795483));
#25611=CARTESIAN_POINT('Ctrl Pts',(-7.40090908890966,0.714551673218083,
16.7730458324274));
#25612=CARTESIAN_POINT('Ctrl Pts',(-8.08394846882832,1.16306574288832,16.8048605147306));
#25613=CARTESIAN_POINT('Ctrl Pts',(-8.89649255801945,1.24955134806578,16.8366751970338));
#25614=CARTESIAN_POINT('Ctrl Pts',(-9.786007031784,0.567944701423324,16.8764435499129));
#25615=CARTESIAN_POINT('Ctrl Pts',(-9.67209996192896,-0.776043466300687,
16.9241655733677));
#25616=CARTESIAN_POINT('Ctrl Pts',(-8.48162831789962,-1.40459717952674,
16.9718875968226));
#25617=CARTESIAN_POINT('Ctrl Pts',(-7.30800368174657,-0.745121842437952,
17.0196096202774));
#25618=CARTESIAN_POINT('Ctrl Pts',(-7.22928743756428,0.601385776393804,
17.0673316437324));
#25619=CARTESIAN_POINT('Ctrl Pts',(-8.13632495384472,1.25949409775313,17.1070999966114));
#25620=CARTESIAN_POINT('Ctrl Pts',(-8.94632905408739,1.15178607994229,17.1389146789146));
#25621=CARTESIAN_POINT('Ctrl Pts',(-9.61740393037904,0.685560630316964,
17.1707293612179));
#25622=CARTESIAN_POINT('Ctrl Pts',(-9.84414133781144,-0.411897235285352,
17.2104977140969));
#25623=CARTESIAN_POINT('Ctrl Pts',(-8.87865560148491,-1.35376575451348,
17.2582197375518));
#25624=CARTESIAN_POINT('Ctrl Pts',(-7.56710801788738,-1.05021107655027,
17.3059417610066));
#25625=CARTESIAN_POINT('Ctrl Pts',(-7.11103130626957,0.216397205310442,
17.3536637844615));
#25626=CARTESIAN_POINT('Ctrl Pts',(-7.93249344605425,1.28620044303824,17.4013858079163));
#25627=CARTESIAN_POINT('Ctrl Pts',(-9.04902998642944,1.19044151283572,17.4411541607954));
#25628=CARTESIAN_POINT('Ctrl Pts',(-9.59112719047142,0.579018352620608,
17.4729688430987));
#25629=CARTESIAN_POINT('Ctrl Pts',(-9.79358830678465,-0.212636342217181,
17.5047835254019));
#25630=CARTESIAN_POINT('Ctrl Pts',(-9.24701566858587,-1.19094200502388,
17.5445518782809));
#25631=CARTESIAN_POINT('Ctrl Pts',(-7.9006191498078,-1.27153622797434,17.5922739017358));
#25632=CARTESIAN_POINT('Ctrl Pts',(-7.10736636384562,-0.183854048235282,
17.6399959251907));
#25633=CARTESIAN_POINT('Ctrl Pts',(-7.59117194467839,1.07242405255042,17.6877179486456));
#25634=CARTESIAN_POINT('Ctrl Pts',(-8.91235513076913,1.34400093548014,17.7354399721004));
#25635=CARTESIAN_POINT('Ctrl Pts',(-9.69408654676645,0.541056596219814,
17.7752083249795));
#25636=CARTESIAN_POINT('Ctrl Pts',(-9.70400806777014,-0.276016976292779,
17.8070230072827));
#25637=CARTESIAN_POINT('Ctrl Pts',(-9.33915697445163,-1.0071745100581,17.8388376895859));
#25638=CARTESIAN_POINT('Ctrl Pts',(-8.28572482191837,-1.38941045645308,
17.878606042465));
#25639=CARTESIAN_POINT('Ctrl Pts',(-7.21477688206173,-0.569441234672508,
17.9263280659199));
#25640=CARTESIAN_POINT('Ctrl Pts',(-7.32652435883821,0.772130607605336,
17.9740500893747));
#25641=CARTESIAN_POINT('Ctrl Pts',(-8.51436022445611,1.40565129622602,18.0217721128296));
#25642=CARTESIAN_POINT('Ctrl Pts',(-9.69119642771782,0.746609897493594,
18.0694941362844));
#25643=CARTESIAN_POINT('Ctrl Pts',(-9.75703384557922,-0.372089817853069,
18.1092624891635));
#25644=CARTESIAN_POINT('Ctrl Pts',(-9.22994300794511,-0.996495862314252,
18.1410771714668));
#25645=CARTESIAN_POINT('Ctrl Pts',(-8.4756421899822,-1.31072179297238,18.1728918537699));
#25646=CARTESIAN_POINT('Ctrl Pts',(-7.42889170154707,-0.910550537547681,
18.212660206649));
#25647=CARTESIAN_POINT('Ctrl Pts',(-7.15547234904076,0.410252578827254,
18.2603822301039));
#25648=CARTESIAN_POINT('Ctrl Pts',(-8.11774393575135,1.35170672001962,18.3081042535588));
#25649=CARTESIAN_POINT('Ctrl Pts',(-9.43054799017888,1.05363286803438,18.3558262770136));
#25650=CARTESIAN_POINT('Ctrl Pts',(-9.88933737698507,-0.214748507224885,
18.4035483004685));
#25651=CARTESIAN_POINT('Ctrl Pts',(-9.20718549273468,-1.10384491680092,
18.4433166533475));
#25652=CARTESIAN_POINT('Ctrl Pts',(-8.40003557935687,-1.23118963326648,
18.4751313356508));
#25653=CARTESIAN_POINT('Ctrl Pts',(-7.62400167613423,-0.975300906421168,
18.506946017954));
#25654=CARTESIAN_POINT('Ctrl Pts',(-7.09421676335546,0.0121967213730914,
18.5467143708331));
#25655=CARTESIAN_POINT('Ctrl Pts',(-7.75161611674647,1.18995098466898,18.5944363942879));
#25656=CARTESIAN_POINT('Ctrl Pts',(-9.09531080539251,1.27233478321708,18.6421584177428));
#25657=CARTESIAN_POINT('Ctrl Pts',(-9.89309979053325,0.187975413936358,
18.6898804411977));
#25658=CARTESIAN_POINT('Ctrl Pts',(-9.41018558167302,-1.07141844083329,
18.7376024646525));
#25659=CARTESIAN_POINT('Ctrl Pts',(-8.31258890865753,-1.29748294953091,
18.7773708175316));
#25660=CARTESIAN_POINT('Ctrl Pts',(-7.61886014196042,-0.865686634430366,
18.8091854998348));
#25661=CARTESIAN_POINT('Ctrl Pts',(-7.19940452759574,-0.164427305041153,
18.841000182138));
#25662=CARTESIAN_POINT('Ctrl Pts',(-7.44485181710885,0.928998159623897,
18.8807685350171));
#25663=CARTESIAN_POINT('Ctrl Pts',(-8.71259205746091,1.38955618804453,18.9284905584719));
#25664=CARTESIAN_POINT('Ctrl Pts',(-9.78266761091162,0.572708089273526,
18.9762125819268));
#25665=CARTESIAN_POINT('Ctrl Pts',(-9.6765246946901,-0.769318806095816,
19.0239346053817));
#25666=CARTESIAN_POINT('Ctrl Pts',(-8.48732435991086,-1.40577899991123,
19.0716566288365));
#25667=CARTESIAN_POINT('Ctrl Pts',(-7.5093539869978,-0.858606661052929,
19.1114249817156));
#25668=CARTESIAN_POINT('Ctrl Pts',(-7.26723453363784,-0.0781671504038373,
19.1432396640188));
#25669=CARTESIAN_POINT('Ctrl Pts',(-7.40883903449548,0.726603515571496,
19.1750543463221));
#25670=CARTESIAN_POINT('Ctrl Pts',(-8.30986460269802,1.39291916460931,19.2148226992011));
#25671=CARTESIAN_POINT('Ctrl Pts',(-9.56993078200403,0.911761977902418,
19.262544722656));
#25672=CARTESIAN_POINT('Ctrl Pts',(-9.84473247440981,-0.406109994790532,
19.3102667461109));
#25673=CARTESIAN_POINT('Ctrl Pts',(-8.88640162358035,-1.3515752172642,19.3579887695657));
#25674=CARTESIAN_POINT('Ctrl Pts',(-7.57064242851217,-1.05483163242354,
19.4057107930206));
#25675=CARTESIAN_POINT('Ctrl Pts',(-7.18905241771698,-0.00116532738733117,
19.4454791458996));
#25676=CARTESIAN_POINT('Ctrl Pts',(-7.51657390327246,0.747458300330247,
19.4772938282029));
#25677=CARTESIAN_POINT('Ctrl Pts',(-8.15020726559116,1.26341994777524,19.5091085105061));
#25678=CARTESIAN_POINT('Ctrl Pts',(-9.26756713176743,1.17780132733557,19.5488768633852));
#25679=CARTESIAN_POINT('Ctrl Pts',(-9.90568535581634,-0.0105101413827072,
19.59659888684));
#25680=CARTESIAN_POINT('Ctrl Pts',(-9.25124918710935,-1.18695215340324,
19.6443209102949));
#25681=CARTESIAN_POINT('Ctrl Pts',(-7.90791032709937,-1.27494768593567,
19.6920429337497));
#25682=CARTESIAN_POINT('Ctrl Pts',(-7.10701614127563,-0.189660849350813,
19.7397649572047));
#25683=CARTESIAN_POINT('Ctrl Pts',(-7.50782908869113,0.856844095640571,
19.7795333100836));
#25684=CARTESIAN_POINT('Ctrl Pts',(-8.24532696405019,1.20870279358388,19.8113479923869));
#25685=CARTESIAN_POINT('Ctrl Pts',(-9.0620971317096,1.18432754591179,19.8431626746901));
#25686=CARTESIAN_POINT('Ctrl Pts',(-9.85108578157514,0.388513164858798,
19.8829310275692));
#25687=CARTESIAN_POINT('Ctrl Pts',(-9.55617765393731,-0.927658636542429,
19.9306530510241));
#25688=CARTESIAN_POINT('Ctrl Pts',(-8.29153691019929,-1.38916301987629,
19.9783750744789));
#25689=CARTESIAN_POINT('Ctrl Pts',(-7.21805881404244,-0.57679162474335,
20.0260970979338));
#25690=CARTESIAN_POINT('Ctrl Pts',(-7.32246023424974,0.767968338227514,
20.0738191213886));
#25691=CARTESIAN_POINT('Ctrl Pts',(-8.31028248984177,1.29714771241403,20.1135874742677));
#25692=CARTESIAN_POINT('Ctrl Pts',(-9.09823143854941,1.08071270205753,20.1454021565709));
#25693=CARTESIAN_POINT('Ctrl Pts',(-9.69996837905173,0.527883330630518,
20.1772168388742));
#25694=CARTESIAN_POINT('Ctrl Pts',(-9.77595908553397,-0.590172585339566,
20.2169851917532));
#25695=CARTESIAN_POINT('Ctrl Pts',(-8.69179035992437,-1.39257970704315,
20.2647072152081));
#25696=CARTESIAN_POINT('Ctrl Pts',(-7.43344900514689,-0.914166139702682,
20.312429238663));
#25697=CARTESIAN_POINT('Ctrl Pts',(-7.1531451156656,0.40254652299194,20.3601512621178));
#25698=CARTESIAN_POINT('Ctrl Pts',(-8.11194714289106,1.35121806105923,20.4078732855727));
#25699=CARTESIAN_POINT('Ctrl Pts',(-9.20522191726533,1.10510043384764,20.4476416384518));
#25700=CARTESIAN_POINT('Ctrl Pts',(-9.65950205965873,0.425882345377853,
20.479456320755));
#25701=CARTESIAN_POINT('Ctrl Pts',(-9.75286301069235,-0.385900502617611,
20.5112710030582));
#25702=CARTESIAN_POINT('Ctrl Pts',(-9.07881080904158,-1.28115311956834,
20.5510393559372));
#25703=CARTESIAN_POINT('Ctrl Pts',(-7.73390653914345,-1.17862741859382,
20.5987613793922));
#25704=CARTESIAN_POINT('Ctrl Pts',(-7.09529762703471,0.00648066252536313,
20.646483402847));
#25705=CARTESIAN_POINT('Ctrl Pts',(-7.7448142288305,1.1856459141124,20.6942054263018));
#25706=CARTESIAN_POINT('Ctrl Pts',(-9.09060724228286,1.2757579526721,20.7419274497568));
#25707=CARTESIAN_POINT('Ctrl Pts',(-9.75637034345738,0.374324032841098,
20.7816958026357));
#25708=CARTESIAN_POINT('Ctrl Pts',(-9.65552312703059,-0.43656282635472,
20.8135104849391));
#25709=CARTESIAN_POINT('Ctrl Pts',(-9.19499524498417,-1.11156040363579,
20.8453251672422));
#25710=CARTESIAN_POINT('Ctrl Pts',(-8.09949610707047,-1.34758001624817,
20.8850935201213));
#25711=CARTESIAN_POINT('Ctrl Pts',(-7.14948819284198,-0.390102090939205,
20.9328155435762));
#25712=CARTESIAN_POINT('Ctrl Pts',(-7.44192932700205,0.923968184810892,
20.980537567031));
#25713=CARTESIAN_POINT('Ctrl Pts',(-8.70463139019127,1.39075079607264,21.0282595904859));
#25714=CARTESIAN_POINT('Ctrl Pts',(-9.78135023333184,0.578374314768165,
21.0759816139408));
#25715=CARTESIAN_POINT('Ctrl Pts',(-9.69504657087012,-0.538932848259564,
21.1157499668198));
#25716=CARTESIAN_POINT('Ctrl Pts',(-9.08823434389678,-1.08618651948812,
21.147564649123));
#25717=CARTESIAN_POINT('Ctrl Pts',(-8.29832191286535,-1.29534198984334,
21.1793793314263));
#25718=CARTESIAN_POINT('Ctrl Pts',(-7.315424393124,-0.757070604393955,21.2191476843053));
#25719=CARTESIAN_POINT('Ctrl Pts',(-7.22343538367285,0.588595415348976,
21.2668697077602));
#25720=CARTESIAN_POINT('Ctrl Pts',(-8.30436345332364,1.39102735314789,21.314591731215));
#25721=CARTESIAN_POINT('Ctrl Pts',(-9.56469210780724,0.917873901035059,
21.36231375467));
#25722=CARTESIAN_POINT('Ctrl Pts',(-9.84744349518117,-0.400962960555038,
21.4100357781248));
#25723=CARTESIAN_POINT('Ctrl Pts',(-9.05114553138379,-1.18946354492994,
21.4498041310038));
#25724=CARTESIAN_POINT('Ctrl Pts',(-8.23418522462471,-1.20630149782281,
21.4816188133071));
#25725=CARTESIAN_POINT('Ctrl Pts',(-7.49996530886433,-0.847652958472259,
21.5134334956103));
#25726=CARTESIAN_POINT('Ctrl Pts',(-7.10882542066799,0.202505699335723,
21.5532018484894));
#25727=CARTESIAN_POINT('Ctrl Pts',(-7.9196993471952,1.28035656556392,21.6009238719442));
#25728=CARTESIAN_POINT('Ctrl Pts',(-9.26216909691203,1.17996992474953,21.6486458953991));
#25729=CARTESIAN_POINT('Ctrl Pts',(-9.90572249357285,-0.00246042508295246,
21.696367918854));
#25730=CARTESIAN_POINT('Ctrl Pts',(-9.25666700161002,-1.18483345543481,
21.7440899423088));
#25731=CARTESIAN_POINT('Ctrl Pts',(-8.13856470554957,-1.26013866276976,
21.7838582951879));
#25732=CARTESIAN_POINT('Ctrl Pts',(-7.50971904305091,-0.738352507113889,
21.8156729774912));
#25733=CARTESIAN_POINT('Ctrl Pts',(-7.18911897548137,0.0132612608227678,
21.8474876597943));
#25734=CARTESIAN_POINT('Ctrl Pts',(-7.58041481673441,1.06336181949582,21.8872560126734));
#25735=CARTESIAN_POINT('Ctrl Pts',(-8.89885602513675,1.34795239301706,21.9349780361283));
#25736=CARTESIAN_POINT('Ctrl Pts',(-9.84842236738186,0.393684994310642,
21.9827000595832));
#25737=CARTESIAN_POINT('Ctrl Pts',(-9.56147249923753,-0.921595310312913,
22.030422083038));
#25738=CARTESIAN_POINT('Ctrl Pts',(-8.29702036984018,-1.39110550936414,
22.0781441064929));
#25739=CARTESIAN_POINT('Ctrl Pts',(-7.40218118543914,-0.71650455119125,
22.1179124593719));
#25740=CARTESIAN_POINT('Ctrl Pts',(-7.2680082514545,0.0895384273548286,
22.1497271416752));
#25741=CARTESIAN_POINT('Ctrl Pts',(-7.51731843588521,0.867710703535758,
22.1815418239784));
#25742=CARTESIAN_POINT('Ctrl Pts',(-8.50029588260379,1.4058361145228,22.2213101768575));
#25743=CARTESIAN_POINT('Ctrl Pts',(-9.68357303965896,0.758430380734344,
22.2690322003123));
#25744=CARTESIAN_POINT('Ctrl Pts',(-9.77732868873411,-0.584518756361056,
22.3167542237672));
#25745=CARTESIAN_POINT('Ctrl Pts',(-8.69976171084787,-1.39145860215367,
22.3644762472221));
#25746=CARTESIAN_POINT('Ctrl Pts',(-7.43632495976926,-0.919222865921664,
22.4121982706769));
#25747=CARTESIAN_POINT('Ctrl Pts',(-7.20097704672433,0.176420770728819,
22.4519666235559));
#25748=CARTESIAN_POINT('Ctrl Pts',(-7.62688525551803,0.873779973119977,
22.4837813058592));
#25749=CARTESIAN_POINT('Ctrl Pts',(-8.32456863272794,1.29915694081149,22.5155959881624));
#25750=CARTESIAN_POINT('Ctrl Pts',(-9.42003270766891,1.06297463999032,22.5553643410415));
#25751=CARTESIAN_POINT('Ctrl Pts',(-9.89130605755087,-0.200821405359406,
22.6030863644963));
#25752=CARTESIAN_POINT('Ctrl Pts',(-9.08354575717079,-1.27777349514265,
22.6508083879512));
#25753=CARTESIAN_POINT('Ctrl Pts',(-7.74066841505343,-1.18299506623269,
22.6985304114061));
#25754=CARTESIAN_POINT('Ctrl Pts',(-7.09416406785961,0.000774820024847972,
22.7462524348609));
#25755=CARTESIAN_POINT('Ctrl Pts',(-7.63303797081583,0.983342138543073,
22.78602078774));
#25756=CARTESIAN_POINT('Ctrl Pts',(-8.4113998990915,1.23205958483199,22.8178354700432));
#25757=CARTESIAN_POINT('Ctrl Pts',(-9.21734045606203,1.09727279724702,22.8496501523464));
#25758=CARTESIAN_POINT('Ctrl Pts',(-9.89125969775638,0.201920087762355,
22.8894185052255));
#25759=CARTESIAN_POINT('Ctrl Pts',(-9.42078661216186,-1.06217409001151,
22.9371405286804));
#25760=CARTESIAN_POINT('Ctrl Pts',(-8.1052881443608,-1.34812214083849,22.9848625521353));
#25761=CARTESIAN_POINT('Ctrl Pts',(-7.1517442241385,-0.397829291888364,
23.0325845755901));
#25762=CARTESIAN_POINT('Ctrl Pts',(-7.43733885659921,0.920394786354866,
23.080306599045));
#25763=CARTESIAN_POINT('Ctrl Pts',(-8.48773712657024,1.31089074427156,23.120074951924));
#25764=CARTESIAN_POINT('Ctrl Pts',(-9.23910650345744,0.989718331144916,
23.1518896342273));
#25765=CARTESIAN_POINT('Ctrl Pts',(-9.76041357098137,0.360475452101273,
23.1837043165305));
#25766=CARTESIAN_POINT('Ctrl Pts',(-9.68425682465483,-0.757569166282248,
23.2234726694096));
#25767=CARTESIAN_POINT('Ctrl Pts',(-8.50138980836165,-1.40572395976629,
23.2711946928644));
#25768=CARTESIAN_POINT('Ctrl Pts',(-7.31944993986188,-0.761270195862776,
23.3189167163193));
#25769=CARTESIAN_POINT('Ctrl Pts',(-7.22008577008131,0.581275620235319,
23.3666387397741));
#25770=CARTESIAN_POINT('Ctrl Pts',(-8.29855389552885,1.39132840675251,23.414360763229));
#25771=CARTESIAN_POINT('Ctrl Pts',(-9.34841435168295,0.999388817898224,
23.4541291161081));
#25772=CARTESIAN_POINT('Ctrl Pts',(-9.70650359585349,0.264895963823484,
23.4859437984113));
#25773=CARTESIAN_POINT('Ctrl Pts',(-9.68904344055486,-0.552051281997461,
23.5177584807146));
#25774=CARTESIAN_POINT('Ctrl Pts',(-8.89993661427864,-1.34774848284182,
23.5575268335936));
#25775=CARTESIAN_POINT('Ctrl Pts',(-7.58131548221499,-1.06399273466057,
23.6052488570485));
#25776=CARTESIAN_POINT('Ctrl Pts',(-7.10912204955266,0.196695913939611,
23.6529708805033));
#25777=CARTESIAN_POINT('Ctrl Pts',(-7.91237700309648,1.27701252779228,23.7006929039582));
#25778=CARTESIAN_POINT('Ctrl Pts',(-9.25797257256842,1.1839986687818,23.7484149274131));
#25779=CARTESIAN_POINT('Ctrl Pts',(-9.79549521473797,0.200691479820764,
23.7881832802921));
#25780=CARTESIAN_POINT('Ctrl Pts',(-9.58573819775806,-0.589061426666565,
23.8199979625954));
#25781=CARTESIAN_POINT('Ctrl Pts',(-9.03802252939069,-1.19545668233927,
23.8518126448985));
#25782=CARTESIAN_POINT('Ctrl Pts',(-7.9206499604527,-1.28090936452179,23.8915809977777));
#25783=CARTESIAN_POINT('Ctrl Pts',(-7.10909375743094,-0.203572117468884,
23.9393030212324));
#25784=CARTESIAN_POINT('Ctrl Pts',(-7.57683792315452,1.05877407196975,23.9870250446874));
#25785=CARTESIAN_POINT('Ctrl Pts',(-8.89113054465059,1.3502143087931,24.0347470681422));
#25786=CARTESIAN_POINT('Ctrl Pts',(-9.84788465423753,0.399477442810103,
24.0824690915971));
#25787=CARTESIAN_POINT('Ctrl Pts',(-9.61103076409583,-0.6958416218611,24.1222374444761));
#25788=CARTESIAN_POINT('Ctrl Pts',(-8.93568263873,-1.15585528366082,24.1540521267794));
#25789=CARTESIAN_POINT('Ctrl Pts',(-8.12471920819932,-1.25608488916436,
24.1858668090826));
#25790=CARTESIAN_POINT('Ctrl Pts',(-7.22379260339601,-0.589635437619165,
24.2256351619617));
#25791=CARTESIAN_POINT('Ctrl Pts',(-7.31492958877942,0.756088555050138,
24.2733571854165));
#25792=CARTESIAN_POINT('Ctrl Pts',(-8.49458917842518,1.40470690131819,24.3210792088714));
#25793=CARTESIAN_POINT('Ctrl Pts',(-9.67921054321693,0.765195581138799,
24.3688012323263));
#25794=CARTESIAN_POINT('Ctrl Pts',(-9.78071191837591,-0.579786383569809,
24.4165232557811));
#25795=CARTESIAN_POINT('Ctrl Pts',(-8.88494619440142,-1.25315655402566,
24.4562916086602));
#25796=CARTESIAN_POINT('Ctrl Pts',(-8.07323468672448,-1.15917736599807,
24.4881062909634));
#25797=CARTESIAN_POINT('Ctrl Pts',(-7.39436278074097,-0.704380054282347,
24.5199209732667));
#25798=CARTESIAN_POINT('Ctrl Pts',(-7.14907787678811,0.389081849306566,
24.5596893261457));
#25799=CARTESIAN_POINT('Ctrl Pts',(-8.09847937545032,1.34716107822693,24.6074113496006));
#25800=CARTESIAN_POINT('Ctrl Pts',(-9.41497817327985,1.06585444504516,24.6551333730554));
#25801=CARTESIAN_POINT('Ctrl Pts',(-9.89243323319677,-0.19285091059547,
24.7028553965103));
#25802=CARTESIAN_POINT('Ctrl Pts',(-9.0892006276166,-1.27640819836731,24.7505774199652));
#25803=CARTESIAN_POINT('Ctrl Pts',(-7.97120291139482,-1.19956598841592,
24.7903457728442));
#25804=CARTESIAN_POINT('Ctrl Pts',(-7.41883199075804,-0.597408180601113,
24.8221604551474));
#25805=CARTESIAN_POINT('Ctrl Pts',(-7.20299715504592,0.190705379217913,
24.8539751374507));
#25806=CARTESIAN_POINT('Ctrl Pts',(-7.73292871366386,1.17812431861909,24.8937434903297));
#25807=CARTESIAN_POINT('Ctrl Pts',(-9.07776780005844,1.28150152237285,24.9414655137846));
#25808=CARTESIAN_POINT('Ctrl Pts',(-9.88932138510403,0.207405025237497,
24.9891875372394));
#25809=CARTESIAN_POINT('Ctrl Pts',(-9.42685396925393,-1.0568838641528,25.0369095606943));
#25810=CARTESIAN_POINT('Ctrl Pts',(-8.11045794382281,-1.35078949318993,
25.0846315841492));
#25811=CARTESIAN_POINT('Ctrl Pts',(-7.31524469729938,-0.561194969867331,
25.1243999370282));
#25812=CARTESIAN_POINT('Ctrl Pts',(-7.29149151917362,0.255593525403265,
25.1562146193315));
#25813=CARTESIAN_POINT('Ctrl Pts',(-7.64391180276608,0.992823206839166,
25.1880293016347));
#25814=CARTESIAN_POINT('Ctrl Pts',(-8.69072170844657,1.39283900662292,25.2277976545138));
#25815=CARTESIAN_POINT('Ctrl Pts',(-9.77539825914043,0.59111848491638,25.2755196779686));
#25816=CARTESIAN_POINT('Ctrl Pts',(-9.68637964828473,-0.752152966980069,
25.3232417014235));
#25817=CARTESIAN_POINT('Ctrl Pts',(-8.50943955061137,-1.40569295278612,
25.3709637248783));
#25818=CARTESIAN_POINT('Ctrl Pts',(-7.32161442543538,-0.76666988078383,
25.4186857483332));
#25819=CARTESIAN_POINT('Ctrl Pts',(-7.23684682521555,0.350754869550781,
25.4584541012123));
#25820=CARTESIAN_POINT('Ctrl Pts',(-7.75329090619035,0.983995085190644,
25.4902687835155));
#25821=CARTESIAN_POINT('Ctrl Pts',(-8.50216376128743,1.31094631454484,25.5220834658187));
#25822=CARTESIAN_POINT('Ctrl Pts',(-9.55553913695975,0.928553928853571,
25.5618518186978));
#25823=CARTESIAN_POINT('Ctrl Pts',(-9.85128053691354,-0.387430888271607,
25.6095738421527));
#25824=CARTESIAN_POINT('Ctrl Pts',(-8.90508571176895,-1.34504138290304,
25.6572958656075));
#25825=CARTESIAN_POINT('Ctrl Pts',(-7.58742341373451,-1.06923606225583,
25.7050178890624));
#25826=CARTESIAN_POINT('Ctrl Pts',(-7.10722604889511,0.191196206988292,
25.7527399125173));
#25827=CARTESIAN_POINT('Ctrl Pts',(-7.77422773713762,1.09171403945412,25.7925082653963));
#25828=CARTESIAN_POINT('Ctrl Pts',(-8.57910601748431,1.23270557573783,25.8243229476995));
#25829=CARTESIAN_POINT('Ctrl Pts',(-9.35936090055085,0.989991800009503,
25.8561376300028));
#25830=CARTESIAN_POINT('Ctrl Pts',(-9.90578824612508,0.0116049773692086,
25.8959059828818));
#25831=CARTESIAN_POINT('Ctrl Pts',(-9.26842252690367,-1.17711027638675,
25.9436280063367));
#25832=CARTESIAN_POINT('Ctrl Pts',(-7.92631518097252,-1.2822310571884,25.9913500297916));
#25833=CARTESIAN_POINT('Ctrl Pts',(-7.11028230216784,-0.211533692258238,
26.0390720532464));
#25834=CARTESIAN_POINT('Ctrl Pts',(-7.57180572399499,1.05585541360293,26.0867940767013));
#25835=CARTESIAN_POINT('Ctrl Pts',(-8.66541780729333,1.30046986528404,26.1265624295803));
#25836=CARTESIAN_POINT('Ctrl Pts',(-9.36635747060411,0.880480284609375,
26.1583771118836));
#25837=CARTESIAN_POINT('Ctrl Pts',(-9.79762530788041,0.186422857584386,
26.1901917941868));
#25838=CARTESIAN_POINT('Ctrl Pts',(-9.57072492125683,-0.9110013235131,26.2299601470659));
#25839=CARTESIAN_POINT('Ctrl Pts',(-8.31096363818387,-1.39295622204707,
26.2776821705207));
#25840=CARTESIAN_POINT('Ctrl Pts',(-7.22721218956511,-0.594341606493663,
26.3254041939756));
#25841=CARTESIAN_POINT('Ctrl Pts',(-7.31061933906771,0.749289947903038,
26.3731262174305));
#25842=CARTESIAN_POINT('Ctrl Pts',(-8.48887394443472,1.4057921181066,26.4208482408854));
#25843=CARTESIAN_POINT('Ctrl Pts',(-9.47596779494645,0.875255268312624,
26.4606165937644));
#25844=CARTESIAN_POINT('Ctrl Pts',(-9.73126541035378,0.0990267020740463,
26.4924312760676));
#25845=CARTESIAN_POINT('Ctrl Pts',(-9.60330599525195,-0.70802598986389,
26.5242459583709));
#25846=CARTESIAN_POINT('Ctrl Pts',(-8.71369030804601,-1.38950052921557,
26.5640143112499));
#25847=CARTESIAN_POINT('Ctrl Pts',(-7.44565872044378,-0.929745260193386,
26.6117363347048));
#25848=CARTESIAN_POINT('Ctrl Pts',(-7.14858480305884,0.383285430296478,
26.6594583581596));
#25849=CARTESIAN_POINT('Ctrl Pts',(-8.09077154939971,1.3448397145562,26.7071803816145));
#25850=CARTESIAN_POINT('Ctrl Pts',(-9.41136604307352,1.07041450101146,26.7549024050693));
#25851=CARTESIAN_POINT('Ctrl Pts',(-9.81073996404354,0.0233595406792121,
26.7946707579485));
#25852=CARTESIAN_POINT('Ctrl Pts',(-9.49593963948833,-0.730701740078134,
26.8264854402517));
#25853=CARTESIAN_POINT('Ctrl Pts',(-8.87113233708174,-1.25731686931094,
26.8583001225549));
#25854=CARTESIAN_POINT('Ctrl Pts',(-7.75248308879724,-1.19062745470989,
26.898068475434));
#25855=CARTESIAN_POINT('Ctrl Pts',(-7.09433817452238,-0.0132896585083106,
26.9457904988888));
#25856=CARTESIAN_POINT('Ctrl Pts',(-7.72876335020465,1.17406336524635,26.9935125223437));
#25857=CARTESIAN_POINT('Ctrl Pts',(-9.07041991168043,1.28478905155158,27.0412345457985));
#25858=CARTESIAN_POINT('Ctrl Pts',(-9.88957324816892,0.213216923381752,
27.0889565692534));
#25859=CARTESIAN_POINT('Ctrl Pts',(-9.50653510539861,-0.839923807902734,
27.1287249221325));
#25860=CARTESIAN_POINT('Ctrl Pts',(-8.7750999084873,-1.20421793659106,27.1605396044357));
#25861=CARTESIAN_POINT('Ctrl Pts',(-7.9580341293038,-1.19367412491104,27.192354286739));
#25862=CARTESIAN_POINT('Ctrl Pts',(-7.15568539944002,-0.411331403085548,
27.232122639618));
#25863=CARTESIAN_POINT('Ctrl Pts',(-7.42826843340841,0.909644563441927,
27.2798446630729));
#25864=CARTESIAN_POINT('Ctrl Pts',(-8.68491464228127,1.39249320668759,27.3275666865277));
#25865=CARTESIAN_POINT('Ctrl Pts',(-9.77199235522125,0.598412258302711,
27.3752887099826));
#25866=CARTESIAN_POINT('Ctrl Pts',(-9.69037272304938,-0.747922488405797,
27.4230107334374));
#25867=CARTESIAN_POINT('Ctrl Pts',(-8.71165106735223,-1.29374987813343,
27.4627790863165));
#25868=CARTESIAN_POINT('Ctrl Pts',(-7.92015079905928,-1.09068588632374,
27.4945937686197));
#25869=CARTESIAN_POINT('Ctrl Pts',(-7.30914068425147,-0.548123171902564,
27.526408450923));
#25870=CARTESIAN_POINT('Ctrl Pts',(-7.21423215015474,0.56848597585817,27.5661768038021));
#25871=CARTESIAN_POINT('Ctrl Pts',(-8.2846607135526,1.3891331017367,27.6138988272568));
#25872=CARTESIAN_POINT('Ctrl Pts',(-9.55092127427873,0.932091857527698,
27.6616208507118));
#25873=CARTESIAN_POINT('Ctrl Pts',(-9.85347697299502,-0.379686536764967,
27.7093428741665));
#25874=CARTESIAN_POINT('Ctrl Pts',(-8.91087340080395,-1.34445465410882,
27.7570648976215));
#25875=CARTESIAN_POINT('Ctrl Pts',(-7.81358853956333,-1.11688147467079,
27.7968332505005));
#25876=CARTESIAN_POINT('Ctrl Pts',(-7.34787432426479,-0.445451709806008,
27.8286479328038));
#25877=CARTESIAN_POINT('Ctrl Pts',(-7.24078324703436,0.364634187278428,
27.860462615107));
#25878=CARTESIAN_POINT('Ctrl Pts',(-7.89958218878159,1.27117021693195,27.9002309679861));
#25879=CARTESIAN_POINT('Ctrl Pts',(-9.2460294657544,1.19142847827918,27.9479529914409));
#25880=CARTESIAN_POINT('Ctrl Pts',(-9.90461076431774,0.0173019179198019,
27.9956750148958));
#25881=CARTESIAN_POINT('Ctrl Pts',(-9.27515055498282,-1.17269066668845,
28.0433970383506));
#25882=CARTESIAN_POINT('Ctrl Pts',(-7.93107602430974,-1.28557410456496,
28.0911190618055));
#25883=CARTESIAN_POINT('Ctrl Pts',(-7.25014704022386,-0.395540769605531,
28.1308874146846));
#25884=CARTESIAN_POINT('Ctrl Pts',(-7.3372514650321,0.416937216961606,28.1627020969878));
#25885=CARTESIAN_POINT('Ctrl Pts',(-7.78628561432887,1.09963480172617,28.1945167792911));
#25886=CARTESIAN_POINT('Ctrl Pts',(-8.87763192295398,1.35416741919462,28.2342851321701));
#25887=CARTESIAN_POINT('Ctrl Pts',(-9.84371380784354,0.412910384032882,
28.2820071556249));
#25888=CARTESIAN_POINT('Ctrl Pts',(-9.57356183488256,-0.905922591770999,
28.3297291790799));
#25889=CARTESIAN_POINT('Ctrl Pts',(-8.3189433892574,-1.39401588453317,28.3774512025346));
#25890=CARTESIAN_POINT('Ctrl Pts',(-7.22862530768708,-0.599984716648168,
28.4251732259896));
#25891=CARTESIAN_POINT('Ctrl Pts',(-7.29600055841505,0.518623433827608,
28.4649415788686));
#25892=CARTESIAN_POINT('Ctrl Pts',(-7.89346079467198,1.07607201936972,28.4967562611719));
#25893=CARTESIAN_POINT('Ctrl Pts',(-8.67971900484753,1.29857075310551,28.5285709434751));
#25894=CARTESIAN_POINT('Ctrl Pts',(-9.67158860247685,0.777016997712584,
28.5683392963541));
#25895=CARTESIAN_POINT('Ctrl Pts',(-9.78634659247671,-0.56689878022201,
28.616061319809));
#25896=CARTESIAN_POINT('Ctrl Pts',(-8.71915864026611,-1.38751585434476,
28.6637833432638));
#25897=CARTESIAN_POINT('Ctrl Pts',(-7.45100011939933,-0.935767616313009,
28.7115053667187));
#25898=CARTESIAN_POINT('Ctrl Pts',(-7.14596130919067,0.378093235837449,
28.7592273901736));
#25899=CARTESIAN_POINT('Ctrl Pts',(-7.92879581040033,1.17996215792724,28.7989957430527));
#25900=CARTESIAN_POINT('Ctrl Pts',(-8.74535395632626,1.21062885803138,28.8308104253558));
#25901=CARTESIAN_POINT('Ctrl Pts',(-9.48554058013625,0.864462087680875,
28.8626251076592));
#25902=CARTESIAN_POINT('Ctrl Pts',(-9.89440360594169,-0.17892405294294,
28.9023934605382));
#25903=CARTESIAN_POINT('Ctrl Pts',(-9.10189397776309,-1.27034854886995,
28.950115483993));
#25904=CARTESIAN_POINT('Ctrl Pts',(-7.75791702419191,-1.19270436179798,
28.9978375074479));
#25905=CARTESIAN_POINT('Ctrl Pts',(-7.09443740014052,-0.0213388321030302,
29.0455595309027));
#25906=CARTESIAN_POINT('Ctrl Pts',(-7.72338203077529,1.1718532119868,29.0932815543577));
#25907=CARTESIAN_POINT('Ctrl Pts',(-8.84004957245219,1.26607722708656,29.1330499072366));
#25908=CARTESIAN_POINT('Ctrl Pts',(-9.47763834518235,0.755012087082805,
29.1648645895399));
#25909=CARTESIAN_POINT('Ctrl Pts',(-9.81091851614448,0.00893409317460413,
29.1966792718431));
#25910=CARTESIAN_POINT('Ctrl Pts',(-9.43745431001592,-1.04764123587576,
29.2364476247222));
#25911=CARTESIAN_POINT('Ctrl Pts',(-8.12402506966911,-1.35451113192694,
29.2841696481771));
#25912=CARTESIAN_POINT('Ctrl Pts',(-7.15843040209203,-0.416458701888962,
29.3318916716319));
#25913=CARTESIAN_POINT('Ctrl Pts',(-7.42308757914243,0.903494929509393,
29.3796136950868));
#25914=CARTESIAN_POINT('Ctrl Pts',(-8.67937808940375,1.39433769122377,29.4273357185416));
#25915=CARTESIAN_POINT('Ctrl Pts',(-9.58556770780354,0.734996509965079,
29.4671040714208));
#25916=CARTESIAN_POINT('Ctrl Pts',(-9.73328209692014,-0.0686793482256725,
29.4989187537239));
#25917=CARTESIAN_POINT('Ctrl Pts',(-9.49735030797155,-0.850921733780152,
29.5307334360272));
#25918=CARTESIAN_POINT('Ctrl Pts',(-8.52325181788503,-1.40569864308938,
29.5705017889063));
#25919=CARTESIAN_POINT('Ctrl Pts',(-7.32986179028487,-0.778260502859741,
29.6182238123611));
#25920=CARTESIAN_POINT('Ctrl Pts',(-7.21218073812471,0.56262788812223,29.665945835816));
#25921=CARTESIAN_POINT('Ctrl Pts',(-8.27818752900583,1.38822684395199,29.7136678592708));
#25922=CARTESIAN_POINT('Ctrl Pts',(-9.33384484159048,1.01168221201436,29.7534362121499));
#25923=CARTESIAN_POINT('Ctrl Pts',(-9.70261207523359,0.282249903129775,
29.7852508944531));
#25924=CARTESIAN_POINT('Ctrl Pts',(-9.69665295292861,-0.534421386281917,
29.8170655767564));
#25925=CARTESIAN_POINT('Ctrl Pts',(-8.92010172213024,-1.34249070178533,
29.8568339296354));
#25926=CARTESIAN_POINT('Ctrl Pts',(-7.5957088359255,-1.076002984984,29.9045559530903));
#25927=CARTESIAN_POINT('Ctrl Pts',(-7.18991001744901,-0.0344549071388059,
29.9443243059693));
#25928=CARTESIAN_POINT('Ctrl Pts',(-7.49844573549237,0.725568290707585,
29.9761389882726));
#25929=CARTESIAN_POINT('Ctrl Pts',(-7.80953045183888,0.987070987050173,
29.9920463294242));
#25930=CARTESIAN_POINT('Ctrl Pts',(-7.9881611888325,1.07233375495115,30.));
#25931=CARTESIAN_POINT('Ctrl Pts',(-7.84336223800221,-0.920831852263776,
1.73389339417779));
#25932=CARTESIAN_POINT('Ctrl Pts',(-7.68996888294128,-0.811448288777214,
1.7418470647536));
#25933=CARTESIAN_POINT('Ctrl Pts',(-7.44147150789439,-0.515011305712358,
1.75775440590522));
#25934=CARTESIAN_POINT('Ctrl Pts',(-7.27756915484984,0.248331434474109,
1.78956908820846));
#25935=CARTESIAN_POINT('Ctrl Pts',(-7.82972574274999,1.15778987946338,1.82933744108751));
#25936=CARTESIAN_POINT('Ctrl Pts',(-9.11518963502401,1.1892113537284,1.87705946454237));
#25937=CARTESIAN_POINT('Ctrl Pts',(-9.70989914651746,0.303653650183944,
1.91682781742143));
#25938=CARTESIAN_POINT('Ctrl Pts',(-9.58081711606472,-0.462897910902464,
1.94864249972467));
#25939=CARTESIAN_POINT('Ctrl Pts',(-9.1148424724598,-1.08587738685965,1.98045718202791));
#25940=CARTESIAN_POINT('Ctrl Pts',(-8.06315002296502,-1.26478329921431,
2.02022553490696));
#25941=CARTESIAN_POINT('Ctrl Pts',(-7.19998796076663,-0.315061926834089,
2.06794755836182));
#25942=CARTESIAN_POINT('Ctrl Pts',(-7.53141637453974,0.922516240590291,
2.11566958181669));
#25943=CARTESIAN_POINT('Ctrl Pts',(-8.7535951383005,1.31390426831436,2.16339160527155));
#25944=CARTESIAN_POINT('Ctrl Pts',(-9.57525824943383,0.633214111788618,
2.2031599581506));
#25945=CARTESIAN_POINT('Ctrl Pts',(-9.66743586945616,-0.138985158650247,
2.23497464045384));
#25946=CARTESIAN_POINT('Ctrl Pts',(-9.39643922585092,-0.868013858452754,
2.26678932275708));
#25947=CARTESIAN_POINT('Ctrl Pts',(-8.43822881651588,-1.33666768258406,
2.30655767563613));
#25948=CARTESIAN_POINT('Ctrl Pts',(-7.3414888899664,-0.669377881206568,
2.354279699091));
#25949=CARTESIAN_POINT('Ctrl Pts',(-7.31105138266357,0.611622684002372,
2.40200172254586));
#25950=CARTESIAN_POINT('Ctrl Pts',(-8.37090883221922,1.33175184955348,2.44972374600072));
#25951=CARTESIAN_POINT('Ctrl Pts',(-9.55154902931157,0.827500878887315,
2.49744576945558));
#25952=CARTESIAN_POINT('Ctrl Pts',(-9.72741589040921,-0.224544184030281,
2.53721412233464));
#25953=CARTESIAN_POINT('Ctrl Pts',(-9.29196288579558,-0.868979538690168,
2.56902880463787));
#25954=CARTESIAN_POINT('Ctrl Pts',(-8.60999646405335,-1.24292755198912,
2.60084348694112));
#25955=CARTESIAN_POINT('Ctrl Pts',(-7.57874071102671,-0.97046216532521,
2.64061183982017));
#25956=CARTESIAN_POINT('Ctrl Pts',(-7.18590781273401,0.251779422282229,
2.68833386327503));
#25957=CARTESIAN_POINT('Ctrl Pts',(-8.00102785596058,1.24044081982532,2.7360558867299));
#25958=CARTESIAN_POINT('Ctrl Pts',(-9.27371025598029,1.09160606477469,2.78377791018476));
#25959=CARTESIAN_POINT('Ctrl Pts',(-9.83665460260352,-0.0622076783418028,
2.83149993363962));
#25960=CARTESIAN_POINT('Ctrl Pts',(-9.28132245236828,-0.972883886508404,
2.87126828651867));
#25961=CARTESIAN_POINT('Ctrl Pts',(-8.53036971029236,-1.1753335976729,2.90308296882191));
#25962=CARTESIAN_POINT('Ctrl Pts',(-7.76996377379206,-1.01193622592224,
2.93489765112516));
#25963=CARTESIAN_POINT('Ctrl Pts',(-7.16834172261016,-0.131154827519332,
2.97466600400421));
#25964=CARTESIAN_POINT('Ctrl Pts',(-7.67094735813036,1.05019191790059,3.02238802745907));
#25965=CARTESIAN_POINT('Ctrl Pts',(-8.93424496562127,1.26455441305742,3.07011005091393));
#25966=CARTESIAN_POINT('Ctrl Pts',(-9.79933578640807,0.319308413861016,
3.11783207436879));
#25967=CARTESIAN_POINT('Ctrl Pts',(-9.4701483140956,-0.921589714816724,
3.16555409782365));
#25968=CARTESIAN_POINT('Ctrl Pts',(-8.45434027041126,-1.24694948055712,
3.20532245070271));
#25969=CARTESIAN_POINT('Ctrl Pts',(-7.75397118940257,-0.908720199684656,
3.23713713300595));
#25970=CARTESIAN_POINT('Ctrl Pts',(-7.28581913026257,-0.287632810134478,
3.26895181530919));
#25971=CARTESIAN_POINT('Ctrl Pts',(-7.40711716645252,0.772089674964555,
3.30872016818824));
#25972=CARTESIAN_POINT('Ctrl Pts',(-8.56014462832698,1.33664279908732,3.35644219164311));
#25973=CARTESIAN_POINT('Ctrl Pts',(-9.65577050263654,0.672206143179195,
3.40416421509796));
#25974=CARTESIAN_POINT('Ctrl Pts',(-9.6915437695127,-0.608649976596257,
3.45188623855283));
#25975=CARTESIAN_POINT('Ctrl Pts',(-8.63070115364378,-1.33170288070012,
3.49960826200769));
#25976=CARTESIAN_POINT('Ctrl Pts',(-7.64961690888714,-0.913135486265902,
3.53937661488675));
#25977=CARTESIAN_POINT('Ctrl Pts',(-7.34125675698761,-0.199111738272663,
3.57119129718998));
#25978=CARTESIAN_POINT('Ctrl Pts',(-7.39357959894616,0.576889689681292,
3.60300597949323));
#25979=CARTESIAN_POINT('Ctrl Pts',(-8.17866573276028,1.29894558882475,3.64277433237228));
#25980=CARTESIAN_POINT('Ctrl Pts',(-9.42002179212659,0.971489192263309,
3.69049635582714));
#25981=CARTESIAN_POINT('Ctrl Pts',(-9.81386559492375,-0.247838157214267,
3.738218379282));
#25982=CARTESIAN_POINT('Ctrl Pts',(-9.00288207825834,-1.23989554561616,
3.78594040273686));
#25983=CARTESIAN_POINT('Ctrl Pts',(-7.72753804870358,-1.09261973615206,
3.83366242619173));
#25984=CARTESIAN_POINT('Ctrl Pts',(-7.25944965685775,-0.13417400664288,
3.87343077907078));
#25985=CARTESIAN_POINT('Ctrl Pts',(-7.49342196021817,0.607562373237147,
3.90524546137402));
#25986=CARTESIAN_POINT('Ctrl Pts',(-8.04071266532901,1.16018229694294,3.93706014367726));
#25987=CARTESIAN_POINT('Ctrl Pts',(-9.10686262033383,1.19257415453766,3.97682849655631));
#25988=CARTESIAN_POINT('Ctrl Pts',(-9.83139444220645,0.13274105594708,4.02455052001118));
#25989=CARTESIAN_POINT('Ctrl Pts',(-9.33145993517061,-1.04706300187806,
4.07227254346604));
#25990=CARTESIAN_POINT('Ctrl Pts',(-8.06906871353424,-1.26670027039436,
4.1199945669209));
#25991=CARTESIAN_POINT('Ctrl Pts',(-7.20094501503803,-0.32089172640491,
4.16771659037576));
#25992=CARTESIAN_POINT('Ctrl Pts',(-7.47404245851617,0.710196410158088,
4.20748494325482));
#25993=CARTESIAN_POINT('Ctrl Pts',(-8.13628727307677,1.11805386266434,4.23929962555805));
#25994=CARTESIAN_POINT('Ctrl Pts',(-8.91174525720005,1.17789373930854,4.2711143078613));
#25995=CARTESIAN_POINT('Ctrl Pts',(-9.73921801071789,0.504830739894083,
4.31088266074035));
#25996=CARTESIAN_POINT('Ctrl Pts',(-9.59372114360799,-0.770717463599363,
4.35860468419521));
#25997=CARTESIAN_POINT('Ctrl Pts',(-8.44372307881386,-1.33585158675566,
4.40632670765008));
#25998=CARTESIAN_POINT('Ctrl Pts',(-7.34533148911299,-0.675997025613394,
4.45404873110494));
#25999=CARTESIAN_POINT('Ctrl Pts',(-7.3076326594131,0.607268868896949,4.5017707545598));
#26000=CARTESIAN_POINT('Ctrl Pts',(-8.18878274818164,1.20835079347829,4.54153910743885));
#26001=CARTESIAN_POINT('Ctrl Pts',(-8.95646012486506,1.08350151912803,4.57335378974209));
#26002=CARTESIAN_POINT('Ctrl Pts',(-9.58205477061933,0.621389806248012,
4.60516847204534));
#26003=CARTESIAN_POINT('Ctrl Pts',(-9.76746285062318,-0.429014307826431,
4.64493682492438));
#26004=CARTESIAN_POINT('Ctrl Pts',(-8.82286605099045,-1.2984563380376,4.69265884837925));
#26005=CARTESIAN_POINT('Ctrl Pts',(-7.5834208477958,-0.973421394587389,
4.7403808718341));
#26006=CARTESIAN_POINT('Ctrl Pts',(-7.18448749550299,0.244250279803643,
4.78810289528898));
#26007=CARTESIAN_POINT('Ctrl Pts',(-7.99559146371714,1.2393899235328,4.83582491874383));
#26008=CARTESIAN_POINT('Ctrl Pts',(-9.05523938128985,1.11744218973236,4.87559327162289));
#26009=CARTESIAN_POINT('Ctrl Pts',(-9.55411169716992,0.520749380637289,
4.90740795392613));
#26010=CARTESIAN_POINT('Ctrl Pts',(-9.72486976937421,-0.238037530658888,
4.93922263622937));
#26011=CARTESIAN_POINT('Ctrl Pts',(-9.17782796817209,-1.15371772959998,
4.97899098910842));
#26012=CARTESIAN_POINT('Ctrl Pts',(-7.8946159026944,-1.19320637083518,5.02671301256328));
#26013=CARTESIAN_POINT('Ctrl Pts',(-7.16994486640164,-0.136454737127305,
5.07443503601815));
#26014=CARTESIAN_POINT('Ctrl Pts',(-7.66494711141124,1.0454271959021,5.12215705947301));
#26015=CARTESIAN_POINT('Ctrl Pts',(-8.92944607964153,1.26731662133429,5.16987908292787));
#26016=CARTESIAN_POINT('Ctrl Pts',(-9.65102050340854,0.481787939515094,
5.20964743580693));
#26017=CARTESIAN_POINT('Ctrl Pts',(-9.63789081754475,-0.295864622575736,
5.24146211811016));
#26018=CARTESIAN_POINT('Ctrl Pts',(-9.27056889001754,-0.981423152195916,
5.27327680041342));
#26019=CARTESIAN_POINT('Ctrl Pts',(-8.25775645274699,-1.3159914201255,5.31304515329245));
#26020=CARTESIAN_POINT('Ctrl Pts',(-7.26148648143051,-0.506276222029801,
5.36076717674732));
#26021=CARTESIAN_POINT('Ctrl Pts',(-7.40486192963386,0.767032698475483,
5.40848920020218));
#26022=CARTESIAN_POINT('Ctrl Pts',(-8.55248946485333,1.33696529676413,5.45621122365705));
#26023=CARTESIAN_POINT('Ctrl Pts',(-9.65394858372652,0.677434882586624,
5.5039332471119));
#26024=CARTESIAN_POINT('Ctrl Pts',(-9.68568677413502,-0.388734731623442,
5.54370159999096));
#26025=CARTESIAN_POINT('Ctrl Pts',(-9.16695572119068,-0.968246587143773,
5.5755162822942));
#26026=CARTESIAN_POINT('Ctrl Pts',(-8.44062079418711,-1.24637150474729,
5.60733096459744));
#26027=CARTESIAN_POINT('Ctrl Pts',(-7.4557770578489,-0.836728032944395,
5.6470993174765));
#26028=CARTESIAN_POINT('Ctrl Pts',(-7.23212417540165,0.427460222794115,
5.69482134093136));
#26029=CARTESIAN_POINT('Ctrl Pts',(-8.17365152926984,1.29659678749714,5.74254336438622));
#26030=CARTESIAN_POINT('Ctrl Pts',(-9.41444355276615,0.976741694347395,
5.79026538784108));
#26031=CARTESIAN_POINT('Ctrl Pts',(-9.81590881670993,-0.242691862522644,
5.83798741129594));
#26032=CARTESIAN_POINT('Ctrl Pts',(-9.14233861671162,-1.06975180271407,
5.877755764175));
#26033=CARTESIAN_POINT('Ctrl Pts',(-8.37088414006259,-1.16861477068245,
5.90957044647823));
#26034=CARTESIAN_POINT('Ctrl Pts',(-7.63961966684838,-0.903722025987471,
5.94138512878148));
#26035=CARTESIAN_POINT('Ctrl Pts',(-7.16284941248119,0.0504347135191421,
5.98115348166053));
#26036=CARTESIAN_POINT('Ctrl Pts',(-7.82084291379945,1.15281264780352,6.02887550511539));
#26037=CARTESIAN_POINT('Ctrl Pts',(-9.10153384108041,1.19407855341718,6.07659752857025));
#26038=CARTESIAN_POINT('Ctrl Pts',(-9.83061248159845,0.140363002556222,
6.12431955202512));
#26039=CARTESIAN_POINT('Ctrl Pts',(-9.3363722406032,-1.04450793638824,6.17204157547998));
#26040=CARTESIAN_POINT('Ctrl Pts',(-8.28585464946359,-1.2292719742891,6.21180992835902));
#26041=CARTESIAN_POINT('Ctrl Pts',(-7.6377556831852,-0.799291014377838,
6.24362461066228));
#26042=CARTESIAN_POINT('Ctrl Pts',(-7.25804823806631,-0.120514061249209,
6.2754392929655));
#26043=CARTESIAN_POINT('Ctrl Pts',(-7.5217737984046,0.913010872083068,6.31520764584457));
#26044=CARTESIAN_POINT('Ctrl Pts',(-8.74064622138336,1.31617656292995,6.36292966929942));
#26045=CARTESIAN_POINT('Ctrl Pts',(-9.73617240019874,0.509454954517775,
6.4106516927543));
#26046=CARTESIAN_POINT('Ctrl Pts',(-9.59811666235571,-0.764441720819152,
6.45837371620915));
#26047=CARTESIAN_POINT('Ctrl Pts',(-8.44910975161753,-1.33713332792554,
6.50609573966402));
#26048=CARTESIAN_POINT('Ctrl Pts',(-7.53376511844561,-0.78953022209195,
6.54586409254306));
#26049=CARTESIAN_POINT('Ctrl Pts',(-7.32496560452136,-0.0403181967197514,
6.57767877484631));
#26050=CARTESIAN_POINT('Ctrl Pts',(-7.48192004532567,0.721443708004499,
6.60949345714955));
#26051=CARTESIAN_POINT('Ctrl Pts',(-8.3575769611271,1.33050029388492,6.6492618100286));
#26052=CARTESIAN_POINT('Ctrl Pts',(-9.54313609419374,0.83791314446213,6.69698383348346));
#26053=CARTESIAN_POINT('Ctrl Pts',(-9.76818512374022,-0.423524551377841,
6.74470585693832));
#26054=CARTESIAN_POINT('Ctrl Pts',(-8.83029626289538,-1.29658618201396,
6.79242788039319));
#26055=CARTESIAN_POINT('Ctrl Pts',(-7.58665592075209,-0.977915102108791,
6.84014990384804));
#26056=CARTESIAN_POINT('Ctrl Pts',(-7.25270867534208,0.0351022700415088,
6.8799182567271));
#26057=CARTESIAN_POINT('Ctrl Pts',(-7.58499699015572,0.738309474082838,
6.91173293903034));
#26058=CARTESIAN_POINT('Ctrl Pts',(-8.20209906933813,1.21170246077153,6.94354762133359));
#26059=CARTESIAN_POINT('Ctrl Pts',(-9.26281040945734,1.09937965837702,6.98331597421263));
#26060=CARTESIAN_POINT('Ctrl Pts',(-9.83710404863512,-0.0488273672825927,
7.0310379976675));
#26061=CARTESIAN_POINT('Ctrl Pts',(-9.18196602157746,-1.15003865113727,
7.07876002112236));
#26062=CARTESIAN_POINT('Ctrl Pts',(-7.90145862879751,-1.19665349020977,
7.12648204457722));
#26063=CARTESIAN_POINT('Ctrl Pts',(-7.16945126292874,-0.141969758426622,
7.17420406803208));
#26064=CARTESIAN_POINT('Ctrl Pts',(-7.57969846964756,0.842622638646724,
7.21397242091114));
#26065=CARTESIAN_POINT('Ctrl Pts',(-8.2910862664808,1.15701617944247,7.24578710321438));
#26066=CARTESIAN_POINT('Ctrl Pts',(-9.06750281866429,1.11126431092565,7.27760178551762));
#26067=CARTESIAN_POINT('Ctrl Pts',(-9.79617884906223,0.332318740478792,
7.31737013839667));
#26068=CARTESIAN_POINT('Ctrl Pts',(-9.47924265918208,-0.911764861743525,
7.36509216185153));
#26069=CARTESIAN_POINT('Ctrl Pts',(-8.2632930128867,-1.31591654596617,7.4128141853064));
#26070=CARTESIAN_POINT('Ctrl Pts',(-7.26440593819962,-0.513360169000101,
7.46053620876126));
#26071=CARTESIAN_POINT('Ctrl Pts',(-7.40088027814676,0.763184899655971,
7.50825823221612));
#26072=CARTESIAN_POINT('Ctrl Pts',(-8.35532914820361,1.23937006683617,7.54802658509517));
#26073=CARTESIAN_POINT('Ctrl Pts',(-9.09901960048363,1.01168518116112,7.57984126739841));
#26074=CARTESIAN_POINT('Ctrl Pts',(-9.65625271272335,0.469092189498902,
7.61165594970165));
#26075=CARTESIAN_POINT('Ctrl Pts',(-9.69766870777694,-0.59674535644745,
7.65142430258072));
#26076=CARTESIAN_POINT('Ctrl Pts',(-8.64400697660681,-1.33022304120803,
7.69914632603556));
#26077=CARTESIAN_POINT('Ctrl Pts',(-7.46001308842361,-0.840293863743886,
7.74686834949043));
#26078=CARTESIAN_POINT('Ctrl Pts',(-7.22969714705018,0.420192825331074,
7.7945903729453));
#26079=CARTESIAN_POINT('Ctrl Pts',(-8.16812285842602,1.2962919875284,7.84231239640014));
#26080=CARTESIAN_POINT('Ctrl Pts',(-9.20148590623969,1.03193281819899,7.88208074927922));
#26081=CARTESIAN_POINT('Ctrl Pts',(-9.61493485738788,0.373164375746146,
7.91389543158245));
#26082=CARTESIAN_POINT('Ctrl Pts',(-9.68133708809676,-0.4017592590297,7.94571011388569));
#26083=CARTESIAN_POINT('Ctrl Pts',(-9.0153030252643,-1.23490005513933,7.98547846676475));
#26084=CARTESIAN_POINT('Ctrl Pts',(-7.73856884929759,-1.10020632220151,
8.0332004902196));
#26085=CARTESIAN_POINT('Ctrl Pts',(-7.16371987671753,0.0449664965946314,
8.08092251367447));
#26086=CARTESIAN_POINT('Ctrl Pts',(-7.81425256053065,1.14890460784758,8.12864453712933));
#26087=CARTESIAN_POINT('Ctrl Pts',(-9.0971533411999,1.19746534025978,8.1763665605842));
#26088=CARTESIAN_POINT('Ctrl Pts',(-9.70567294360804,0.321435173838384,
8.21613491346324));
#26089=CARTESIAN_POINT('Ctrl Pts',(-9.58732677568735,-0.447271584630546,
8.2479495957665));
#26090=CARTESIAN_POINT('Ctrl Pts',(-9.1305274783773,-1.07675573689679,8.27976427806972));
#26091=CARTESIAN_POINT('Ctrl Pts',(-8.08173054010407,-1.27104917802106,
8.3195326309488));
#26092=CARTESIAN_POINT('Ctrl Pts',(-7.20432335123046,-0.333846327680171,
8.36725465440363));
#26093=CARTESIAN_POINT('Ctrl Pts',(-7.5188543507682,0.908305988469376,8.41497667785851));
#26094=CARTESIAN_POINT('Ctrl Pts',(-8.73310529664872,1.31753302400603,8.46269870131337));
#26095=CARTESIAN_POINT('Ctrl Pts',(-9.73507553588205,0.514882292077843,
8.51042072476822));
#26096=CARTESIAN_POINT('Ctrl Pts',(-9.62210242793819,-0.545759983091655,
8.55018907764729));
#26097=CARTESIAN_POINT('Ctrl Pts',(-9.02965411186355,-1.04966561786629,
8.58200375995052));
#26098=CARTESIAN_POINT('Ctrl Pts',(-8.27233991033248,-1.22684094384789,
8.61381844225377));
#26099=CARTESIAN_POINT('Ctrl Pts',(-7.35206163888205,-0.687570267757052,
8.65358679513281));
#26100=CARTESIAN_POINT('Ctrl Pts',(-7.30171161474597,0.595261534485032,
8.70130881858769));
#26101=CARTESIAN_POINT('Ctrl Pts',(-8.35229081295244,1.32885234309819,8.74903084204254));
#26102=CARTESIAN_POINT('Ctrl Pts',(-9.53832074872148,0.843872840804017,
8.79675286549741));
#26103=CARTESIAN_POINT('Ctrl Pts',(-9.77090660905737,-0.418702454117434,
8.84447488895226));
#26104=CARTESIAN_POINT('Ctrl Pts',(-8.99151443062067,-1.14690077270034,
8.88424324183132));
#26105=CARTESIAN_POINT('Ctrl Pts',(-8.21377858598168,-1.14035463330576,
8.91605792413455));
#26106=CARTESIAN_POINT('Ctrl Pts',(-7.52513512409165,-0.778849338222222,
8.94787260643781));
#26107=CARTESIAN_POINT('Ctrl Pts',(-7.18200506515434,0.23109458182923,8.98764095931685));
#26108=CARTESIAN_POINT('Ctrl Pts',(-7.98325750814354,1.23418335176835,9.03536298277172));
#26109=CARTESIAN_POINT('Ctrl Pts',(-9.2577345228738,1.10159200548163,9.08308500622657));
#26110=CARTESIAN_POINT('Ctrl Pts',(-9.8373617313639,-0.0411697480627666,
9.13080702968145));
#26111=CARTESIAN_POINT('Ctrl Pts',(-9.18717915050991,-1.14817253456704,
9.1785290531363));
#26112=CARTESIAN_POINT('Ctrl Pts',(-8.12131641256235,-1.1889350522776,9.21829740601535));
#26113=CARTESIAN_POINT('Ctrl Pts',(-7.53743409861438,-0.675128338195253,
9.25011208831859));
#26114=CARTESIAN_POINT('Ctrl Pts',(-7.25317049070035,0.0488261473858512,
9.28192677062183));
#26115=CARTESIAN_POINT('Ctrl Pts',(-7.6544622692538,1.03710235749143,9.3216951235009));
#26116=CARTESIAN_POINT('Ctrl Pts',(-8.91671193459285,1.27144898137521,9.36941714695573));
#26117=CARTESIAN_POINT('Ctrl Pts',(-9.7937876850699,0.337312880953606,9.41713917041064));
#26118=CARTESIAN_POINT('Ctrl Pts',(-9.48444775149291,-0.906142358160533,
9.46486119386546));
#26119=CARTESIAN_POINT('Ctrl Pts',(-8.26845641970075,-1.3179161295211,9.51258321732035));
#26120=CARTESIAN_POINT('Ctrl Pts',(-7.43572412851178,-0.651371389682554,
9.55235157019938));
#26121=CARTESIAN_POINT('Ctrl Pts',(-7.33033409569525,0.11921853820403,9.58416625250264));
#26122=CARTESIAN_POINT('Ctrl Pts',(-7.58902696279783,0.852699210401694,
9.61598093480587));
#26123=CARTESIAN_POINT('Ctrl Pts',(-8.53911350180821,1.33752962135646,9.65574928768493));
#26124=CARTESIAN_POINT('Ctrl Pts',(-9.64702206034544,0.688891676356318,
9.70347131113978));
#26125=CARTESIAN_POINT('Ctrl Pts',(-9.69912794294225,-0.591404032917394,
9.75119333459465));
#26126=CARTESIAN_POINT('Ctrl Pts',(-8.65162203056557,-1.32937658641912,
9.7989153580495));
#26127=CARTESIAN_POINT('Ctrl Pts',(-7.46260964658798,-0.845184363720304,
9.84663738150439));
#26128=CARTESIAN_POINT('Ctrl Pts',(-7.26895926387031,0.203731499573094,
9.8864057343834));
#26129=CARTESIAN_POINT('Ctrl Pts',(-7.69343845327961,0.855447168968696,
9.91822041668668));
#26130=CARTESIAN_POINT('Ctrl Pts',(-8.36897674068639,1.24088707119054,9.95003509898991));
#26131=CARTESIAN_POINT('Ctrl Pts',(-9.40469716198697,0.985920077451709,
9.98980345186895));
#26132=CARTESIAN_POINT('Ctrl Pts',(-9.81816654914519,-0.229495745901432,
10.0375254753238));
#26133=CARTESIAN_POINT('Ctrl Pts',(-9.01990129213503,-1.23181540830278,
10.0852474987787));
#26134=CARTESIAN_POINT('Ctrl Pts',(-7.7448815766716,-1.10454855729489,10.1329695222335));
#26135=CARTESIAN_POINT('Ctrl Pts',(-7.16248378137103,0.0395691664569845,
10.1806915456884));
#26136=CARTESIAN_POINT('Ctrl Pts',(-7.70231858265184,0.959516635784098,
10.2204598985675));
#26137=CARTESIAN_POINT('Ctrl Pts',(-8.44973620845025,1.17465098595439,10.2522745808707));
#26138=CARTESIAN_POINT('Ctrl Pts',(-9.21279948735437,1.02415072560454,10.2840892631739));
#26139=CARTESIAN_POINT('Ctrl Pts',(-9.82924696386352,0.153681043363534,
10.323857616053));
#26140=CARTESIAN_POINT('Ctrl Pts',(-9.34671359928637,-1.03600551613187,
10.3715796395079));
#26141=CARTESIAN_POINT('Ctrl Pts',(-8.08722621411818,-1.27172495272547,
10.4193016629627));
#26142=CARTESIAN_POINT('Ctrl Pts',(-7.20625633934821,-0.341260441884946,
10.4670236864176));
#26143=CARTESIAN_POINT('Ctrl Pts',(-7.51438819018325,0.905032990768513,
10.5147457098724));
#26144=CARTESIAN_POINT('Ctrl Pts',(-8.52454229492433,1.24754378427726,10.5545140627515));
#26145=CARTESIAN_POINT('Ctrl Pts',(-9.23053722819551,0.921220248238709,
10.5863287450547));
#26146=CARTESIAN_POINT('Ctrl Pts',(-9.70913721769566,0.308147702753446,
10.618143427358));
#26147=CARTESIAN_POINT('Ctrl Pts',(-9.60579769849225,-0.753476478756218,
10.657911780237));
#26148=CARTESIAN_POINT('Ctrl Pts',(-8.46249339286839,-1.33746947744375,
10.7056338036919));
#26149=CARTESIAN_POINT('Ctrl Pts',(-7.35577561545489,-0.691677028321873,
10.7533558271468));
#26150=CARTESIAN_POINT('Ctrl Pts',(-7.29832254473717,0.588389872605941,
10.8010778506016));
#26151=CARTESIAN_POINT('Ctrl Pts',(-8.34677181075405,1.32929924247705,10.8487998740565));
#26152=CARTESIAN_POINT('Ctrl Pts',(-9.33480180140853,0.927401622973597,
10.8885682269355));
#26153=CARTESIAN_POINT('Ctrl Pts',(-9.6552062007518,0.218700757404208,10.9203829092388));
#26154=CARTESIAN_POINT('Ctrl Pts',(-9.61602858438752,-0.558075278756368,
10.952197591542));
#26155=CARTESIAN_POINT('Ctrl Pts',(-8.84327939879723,-1.29331922138004,
10.9919659444211));
#26156=CARTESIAN_POINT('Ctrl Pts',(-7.59655740834266,-0.986925950743844,
11.0396879678759));
#26157=CARTESIAN_POINT('Ctrl Pts',(-7.18212680537146,0.22555885390601,11.0874099913308));
#26158=CARTESIAN_POINT('Ctrl Pts',(-7.97619852913042,1.23120403174577,11.1351320147857));
#26159=CARTESIAN_POINT('Ctrl Pts',(-9.25385315598159,1.10554094146089,11.1828540382405));
#26160=CARTESIAN_POINT('Ctrl Pts',(-9.73810097369181,0.155157329418831,
11.2226223911196));
#26161=CARTESIAN_POINT('Ctrl Pts',(-9.5167198222586,-0.590433900255586,
11.2544370734228));
#26162=CARTESIAN_POINT('Ctrl Pts',(-8.9788634278258,-1.15224026809512,11.286251755726));
#26163=CARTESIAN_POINT('Ctrl Pts',(-7.91341467193457,-1.20267743261775,
11.3260201086051));
#26164=CARTESIAN_POINT('Ctrl Pts',(-7.17104368741518,-0.155262577310692,
11.3737421320599));
#26165=CARTESIAN_POINT('Ctrl Pts',(-7.65093242556789,1.03283629280916,11.4214641555148));
#26166=CARTESIAN_POINT('Ctrl Pts',(-8.90942425196499,1.27381440193424,11.4691861789697));
#26167=CARTESIAN_POINT('Ctrl Pts',(-9.79343609406736,0.342838773468614,
11.5169082024246));
#26168=CARTESIAN_POINT('Ctrl Pts',(-9.53783414362817,-0.692725131815334,
11.5566765553036));
#26169=CARTESIAN_POINT('Ctrl Pts',(-8.88258928253219,-1.11173595265966,
11.5884912376068));
#26170=CARTESIAN_POINT('Ctrl Pts',(-8.10825553036941,-1.18469577885752,
11.6203059199101));
#26171=CARTESIAN_POINT('Ctrl Pts',(-7.2695063969436,-0.525738382531577,
11.6600742727892));
#26172=CARTESIAN_POINT('Ctrl Pts',(-7.39338734316738,0.752090271450184,
11.707796296244));
#26173=CARTESIAN_POINT('Ctrl Pts',(-8.53365284957409,1.33661289811649,11.7555183196989));
#26174=CARTESIAN_POINT('Ctrl Pts',(-9.64305837098596,0.695448710683353,
11.8032403431537));
#26175=CARTESIAN_POINT('Ctrl Pts',(-9.70247752610808,-0.586995019769853,
11.8509623666086));
#26176=CARTESIAN_POINT('Ctrl Pts',(-8.83163006088557,-1.20290869173268,
11.8907307194876));
#26177=CARTESIAN_POINT('Ctrl Pts',(-8.06194900837746,-1.09107411126975,
11.9225454017909));
#26178=CARTESIAN_POINT('Ctrl Pts',(-7.42862046025152,-0.639619965086561,
11.9543600840941));
#26179=CARTESIAN_POINT('Ctrl Pts',(-7.22545558163593,0.407494637567971,
11.9941284369732));
#26180=CARTESIAN_POINT('Ctrl Pts',(-8.15519732002207,1.29280410757092,12.0418504604281));
#26181=CARTESIAN_POINT('Ctrl Pts',(-9.39996773290423,0.988799592145459,
12.0895724838829));
#26182=CARTESIAN_POINT('Ctrl Pts',(-9.81945912529353,-0.221943608495,12.1372945073378));
#26183=CARTESIAN_POINT('Ctrl Pts',(-9.02531914992084,-1.23067263915149,
12.1850165307926));
#26184=CARTESIAN_POINT('Ctrl Pts',(-7.9637585258431,-1.12668225304343,12.2247848836717));
#26185=CARTESIAN_POINT('Ctrl Pts',(-7.45485568350695,-0.538520886546523,
12.2565995659749));
#26186=CARTESIAN_POINT('Ctrl Pts',(-7.27127580064357,0.217266333896634,
12.2884142482782));
#26187=CARTESIAN_POINT('Ctrl Pts',(-7.80273670592906,1.14207672805771,12.3281826011572));
#26188=CARTESIAN_POINT('Ctrl Pts',(-9.08509631350376,1.20328452686656,12.3759046246121));
#26189=CARTESIAN_POINT('Ctrl Pts',(-9.82755432320141,0.158953051700929,
12.4236266480669));
#26190=CARTESIAN_POINT('Ctrl Pts',(-9.35263231865442,-1.03113989247735,
12.4713486715218));
#26191=CARTESIAN_POINT('Ctrl Pts',(-8.09207117683376,-1.27440551994248,
12.5190706949767));
#26192=CARTESIAN_POINT('Ctrl Pts',(-7.35730114822946,-0.501205698382691,
12.5588390478557));
#26193=CARTESIAN_POINT('Ctrl Pts',(-7.35726327203958,0.276557694007757,
12.590653730159));
#26194=CARTESIAN_POINT('Ctrl Pts',(-7.71292602816593,0.968236737988355,
12.6224684124622));
#26195=CARTESIAN_POINT('Ctrl Pts',(-8.71992905550032,1.31990399824245,12.6622367653413));
#26196=CARTESIAN_POINT('Ctrl Pts',(-9.72976473982391,0.527171730423799,
12.7099587887961));
#26197=CARTESIAN_POINT('Ctrl Pts',(-9.60796699733264,-0.748382045827872,
12.757680812251));
#26198=CARTESIAN_POINT('Ctrl Pts',(-8.47015291907083,-1.3376623267597,12.8054028357058));
#26199=CARTESIAN_POINT('Ctrl Pts',(-7.35768579595222,-0.696874173190761,
12.8531248591607));
#26200=CARTESIAN_POINT('Ctrl Pts',(-7.30790187209926,0.368605305692363,
12.8928932120397));
#26201=CARTESIAN_POINT('Ctrl Pts',(-7.81674742644668,0.956816235375078,
12.924707894343));
#26202=CARTESIAN_POINT('Ctrl Pts',(-8.53826958993604,1.24719816244858,12.9565225766462));
#26203=CARTESIAN_POINT('Ctrl Pts',(-9.5299074510817,0.854286834872281,12.9962909295253));
#26204=CARTESIAN_POINT('Ctrl Pts',(-9.77493102244612,-0.405933783610824,
13.0440129529801));
#26205=CARTESIAN_POINT('Ctrl Pts',(-8.84825311836191,-1.29088586608074,
13.091734976435));
#26206=CARTESIAN_POINT('Ctrl Pts',(-7.60222377322338,-0.992083260269492,
13.1394569998899));
#26207=CARTESIAN_POINT('Ctrl Pts',(-7.18017100334371,0.220378704994195,
13.1871790233447));
#26208=CARTESIAN_POINT('Ctrl Pts',(-7.83964251650143,1.05872367117979,13.2269473762238));
#26209=CARTESIAN_POINT('Ctrl Pts',(-8.60931267292587,1.17063321629039,13.258762058527));
#26210=CARTESIAN_POINT('Ctrl Pts',(-9.34495698076375,0.918158765458134,
13.2905767408303));
#26211=CARTESIAN_POINT('Ctrl Pts',(-9.83781280395867,-0.0277894871107221,
13.3303450937093));
#26212=CARTESIAN_POINT('Ctrl Pts',(-9.19857689854507,-1.14114927397397,
13.3780671171642));
#26213=CARTESIAN_POINT('Ctrl Pts',(-7.91876815696661,-1.20409139949583,
13.425789140619));
#26214=CARTESIAN_POINT('Ctrl Pts',(-7.17195457572563,-0.162870192902413,
13.4735111640739));
#26215=CARTESIAN_POINT('Ctrl Pts',(-7.64606408151493,1.0301984280471,13.5212331875288));
#26216=CARTESIAN_POINT('Ctrl Pts',(-8.69330304862208,1.23272127803588,13.5610015404078));
#26217=CARTESIAN_POINT('Ctrl Pts',(-9.34858871730795,0.813774278533218,
13.5928162227111));
#26218=CARTESIAN_POINT('Ctrl Pts',(-9.73973345489619,0.14152306787283,13.6246309050143));
#26219=CARTESIAN_POINT('Ctrl Pts',(-9.49354329942793,-0.896318618679486,
13.6643992578933));
#26220=CARTESIAN_POINT('Ctrl Pts',(-8.28167117590845,-1.32006207173866,
13.7121212813482));
#26221=CARTESIAN_POINT('Ctrl Pts',(-7.27262985904281,-0.530310372124225,
13.7598433048031));
#26222=CARTESIAN_POINT('Ctrl Pts',(-7.38909870290544,0.745741011870611,
13.8075653282579));
#26223=CARTESIAN_POINT('Ctrl Pts',(-8.52824524889072,1.33780325905745,13.8552873517128));
#26224=CARTESIAN_POINT('Ctrl Pts',(-9.45272962828058,0.805775448450338,
13.8950557045918));
#26225=CARTESIAN_POINT('Ctrl Pts',(-9.67418339754811,0.0602057843313418,
13.9268703868951));
#26226=CARTESIAN_POINT('Ctrl Pts',(-9.53014810293605,-0.704104185434403,
13.9586850691983));
#26227=CARTESIAN_POINT('Ctrl Pts',(-8.66492803462685,-1.3278983761658,13.9984534220774));
#26228=CARTESIAN_POINT('Ctrl Pts',(-7.47119930507729,-0.855453376168864,
14.0461754455322));
#26229=CARTESIAN_POINT('Ctrl Pts',(-7.22482635377211,0.401993439824162,
14.0938974689871));
#26230=CARTESIAN_POINT('Ctrl Pts',(-8.14779983483422,1.29080842588256,14.141619492442));
#26231=CARTESIAN_POINT('Ctrl Pts',(-9.39665704501126,0.993237885736016,
14.1893415158968));
#26232=CARTESIAN_POINT('Ctrl Pts',(-9.74770684130611,-0.0139805610353641,
14.2291098687759));
#26233=CARTESIAN_POINT('Ctrl Pts',(-9.42737146932972,-0.722712629900664,
14.2609245510791));
#26234=CARTESIAN_POINT('Ctrl Pts',(-8.81837239209062,-1.20648532435468,
14.2927392333824));
#26235=CARTESIAN_POINT('Ctrl Pts',(-7.75591144824565,-1.11213649395108,
14.3325075862614));
#26236=CARTESIAN_POINT('Ctrl Pts',(-7.16226094067262,0.0261831591490891,
14.3802296097163));
#26237=CARTESIAN_POINT('Ctrl Pts',(-7.79866153250768,1.1383281195285,14.4279516331712));
#26238=CARTESIAN_POINT('Ctrl Pts',(-9.07819620829063,1.20661530463999,14.475673656626));
#26239=CARTESIAN_POINT('Ctrl Pts',(-9.82795448646243,0.164475639288861,
14.5233956800809));
#26240=CARTESIAN_POINT('Ctrl Pts',(-9.4344352553121,-0.826921139859,14.5631640329599));
#26241=CARTESIAN_POINT('Ctrl Pts',(-8.72847210856683,-1.15331343665297,
14.5949787152632));
#26242=CARTESIAN_POINT('Ctrl Pts',(-7.95139225442456,-1.12071288000722,
14.6267933975664));
#26243=CARTESIAN_POINT('Ctrl Pts',(-7.20963308932079,-0.354215456745463,
14.6665617504455));
#26244=CARTESIAN_POINT('Ctrl Pts',(-7.505461483611,0.895055578304256,14.7142837739003));
#26245=CARTESIAN_POINT('Ctrl Pts',(-8.71439455658622,1.31973540062164,14.7620057973552));
#26246=CARTESIAN_POINT('Ctrl Pts',(-9.72672576989096,0.534205235745722,
14.80972782081));
#26247=CARTESIAN_POINT('Ctrl Pts',(-9.61188293513649,-0.744467389276269,
14.8574498442649));
#26248=CARTESIAN_POINT('Ctrl Pts',(-8.66563268745192,-1.23674315419584,
14.897218197144));
#26249=CARTESIAN_POINT('Ctrl Pts',(-7.91819411292805,-1.02168160289173,
14.9290328794472));
#26250=CARTESIAN_POINT('Ctrl Pts',(-7.35185474755516,-0.488600347920775,
14.9608475617504));
#26251=CARTESIAN_POINT('Ctrl Pts',(-7.29240003379382,0.57638326010828,15.0006159146295));
#26252=CARTESIAN_POINT('Ctrl Pts',(-8.33349294198175,1.32759435244437,15.0483379380844));
#26253=CARTESIAN_POINT('Ctrl Pts',(-9.52561167002035,0.857780428739866,
15.0960599615392));
#26254=CARTESIAN_POINT('Ctrl Pts',(-9.7772346429653,-0.398626319625639,
15.1437819849941));
#26255=CARTESIAN_POINT('Ctrl Pts',(-8.85377588165687,-1.29048754584707,
15.1915040084489));
#26256=CARTESIAN_POINT('Ctrl Pts',(-7.81608520647529,-1.04366103090559,
15.231272361328));
#26257=CARTESIAN_POINT('Ctrl Pts',(-7.39154272749966,-0.391986857252505,
15.2630870436313));
#26258=CARTESIAN_POINT('Ctrl Pts',(-7.31203017292505,0.381701814578057,
15.2949017259345));
#26259=CARTESIAN_POINT('Ctrl Pts',(-7.96386448015173,1.22599852877905,15.3346700788135));
#26260=CARTESIAN_POINT('Ctrl Pts',(-9.24269458235218,1.11294042920609,15.3823921022684));
#26261=CARTESIAN_POINT('Ctrl Pts',(-9.83685155659984,-0.0223381454316971,
15.4301141257232));
#26262=CARTESIAN_POINT('Ctrl Pts',(-9.20509698430864,-1.13712765515967,
15.4778361491781));
#26263=CARTESIAN_POINT('Ctrl Pts',(-7.92321163699227,-1.2074086266698,15.525558172633));
#26264=CARTESIAN_POINT('Ctrl Pts',(-7.29993080976771,-0.341792293020232,
15.565326525512));
#26265=CARTESIAN_POINT('Ctrl Pts',(-7.4052713667291,0.428787139267935,15.5971412078153));
#26266=CARTESIAN_POINT('Ctrl Pts',(-7.85129778173277,1.06595545650788,15.6289558901185));
#26267=CARTESIAN_POINT('Ctrl Pts',(-8.89676621122576,1.27788697335264,15.6687242429976));
#26268=CARTESIAN_POINT('Ctrl Pts',(-9.78971211575288,0.355837225553599,
15.7164462664524));
#26269=CARTESIAN_POINT('Ctrl Pts',(-9.49661412050732,-0.891752812389575,
15.7641682899073));
#26270=CARTESIAN_POINT('Ctrl Pts',(-8.28879921167558,-1.32093775301506,
15.8118903133622));
#26271=CARTESIAN_POINT('Ctrl Pts',(-7.27465414055275,-0.536397493183267,
15.859612336817));
#26272=CARTESIAN_POINT('Ctrl Pts',(-7.38611196025228,0.74057287343298,15.9073343602719));
#26273=CARTESIAN_POINT('Ctrl Pts',(-8.52084029087267,1.33755299057858,15.9550563837267));
#26274=CARTESIAN_POINT('Ctrl Pts',(-9.63603663835765,0.705608630834653,
16.0027784071816));
#26275=CARTESIAN_POINT('Ctrl Pts',(-9.7085623613501,-0.57389414645679,16.0505004306365));
#26276=CARTESIAN_POINT('Ctrl Pts',(-8.66937749713867,-1.32730170138437,
16.0982224540913));
#26277=CARTESIAN_POINT('Ctrl Pts',(-7.67643438972821,-0.937451486116148,
16.1379908069704));
#26278=CARTESIAN_POINT('Ctrl Pts',(-7.34753951593156,-0.232645704807778,
16.1698054892736));
#26279=CARTESIAN_POINT('Ctrl Pts',(-7.37729180242736,0.544531299390573,
16.2016201715769));
#26280=CARTESIAN_POINT('Ctrl Pts',(-8.14111244251711,1.28907723916828,16.2413885244559));
#26281=CARTESIAN_POINT('Ctrl Pts',(-9.39143791719134,0.997777280360524,
16.2891105479108));
#26282=CARTESIAN_POINT('Ctrl Pts',(-9.82050642331186,-0.20960406273945,
16.3368325713656));
#26283=CARTESIAN_POINT('Ctrl Pts',(-9.03865128869567,-1.22478015611096,
16.3845545948205));
#26284=CARTESIAN_POINT('Ctrl Pts',(-7.75957206601839,-1.1145762256531,16.4322766182754));
#26285=CARTESIAN_POINT('Ctrl Pts',(-7.26386561656706,-0.170118697936401,
16.4720449711544));
#26286=CARTESIAN_POINT('Ctrl Pts',(-7.47621443170938,0.578095434489346,
16.5038596534576));
#26287=CARTESIAN_POINT('Ctrl Pts',(-8.0072372736111,1.14636498887337,16.5356743357609));
#26288=CARTESIAN_POINT('Ctrl Pts',(-9.07199831336541,1.2096831857704,16.5754426886399));
#26289=CARTESIAN_POINT('Ctrl Pts',(-9.82698149184862,0.171322491752237,
16.6231647120948));
#26290=CARTESIAN_POINT('Ctrl Pts',(-9.36149575518903,-1.02249284858247,
16.6708867355496));
#26291=CARTESIAN_POINT('Ctrl Pts',(-8.10601012202046,-1.27867249171228,
16.7186087590046));
#26292=CARTESIAN_POINT('Ctrl Pts',(-7.21080449715534,-0.358455431482571,
16.7663307824594));
#26293=CARTESIAN_POINT('Ctrl Pts',(-7.45386450952434,0.680123780107074,
16.8060991353384));
#26294=CARTESIAN_POINT('Ctrl Pts',(-8.10399429361696,1.10702794383478,16.8379138176417));
#26295=CARTESIAN_POINT('Ctrl Pts',(-8.87738910627695,1.18934657651432,16.8697284999449));
#26296=CARTESIAN_POINT('Ctrl Pts',(-9.72404578490763,0.540580495017656,
16.909496852824));
#26297=CARTESIAN_POINT('Ctrl Pts',(-9.6156268841698,-0.738652830313552,
16.9572188762788));
#26298=CARTESIAN_POINT('Ctrl Pts',(-8.48251348594472,-1.33692212764018,
17.0049408997337));
#26299=CARTESIAN_POINT('Ctrl Pts',(-7.36543538804804,-0.709221044626535,
17.0526629231886));
#26300=CARTESIAN_POINT('Ctrl Pts',(-7.29051177992318,0.572410341860231,
17.1003849466434));
#26301=CARTESIAN_POINT('Ctrl Pts',(-8.15384722142223,1.19881027348046,17.1401532995225));
#26302=CARTESIAN_POINT('Ctrl Pts',(-8.92482442462193,1.09629174757539,17.1719679818257));
#26303=CARTESIAN_POINT('Ctrl Pts',(-9.5635661681587,0.652529557847061,17.203782664129));
#26304=CARTESIAN_POINT('Ctrl Pts',(-9.77937911551377,-0.392051569085598,
17.243551017008));
#26305=CARTESIAN_POINT('Ctrl Pts',(-8.86041155411601,-1.28853981713131,
17.2912730404629));
#26306=CARTESIAN_POINT('Ctrl Pts',(-7.61205578954346,-0.99961074064383,
17.3389950639177));
#26307=CARTESIAN_POINT('Ctrl Pts',(-7.17795336035532,0.205970947653733,
17.3867170873726));
#26308=CARTESIAN_POINT('Ctrl Pts',(-7.95983654202789,1.22422987739285,17.4344391108275));
#26309=CARTESIAN_POINT('Ctrl Pts',(-9.02257711199641,1.13308471878594,17.4742074637065));
#26310=CARTESIAN_POINT('Ctrl Pts',(-9.53855547075963,0.551120605403174,
17.5060221460098));
#26311=CARTESIAN_POINT('Ctrl Pts',(-9.73126178565995,-0.202391287120677,
17.537836828313));
#26312=CARTESIAN_POINT('Ctrl Pts',(-9.21102362412759,-1.13356109670459,
17.5776051811921));
#26313=CARTESIAN_POINT('Ctrl Pts',(-7.92949798477055,-1.21027220049513,
17.6253272046469));
#26314=CARTESIAN_POINT('Ctrl Pts',(-7.17446499892724,-0.174995756025178,
17.6730492281018));
#26315=CARTESIAN_POINT('Ctrl Pts',(-7.63496028961901,1.0207534707931,17.7207712515566));
#26316=CARTESIAN_POINT('Ctrl Pts',(-8.89248740265649,1.27924547792269,17.7684932750115));
#26317=CARTESIAN_POINT('Ctrl Pts',(-9.63655413093407,0.514987888581546,
17.8082616278906));
#26318=CARTESIAN_POINT('Ctrl Pts',(-9.64599762203821,-0.262718171863597,
17.8400763101938));
#26319=CARTESIAN_POINT('Ctrl Pts',(-9.29872545955566,-0.958647723716373,
17.871890992497));
#26320=CARTESIAN_POINT('Ctrl Pts',(-8.29604883794672,-1.32246711774878,
17.9116593453761));
#26321=CARTESIAN_POINT('Ctrl Pts',(-7.2767003590985,-0.542004923633025,
17.959381368831));
#26322=CARTESIAN_POINT('Ctrl Pts',(-7.38306371835046,0.734928497495294,
18.0071033922858));
#26323=CARTESIAN_POINT('Ctrl Pts',(-8.51366833289497,1.33792545582631,18.0548254157407));
#26324=CARTESIAN_POINT('Ctrl Pts',(-9.63380326103061,0.710637403537144,
18.1025474391955));
#26325=CARTESIAN_POINT('Ctrl Pts',(-9.69646855898839,-0.354162117230549,
18.1423157920746));
#26326=CARTESIAN_POINT('Ctrl Pts',(-9.19477354323534,-0.948483585079254,
18.1741304743779));
#26327=CARTESIAN_POINT('Ctrl Pts',(-8.47681577631781,-1.24756976145674,
18.2059451566811));
#26328=CARTESIAN_POINT('Ctrl Pts',(-7.48049888881085,-0.866679201500626,
18.2457135095602));
#26329=CARTESIAN_POINT('Ctrl Pts',(-7.22025318433492,0.39048615400201,18.293435533015));
#26330=CARTESIAN_POINT('Ctrl Pts',(-8.13616145741442,1.28657998920588,18.3411575564699));
#26331=CARTESIAN_POINT('Ctrl Pts',(-9.38571315465714,1.00286766641441,18.3888795799247));
#26332=CARTESIAN_POINT('Ctrl Pts',(-9.82239755933068,-0.204401685672783,
18.4366016033796));
#26333=CARTESIAN_POINT('Ctrl Pts',(-9.17311251037952,-1.05066044291179,
18.4763699562587));
#26334=CARTESIAN_POINT('Ctrl Pts',(-8.40485197615202,-1.17186954952435,
18.5081846385619));
#26335=CARTESIAN_POINT('Ctrl Pts',(-7.66620824815671,-0.928309825697792,
18.5399993208651));
#26336=CARTESIAN_POINT('Ctrl Pts',(-7.16194896079103,0.0116090697930224,
18.5797676737441));
#26337=CARTESIAN_POINT('Ctrl Pts',(-7.78767408330682,1.1326178248109,18.627489697199));
#26338=CARTESIAN_POINT('Ctrl Pts',(-9.06662806970791,1.2110322804595,18.6752117206539));
#26339=CARTESIAN_POINT('Ctrl Pts',(-9.82597869561601,0.178918549750082,
18.7229337441087));
#26340=CARTESIAN_POINT('Ctrl Pts',(-9.36633182960527,-1.01979631056521,
18.7706557675636));
#26341=CARTESIAN_POINT('Ctrl Pts',(-8.32161858315476,-1.23496878019377,
18.8104241204427));
#26342=CARTESIAN_POINT('Ctrl Pts',(-7.66131443880895,-0.823976891055952,
18.8422388027459));
#26343=CARTESIAN_POINT('Ctrl Pts',(-7.26206866174134,-0.156505014891145,
18.8740534850491));
#26344=CARTESIAN_POINT('Ctrl Pts',(-7.49569002828134,0.884237996659342,
18.9138218379282));
#26345=CARTESIAN_POINT('Ctrl Pts',(-8.70234913605313,1.32260582783032,18.961543861383));
#26346=CARTESIAN_POINT('Ctrl Pts',(-9.72086726104124,0.545114377551589,
19.009265884838));
#26347=CARTESIAN_POINT('Ctrl Pts',(-9.61983842839294,-0.732252171704951,
19.0569879082928));
#26348=CARTESIAN_POINT('Ctrl Pts',(-8.48793508632651,-1.33804700660616,
19.1047099317477));
#26349=CARTESIAN_POINT('Ctrl Pts',(-7.55708441199681,-0.817238038658018,
19.1444782846267));
#26350=CARTESIAN_POINT('Ctrl Pts',(-7.32663054276847,-0.0744009702944177,
19.1762929669299));
#26351=CARTESIAN_POINT('Ctrl Pts',(-7.46141238152576,0.691594951312568,
19.2081076492332));
#26352=CARTESIAN_POINT('Ctrl Pts',(-8.31902553728147,1.32580677244966,19.2478760021122));
#26353=CARTESIAN_POINT('Ctrl Pts',(-9.51838032879036,0.86783227331379,19.2955980255671));
#26354=CARTESIAN_POINT('Ctrl Pts',(-9.77994177049436,-0.386543164264433,
19.343320049022));
#26355=CARTESIAN_POINT('Ctrl Pts',(-8.86778436426511,-1.28645482239925,
19.3910420724768));
#26356=CARTESIAN_POINT('Ctrl Pts',(-7.61541990833944,-1.00400867300409,
19.4387640959317));
#26357=CARTESIAN_POINT('Ctrl Pts',(-7.25221532801234,-0.00110918061983182,
19.4785324488107));
#26358=CARTESIAN_POINT('Ctrl Pts',(-7.56395646468766,0.711444929382833,
19.510347131114));
#26359=CARTESIAN_POINT('Ctrl Pts',(-8.16706066797269,1.20254697168893,19.5421618134172));
#26360=CARTESIAN_POINT('Ctrl Pts',(-9.23058489499091,1.12105355145988,19.5819301662963));
#26361=CARTESIAN_POINT('Ctrl Pts',(-9.83795787438773,-0.0100037510994853,
19.6296521897511));
#26362=CARTESIAN_POINT('Ctrl Pts',(-9.2150531670274,-1.12976348056569,19.677374213206));
#26363=CARTESIAN_POINT('Ctrl Pts',(-7.93643786504349,-1.21351929062353,
19.7250962366609));
#26364=CARTESIAN_POINT('Ctrl Pts',(-7.1741316504696,-0.180522779014628,
19.7728182601157));
#26365=CARTESIAN_POINT('Ctrl Pts',(-7.55563298498379,0.815560395604377,
19.8125866129948));
#26366=CARTESIAN_POINT('Ctrl Pts',(-8.25759739373146,1.15046615074881,19.844401295298));
#26367=CARTESIAN_POINT('Ctrl Pts',(-9.03501466770616,1.12726532957784,19.8762159776013));
#26368=CARTESIAN_POINT('Ctrl Pts',(-9.7859889682652,0.369794169139932,19.9159843304803));
#26369=CARTESIAN_POINT('Ctrl Pts',(-9.50528984170661,-0.882963013287452,
19.9637063539352));
#26370=CARTESIAN_POINT('Ctrl Pts',(-8.30158089336006,-1.32223160294103,
20.0114283773901));
#26371=CARTESIAN_POINT('Ctrl Pts',(-7.27982416395186,-0.549001163747792,
20.0591504008449));
#26372=CARTESIAN_POINT('Ctrl Pts',(-7.37919540779779,0.730966770878209,
20.1068724242998));
#26373=CARTESIAN_POINT('Ctrl Pts',(-8.31942329015859,1.23464969517342,20.1466407771788));
#26374=CARTESIAN_POINT('Ctrl Pts',(-9.06940798351601,1.02864276396269,20.1784554594821));
#26375=CARTESIAN_POINT('Ctrl Pts',(-9.6421525700082,0.502449325556989,20.2102701417853));
#26376=CARTESIAN_POINT('Ctrl Pts',(-9.71448195986604,-0.561737414803009,
20.2500384946644));
#26377=CARTESIAN_POINT('Ctrl Pts',(-8.68254968740398,-1.325483670326,20.2977605181192));
#26378=CARTESIAN_POINT('Ctrl Pts',(-7.48483661646242,-0.870120599928743,
20.3454825415741));
#26379=CARTESIAN_POINT('Ctrl Pts',(-7.21803807964812,0.38315138449426,20.3932045650289));
#26380=CARTESIAN_POINT('Ctrl Pts',(-8.13064396047136,1.28611487437685,20.4409265884838));
#26381=CARTESIAN_POINT('Ctrl Pts',(-9.17124354215662,1.05185546775307,20.4806949413628));
#26382=CARTESIAN_POINT('Ctrl Pts',(-9.6036359628206,0.405362861043841,20.5125096236661));
#26383=CARTESIAN_POINT('Ctrl Pts',(-9.692498679558,-0.367307387866645,20.5443243059693));
#26384=CARTESIAN_POINT('Ctrl Pts',(-9.05092306150429,-1.21942573957269,
20.5840926588484));
#26385=CARTESIAN_POINT('Ctrl Pts',(-7.77081777281899,-1.12183984072394,
20.6318146823033));
#26386=CARTESIAN_POINT('Ctrl Pts',(-7.16297774725796,0.00616841700814254,
20.6795367057581));
#26387=CARTESIAN_POINT('Ctrl Pts',(-7.78119991790399,1.12852017733444,20.727258729213));
#26388=CARTESIAN_POINT('Ctrl Pts',(-9.06215112949211,1.21429051780881,20.7749807526679));
#26389=CARTESIAN_POINT('Ctrl Pts',(-9.69583702513552,0.356288685259583,
20.8147491055469));
#26390=CARTESIAN_POINT('Ctrl Pts',(-9.59984873958507,-0.415528744586615,
20.8465637878501));
#26391=CARTESIAN_POINT('Ctrl Pts',(-9.16150960230265,-1.05800418902307,
20.8783784701533));
#26392=CARTESIAN_POINT('Ctrl Pts',(-8.11879282938344,-1.28265211460481,
20.9181468230325));
#26393=CARTESIAN_POINT('Ctrl Pts',(-7.21455735142713,-0.371306538997314,
20.9658688464872));
#26394=CARTESIAN_POINT('Ctrl Pts',(-7.49290834699324,0.879450371618512,
21.0135908699422));
#26395=CARTESIAN_POINT('Ctrl Pts',(-8.69477202257272,1.32374287831705,21.061312893397));
#26396=CARTESIAN_POINT('Ctrl Pts',(-9.71961335617614,0.550507598009665,
21.1090349168519));
#26397=CARTESIAN_POINT('Ctrl Pts',(-9.63746790001045,-0.512966465156227,
21.1488032697309));
#26398=CARTESIAN_POINT('Ctrl Pts',(-9.05989255998547,-1.03385284679082,
21.1806179520342));
#26399=CARTESIAN_POINT('Ctrl Pts',(-8.30803898706308,-1.23293097432144,
21.2124326343374));
#26400=CARTESIAN_POINT('Ctrl Pts',(-7.37249856131074,-0.720594101962636,
21.2522009872164));
#26401=CARTESIAN_POINT('Ctrl Pts',(-7.28494168448683,0.56023623461398,21.2999230106713));
#26402=CARTESIAN_POINT('Ctrl Pts',(-8.31378943939285,1.32400611056527,21.3476450341262));
#26403=CARTESIAN_POINT('Ctrl Pts',(-9.51339405973382,0.873649717202732,
21.395367057581));
#26404=CARTESIAN_POINT('Ctrl Pts',(-9.78252217127443,-0.381644119854083,
21.4430890810359));
#26405=CARTESIAN_POINT('Ctrl Pts',(-9.02459072764576,-1.1321538704598,21.482857433915));
#26406=CARTESIAN_POINT('Ctrl Pts',(-8.24699247568435,-1.14818055208414,
21.5146721162182));
#26407=CARTESIAN_POINT('Ctrl Pts',(-7.54814809080176,-0.806812097631549,
21.5464867985215));
#26408=CARTESIAN_POINT('Ctrl Pts',(-7.17585375677161,0.192748749863114,
21.5862551514005));
#26409=CARTESIAN_POINT('Ctrl Pts',(-7.94765887705949,1.21866756442476,21.6339771748554));
#26410=CARTESIAN_POINT('Ctrl Pts',(-9.22544694344921,1.12311766344225,21.6816991983102));
#26411=CARTESIAN_POINT('Ctrl Pts',(-9.83799322280595,-0.00234187907010109,
21.7294212217651));
#26412=CARTESIAN_POINT('Ctrl Pts',(-9.22020994520899,-1.12774686381815,
21.7771432452199));
#26413=CARTESIAN_POINT('Ctrl Pts',(-8.15597905940294,-1.19942378263886,
21.816911598099));
#26414=CARTESIAN_POINT('Ctrl Pts',(-7.55743187924388,-0.702777863395583,
21.8487262804022));
#26415=CARTESIAN_POINT('Ctrl Pts',(-7.25227867894974,0.0126223185498688,
21.8805409627055));
#26416=CARTESIAN_POINT('Ctrl Pts',(-7.62472145204494,1.0121278661905,21.9203093155845));
#26417=CARTESIAN_POINT('Ctrl Pts',(-8.87963869892395,1.28300654984747,21.9680313390394));
#26418=CARTESIAN_POINT('Ctrl Pts',(-9.78345388032542,0.374716814105572,
22.0157533624942));
#26419=CARTESIAN_POINT('Ctrl Pts',(-9.51032957548044,-0.877191824848875,
22.0634753859492));
#26420=CARTESIAN_POINT('Ctrl Pts',(-8.30680015382619,-1.32408050112826,
22.1111974094039));
#26421=CARTESIAN_POINT('Ctrl Pts',(-7.45507531503048,-0.681982566251019,
22.150965762283));
#26422=CARTESIAN_POINT('Ctrl Pts',(-7.32736698200152,0.0852243664941577,
22.1827804445863));
#26423=CARTESIAN_POINT('Ctrl Pts',(-7.56466512489233,0.825903438264024,
22.2145951268895));
#26424=CARTESIAN_POINT('Ctrl Pts',(-8.50028162665128,1.33810136937232,22.2543634797686));
#26425=CARTESIAN_POINT('Ctrl Pts',(-9.62654717627403,0.721888362768944,
22.3020855032234));
#26426=CARTESIAN_POINT('Ctrl Pts',(-9.7157855740631,-0.55635599358315,22.3498075266783));
#26427=CARTESIAN_POINT('Ctrl Pts',(-8.69013696978794,-1.32441658151506,
22.3975295501331));
#26428=CARTESIAN_POINT('Ctrl Pts',(-7.48757400439743,-0.874933687463104,
22.4452515735881));
#26429=CARTESIAN_POINT('Ctrl Pts',(-7.26356541515204,0.167920622083289,
22.485019926467));
#26430=CARTESIAN_POINT('Ctrl Pts',(-7.6689528934835,0.83168028369988,22.5168346087703));
#26431=CARTESIAN_POINT('Ctrl Pts',(-8.33302111081603,1.23656211671549,22.5486492910735));
#26432=CARTESIAN_POINT('Ctrl Pts',(-9.37570451013549,1.01175934142366,22.5884176439526));
#26433=CARTESIAN_POINT('Ctrl Pts',(-9.82427138668064,-0.19114560704095,
22.6361396674074));
#26434=CARTESIAN_POINT('Ctrl Pts',(-9.05542987457454,-1.21620894920483,
22.6838616908623));
#26435=CARTESIAN_POINT('Ctrl Pts',(-7.77725385403873,-1.12599705024939,
22.7315837143172));
#26436=CARTESIAN_POINT('Ctrl Pts',(-7.1618988042227,0.000737488335527086,
22.7793057377721));
#26437=CARTESIAN_POINT('Ctrl Pts',(-7.67480916412578,0.935963622326308,
22.8190740906511));
#26438=CARTESIAN_POINT('Ctrl Pts',(-8.41566875034181,1.17269758585735,22.8508887729544));
#26439=CARTESIAN_POINT('Ctrl Pts',(-9.18277819629672,1.04440497537631,22.8827034552576));
#26440=CARTESIAN_POINT('Ctrl Pts',(-9.8242272605525,0.192191353705862,22.9224718081366));
#26441=CARTESIAN_POINT('Ctrl Pts',(-9.37642209067293,-1.01099736283169,
22.9701938315915));
#26442=CARTESIAN_POINT('Ctrl Pts',(-8.1243057998852,-1.28316811903035,23.0179158550463));
#26443=CARTESIAN_POINT('Ctrl Pts',(-7.21670468463048,-0.378661434823841,
23.0656378785012));
#26444=CARTESIAN_POINT('Ctrl Pts',(-7.48853905055207,0.876049143468286,
23.1133599019561));
#26445=CARTESIAN_POINT('Ctrl Pts',(-8.48832796542965,1.24773057249471,23.1531282548351));
#26446=CARTESIAN_POINT('Ctrl Pts',(-9.20349553135788,0.942032602888077,
23.1849429371384));
#26447=CARTESIAN_POINT('Ctrl Pts',(-9.69968544546749,0.343107344518375,
23.2167576194416));
#26448=CARTESIAN_POINT('Ctrl Pts',(-9.6271980157496,-0.72106864258534,23.2565259723207));
#26449=CARTESIAN_POINT('Ctrl Pts',(-8.50132284585153,-1.33799461835653,
23.3042479957755));
#26450=CARTESIAN_POINT('Ctrl Pts',(-7.37633015273652,-0.724591352450931,
23.3519700192304));
#26451=CARTESIAN_POINT('Ctrl Pts',(-7.2817534589978,0.553269115357387,23.3996920426852));
#26452=CARTESIAN_POINT('Ctrl Pts',(-8.30825979254401,1.3242926590729,23.4474140661402));
#26453=CARTESIAN_POINT('Ctrl Pts',(-9.3075368060717,0.951237154850738,23.4871824190191));
#26454=CARTESIAN_POINT('Ctrl Pts',(-9.64837291280723,0.252132982124907,
23.5189971013224));
#26455=CARTESIAN_POINT('Ctrl Pts',(-9.63175400718011,-0.525452838188874,
23.5508117836256));
#26456=CARTESIAN_POINT('Ctrl Pts',(-8.8806672240812,-1.28281246429085,23.5905801365047));
#26457=CARTESIAN_POINT('Ctrl Pts',(-7.62557872246267,-1.01272838316213,
23.6383021599596));
#26458=CARTESIAN_POINT('Ctrl Pts',(-7.17613609374723,0.187218886379039,
23.6860241834144));
#26459=CARTESIAN_POINT('Ctrl Pts',(-7.94068933163074,1.21548464610644,23.7337462068693));
#26460=CARTESIAN_POINT('Ctrl Pts',(-9.22145261230867,1.1269522981132,23.7814682303241));
#26461=CARTESIAN_POINT('Ctrl Pts',(-9.73307681667046,0.191021941459234,
23.8212365832032));
#26462=CARTESIAN_POINT('Ctrl Pts',(-9.53342612569965,-0.560679792988806,
23.8530512655064));
#26463=CARTESIAN_POINT('Ctrl Pts',(-9.01210000646154,-1.13785825185349,
23.8848659478097));
#26464=CARTESIAN_POINT('Ctrl Pts',(-7.94856368871474,-1.21919372891504,
23.9246343006887));
#26465=CARTESIAN_POINT('Ctrl Pts',(-7.1761091647714,-0.193763786786585,
23.9723563241436));
#26466=CARTESIAN_POINT('Ctrl Pts',(-7.62131689716979,1.00776116143484,24.0200783475984));
#26467=CARTESIAN_POINT('Ctrl Pts',(-8.87228544066663,1.28515948400961,24.0678003710534));
#26468=CARTESIAN_POINT('Ctrl Pts',(-9.78294207479748,0.380230176003933,
24.1155223945081));
#26469=CARTESIAN_POINT('Ctrl Pts',(-9.55750006810439,-0.662315199801606,
24.1552907473873));
#26470=CARTESIAN_POINT('Ctrl Pts',(-8.91469096537924,-1.10016489253993,
24.1871054296905));
#26471=CARTESIAN_POINT('Ctrl Pts',(-8.14280065349016,-1.19556532434741,
24.2189201119937));
#26472=CARTESIAN_POINT('Ctrl Pts',(-7.28528169296711,-0.561226147456453,
24.2586884648727));
#26473=CARTESIAN_POINT('Ctrl Pts',(-7.37202759718887,0.719659368846581,
24.3064104883277));
#26474=CARTESIAN_POINT('Ctrl Pts',(-8.49484987781715,1.33702656291388,24.3541325117825));
#26475=CARTESIAN_POINT('Ctrl Pts',(-9.62239486975506,0.728327608305291,
24.4018545352374));
#26476=CARTESIAN_POINT('Ctrl Pts',(-9.71900579594374,-0.551851631768187,
24.4495765586922));
#26477=CARTESIAN_POINT('Ctrl Pts',(-8.86639905928022,-1.19277807964749,
24.4893449115712));
#26478=CARTESIAN_POINT('Ctrl Pts',(-8.09379671343249,-1.10332691326113,
24.5211595938745));
#26479=CARTESIAN_POINT('Ctrl Pts',(-7.44763360975285,-0.6704422410672,24.5529742761777));
#26480=CARTESIAN_POINT('Ctrl Pts',(-7.21416680485634,0.3703354537393,24.5927426290568));
#26481=CARTESIAN_POINT('Ctrl Pts',(-8.11782508502159,1.2822533614826,24.6404646525117));
#26482=CARTESIAN_POINT('Ctrl Pts',(-9.37089350882629,1.014500394273,24.6881866759665));
#26483=CARTESIAN_POINT('Ctrl Pts',(-9.82534425375221,-0.183559139565816,
24.7359086994214));
#26484=CARTESIAN_POINT('Ctrl Pts',(-9.06081228708266,-1.21490943394426,
24.7836307228763));
#26485=CARTESIAN_POINT('Ctrl Pts',(-7.99668094234245,-1.14176956700014,
24.8233990757553));
#26486=CARTESIAN_POINT('Ctrl Pts',(-7.47092386605872,-0.568624391050042,
24.8552137580586));
#26487=CARTESIAN_POINT('Ctrl Pts',(-7.26548819241141,0.181516982272607,
24.8870284403618));
#26488=CARTESIAN_POINT('Ctrl Pts',(-7.76988706005669,1.12136098066457,24.9267967932408));
#26489=CARTESIAN_POINT('Ctrl Pts',(-9.04993030585202,1.21975735594326,24.9745188166957));
#26490=CARTESIAN_POINT('Ctrl Pts',(-9.82238233795618,0.19741202080254,25.0222408401506));
#26491=CARTESIAN_POINT('Ctrl Pts',(-9.38219711576266,-1.00596202592954,
25.0699628636054));
#26492=CARTESIAN_POINT('Ctrl Pts',(-8.12922651266813,-1.28570695538346,
25.1176848870603));
#26493=CARTESIAN_POINT('Ctrl Pts',(-7.37232752343053,-0.534155973023465,
25.1574532399393));
#26494=CARTESIAN_POINT('Ctrl Pts',(-7.34971879980421,0.243278745517771,
25.1892679222426));
#26495=CARTESIAN_POINT('Ctrl Pts',(-7.68515908277749,0.94498788222336,25.2210826045458));
#26496=CARTESIAN_POINT('Ctrl Pts',(-8.68153252474089,1.32573047656409,25.2608509574249));
#26497=CARTESIAN_POINT('Ctrl Pts',(-9.71394815471084,0.562637739887994,
25.3085729808797));
#26498=CARTESIAN_POINT('Ctrl Pts',(-9.62921855937965,-0.715913401780119,
25.3562950043346));
#26499=CARTESIAN_POINT('Ctrl Pts',(-8.50898474258058,-1.33796510532709,
25.4040170277894));
#26500=CARTESIAN_POINT('Ctrl Pts',(-7.37839035099148,-0.729730874556245,
25.4517390512443));
#26501=CARTESIAN_POINT('Ctrl Pts',(-7.29770694788286,0.333855110429494,
25.4915074041234));
#26502=CARTESIAN_POINT('Ctrl Pts',(-7.78926817953549,0.936585109279324,
25.5233220864266));
#26503=CARTESIAN_POINT('Ctrl Pts',(-8.50205950886568,1.24778346533051,25.5551367687299));
#26504=CARTESIAN_POINT('Ctrl Pts',(-9.50468208918595,0.883815169420991,
25.5949051216089));
#26505=CARTESIAN_POINT('Ctrl Pts',(-9.7861743400752,-0.368764037840361,
25.6426271450638));
#26506=CARTESIAN_POINT('Ctrl Pts',(-8.88556823233645,-1.2802357954333,25.6903491685186));
#26507=CARTESIAN_POINT('Ctrl Pts',(-7.63139236705886,-1.01771908141124,
25.7380711919735));
#26508=CARTESIAN_POINT('Ctrl Pts',(-7.17433144450681,0.181984161415946,
25.7857932154284));
#26509=CARTESIAN_POINT('Ctrl Pts',(-7.80919625071778,1.03911404470665,25.8255615683074));
#26510=CARTESIAN_POINT('Ctrl Pts',(-8.57529460171618,1.173312452204,25.8573762506107));
#26511=CARTESIAN_POINT('Ctrl Pts',(-9.31795593805921,0.942292895719095,
25.8891909329139));
#26512=CARTESIAN_POINT('Ctrl Pts',(-9.83805580732715,0.0110458366725677,
25.928959285793));
#26513=CARTESIAN_POINT('Ctrl Pts',(-9.23139907623976,-1.12039579611305,
25.9766813092478));
#26514=CARTESIAN_POINT('Ctrl Pts',(-7.95395595261882,-1.22045174096127,
26.0244033327027));
#26515=CARTESIAN_POINT('Ctrl Pts',(-7.17724044410301,-0.20134176406142,
26.0721253561575));
#26516=CARTESIAN_POINT('Ctrl Pts',(-7.61652715495395,1.00498312726924,26.1198473796124));
#26517=CARTESIAN_POINT('Ctrl Pts',(-8.65744779364467,1.237811783029,26.1596157324915));
#26518=CARTESIAN_POINT('Ctrl Pts',(-9.32461540559779,0.838057766741282,
26.1914304147947));
#26519=CARTESIAN_POINT('Ctrl Pts',(-9.73510427955986,0.177440797287226,
26.223245097098));
#26520=CARTESIAN_POINT('Ctrl Pts',(-9.51913620553223,-0.867108268097489,
26.263013449977));
#26521=CARTESIAN_POINT('Ctrl Pts',(-8.32007162001735,-1.32584204441894,
26.3107354734319));
#26522=CARTESIAN_POINT('Ctrl Pts',(-7.28853651967721,-0.565705567888474,
26.3584574968867));
#26523=CARTESIAN_POINT('Ctrl Pts',(-7.3679250200947,0.713188326141545,26.4061795203416));
#26524=CARTESIAN_POINT('Ctrl Pts',(-8.48941001014702,1.33805949275231,26.4539015437964));
#26525=CARTESIAN_POINT('Ctrl Pts',(-9.42894458279322,0.833084497531996,
26.4936698966755));
#26526=CARTESIAN_POINT('Ctrl Pts',(-9.67194167558743,0.0942554856010431,
26.5254845789787));
#26527=CARTESIAN_POINT('Ctrl Pts',(-9.55014748720162,-0.673912511423524,
26.557299261282));
#26528=CARTESIAN_POINT('Ctrl Pts',(-8.70339447170565,-1.32255285070552,
26.597067614161));
#26529=CARTESIAN_POINT('Ctrl Pts',(-7.49645805411769,-0.884949101093904,
26.6447896376159));
#26530=CARTESIAN_POINT('Ctrl Pts',(-7.21369748796687,0.364818312633921,
26.6925116610707));
#26531=CARTESIAN_POINT('Ctrl Pts',(-8.11048863058951,1.28004384369136,26.7402336845256));
#26532=CARTESIAN_POINT('Ctrl Pts',(-9.36745541506446,1.01884074167898,26.7879557079805));
#26533=CARTESIAN_POINT('Ctrl Pts',(-9.74758705702552,0.0222340520690824,
26.8277240608595));
#26534=CARTESIAN_POINT('Ctrl Pts',(-9.44795416168687,-0.69549571881149,
26.8595387431628));
#26535=CARTESIAN_POINT('Ctrl Pts',(-8.85325076894622,-1.19673794632238,
26.891353425466));
#26536=CARTESIAN_POINT('Ctrl Pts',(-7.78849928368159,-1.13326170177414,
26.9311217783451));
#26537=CARTESIAN_POINT('Ctrl Pts',(-7.16206452223313,-0.0126493480035826,
26.9788438017999));
#26538=CARTESIAN_POINT('Ctrl Pts',(-7.76592238843451,1.11749568853494,27.0265658252548));
#26539=CARTESIAN_POINT('Ctrl Pts',(-9.04293644689573,1.22288648831542,27.0742878487096));
#26540=CARTESIAN_POINT('Ctrl Pts',(-9.82262206597892,0.202943895240207,
27.1220098721645));
#26541=CARTESIAN_POINT('Ctrl Pts',(-9.45803912628356,-0.799455346119385,
27.1617782250435));
#26542=CARTESIAN_POINT('Ctrl Pts',(-8.76184528940354,-1.14619737914625,
27.1935929073468));
#26543=CARTESIAN_POINT('Ctrl Pts',(-7.98414664679625,-1.13616158002172,
27.22540758965));
#26544=CARTESIAN_POINT('Ctrl Pts',(-7.22045596972938,-0.391512999309722,
27.2651759425291));
#26545=CARTESIAN_POINT('Ctrl Pts',(-7.47990565042312,0.8658168782332,27.312897965984));
#26546=CARTESIAN_POINT('Ctrl Pts',(-8.67600524947205,1.32540133765365,27.3606199894388));
#26547=CARTESIAN_POINT('Ctrl Pts',(-9.71070635102469,0.569580091172984,
27.4083420128937));
#26548=CARTESIAN_POINT('Ctrl Pts',(-9.63301924336791,-0.711886752361416,
27.4560640363486));
#26549=CARTESIAN_POINT('Ctrl Pts',(-8.70145348389303,-1.23141557232169,
27.4958323892276));
#26550=CARTESIAN_POINT('Ctrl Pts',(-7.94808857747159,-1.03813542913593,
27.5276470715309));
#26551=CARTESIAN_POINT('Ctrl Pts',(-7.36651760850961,-0.521713988800611,
27.5594617538341));
#26552=CARTESIAN_POINT('Ctrl Pts',(-7.27618187297965,0.541095690248971,
27.5992301067131));
#26553=CARTESIAN_POINT('Ctrl Pts',(-8.29503599950346,1.3222031262906,27.646952130168));
#26554=CARTESIAN_POINT('Ctrl Pts',(-9.50028672025696,0.8871826367628,27.6946741536229));
#26555=CARTESIAN_POINT('Ctrl Pts',(-9.78826494942713,-0.361392817789259,
27.7423961770777));
#26556=CARTESIAN_POINT('Ctrl Pts',(-8.89107706408667,-1.27967733588393,
27.7901182005326));
#26557=CARTESIAN_POINT('Ctrl Pts',(-7.84666060597338,-1.06306888494675,
27.8298865534116));
#26558=CARTESIAN_POINT('Ctrl Pts',(-7.40338501873419,-0.42398935176246,
27.8617012357149));
#26559=CARTESIAN_POINT('Ctrl Pts',(-7.30145370852712,0.34706570721632,27.8935159180181));
#26560=CARTESIAN_POINT('Ctrl Pts',(-7.92851098567795,1.20992382427112,27.9332842708972));
#26561=CARTESIAN_POINT('Ctrl Pts',(-9.2100849376435,1.13402413113834,27.981006294352));
#26562=CARTESIAN_POINT('Ctrl Pts',(-9.8369350579009,0.0164682923010958,
28.0287283178069));
#26563=CARTESIAN_POINT('Ctrl Pts',(-9.23780294045469,-1.11618912811791,
28.0764503412618));
#26564=CARTESIAN_POINT('Ctrl Pts',(-7.95848741323725,-1.22363371660283,
28.1241723647166));
#26565=CARTESIAN_POINT('Ctrl Pts',(-7.31036634376251,-0.376483176085945,
28.1639407175957));
#26566=CARTESIAN_POINT('Ctrl Pts',(-7.39327398065573,0.396848718847905,
28.1957553998989));
#26567=CARTESIAN_POINT('Ctrl Pts',(-7.82067316599591,1.04665317585658,28.2275700822022));
#26568=CARTESIAN_POINT('Ctrl Pts',(-8.85943719755328,1.28892212916213,28.2673384350812));
#26569=CARTESIAN_POINT('Ctrl Pts',(-9.77897218441442,0.393015903201587,
28.3150604585361));
#26570=CARTESIAN_POINT('Ctrl Pts',(-9.52183643350912,-0.862274235290551,
28.3627824819909));
#26571=CARTESIAN_POINT('Ctrl Pts',(-8.32766689782281,-1.32685065118973,
28.4105045054458));
#26572=CARTESIAN_POINT('Ctrl Pts',(-7.28988155219882,-0.571076786729173,
28.4582265289006));
#26573=CARTESIAN_POINT('Ctrl Pts',(-7.35401058852779,0.4936355808648,28.4979948817797));
#26574=CARTESIAN_POINT('Ctrl Pts',(-7.92268452713421,1.02422567452007,28.529809564083));
#26575=CARTESIAN_POINT('Ctrl Pts',(-8.67105994361954,1.23600417218416,28.5616242463862));
#26576=CARTESIAN_POINT('Ctrl Pts',(-9.61514016258385,0.739579455901104,
28.6013925992652));
#26577=CARTESIAN_POINT('Ctrl Pts',(-9.72436898518915,-0.539584967461109,
28.6491146227201));
#26578=CARTESIAN_POINT('Ctrl Pts',(-8.70859933360693,-1.32066379967392,
28.696836646175));
#26579=CARTESIAN_POINT('Ctrl Pts',(-7.50154209854002,-0.890681293407978,
28.7445586696298));
#26580=CARTESIAN_POINT('Ctrl Pts',(-7.21120039694662,0.359876283869756,
28.7922806930847));
#26581=CARTESIAN_POINT('Ctrl Pts',(-7.95631706256593,1.12311027083399,28.8320490459638));
#26582=CARTESIAN_POINT('Ctrl Pts',(-8.73353253024973,1.15229941527241,28.863863728267));
#26583=CARTESIAN_POINT('Ctrl Pts',(-9.43805614056221,0.822811344328694,
28.8956784105702));
#26584=CARTESIAN_POINT('Ctrl Pts',(-9.82721969175024,-0.170303293380481,
28.9354467634493));
#26585=CARTESIAN_POINT('Ctrl Pts',(-9.07289405752337,-1.2091417450888,28.9831687869042));
#26586=CARTESIAN_POINT('Ctrl Pts',(-7.79367140603468,-1.13523854117236,
29.030890810359));
#26587=CARTESIAN_POINT('Ctrl Pts',(-7.16215896705078,-0.0203107034760627,
29.0786128338139));
#26588=CARTESIAN_POINT('Ctrl Pts',(-7.76080034695112,1.11539202291376,29.1263348572687));
#26589=CARTESIAN_POINT('Ctrl Pts',(-8.82366560643313,1.20507622033222,29.1661032101478));
#26590=CARTESIAN_POINT('Ctrl Pts',(-9.43053464406366,0.718634766301466,
29.197917892451));
#26591=CARTESIAN_POINT('Ctrl Pts',(-9.74775700628796,0.00850363864441496,
29.2297325747543));
#26592=CARTESIAN_POINT('Ctrl Pts',(-9.39228672033525,-0.997164717746648,
29.2695009276333));
#26593=CARTESIAN_POINT('Ctrl Pts',(-8.14213995932516,-1.28924928143331,
29.3172229510882));
#26594=CARTESIAN_POINT('Ctrl Pts',(-7.22306871510535,-0.396393259163025,
29.364944974543));
#26595=CARTESIAN_POINT('Ctrl Pts',(-7.47497441546891,0.859963540492578,
29.4126669979979));
#26596=CARTESIAN_POINT('Ctrl Pts',(-8.67073545386039,1.32715695287662,29.4603890214527));
#26597=CARTESIAN_POINT('Ctrl Pts',(-9.53326385014039,0.699583561916176,
29.5001573743319));
#26598=CARTESIAN_POINT('Ctrl Pts',(-9.67386119595553,-0.0653703009610333,
29.531972056635));
#26599=CARTESIAN_POINT('Ctrl Pts',(-9.44929686259604,-0.809923379715055,
29.5637867389383));
#26600=CARTESIAN_POINT('Ctrl Pts',(-8.52213151947877,-1.33797052146522,
29.6035550918174));
#26601=CARTESIAN_POINT('Ctrl Pts',(-7.38624034864398,-0.740763047589384,
29.6512771152722));
#26602=CARTESIAN_POINT('Ctrl Pts',(-7.27422930025927,0.535519851685437,
29.6989991387271));
#26603=CARTESIAN_POINT('Ctrl Pts',(-8.2888747001765,1.32134053301234,29.7467211621819));
#26604=CARTESIAN_POINT('Ctrl Pts',(-9.29366927115465,0.962938239586792,
29.786489515061));
#26605=CARTESIAN_POINT('Ctrl Pts',(-9.64466888997224,0.268650789364219,
29.8183041973642));
#26606=CARTESIAN_POINT('Ctrl Pts',(-9.63899688479749,-0.508672370426549,
29.8501188796675));
#26607=CARTESIAN_POINT('Ctrl Pts',(-8.89986075464358,-1.27780800896432,
29.8898872325465));
#26608=CARTESIAN_POINT('Ctrl Pts',(-7.63927858840787,-1.02415996628783,
29.9376092560014));
#26609=CARTESIAN_POINT('Ctrl Pts',(-7.25303160763693,-0.0327948314514716,
29.9773776088804));
#26610=CARTESIAN_POINT('Ctrl Pts',(-7.54670173216219,0.690609604732206,
30.0091922911837));
#26611=CARTESIAN_POINT('Ctrl Pts',(-7.84279804142178,0.939512810771537,
30.0250996323353));
#26612=CARTESIAN_POINT('Ctrl Pts',(-8.01282215114119,1.02066752383247,30.0330533029111));
#26613=CARTESIAN_POINT('Ctrl Pts',(-7.87660126793166,-0.874219306856458,
1.76694669708889));
#26614=CARTESIAN_POINT('Ctrl Pts',(-7.73097269067503,-0.770372743754183,
1.7749003676647));
#26615=CARTESIAN_POINT('Ctrl Pts',(-7.49505426275024,-0.488941412697979,
1.79080770881633));
#26616=CARTESIAN_POINT('Ctrl Pts',(-7.33944865341066,0.235760887270365,
1.82262239111956));
#26617=CARTESIAN_POINT('Ctrl Pts',(-7.86365505261755,1.09918250918611,1.86239074399862));
#26618=CARTESIAN_POINT('Ctrl Pts',(-9.08404871094944,1.12901342715983,1.91011276745348));
#26619=CARTESIAN_POINT('Ctrl Pts',(-9.64865400304555,0.288282690195508,
1.94988112033254));
#26620=CARTESIAN_POINT('Ctrl Pts',(-9.52610611016745,-0.439466000029754,
1.98169580263577));
#26621=CARTESIAN_POINT('Ctrl Pts',(-9.08371912176839,-1.03091022985107,
2.01351048493902));
#26622=CARTESIAN_POINT('Ctrl Pts',(-8.08526338637744,-1.20075991772491,
2.05327883781807));
#26623=CARTESIAN_POINT('Ctrl Pts',(-7.26579462249314,-0.299113479422665,
2.10100086127293));
#26624=CARTESIAN_POINT('Ctrl Pts',(-7.58044611662734,0.875818431377988,
2.14872288472779));
#26625=CARTESIAN_POINT('Ctrl Pts',(-8.74075814219729,1.24739438139292,2.19644490818265));
#26626=CARTESIAN_POINT('Ctrl Pts',(-9.52082863358897,0.601160787975269,
2.23621326106171));
#26627=CARTESIAN_POINT('Ctrl Pts',(-9.60834021877745,-0.131949724327797,
2.26802794336495));
#26628=CARTESIAN_POINT('Ctrl Pts',(-9.35106143617397,-0.824074962016934,
2.29984262566819));
#26629=CARTESIAN_POINT('Ctrl Pts',(-8.44135567630907,-1.26900551071649,
2.33961097854724));
#26630=CARTESIAN_POINT('Ctrl Pts',(-7.40013276896415,-0.635493945930393,
2.38733300200211));
#26631=CARTESIAN_POINT('Ctrl Pts',(-7.37123600950541,0.580662319132022,
2.43505502545696));
#26632=CARTESIAN_POINT('Ctrl Pts',(-8.37744343232561,1.26433851735166,2.48277704891183));
#26633=CARTESIAN_POINT('Ctrl Pts',(-9.49831957514312,0.785612751107122,
2.53049907236669));
#26634=CARTESIAN_POINT('Ctrl Pts',(-9.66528404865682,-0.213177748400982,
2.57026742524574));
#26635=CARTESIAN_POINT('Ctrl Pts',(-9.2518736926554,-0.82499175948189,2.60208210754898));
#26636=CARTESIAN_POINT('Ctrl Pts',(-8.6044284386178,-1.18001050930349,2.63389678985223));
#26637=CARTESIAN_POINT('Ctrl Pts',(-7.6253748932976,-0.921337331474078,
2.67366514273128));
#26638=CARTESIAN_POINT('Ctrl Pts',(-7.25242721212033,0.239034337796918,
2.72138716618614));
#26639=CARTESIAN_POINT('Ctrl Pts',(-8.0262858459658,1.17764965562183,2.769109189641));
#26640=CARTESIAN_POINT('Ctrl Pts',(-9.23454501169552,1.0363489218597,2.81683121309586));
#26641=CARTESIAN_POINT('Ctrl Pts',(-9.76899309284508,-0.059058723161371,
2.86455323655073));
#26642=CARTESIAN_POINT('Ctrl Pts',(-9.24177187839627,-0.923636465033414,
2.90432158942978));
#26643=CARTESIAN_POINT('Ctrl Pts',(-8.52883239433566,-1.11583816367411,
2.93613627173302));
#26644=CARTESIAN_POINT('Ctrl Pts',(-7.8069182369327,-0.960711973455134,
2.96795095403626));
#26645=CARTESIAN_POINT('Ctrl Pts',(-7.23575031818529,-0.124515764873949,
3.00771930691532));
#26646=CARTESIAN_POINT('Ctrl Pts',(-7.71291403621515,0.997031160766364,
3.05544133037017));
#26647=CARTESIAN_POINT('Ctrl Pts',(-8.9122634679914,1.20054261779448,3.10316335382504));
#26648=CARTESIAN_POINT('Ctrl Pts',(-9.73356335662679,0.30314500910545,3.1508853772799));
#26649=CARTESIAN_POINT('Ctrl Pts',(-9.42103936740634,-0.874938806376356,
3.19860740073476));
#26650=CARTESIAN_POINT('Ctrl Pts',(-8.45665156776007,-1.18382884768558,
3.23837575361381));
#26651=CARTESIAN_POINT('Ctrl Pts',(-7.7917351978084,-0.86272074661816,3.27019043591706));
#26652=CARTESIAN_POINT('Ctrl Pts',(-7.34728101473615,-0.273072825713877,
3.3020051182203));
#26653=CARTESIAN_POINT('Ctrl Pts',(-7.46243893945415,0.733006464555997,
3.34177347109935));
#26654=CARTESIAN_POINT('Ctrl Pts',(-8.55710010482131,1.26898188682335,3.38949549455421));
#26655=CARTESIAN_POINT('Ctrl Pts',(-9.59726535329547,0.638179041168183,
3.43721751800907));
#26656=CARTESIAN_POINT('Ctrl Pts',(-9.63122777596328,-0.5778400902944,3.48493954146394));
#26657=CARTESIAN_POINT('Ctrl Pts',(-8.62408505598824,-1.26429202730363,
3.53266156491879));
#26658=CARTESIAN_POINT('Ctrl Pts',(-7.69266333517091,-0.866912531215043,
3.57242991779785));
#26659=CARTESIAN_POINT('Ctrl Pts',(-7.39991238656605,-0.189032694070974,
3.60424460010109));
#26660=CARTESIAN_POINT('Ctrl Pts',(-7.4495866441596,0.547687510380818,3.63605928240433));
#26661=CARTESIAN_POINT('Ctrl Pts',(-8.19493168629539,1.23319291086082,3.67582763528338));
#26662=CARTESIAN_POINT('Ctrl Pts',(-9.37345025199584,0.922312370267252,
3.72354965873824));
#26663=CARTESIAN_POINT('Ctrl Pts',(-9.74735766565093,-0.235292579725254,
3.77127168219311));
#26664=CARTESIAN_POINT('Ctrl Pts',(-8.97742616722564,-1.17713198321507,
3.81899370564797));
#26665=CARTESIAN_POINT('Ctrl Pts',(-7.76664010375505,-1.03731128115117,
3.86671572910283));
#26666=CARTESIAN_POINT('Ctrl Pts',(-7.32224636513591,-0.127382113028792,
3.90648408198189));
#26667=CARTESIAN_POINT('Ctrl Pts',(-7.5443749810873,0.576807541461097,3.93829876428512));
#26668=CARTESIAN_POINT('Ctrl Pts',(-8.06396180868744,1.10145382239662,3.97011344658837));
#26669=CARTESIAN_POINT('Ctrl Pts',(-9.07614321007789,1.13220600285683,4.00988179946742));
#26670=CARTESIAN_POINT('Ctrl Pts',(-9.76399920197892,0.126021698354871,
4.05760382292229));
#26671=CARTESIAN_POINT('Ctrl Pts',(-9.28937139980207,-0.994060630598775,
4.10532584637714));
#26672=CARTESIAN_POINT('Ctrl Pts',(-8.09088247259194,-1.2025798517467,4.15304786983201));
#26673=CARTESIAN_POINT('Ctrl Pts',(-7.26670323063882,-0.304648174304674,
4.20076989328686));
#26674=CARTESIAN_POINT('Ctrl Pts',(-7.52597647054109,0.674246239304052,
4.24053824616593));
#26675=CARTESIAN_POINT('Ctrl Pts',(-8.15469842594599,1.06145793115607,4.27235292846916));
#26676=CARTESIAN_POINT('Ctrl Pts',(-8.89090269571564,1.1182687108372,4.30416761077241));
#26677=CARTESIAN_POINT('Ctrl Pts',(-9.67648874516065,0.479276187531012,
4.34393596365146));
#26678=CARTESIAN_POINT('Ctrl Pts',(-9.53835693531735,-0.731703714585315,
4.39165798710632));
#26679=CARTESIAN_POINT('Ctrl Pts',(-8.44657181882848,-1.26823072569175,
4.43938001056118));
#26680=CARTESIAN_POINT('Ctrl Pts',(-7.40378085558735,-0.641778028981052,
4.48710203401604));
#26681=CARTESIAN_POINT('Ctrl Pts',(-7.36799034216343,0.576528894322393,
4.53482405747091));
#26682=CARTESIAN_POINT('Ctrl Pts',(-8.2045365779891,1.14718402769951,4.57459241034995));
#26683=CARTESIAN_POINT('Ctrl Pts',(-8.93335409498056,1.0286546286397,4.6064070926532));
#26684=CARTESIAN_POINT('Ctrl Pts',(-9.52728111459864,0.589935029256832,
4.63822177495644));
#26685=CARTESIAN_POINT('Ctrl Pts',(-9.70330383013366,-0.407297586304579,
4.67799012783549));
#26686=CARTESIAN_POINT('Ctrl Pts',(-8.80652255850025,-1.23272842596821,
4.72571215129035));
#26687=CARTESIAN_POINT('Ctrl Pts',(-7.62981812135516,-0.924146764431953,
4.77343417474522));
#26688=CARTESIAN_POINT('Ctrl Pts',(-7.25107879140469,0.2318863208135,4.82115619820008));
#26689=CARTESIAN_POINT('Ctrl Pts',(-8.02112464411643,1.17665195574191,4.86887822165494));
#26690=CARTESIAN_POINT('Ctrl Pts',(-9.02713314147116,1.06087722113259,4.90864657453399));
#26691=CARTESIAN_POINT('Ctrl Pts',(-9.50075252065141,0.494389026039362,
4.94046125683723));
#26692=CARTESIAN_POINT('Ctrl Pts',(-9.66286681237104,-0.225988061280402,
4.97227593914048));
#26693=CARTESIAN_POINT('Ctrl Pts',(-9.14351628915378,-1.09531649171262,
5.01204429201953));
#26694=CARTESIAN_POINT('Ctrl Pts',(-7.92526047005516,-1.13280621633993,
5.05976631547439));
#26695=CARTESIAN_POINT('Ctrl Pts',(-7.23727231077356,-0.129547392844347,
5.10748833892925));
#26696=CARTESIAN_POINT('Ctrl Pts',(-7.70721752222633,0.992507629187124,
5.15521036238412));
#26697=CARTESIAN_POINT('Ctrl Pts',(-8.90770750181304,1.20316500297725,5.20293238583897));
#26698=CARTESIAN_POINT('Ctrl Pts',(-9.59275579921949,0.45739981463423,5.24270073871803));
#26699=CARTESIAN_POINT('Ctrl Pts',(-9.58029073858244,-0.280887943477999,
5.27451542102127));
#26700=CARTESIAN_POINT('Ctrl Pts',(-9.23156266180433,-0.931743472748283,
5.30633010332451));
#26701=CARTESIAN_POINT('Ctrl Pts',(-8.2700188308547,-1.24937588149542,5.34609845620357));
#26702=CARTESIAN_POINT('Ctrl Pts',(-7.32418008556689,-0.480648499302866,
5.39382047965842));
#26703=CARTESIAN_POINT('Ctrl Pts',(-7.460297862814,0.728205472420246,5.44154250311328));
#26704=CARTESIAN_POINT('Ctrl Pts',(-8.54983244603065,1.26928805965479,5.48926452656816));
#26705=CARTESIAN_POINT('Ctrl Pts',(-9.59553565999399,0.64314310157645,5.53698655002299));
#26706=CARTESIAN_POINT('Ctrl Pts',(-9.62566726192722,-0.369056963869468,
5.57675490290208));
#26707=CARTESIAN_POINT('Ctrl Pts',(-9.13319439575196,-0.919233905949193,
5.6085695852053));
#26708=CARTESIAN_POINT('Ctrl Pts',(-8.4436265719743,-1.18328012903449,5.64038426750855));
#26709=CARTESIAN_POINT('Ctrl Pts',(-7.50863566519058,-0.794372826254617,
5.6801526203876));
#26710=CARTESIAN_POINT('Ctrl Pts',(-7.2963041006504,0.40582216911912,5.72787464384246));
#26711=CARTESIAN_POINT('Ctrl Pts',(-8.19017130198736,1.23096300595092,5.77559666729732));
#26712=CARTESIAN_POINT('Ctrl Pts',(-9.36815438333627,0.927298990484527,
5.82331869075219));
#26713=CARTESIAN_POINT('Ctrl Pts',(-9.74929745946807,-0.23040679067796,
5.87104071420704));
#26714=CARTESIAN_POINT('Ctrl Pts',(-9.10982341009197,-1.01560092342369,
5.91080906708611));
#26715=CARTESIAN_POINT('Ctrl Pts',(-8.37741999008716,-1.10945944397624,
5.94262374938933));
#26716=CARTESIAN_POINT('Ctrl Pts',(-7.68317215392635,-0.857975580674617,
5.97443843169259));
#26717=CARTESIAN_POINT('Ctrl Pts',(-7.23053602901599,0.0478817062916687,
6.01420678457163));
#26718=CARTESIAN_POINT('Ctrl Pts',(-7.85522187282586,1.0944572251931,6.0619288080265));
#26719=CARTESIAN_POINT('Ctrl Pts',(-9.07108417384462,1.13363424900455,6.10965083148136));
#26720=CARTESIAN_POINT('Ctrl Pts',(-9.76325682424838,0.13325782172002,6.15737285493622));
#26721=CARTESIAN_POINT('Ctrl Pts',(-9.29403504413602,-0.991634902626839,
6.20509487839108));
#26722=CARTESIAN_POINT('Ctrl Pts',(-8.29669469572309,-1.16704617749604,
6.24486323127014));
#26723=CARTESIAN_POINT('Ctrl Pts',(-7.68140252519118,-0.758830871074005,
6.27667791357338));
#26724=CARTESIAN_POINT('Ctrl Pts',(-7.32091588622009,-0.114413634620499,
6.30849259587662));
#26725=CARTESIAN_POINT('Ctrl Pts',(-7.57129164808408,0.86679422500701,6.34826094875567));
#26726=CARTESIAN_POINT('Ctrl Pts',(-8.72846469997545,1.24955165236365,6.39598297221053));
#26727=CARTESIAN_POINT('Ctrl Pts',(-9.67359730356846,0.483666324224417,
6.4437049956654));
#26728=CARTESIAN_POINT('Ctrl Pts',(-9.54252995272924,-0.725745650157118,
6.49142701912026));
#26729=CARTESIAN_POINT('Ctrl Pts',(-8.45168581803811,-1.26944758507204,
6.53914904257512));
#26730=CARTESIAN_POINT('Ctrl Pts',(-7.58267596702233,-0.749564170486322,
6.57891739545417));
#26731=CARTESIAN_POINT('Ctrl Pts',(-7.38444589289304,-0.0382772879798582,
6.61073207775742));
#26732=CARTESIAN_POINT('Ctrl Pts',(-7.53345529358936,0.684924198480989,
6.64254676006065));
#26733=CARTESIAN_POINT('Ctrl Pts',(-8.36478642108454,1.2631503154814,6.68231511293971));
#26734=CARTESIAN_POINT('Ctrl Pts',(-9.49033250313942,0.795497947379644,
6.73003713639457));
#26735=CARTESIAN_POINT('Ctrl Pts',(-9.70398954175645,-0.402085721548271,
6.77775915984943));
#26736=CARTESIAN_POINT('Ctrl Pts',(-8.81357665277965,-1.23095293731772,
6.8254811833043));
#26737=CARTESIAN_POINT('Ctrl Pts',(-7.63288943478823,-0.928413000297835,
6.87320320675915));
#26738=CARTESIAN_POINT('Ctrl Pts',(-7.31584661237576,0.0333253917197164,
6.91297155963821));
#26739=CARTESIAN_POINT('Ctrl Pts',(-7.63131447932525,0.700936218801929,
6.94478624194145));
#26740=CARTESIAN_POINT('Ctrl Pts',(-8.21717882643293,1.15036603345952,6.97660092424469));
#26741=CARTESIAN_POINT('Ctrl Pts',(-9.22419691584206,1.04372901584115,7.01636927712374));
#26742=CARTESIAN_POINT('Ctrl Pts',(-9.76941978790048,-0.0463557239862788,
7.06409130057861));
#26743=CARTESIAN_POINT('Ctrl Pts',(-9.14744487412929,-1.0918236483497,7.11181332403347));
#26744=CARTESIAN_POINT('Ctrl Pts',(-7.93175681708765,-1.1360788423931,7.15953534748832));
#26745=CARTESIAN_POINT('Ctrl Pts',(-7.2368036935283,-0.134783243543619,
7.2072573709432));
#26746=CARTESIAN_POINT('Ctrl Pts',(-7.62628417013839,0.799969046778991,
7.24702572382224));
#26747=CARTESIAN_POINT('Ctrl Pts',(-8.3016614880762,1.09844797389141,7.2788404061255));
#26748=CARTESIAN_POINT('Ctrl Pts',(-9.03877580315234,1.05501206679962,7.31065508842871));
#26749=CARTESIAN_POINT('Ctrl Pts',(-9.73056622357639,0.315496752466419,
7.35042344130779));
#26750=CARTESIAN_POINT('Ctrl Pts',(-9.42967335637867,-0.865611287760983,
7.39814546476263));
#26751=CARTESIAN_POINT('Ctrl Pts',(-8.27527513009739,-1.24930479746904,
7.44586748821751));
#26752=CARTESIAN_POINT('Ctrl Pts',(-7.3269517593169,-0.487373856592538,
7.49358951167236));
#26753=CARTESIAN_POINT('Ctrl Pts',(-7.45651776268534,0.724552449331778,
7.54131153512723));
#26754=CARTESIAN_POINT('Ctrl Pts',(-8.36265239254167,1.1766331041921,7.58107988800629));
#26755=CARTESIAN_POINT('Ctrl Pts',(-9.06869720420805,0.960473636589914,
7.61289457030951));
#26756=CARTESIAN_POINT('Ctrl Pts',(-9.59772315388831,0.445346723994618,
7.64470925261277));
#26757=CARTESIAN_POINT('Ctrl Pts',(-9.63704266960617,-0.566538082496456,
7.68447760549181));
#26758=CARTESIAN_POINT('Ctrl Pts',(-8.63671733765756,-1.26288709734616,
7.73219962894668));
#26759=CARTESIAN_POINT('Ctrl Pts',(-7.51265726772717,-0.797758154555581,
7.77992165240153));
#26760=CARTESIAN_POINT('Ctrl Pts',(-7.29399992857171,0.398922647608031,
7.82764367585641));
#26761=CARTESIAN_POINT('Ctrl Pts',(-8.18492249268409,1.23067363496886,7.87536569931125));
#26762=CARTESIAN_POINT('Ctrl Pts',(-9.16597666144441,0.979696337426352,
7.91513405219033));
#26763=CARTESIAN_POINT('Ctrl Pts',(-9.55849681005219,0.354274780033274,
7.94694873449355));
#26764=CARTESIAN_POINT('Ctrl Pts',(-9.62153775717122,-0.381422189174436,
7.9787634167968));
#26765=CARTESIAN_POINT('Ctrl Pts',(-8.98921836539449,-1.17238936466715,
8.01853176967584));
#26766=CARTESIAN_POINT('Ctrl Pts',(-7.7771125247792,-1.04451383390958,8.06625379313071));
#26767=CARTESIAN_POINT('Ctrl Pts',(-7.23136243031766,0.0426902907278673,
8.11397581658558));
#26768=CARTESIAN_POINT('Ctrl Pts',(-7.84896512350466,1.09074701037696,8.16169784004043));
#26769=CARTESIAN_POINT('Ctrl Pts',(-9.06692541504432,1.13684959656092,8.20941986349531));
#26770=CARTESIAN_POINT('Ctrl Pts',(-9.64464173069743,0.305164112407195,
8.24918821637434));
#26771=CARTESIAN_POINT('Ctrl Pts',(-9.5322862505581,-0.424630679022379,
8.2810028986776));
#26772=CARTESIAN_POINT('Ctrl Pts',(-9.09861015205532,-1.0222503181763,8.31281758098083));
#26773=CARTESIAN_POINT('Ctrl Pts',(-8.10290335699141,-1.20670861749438,
8.35258593385989));
#26774=CARTESIAN_POINT('Ctrl Pts',(-7.26991055531728,-0.316947013142206,
8.40030795731474));
#26775=CARTESIAN_POINT('Ctrl Pts',(-7.56851998300448,0.862327502791123,
8.44802998076961));
#26776=CARTESIAN_POINT('Ctrl Pts',(-8.72130549715427,1.25083944932549,8.49575200422448));
#26777=CARTESIAN_POINT('Ctrl Pts',(-9.67255596256759,0.488818929738847,
8.54347402767932));
#26778=CARTESIAN_POINT('Ctrl Pts',(-9.56530155789297,-0.518133590791118,
8.58324238055841));
#26779=CARTESIAN_POINT('Ctrl Pts',(-9.0028429994127,-0.996531502060991,
8.61505706286162));
#26780=CARTESIAN_POINT('Ctrl Pts',(-8.28386407323049,-1.16473820591356,
8.64687174516488));
#26781=CARTESIAN_POINT('Ctrl Pts',(-7.41017032490435,-0.652765433141797,
8.68664009804392));
#26782=CARTESIAN_POINT('Ctrl Pts',(-7.36236902101554,0.56512937166147,8.73436212149877));
#26783=CARTESIAN_POINT('Ctrl Pts',(-8.35976785794315,1.26158578402979,8.78208414495366));
#26784=CARTESIAN_POINT('Ctrl Pts',(-9.48576091064866,0.801155963652941,
8.8298061684085));
#26785=CARTESIAN_POINT('Ctrl Pts',(-9.70657326537737,-0.397507719045183,
8.87752819186338));
#26786=CARTESIAN_POINT('Ctrl Pts',(-8.96663395036875,-1.0888446094455,8.91729654474242));
#26787=CARTESIAN_POINT('Ctrl Pts',(-8.22826712547428,-1.0826298358905,8.94911122704566));
#26788=CARTESIAN_POINT('Ctrl Pts',(-7.57448282332976,-0.73942395338778,
8.98092590934891));
#26789=CARTESIAN_POINT('Ctrl Pts',(-7.24872202178017,0.219396564799815,
9.02069426222796));
#26790=CARTESIAN_POINT('Ctrl Pts',(-8.00941503387016,1.17170894084964,9.06841628568281));
#26791=CARTESIAN_POINT('Ctrl Pts',(-9.2193779708416,1.04582937384631,9.1161383091377));
#26792=CARTESIAN_POINT('Ctrl Pts',(-9.76966442671916,-0.0390857337594308,
9.16386033259253));
#26793=CARTESIAN_POINT('Ctrl Pts',(-9.15239411426545,-1.09005199467533,
9.21158235604742));
#26794=CARTESIAN_POINT('Ctrl Pts',(-8.14048539099326,-1.12875111209956,
9.25135070892645));
#26795=CARTESIAN_POINT('Ctrl Pts',(-7.58615922326735,-0.640953314554951,
9.2831653912297));
#26796=CARTESIAN_POINT('Ctrl Pts',(-7.316285050622,0.0463545658407663,9.31498007353294));
#26797=CARTESIAN_POINT('Ctrl Pts',(-7.69726342320074,0.98460419443171,9.35474842641199));
#26798=CARTESIAN_POINT('Ctrl Pts',(-8.895617959699,1.20708818278666,9.40247044986686));
#26799=CARTESIAN_POINT('Ctrl Pts',(-9.72829610040157,0.320238089349479,
9.45019247332171));
#26800=CARTESIAN_POINT('Ctrl Pts',(-9.43461496670731,-0.860273395535559,
9.49791449677658));
#26801=CARTESIAN_POINT('Ctrl Pts',(-8.28017716505078,-1.25120316202397,
9.54563652023144));
#26802=CARTESIAN_POINT('Ctrl Pts',(-7.4895978159432,-0.618398943731734,
9.58540487311049));
#26803=CARTESIAN_POINT('Ctrl Pts',(-7.38954263082771,0.113183691003795,
9.61721955541374));
#26804=CARTESIAN_POINT('Ctrl Pts',(-7.63514045459009,0.809535542066336,
9.64903423771697));
#26805=CARTESIAN_POINT('Ctrl Pts',(-8.537133574773,1.26982381811355,9.68880259059603));
#26806=CARTESIAN_POINT('Ctrl Pts',(-9.58895975750512,0.654019951984606,
9.7365246140509));
#26807=CARTESIAN_POINT('Ctrl Pts',(-9.6384280382287,-0.561467136978377,
9.78424663750574));
#26808=CARTESIAN_POINT('Ctrl Pts',(-8.64394691727858,-1.26208349013273,
9.83196866096063));
#26809=CARTESIAN_POINT('Ctrl Pts',(-7.51512238801277,-0.802401097226443,
9.87969068441545));
#26810=CARTESIAN_POINT('Ctrl Pts',(-7.33127459545891,0.193418602868329,
9.91945903729455));
#26811=CARTESIAN_POINT('Ctrl Pts',(-7.73426663122311,0.812144398860134,
9.95127371959776));
#26812=CARTESIAN_POINT('Ctrl Pts',(-8.37560914334392,1.17807331772501,9.98308840190104));
#26813=CARTESIAN_POINT('Ctrl Pts',(-9.35890135525045,0.936012763466847,
10.02285675478));
#26814=CARTESIAN_POINT('Ctrl Pts',(-9.75144090539661,-0.217878662011005,
10.0705787782349));
#26815=CARTESIAN_POINT('Ctrl Pts',(-8.99358386781122,-1.16946086277756,
10.1183008016898));
#26816=CARTESIAN_POINT('Ctrl Pts',(-7.78310570163958,-1.04863626488784,
10.1660228251447));
#26817=CARTESIAN_POINT('Ctrl Pts',(-7.23018890616732,0.0375661736589278,
10.2137448485995));
#26818=CARTESIAN_POINT('Ctrl Pts',(-7.74269724808928,0.910945865078545,
10.2535132014786));
#26819=CARTESIAN_POINT('Ctrl Pts',(-8.45228056360055,1.11519010578825,10.2853278837818));
#26820=CARTESIAN_POINT('Ctrl Pts',(-9.17671754862795,0.972308174672121,
10.317142566085));
#26821=CARTESIAN_POINT('Ctrl Pts',(-9.76196042907608,0.145901702765871,
10.3569109189641));
#26822=CARTESIAN_POINT('Ctrl Pts',(-9.30385292282665,-0.983562875225906,
10.404632942419));
#26823=CARTESIAN_POINT('Ctrl Pts',(-8.10812083976582,-1.20735018445606,
10.4523549658738));
#26824=CARTESIAN_POINT('Ctrl Pts',(-7.27174569549875,-0.323985824587662,
10.5000769893287));
#26825=CARTESIAN_POINT('Ctrl Pts',(-7.56427989964802,0.859220184365555,
10.5477990127836));
#26826=CARTESIAN_POINT('Ctrl Pts',(-8.5232999629678,1.1843930677275,10.5875673656626));
#26827=CARTESIAN_POINT('Ctrl Pts',(-9.19355740431409,0.87458804221152,10.6193820479658));
#26828=CARTESIAN_POINT('Ctrl Pts',(-9.64793064309135,0.292549253643142,
10.6511967302691));
#26829=CARTESIAN_POINT('Ctrl Pts',(-9.54982217450754,-0.715335469088547,
10.6909650831482));
#26830=CARTESIAN_POINT('Ctrl Pts',(-8.4643919788304,-1.26976671868812,10.738687106603));
#26831=CARTESIAN_POINT('Ctrl Pts',(-7.41369629983366,-0.656664309321609,
10.7864091300579));
#26832=CARTESIAN_POINT('Ctrl Pts',(-7.35915150586694,0.558605553583151,
10.8341311535127));
#26833=CARTESIAN_POINT('Ctrl Pts',(-8.35452822785808,1.26201006134411,10.8818531769676));
#26834=CARTESIAN_POINT('Ctrl Pts',(-9.29254410063642,0.880456515508654,
10.9216215298466));
#26835=CARTESIAN_POINT('Ctrl Pts',(-9.59672961639489,0.207630116265999,
10.9534362121499));
#26836=CARTESIAN_POINT('Ctrl Pts',(-9.55953517254716,-0.529825485693832,
10.9852508944531));
#26837=CARTESIAN_POINT('Ctrl Pts',(-8.82590258181982,-1.22785135036252,
11.0250192473322));
#26838=CARTESIAN_POINT('Ctrl Pts',(-7.64228970867862,-0.936967719412468,
11.072741270787));
#26839=CARTESIAN_POINT('Ctrl Pts',(-7.2488375995026,0.214141055646775,11.1204632942419));
#26840=CARTESIAN_POINT('Ctrl Pts',(-8.00271338065867,1.16888043412647,11.1681853176968));
#26841=CARTESIAN_POINT('Ctrl Pts',(-9.21569307889762,1.04957841452743,11.2159073411516));
#26842=CARTESIAN_POINT('Ctrl Pts',(-9.67542825259376,0.147303259161649,
11.2556756940307));
#26843=CARTESIAN_POINT('Ctrl Pts',(-9.46525342395248,-0.560546112470954,
11.2874903763339));
#26844=CARTESIAN_POINT('Ctrl Pts',(-8.95462334184431,-1.09391381936859,
11.3193050586371));
#26845=CARTESIAN_POINT('Ctrl Pts',(-7.94310764484011,-1.14179785259405,
11.3590734115162));
#26846=CARTESIAN_POINT('Ctrl Pts',(-7.23831550942318,-0.147403179400998,
11.406795434971));
#26847=CARTESIAN_POINT('Ctrl Pts',(-7.6939122603442,0.98055407811529,11.4545174584259));
#26848=CARTESIAN_POINT('Ctrl Pts',(-8.88869917985897,1.20933386566182,11.5022394818808));
#26849=CARTESIAN_POINT('Ctrl Pts',(-9.72796230694971,0.325484260963068,
11.5499615053357));
#26850=CARTESIAN_POINT('Ctrl Pts',(-9.48529893752489,-0.65765935777389,
11.5897298582147));
#26851=CARTESIAN_POINT('Ctrl Pts',(-8.86322259765864,-1.05545983401,11.621544540518));
#26852=CARTESIAN_POINT('Ctrl Pts',(-8.12808565118239,-1.12472643087056,
11.6533592228212));
#26853=CARTESIAN_POINT('Ctrl Pts',(-7.33179403263406,-0.499125484457065,
11.6931275757003));
#26854=CARTESIAN_POINT('Ctrl Pts',(-7.44940412037606,0.714019431652113,
11.7408495991551));
#26855=CARTESIAN_POINT('Ctrl Pts',(-8.53194934097467,1.26895349944086,11.78857162261));
#26856=CARTESIAN_POINT('Ctrl Pts',(-9.58519671026048,0.660245068970213,
11.8362936460648));
#26857=CARTESIAN_POINT('Ctrl Pts',(-9.64160806535992,-0.557281308253744,
11.8840156695197));
#26858=CARTESIAN_POINT('Ctrl Pts',(-8.81484293386192,-1.1420174053632,11.9237840223988));
#26859=CARTESIAN_POINT('Ctrl Pts',(-8.08412316719659,-1.03584389586256,
11.955598704702));
#26860=CARTESIAN_POINT('Ctrl Pts',(-7.48285373565609,-0.607242376721559,
11.9874133870052));
#26861=CARTESIAN_POINT('Ctrl Pts',(-7.28997307136937,0.386867242620354,
12.0271817398843));
#26862=CARTESIAN_POINT('Ctrl Pts',(-8.17265124555415,1.22736231163514,12.0749037633391));
#26863=CARTESIAN_POINT('Ctrl Pts',(-9.35441133005812,0.938746517010956,
12.122625786794));
#26864=CARTESIAN_POINT('Ctrl Pts',(-9.75266805128835,-0.210708814103916,
12.1703478102489));
#26865=CARTESIAN_POINT('Ctrl Pts',(-8.99872747341793,-1.16837594064669,
12.2180698337037));
#26866=CARTESIAN_POINT('Ctrl Pts',(-7.99090309083843,-1.06964955206712,
12.2578381865828));
#26867=CARTESIAN_POINT('Ctrl Pts',(-7.50776093085483,-0.511260937604508,
12.289652868886));
#26868=CARTESIAN_POINT('Ctrl Pts',(-7.3334738690475,0.206268303333894,12.3214675511893));
#26869=CARTESIAN_POINT('Ctrl Pts',(-7.83803220192628,1.08426475813674,12.3612359040683));
#26870=CARTESIAN_POINT('Ctrl Pts',(-9.05547871457524,1.14237421570755,12.4089579275232));
#26871=CARTESIAN_POINT('Ctrl Pts',(-9.76035346995239,0.15090684182913,12.456679950978));
#26872=CARTESIAN_POINT('Ctrl Pts',(-9.30947203638216,-0.978943549636521,
12.5044019744329));
#26873=CARTESIAN_POINT('Ctrl Pts',(-8.11272055027382,-1.20989506125271,
12.5521239978878));
#26874=CARTESIAN_POINT('Ctrl Pts',(-7.41514461007779,-0.475834645766756,
12.5918923507668));
#26875=CARTESIAN_POINT('Ctrl Pts',(-7.4151086511821,0.262558332410862,12.6237070330701));
#26876=CARTESIAN_POINT('Ctrl Pts',(-7.75276774428468,0.919224555358408,
12.6555217153733));
#26877=CARTESIAN_POINT('Ctrl Pts',(-8.70879623786288,1.25309040475067,12.6952900682523));
#26878=CARTESIAN_POINT('Ctrl Pts',(-9.66751399921959,0.500486276221317,
12.7430120917072));
#26879=CARTESIAN_POINT('Ctrl Pts',(-9.55188166335335,-0.710498916559987,
12.7907341151621));
#26880=CARTESIAN_POINT('Ctrl Pts',(-8.47166377950834,-1.26994980596394,
12.8384561386169));
#26881=CARTESIAN_POINT('Ctrl Pts',(-7.41550978691736,-0.661598374508149,
12.8861781620718));
#26882=CARTESIAN_POINT('Ctrl Pts',(-7.3682459272926,0.349946490288843,12.9259465149509));
#26883=CARTESIAN_POINT('Ctrl Pts',(-7.85133369920765,0.908382159046878,
12.9577611972541));
#26884=CARTESIAN_POINT('Ctrl Pts',(-8.53633238175378,1.18406494128969,12.9895758795573));
#26885=CARTESIAN_POINT('Ctrl Pts',(-9.47777349447388,0.811042800922508,
13.0293442324364));
#26886=CARTESIAN_POINT('Ctrl Pts',(-9.71039396279849,-0.385385399153313,
13.0770662558912));
#26887=CARTESIAN_POINT('Ctrl Pts',(-8.83062453150002,-1.22554117160637,
13.1247882793461));
#26888=CARTESIAN_POINT('Ctrl Pts',(-7.64766924194114,-0.941863965722445,
13.172510302801));
#26889=CARTESIAN_POINT('Ctrl Pts',(-7.24698080025217,0.209223126081278,
13.2202323262558));
#26890=CARTESIAN_POINT('Ctrl Pts',(-7.87306983888273,1.00513103635134,13.2600006791349));
#26891=CARTESIAN_POINT('Ctrl Pts',(-8.60377926102454,1.11137571578629,13.2918153614381));
#26892=CARTESIAN_POINT('Ctrl Pts',(-9.30218522440413,0.871681531812472,
13.3236300437414));
#26893=CARTESIAN_POINT('Ctrl Pts',(-9.77009266600105,-0.0263827821550767,
13.3633983966204));
#26894=CARTESIAN_POINT('Ctrl Pts',(-9.16321490783652,-1.08338425181604,
13.4111204200753));
#26895=CARTESIAN_POINT('Ctrl Pts',(-7.94819013624447,-1.14314024441186,
13.4588424435301));
#26896=CARTESIAN_POINT('Ctrl Pts',(-7.2391802885307,-0.154625697185406,
13.506564466985));
#26897=CARTESIAN_POINT('Ctrl Pts',(-7.68929035206307,0.978049742173603,
13.5542864904399));
#26898=CARTESIAN_POINT('Ctrl Pts',(-8.68351804052399,1.17032087734838,13.5940548433189));
#26899=CARTESIAN_POINT('Ctrl Pts',(-9.30563312229838,0.772580991815164,
13.6258695256222));
#26900=CARTESIAN_POINT('Ctrl Pts',(-9.67697809753389,0.134359164483624,
13.6576842079254));
#26901=CARTESIAN_POINT('Ctrl Pts',(-9.44325009763995,-0.85094693414226,
13.6974525608044));
#26902=CARTESIAN_POINT('Ctrl Pts',(-8.2927229897676,-1.25324047656015,13.7451745842593));
#26903=CARTESIAN_POINT('Ctrl Pts',(-7.33475938495617,-0.503466039752598,
13.7928966077142));
#26904=CARTESIAN_POINT('Ctrl Pts',(-7.44533257125672,0.707991571847893,
13.8406186311691));
#26905=CARTESIAN_POINT('Ctrl Pts',(-8.52681547325545,1.27008360426311,13.8883406546239));
#26906=CARTESIAN_POINT('Ctrl Pts',(-9.4045024161679,0.764987062832887,13.928109007503));
#26907=CARTESIAN_POINT('Ctrl Pts',(-9.61474618672592,0.0571581651064585,
13.9599236898062));
#26908=CARTESIAN_POINT('Ctrl Pts',(-9.47800196452181,-0.668462403240976,
13.9917383721095));
#26909=CARTESIAN_POINT('Ctrl Pts',(-8.65657937087898,-1.2606801069419,14.0315067249885));
#26910=CARTESIAN_POINT('Ctrl Pts',(-7.52327723764377,-0.812150291851726,
14.0792287484434));
#26911=CARTESIAN_POINT('Ctrl Pts',(-7.28937569504537,0.381644515727654,
14.1269507718982));
#26912=CARTESIAN_POINT('Ctrl Pts',(-8.16562822136408,1.22546765143414,14.1746727953531));
#26913=CARTESIAN_POINT('Ctrl Pts',(-9.35126822931952,0.942960144001402,
14.2223948188079));
#26914=CARTESIAN_POINT('Ctrl Pts',(-9.68454787080297,-0.0132728644732055,
14.262163171687));
#26915=CARTESIAN_POINT('Ctrl Pts',(-9.38042788824344,-0.686128887499729,
14.2939778539902));
#26916=CARTESIAN_POINT('Ctrl Pts',(-8.80225636879473,-1.14541298869798,
14.3257925362935));
#26917=CARTESIAN_POINT('Ctrl Pts',(-7.7935772406708,-1.05584009988523,14.3655608891725));
#26918=CARTESIAN_POINT('Ctrl Pts',(-7.22997734567405,0.0248577665794866,
14.4132829126274));
#26919=CARTESIAN_POINT('Ctrl Pts',(-7.83416331394744,1.08070590432209,14.4610049360822));
#26920=CARTESIAN_POINT('Ctrl Pts',(-9.04892789296556,1.14553638937609,14.5087269595371));
#26921=CARTESIAN_POINT('Ctrl Pts',(-9.76073337693308,0.156149875811182,
14.556448982992));
#26922=CARTESIAN_POINT('Ctrl Pts',(-9.3871341050952,-0.785062358491584,
14.596217335871));
#26923=CARTESIAN_POINT('Ctrl Pts',(-8.71690684123967,-1.09493266409088,
14.6280320181743));
#26924=CARTESIAN_POINT('Ctrl Pts',(-7.97916280057658,-1.06398234893415,
14.6598467004775));
#26925=CARTESIAN_POINT('Ctrl Pts',(-7.27495151425187,-0.336285056074748,
14.6996150533566));
#26926=CARTESIAN_POINT('Ctrl Pts',(-7.55580506332157,0.849747828921635,
14.7473370768114));
#26927=CARTESIAN_POINT('Ctrl Pts',(-8.70354189550648,1.25293034154821,14.7950591002663));
#26928=CARTESIAN_POINT('Ctrl Pts',(-9.66462886206689,0.50716374522088,14.8427811237211));
#26929=CARTESIAN_POINT('Ctrl Pts',(-9.55559937622805,-0.706782420080516,
14.890503147176));
#26930=CARTESIAN_POINT('Ctrl Pts',(-8.65724835414967,-1.1741391659753,14.930271500055));
#26931=CARTESIAN_POINT('Ctrl Pts',(-7.94764515033822,-0.96996403905036,
14.9620861823583));
#26932=CARTESIAN_POINT('Ctrl Pts',(-7.40997390642474,-0.463867378652346,
14.9939008646615));
#26933=CARTESIAN_POINT('Ctrl Pts',(-7.35352879266581,0.547206716293156,
15.0336692175406));
#26934=CARTESIAN_POINT('Ctrl Pts',(-8.34192153595724,1.26039147291347,15.0813912409955));
#26935=CARTESIAN_POINT('Ctrl Pts',(-9.47369516602269,0.814359548927965,
15.1291132644503));
#26936=CARTESIAN_POINT('Ctrl Pts',(-9.71258097395429,-0.378447839289041,
15.1768352879052));
#26937=CARTESIAN_POINT('Ctrl Pts',(-8.83586773229483,-1.22516301435895,
15.2245573113601));
#26938=CARTESIAN_POINT('Ctrl Pts',(-7.85070500083801,-0.99083086753391,
15.2643256642391));
#26939=CARTESIAN_POINT('Ctrl Pts',(-7.44765287922776,-0.372144466768538,
15.2961403465424));
#26940=CARTESIAN_POINT('Ctrl Pts',(-7.3721652533645,0.362380053367863,15.3279550288456));
#26941=CARTESIAN_POINT('Ctrl Pts',(-7.99100368173551,1.16393843392934,15.3677233817246));
#26942=CARTESIAN_POINT('Ctrl Pts',(-9.20509935271424,1.05660333990528,15.4154454051795));
#26943=CARTESIAN_POINT('Ctrl Pts',(-9.7691800770222,-0.0212073876111575,
15.4631674286343));
#26944=CARTESIAN_POINT('Ctrl Pts',(-9.16940494659641,-1.07956620750791,
15.5108894520892));
#26945=CARTESIAN_POINT('Ctrl Pts',(-7.95240868713248,-1.14628955341283,
15.5586114755441));
#26946=CARTESIAN_POINT('Ctrl Pts',(-7.360678360457,-0.324490753397076,15.5983798284231));
#26947=CARTESIAN_POINT('Ctrl Pts',(-7.46068657418702,0.407081917027667,
15.6301945107264));
#26948=CARTESIAN_POINT('Ctrl Pts',(-7.88413511411916,1.01199674841518,15.6620091930296));
#26949=CARTESIAN_POINT('Ctrl Pts',(-8.87668188965118,1.21320028335118,15.7017775459087));
#26950=CARTESIAN_POINT('Ctrl Pts',(-9.72442683656734,0.33782473088057,15.7494995693635));
#26951=CARTESIAN_POINT('Ctrl Pts',(-9.44616547363274,-0.846612249150427,
15.7972215928184));
#26952=CARTESIAN_POINT('Ctrl Pts',(-8.29949020407744,-1.25407183081511,
15.8449436162733));
#26953=CARTESIAN_POINT('Ctrl Pts',(-7.33668119725462,-0.50924503049874,
15.8926656397281));
#26954=CARTESIAN_POINT('Ctrl Pts',(-7.44249701763682,0.703085044785891,
15.940387663183));
#26955=CARTESIAN_POINT('Ctrl Pts',(-8.51978535451018,1.26984600438471,15.9881096866378));
#26956=CARTESIAN_POINT('Ctrl Pts',(-9.57853041802029,0.669890693554712,
16.0358317100927));
#26957=CARTESIAN_POINT('Ctrl Pts',(-9.6473848859972,-0.544843601674845,
16.0835537335476));
#26958=CARTESIAN_POINT('Ctrl Pts',(-8.66080360141944,-1.2601136358619,16.1312757570025));
#26959=CARTESIAN_POINT('Ctrl Pts',(-7.71812331405291,-0.889997654174616,
16.1710441098815));
#26960=CARTESIAN_POINT('Ctrl Pts',(-7.40587711199952,-0.220869169870984,
16.2028587921847));
#26961=CARTESIAN_POINT('Ctrl Pts',(-7.43412333655584,0.516967103108417,
16.234673474488));
#26962=CARTESIAN_POINT('Ctrl Pts',(-8.15927934511513,1.22382409746097,16.274441827367));
#26963=CARTESIAN_POINT('Ctrl Pts',(-9.34631329395978,0.947269754287392,
16.3221638508219));
#26964=CARTESIAN_POINT('Ctrl Pts',(-9.75366233503884,-0.19899389665094,
16.3698858742767));
#26965=CARTESIAN_POINT('Ctrl Pts',(-9.01138473879162,-1.16278173533473,
16.4176078977316));
#26966=CARTESIAN_POINT('Ctrl Pts',(-7.79705255782462,-1.05815633227033,
16.4653299211865));
#26967=CARTESIAN_POINT('Ctrl Pts',(-7.32643878878709,-0.161507282602953,
16.5050982740655));
#26968=CARTESIAN_POINT('Ctrl Pts',(-7.5280384983639,0.548832220338187,16.5369129563688));
#26969=CARTESIAN_POINT('Ctrl Pts',(-8.03218094264503,1.08833594701741,16.568727638672));
#26970=CARTESIAN_POINT('Ctrl Pts',(-9.04304373573084,1.14844897424026,16.6084959915511));
#26971=CARTESIAN_POINT('Ctrl Pts',(-9.75980963534572,0.162650140327407,
16.6562180150059));
#26972=CARTESIAN_POINT('Ctrl Pts',(-9.31788680540282,-0.970734219451476,
16.7039400384608));
#26973=CARTESIAN_POINT('Ctrl Pts',(-8.12595390549439,-1.21394603873985,
16.7516620619157));
#26974=CARTESIAN_POINT('Ctrl Pts',(-7.2760636253747,-0.340310403120085,
16.7993840853705));
#26975=CARTESIAN_POINT('Ctrl Pts',(-7.50681993013901,0.645695886996063,
16.8391524382496));
#26976=CARTESIAN_POINT('Ctrl Pts',(-8.12404011840559,1.05099014478124,16.8709671205528));
#26977=CARTESIAN_POINT('Ctrl Pts',(-8.85828565453448,1.12914180496286,16.902781802856));
#26978=CARTESIAN_POINT('Ctrl Pts',(-9.66208453803124,0.513216288611988,
16.9425501557351));
#26979=CARTESIAN_POINT('Ctrl Pts',(-9.55915380641066,-0.701262194326414,
16.9902721791899));
#26980=CARTESIAN_POINT('Ctrl Pts',(-8.48339865398978,-1.26924707575363,
17.0379942026449));
#26981=CARTESIAN_POINT('Ctrl Pts',(-7.42286709434953,-0.673320246815119,
17.0857162260997));
#26982=CARTESIAN_POINT('Ctrl Pts',(-7.35173612228207,0.543434907326658,
17.1334382495546));
#26983=CARTESIAN_POINT('Ctrl Pts',(-8.17136948899973,1.13812644920779,17.1732066024336));
#26984=CARTESIAN_POINT('Ctrl Pts',(-8.90331979515647,1.0407974152085,17.2050212847369));
#26985=CARTESIAN_POINT('Ctrl Pts',(-9.50972840593837,0.619498485377158,
17.23683596704));
#26986=CARTESIAN_POINT('Ctrl Pts',(-9.71461689321606,-0.372205902885845,
17.2766043199191));
#26987=CARTESIAN_POINT('Ctrl Pts',(-8.84216750674715,-1.22331387974914,
17.324326343374));
#26988=CARTESIAN_POINT('Ctrl Pts',(-7.65700356119952,-0.949010404737396,
17.3720483668289));
#26989=CARTESIAN_POINT('Ctrl Pts',(-7.2448754144411,0.195544689997025,17.4197703902837));
#26990=CARTESIAN_POINT('Ctrl Pts',(-7.98717963800152,1.16225931174747,17.4674924137386));
#26991=CARTESIAN_POINT('Ctrl Pts',(-8.99612423756339,1.07572792473616,17.5072607666176));
#26992=CARTESIAN_POINT('Ctrl Pts',(-9.48598375104783,0.52322285818574,17.5390754489209));
#26993=CARTESIAN_POINT('Ctrl Pts',(-9.66893526453526,-0.192146232024172,
17.5708901312241));
#26994=CARTESIAN_POINT('Ctrl Pts',(-9.17503157966931,-1.07618018838531,
17.6106584841032));
#26995=CARTESIAN_POINT('Ctrl Pts',(-7.9583768197333,-1.14900817301593,17.658380507558));
#26996=CARTESIAN_POINT('Ctrl Pts',(-7.24156363400886,-0.166137463815073,
17.7061025310129));
#26997=CARTESIAN_POINT('Ctrl Pts',(-7.67874863455965,0.969082889035782,
17.7538245544677));
#26998=CARTESIAN_POINT('Ctrl Pts',(-8.87261967454383,1.21449002036524,17.8015465779226));
#26999=CARTESIAN_POINT('Ctrl Pts',(-9.57902171510171,0.488919180943277,
17.8413149308017));
#27000=CARTESIAN_POINT('Ctrl Pts',(-9.58798717630628,-0.249419367434415,
17.8731296131049));
#27001=CARTESIAN_POINT('Ctrl Pts',(-9.2582939446597,-0.910120937374646,
17.9049442954082));
#27002=CARTESIAN_POINT('Ctrl Pts',(-8.30637285397506,-1.25552377904448,
17.9447126482872));
#27003=CARTESIAN_POINT('Ctrl Pts',(-7.33862383613528,-0.514568612593541,
17.9924346717421));
#27004=CARTESIAN_POINT('Ctrl Pts',(-7.4396030778627,0.697726387385249,18.0401566951969));
#27005=CARTESIAN_POINT('Ctrl Pts',(-8.51297644133385,1.27019961542661,18.0878787186518));
#27006=CARTESIAN_POINT('Ctrl Pts',(-9.57641009434339,0.674664909580691,
18.1356007421067));
#27007=CARTESIAN_POINT('Ctrl Pts',(-9.63590327239758,-0.336234416608025,
18.1753690949857));
#27008=CARTESIAN_POINT('Ctrl Pts',(-9.15960407852556,-0.900471307844259,
18.207183777289));
#27009=CARTESIAN_POINT('Ctrl Pts',(-8.47798936265341,-1.1844177299411,18.2389984595921));
#27010=CARTESIAN_POINT('Ctrl Pts',(-7.53210607607463,-0.822807865453571,
18.2787668124713));
#27011=CARTESIAN_POINT('Ctrl Pts',(-7.28503401962905,0.370719729176766,
18.326488835926));
#27012=CARTESIAN_POINT('Ctrl Pts',(-8.15457897907752,1.22145325839214,18.374210859381));
#27013=CARTESIAN_POINT('Ctrl Pts',(-9.34087831913538,0.952102464794442,
18.4219328828358));
#27014=CARTESIAN_POINT('Ctrl Pts',(-9.7554577416763,-0.194054864120685,
18.4696549062907));
#27015=CARTESIAN_POINT('Ctrl Pts',(-9.13903952802435,-0.997475969022656,
18.5094232591697));
#27016=CARTESIAN_POINT('Ctrl Pts',(-8.40966837294719,-1.11254946578222,
18.541237941473));
#27017=CARTESIAN_POINT('Ctrl Pts',(-7.70841482017917,-0.881318744974411,
18.5730526237762));
#27018=CARTESIAN_POINT('Ctrl Pts',(-7.22968115822663,0.011021418212948,
18.6128209766553));
#27019=CARTESIAN_POINT('Ctrl Pts',(-7.82373204986715,1.07528466495283,18.6605430001101));
#27020=CARTESIAN_POINT('Ctrl Pts',(-9.03794533402332,1.14972977770192,18.708265023565));
#27021=CARTESIAN_POINT('Ctrl Pts',(-9.75885760069877,0.169861685563808,
18.7559870470199));
#27022=CARTESIAN_POINT('Ctrl Pts',(-9.32247807753752,-0.968174180297135,
18.8037090704747));
#27023=CARTESIAN_POINT('Ctrl Pts',(-8.330648257652,-1.17245461085662,18.8434774233538));
#27024=CARTESIAN_POINT('Ctrl Pts',(-7.70376873565747,-0.782267147681539,
18.875292105657));
#27025=CARTESIAN_POINT('Ctrl Pts',(-7.32473279588695,-0.148582724741135,
18.9071067879603));
#27026=CARTESIAN_POINT('Ctrl Pts',(-7.54652823945384,0.839477833694785,
18.9468751408393));
#27027=CARTESIAN_POINT('Ctrl Pts',(-8.69210621464535,1.25565546761611,18.9945971642941));
#27028=CARTESIAN_POINT('Ctrl Pts',(-9.65906691117085,0.517520665829651,
19.0423191877491));
#27029=CARTESIAN_POINT('Ctrl Pts',(-9.56315216209578,-0.695185537314083,
19.0900412112039));
#27030=CARTESIAN_POINT('Ctrl Pts',(-8.48854581274214,-1.27031501330109,
19.1377632346588));
#27031=CARTESIAN_POINT('Ctrl Pts',(-7.60481483699583,-0.775869416263104,
19.1775315875378));
#27032=CARTESIAN_POINT('Ctrl Pts',(-7.38602655189909,-0.0706347901850005,
19.2093462698411));
#27033=CARTESIAN_POINT('Ctrl Pts',(-7.51398572855607,0.656586387053644,
19.2411609521443));
#27034=CARTESIAN_POINT('Ctrl Pts',(-8.32818647186491,1.25869438029001,19.2809293050234));
#27035=CARTESIAN_POINT('Ctrl Pts',(-9.4668298755767,0.823902568725164,19.3286513284782));
#27036=CARTESIAN_POINT('Ctrl Pts',(-9.71515106657892,-0.366976333738334,
19.3763733519331));
#27037=CARTESIAN_POINT('Ctrl Pts',(-8.84916710494986,-1.2213344275343,19.4240953753879));
#27038=CARTESIAN_POINT('Ctrl Pts',(-7.66019738816671,-0.953185713584651,
19.4718173988428));
#27039=CARTESIAN_POINT('Ctrl Pts',(-7.31537823830772,-0.0010530338523334,
19.5115857517218));
#27040=CARTESIAN_POINT('Ctrl Pts',(-7.61133902610286,0.675431558435419,
19.5434004340251));
#27041=CARTESIAN_POINT('Ctrl Pts',(-8.18391407035424,1.14167399560261,19.5752151163283));
#27042=CARTESIAN_POINT('Ctrl Pts',(-9.19360265821437,1.06430577558419,19.6149834692074));
#27043=CARTESIAN_POINT('Ctrl Pts',(-9.77023039295916,-0.00949736081626473,
19.6627054926622));
#27044=CARTESIAN_POINT('Ctrl Pts',(-9.1788571469454,-1.07257480772814,19.7104275161171));
#27045=CARTESIAN_POINT('Ctrl Pts',(-7.96496540298764,-1.15209089531139,
19.758149539572));
#27046=CARTESIAN_POINT('Ctrl Pts',(-7.24124715966354,-0.171384708678441,
19.8058715630268));
#27047=CARTESIAN_POINT('Ctrl Pts',(-7.60343688127647,0.77427669556818,19.8456399159059));
#27048=CARTESIAN_POINT('Ctrl Pts',(-8.26986782341272,1.09222950791374,19.8774545982091));
#27049=CARTESIAN_POINT('Ctrl Pts',(-9.00793220370274,1.0702031132439,19.9092692805124));
#27050=CARTESIAN_POINT('Ctrl Pts',(-9.72089215495525,0.351075173421066,
19.9490376333914));
#27051=CARTESIAN_POINT('Ctrl Pts',(-9.45440202947589,-0.838267390032476,
19.9967596568463));
#27052=CARTESIAN_POINT('Ctrl Pts',(-8.31162487652084,-1.25530018600577,
20.0444816803012));
#27053=CARTESIAN_POINT('Ctrl Pts',(-7.34158951386127,-0.521210702752235,
20.092203703756));
#27054=CARTESIAN_POINT('Ctrl Pts',(-7.43593058134585,0.693965203528907,
20.1399257272109));
#27055=CARTESIAN_POINT('Ctrl Pts',(-8.32856409047539,1.17215167793282,20.1796940800899));
#27056=CARTESIAN_POINT('Ctrl Pts',(-9.04058452848265,0.976572825867848,
20.2115087623932));
#27057=CARTESIAN_POINT('Ctrl Pts',(-9.58433676096464,0.477015320483459,
20.2433234446964));
#27058=CARTESIAN_POINT('Ctrl Pts',(-9.65300483419814,-0.533302244266452,
20.2830917975755));
#27059=CARTESIAN_POINT('Ctrl Pts',(-8.67330901488357,-1.25838763360885,
20.3308138210303));
#27060=CARTESIAN_POINT('Ctrl Pts',(-7.53622422777799,-0.826075060154805,
20.3785358444852));
#27061=CARTESIAN_POINT('Ctrl Pts',(-7.28293104363061,0.36375624599658,20.4262578679401));
#27062=CARTESIAN_POINT('Ctrl Pts',(-8.14934077805168,1.22101168769447,20.4739798913949));
#27063=CARTESIAN_POINT('Ctrl Pts',(-9.13726516704792,0.998610501658501,
20.5137482442739));
#27064=CARTESIAN_POINT('Ctrl Pts',(-9.54776986598246,0.384843376709829,
20.5455629265772));
#27065=CARTESIAN_POINT('Ctrl Pts',(-9.63213434842366,-0.348714273115681,
20.5773776088804));
#27066=CARTESIAN_POINT('Ctrl Pts',(-9.02303531396696,-1.15769835957703,
20.6171459617595));
#27067=CARTESIAN_POINT('Ctrl Pts',(-7.80772900649456,-1.06505226285407,
20.6648679852143));
#27068=CARTESIAN_POINT('Ctrl Pts',(-7.2306578674812,0.00585617149092387,
20.7125900086692));
#27069=CARTESIAN_POINT('Ctrl Pts',(-7.81758560697748,1.07139444055647,20.760312032124));
#27070=CARTESIAN_POINT('Ctrl Pts',(-9.03369501670135,1.15282308294553,20.8080340555789));
#27071=CARTESIAN_POINT('Ctrl Pts',(-9.63530370681369,0.33825333767807,20.847802408458));
#27072=CARTESIAN_POINT('Ctrl Pts',(-9.54417435213954,-0.394494662818509,
20.8796170907612));
#27073=CARTESIAN_POINT('Ctrl Pts',(-9.12802395962112,-1.00444797441034,
20.9114317730645));
#27074=CARTESIAN_POINT('Ctrl Pts',(-8.13808955169642,-1.21772421296146,
20.9512001259435));
#27075=CARTESIAN_POINT('Ctrl Pts',(-7.27962651001226,-0.352510987055423,
20.9989221493984));
#27076=CARTESIAN_POINT('Ctrl Pts',(-7.54388736698447,0.834932558426133,
21.0466441728532));
#27077=CARTESIAN_POINT('Ctrl Pts',(-8.68491265495414,1.25673496056146,21.0943661963081));
#27078=CARTESIAN_POINT('Ctrl Pts',(-9.65787647902049,0.522640881251166,
21.1420882197629));
#27079=CARTESIAN_POINT('Ctrl Pts',(-9.57988922915072,-0.487000082052889,
21.181856572642));
#27080=CARTESIAN_POINT('Ctrl Pts',(-9.03155077607419,-0.981519174093523,
21.2136712549453));
#27081=CARTESIAN_POINT('Ctrl Pts',(-8.31775606126076,-1.17051995879953,
21.2454859372485));
#27082=CARTESIAN_POINT('Ctrl Pts',(-7.42957272949752,-0.684117599531321,
21.2852542901276));
#27083=CARTESIAN_POINT('Ctrl Pts',(-7.34644798530079,0.531877053878988,
21.3329763135824));
#27084=CARTESIAN_POINT('Ctrl Pts',(-8.32321542546207,1.25698486798265,21.3806983370373));
#27085=CARTESIAN_POINT('Ctrl Pts',(-9.46209601166041,0.829425533370407,
21.4284203604922));
#27086=CARTESIAN_POINT('Ctrl Pts',(-9.71760084736768,-0.362325279153129,
21.476142383947));
#27087=CARTESIAN_POINT('Ctrl Pts',(-8.99803592390773,-1.07484419598965,
21.5159107368261));
#27088=CARTESIAN_POINT('Ctrl Pts',(-8.25979972674399,-1.09005960634547,
21.5477254191293));
#27089=CARTESIAN_POINT('Ctrl Pts',(-7.59633087273917,-0.765971236790843,
21.5795401014325));
#27090=CARTESIAN_POINT('Ctrl Pts',(-7.24288209287525,0.182991800390507,
21.6193084543116));
#27091=CARTESIAN_POINT('Ctrl Pts',(-7.97561840692373,1.15697856328559,21.6670304777664));
#27092=CARTESIAN_POINT('Ctrl Pts',(-9.18872478998646,1.06626540213497,21.7147525012213));
#27093=CARTESIAN_POINT('Ctrl Pts',(-9.77026395203898,-0.00222333305725054,
21.7624745246762));
#27094=CARTESIAN_POINT('Ctrl Pts',(-9.18375288880803,-1.07066027220149,
21.810196548131));
#27095=CARTESIAN_POINT('Ctrl Pts',(-8.17339341325626,-1.13870890250796,
21.8499649010101));
#27096=CARTESIAN_POINT('Ctrl Pts',(-7.60514471543686,-0.667203219677276,
21.8817795833133));
#27097=CARTESIAN_POINT('Ctrl Pts',(-7.31543838241809,0.011983376276968,
21.9135942656166));
#27098=CARTESIAN_POINT('Ctrl Pts',(-7.66902808735548,0.960893912885179,
21.9533626184956));
#27099=CARTESIAN_POINT('Ctrl Pts',(-8.86042137271117,1.21806070667787,22.0010846419505));
#27100=CARTESIAN_POINT('Ctrl Pts',(-9.71848539326896,0.355748633900504,
22.0488066654053));
#27101=CARTESIAN_POINT('Ctrl Pts',(-9.45918665172335,-0.832788339384839,
22.0965286888602));
#27102=CARTESIAN_POINT('Ctrl Pts',(-8.31657993781219,-1.25705549289238,
22.144250712315));
#27103=CARTESIAN_POINT('Ctrl Pts',(-7.50796944462182,-0.647460581310789,
22.1840190651941));
#27104=CARTESIAN_POINT('Ctrl Pts',(-7.38672571254854,0.080910305633487,
22.2158337474974));
#27105=CARTESIAN_POINT('Ctrl Pts',(-7.61201181389946,0.78409617299229,22.2476484298006));
#27106=CARTESIAN_POINT('Ctrl Pts',(-8.50026737069875,1.27036662422184,22.2874167826797));
#27107=CARTESIAN_POINT('Ctrl Pts',(-9.56952131288912,0.685346344803542,
22.3351388061345));
#27108=CARTESIAN_POINT('Ctrl Pts',(-9.65424245939207,-0.52819323080524,
22.3828608295894));
#27109=CARTESIAN_POINT('Ctrl Pts',(-8.68051222872802,-1.25737456087645,
22.4305828530443));
#27110=CARTESIAN_POINT('Ctrl Pts',(-7.53882304902558,-0.830644509004543,
22.4783048764991));
#27111=CARTESIAN_POINT('Ctrl Pts',(-7.32615378357976,0.159420473437757,
22.5180732293781));
#27112=CARTESIAN_POINT('Ctrl Pts',(-7.71102053144895,0.789580594279784,
22.5498879116814));
#27113=CARTESIAN_POINT('Ctrl Pts',(-8.34147358890413,1.17396729261948,22.5817025939846));
#27114=CARTESIAN_POINT('Ctrl Pts',(-9.33137631260206,0.960544042857,22.6214709468637));
#27115=CARTESIAN_POINT('Ctrl Pts',(-9.75723671581043,-0.181469808722496,
22.6691929703186));
#27116=CARTESIAN_POINT('Ctrl Pts',(-9.0273139919783,-1.15464440326701,22.7169149937734));
#27117=CARTESIAN_POINT('Ctrl Pts',(-7.813839293024,-1.06899903426609,22.7646370172283));
#27118=CARTESIAN_POINT('Ctrl Pts',(-7.2296335405858,0.000700156646207271,
22.8123590406831));
#27119=CARTESIAN_POINT('Ctrl Pts',(-7.71658035743571,0.888585106109542,
22.8521273935622));
#27120=CARTESIAN_POINT('Ctrl Pts',(-8.41993760159213,1.11333558688271,22.8839420758655));
#27121=CARTESIAN_POINT('Ctrl Pts',(-9.1482159365314,0.991537153505591,22.9157567581687));
#27122=CARTESIAN_POINT('Ctrl Pts',(-9.75719482334863,0.18246261964937,22.9555251110477));
#27123=CARTESIAN_POINT('Ctrl Pts',(-9.33205756918401,-0.959820635651876,
23.0032471345026));
#27124=CARTESIAN_POINT('Ctrl Pts',(-8.14332345540958,-1.21821409722222,
23.0509691579575));
#27125=CARTESIAN_POINT('Ctrl Pts',(-7.28166514512249,-0.359493577759317,
23.0986911814123));
#27126=CARTESIAN_POINT('Ctrl Pts',(-7.5397392445049,0.831703500581703,23.1464132048672));
#27127=CARTESIAN_POINT('Ctrl Pts',(-8.48891880428909,1.18457040071786,23.1861815577462));
#27128=CARTESIAN_POINT('Ctrl Pts',(-9.16788455925829,0.894346874631236,
23.2179962400495));
#27129=CARTESIAN_POINT('Ctrl Pts',(-9.63895731995363,0.325739236935478,
23.2498109223527));
#27130=CARTESIAN_POINT('Ctrl Pts',(-9.57013920684436,-0.684568118888431,
23.2895792752318));
#27131=CARTESIAN_POINT('Ctrl Pts',(-8.50125588334141,-1.27026527694676,
23.3373012986866));
#27132=CARTESIAN_POINT('Ctrl Pts',(-7.43321036561117,-0.687912509039083,
23.3850233221415));
#27133=CARTESIAN_POINT('Ctrl Pts',(-7.34342114791428,0.525262610479453,
23.4327453455963));
#27134=CARTESIAN_POINT('Ctrl Pts',(-8.31796568955919,1.2572569113933,23.4804673690513));
#27135=CARTESIAN_POINT('Ctrl Pts',(-9.26665926046044,0.90308549180325,23.5202357219303));
#27136=CARTESIAN_POINT('Ctrl Pts',(-9.59024222976098,0.239370000426331,
23.5520504042335));
#27137=CARTESIAN_POINT('Ctrl Pts',(-9.57446457380535,-0.498854394380288,
23.5838650865367));
#27138=CARTESIAN_POINT('Ctrl Pts',(-8.86139783388378,-1.21787644573988,
23.6236334394159));
#27139=CARTESIAN_POINT('Ctrl Pts',(-7.66984196271033,-0.961464031663683,
23.6713554628706));
#27140=CARTESIAN_POINT('Ctrl Pts',(-7.24315013794179,0.177741858818465,
23.7190774863255));
#27141=CARTESIAN_POINT('Ctrl Pts',(-7.96900166016501,1.1539567644206,23.7667995097804));
#27142=CARTESIAN_POINT('Ctrl Pts',(-9.1849326520489,1.06990592744461,23.8145215332352));
#27143=CARTESIAN_POINT('Ctrl Pts',(-9.67065841860297,0.181352403097706,
23.8542898861143));
#27144=CARTESIAN_POINT('Ctrl Pts',(-9.48111405364124,-0.532298159311048,
23.8861045684176));
#27145=CARTESIAN_POINT('Ctrl Pts',(-8.98617748353237,-1.08025982136771,
23.9179192507208));
#27146=CARTESIAN_POINT('Ctrl Pts',(-7.97647741697682,-1.1574780933083,23.9576876035999));
#27147=CARTESIAN_POINT('Ctrl Pts',(-7.24312457211183,-0.183955456104287,
24.0054096270547));
#27148=CARTESIAN_POINT('Ctrl Pts',(-7.66579587118509,0.956748250899926,
24.0531316505096));
#27149=CARTESIAN_POINT('Ctrl Pts',(-8.85344033668265,1.22010465922611,24.1008536739644));
#27150=CARTESIAN_POINT('Ctrl Pts',(-9.71799949535745,0.36098290919776,24.1485756974193));
#27151=CARTESIAN_POINT('Ctrl Pts',(-9.50396937211297,-0.628788777742109,
24.1883440502983));
#27152=CARTESIAN_POINT('Ctrl Pts',(-8.89369929202849,-1.04447450141904,
24.2201587326016));
#27153=CARTESIAN_POINT('Ctrl Pts',(-8.16088209878099,-1.13504575953045,
24.2519734149049));
#27154=CARTESIAN_POINT('Ctrl Pts',(-7.34677078253822,-0.532816857293743,
24.2917417677839));
#27155=CARTESIAN_POINT('Ctrl Pts',(-7.42912560559831,0.683230182643023,
24.3394637912387));
#27156=CARTESIAN_POINT('Ctrl Pts',(-8.49511057720914,1.26934622450956,24.3871858146936));
#27157=CARTESIAN_POINT('Ctrl Pts',(-9.56557919629318,0.691459635471783,
24.4349078381484));
#27158=CARTESIAN_POINT('Ctrl Pts',(-9.65729967351157,-0.523916879966565,
24.4826298616034));
#27159=CARTESIAN_POINT('Ctrl Pts',(-8.84785192415903,-1.13239960526931,
24.5223982144823));
#27160=CARTESIAN_POINT('Ctrl Pts',(-8.11435874014051,-1.04747646052419,
24.5542128967857));
#27161=CARTESIAN_POINT('Ctrl Pts',(-7.50090443876472,-0.636504427852052,
24.5860275790888));
#27162=CARTESIAN_POINT('Ctrl Pts',(-7.27925573292454,0.351589058172031,
24.625795931968));
#27163=CARTESIAN_POINT('Ctrl Pts',(-8.13717079459291,1.21734564473828,24.6735179554228));
#27164=CARTESIAN_POINT('Ctrl Pts',(-9.32680884437268,0.963146343500833,
24.7212399788777));
#27165=CARTESIAN_POINT('Ctrl Pts',(-9.75825527430768,-0.174267368536162,
24.7689620023325));
#27166=CARTESIAN_POINT('Ctrl Pts',(-9.03242394654871,-1.15341066952121,
24.8166840257874));
#27167=CARTESIAN_POINT('Ctrl Pts',(-8.02215897329008,-1.08397314558436,
24.8564523786664));
#27168=CARTESIAN_POINT('Ctrl Pts',(-7.52301574135941,-0.539840601498972,
24.8882670609697));
#27169=CARTESIAN_POINT('Ctrl Pts',(-7.32797922977689,0.1723285853273,24.9200817432729));
#27170=CARTESIAN_POINT('Ctrl Pts',(-7.80684540644956,1.06459764271005,24.9598500961519));
#27171=CARTESIAN_POINT('Ctrl Pts',(-9.02209281164555,1.15801318951368,25.0075721196068));
#27172=CARTESIAN_POINT('Ctrl Pts',(-9.75544329080836,0.187419016367583,
25.0552941430617));
#27173=CARTESIAN_POINT('Ctrl Pts',(-9.33754026227136,-0.95504018770629,
25.1030161665166));
#27174=CARTESIAN_POINT('Ctrl Pts',(-8.14799508151347,-1.22062441757699,
25.1507381899714));
#27175=CARTESIAN_POINT('Ctrl Pts',(-7.42941034956166,-0.507116976179599,
25.1905065428505));
#27176=CARTESIAN_POINT('Ctrl Pts',(-7.4079460804348,0.230963965632277,25.2223212251537));
#27177=CARTESIAN_POINT('Ctrl Pts',(-7.72640636278891,0.897152557607554,
25.254135907457));
#27178=CARTESIAN_POINT('Ctrl Pts',(-8.67234334103518,1.25862194650527,25.293904260336));
#27179=CARTESIAN_POINT('Ctrl Pts',(-9.65249805028128,0.534156994859609,
25.3416262837909));
#27180=CARTESIAN_POINT('Ctrl Pts',(-9.57205747047455,-0.679673836580168,
25.3893483072457));
#27181=CARTESIAN_POINT('Ctrl Pts',(-8.50852993454981,-1.27023725786806,
25.4370703307006));
#27182=CARTESIAN_POINT('Ctrl Pts',(-7.43516627654756,-0.69279186832866,
25.4847923541554));
#27183=CARTESIAN_POINT('Ctrl Pts',(-7.3585670705502,0.316955351308209,25.5245607070345));
#27184=CARTESIAN_POINT('Ctrl Pts',(-7.82524545288061,0.889175133368002,
25.5563753893377));
#27185=CARTESIAN_POINT('Ctrl Pts',(-8.50195525644396,1.18462061611619,25.588190071641));
#27186=CARTESIAN_POINT('Ctrl Pts',(-9.45382504141213,0.839076409988411,
25.62795842452));
#27187=CARTESIAN_POINT('Ctrl Pts',(-9.72106814323682,-0.350097187409116,
25.6756804479749));
#27188=CARTESIAN_POINT('Ctrl Pts',(-8.86605075290398,-1.21543020796356,
25.7234024714297));
#27189=CARTESIAN_POINT('Ctrl Pts',(-7.67536132038316,-0.966202100566644,
25.7711244948846));
#27190=CARTESIAN_POINT('Ctrl Pts',(-7.24143684011856,0.172772115843602,
25.8188465183395));
#27191=CARTESIAN_POINT('Ctrl Pts',(-7.84416476429791,0.986514049959185,
25.8586148712185));
#27192=CARTESIAN_POINT('Ctrl Pts',(-8.57148318594807,1.11391932867017,25.8904295535218));
#27193=CARTESIAN_POINT('Ctrl Pts',(-9.27655097556757,0.894593991428686,
25.922244235825));
#27194=CARTESIAN_POINT('Ctrl Pts',(-9.77032336852924,0.0104866959759273,
25.962012588704));
#27195=CARTESIAN_POINT('Ctrl Pts',(-9.19437562557584,-1.06368131583936,
26.0097346121589));
#27196=CARTESIAN_POINT('Ctrl Pts',(-7.98159672426513,-1.15867242473413,
26.0574566356138));
#27197=CARTESIAN_POINT('Ctrl Pts',(-7.24419858603817,-0.191149835864602,
26.1051786590687));
#27198=CARTESIAN_POINT('Ctrl Pts',(-7.66124858591289,0.954110840935556,
26.1529006825235));
#27199=CARTESIAN_POINT('Ctrl Pts',(-8.64947777999604,1.17515370077396,26.1926690354026));
#27200=CARTESIAN_POINT('Ctrl Pts',(-9.28287334059143,0.795635248873192,
26.2244837177058));
#27201=CARTESIAN_POINT('Ctrl Pts',(-9.67258325123935,0.168458736990063,
26.2562984000091));
#27202=CARTESIAN_POINT('Ctrl Pts',(-9.46754748980759,-0.823215212681873,
26.2960667528881));
#27203=CARTESIAN_POINT('Ctrl Pts',(-8.32917960185085,-1.25872786679082,
26.343788776343));
#27204=CARTESIAN_POINT('Ctrl Pts',(-7.3498608497893,-0.537069529283282,
26.3915107997978));
#27205=CARTESIAN_POINT('Ctrl Pts',(-7.42523070112171,0.67708670438005,26.4392328232527));
#27206=CARTESIAN_POINT('Ctrl Pts',(-8.48994607585931,1.27032686739802,26.4869548467075));
#27207=CARTESIAN_POINT('Ctrl Pts',(-9.38192137064002,0.790913726751365,
26.5267231995866));
#27208=CARTESIAN_POINT('Ctrl Pts',(-9.61261794082105,0.0894842691280413,
26.5585378818898));
#27209=CARTESIAN_POINT('Ctrl Pts',(-9.49698897915128,-0.639799032983159,
26.5903525641931));
#27210=CARTESIAN_POINT('Ctrl Pts',(-8.6930986353653,-1.25560517219546,26.6301209170721));
#27211=CARTESIAN_POINT('Ctrl Pts',(-7.54725738779159,-0.840152941994423,
26.677842940527));
#27212=CARTESIAN_POINT('Ctrl Pts',(-7.2788101728749,0.346351194971367,26.7255649639818));
#27213=CARTESIAN_POINT('Ctrl Pts',(-8.13020571177932,1.21524797282651,26.7732869874367));
#27214=CARTESIAN_POINT('Ctrl Pts',(-9.32354478705541,0.967266982346513,
26.8210090108916));
#27215=CARTESIAN_POINT('Ctrl Pts',(-9.68443415000749,0.0211085634589513,
26.8607773637706));
#27216=CARTESIAN_POINT('Ctrl Pts',(-9.3999686838854,-0.660289697544845,
26.8925920460739));
#27217=CARTESIAN_POINT('Ctrl Pts',(-8.83536920081072,-1.13615902333382,
26.9244067283771));
#27218=CARTESIAN_POINT('Ctrl Pts',(-7.82451547856594,-1.07589594883839,
26.9641750812562));
#27219=CARTESIAN_POINT('Ctrl Pts',(-7.22979086994386,-0.0120090374988551,
27.011897104711));
#27220=CARTESIAN_POINT('Ctrl Pts',(-7.80308142666439,1.06092801182352,27.0596191281659));
#27221=CARTESIAN_POINT('Ctrl Pts',(-9.01545298211099,1.16098392507927,27.1073411516207));
#27222=CARTESIAN_POINT('Ctrl Pts',(-9.75567088378897,0.192670867098664,
27.1550631750756));
#27223=CARTESIAN_POINT('Ctrl Pts',(-9.40954314716847,-0.758986884336038,
27.1948315279547));
#27224=CARTESIAN_POINT('Ctrl Pts',(-8.74859067031979,-1.08817682170144,
27.2266462102579));
#27225=CARTESIAN_POINT('Ctrl Pts',(-8.01025916428869,-1.0786490351324,27.2584608925611));
#27226=CARTESIAN_POINT('Ctrl Pts',(-7.28522654001878,-0.371694595533894,
27.2982292454403));
#27227=CARTESIAN_POINT('Ctrl Pts',(-7.53154286743781,0.821989193024468,
27.345951268895));
#27228=CARTESIAN_POINT('Ctrl Pts',(-8.66709585666284,1.25830946861972,27.3936732923499));
#27229=CARTESIAN_POINT('Ctrl Pts',(-9.64942034682812,0.540747924043256,
27.4413953158048));
#27230=CARTESIAN_POINT('Ctrl Pts',(-9.57566576368643,-0.675851016317035,
27.4891173392597));
#27231=CARTESIAN_POINT('Ctrl Pts',(-8.69125590043384,-1.16908126650995,
27.5288856921387));
#27232=CARTESIAN_POINT('Ctrl Pts',(-7.97602635588388,-0.985584971948125,
27.5607003744419));
#27233=CARTESIAN_POINT('Ctrl Pts',(-7.42389453276778,-0.495304805698656,
27.5925150567452));
#27234=CARTESIAN_POINT('Ctrl Pts',(-7.33813159580452,0.513705404639772,
27.6322834096242));
#27235=CARTESIAN_POINT('Ctrl Pts',(-8.30541128545435,1.2552731508445,27.6800054330791));
#27236=CARTESIAN_POINT('Ctrl Pts',(-9.44965216623517,0.842273415997902,
27.727727456534));
#27237=CARTESIAN_POINT('Ctrl Pts',(-9.72305292585927,-0.34309909881355,
27.7754494799888));
#27238=CARTESIAN_POINT('Ctrl Pts',(-8.87128072736936,-1.21490001765905,
27.8231715034437));
#27239=CARTESIAN_POINT('Ctrl Pts',(-7.87973267238346,-1.00925629522272,
27.8629398563227));
#27240=CARTESIAN_POINT('Ctrl Pts',(-7.45889571320355,-0.402526993718913,
27.894754538626));
#27241=CARTESIAN_POINT('Ctrl Pts',(-7.3621241700199,0.329497227154213,27.9265692209292));
#27242=CARTESIAN_POINT('Ctrl Pts',(-7.95743978257428,1.1486774316103,27.9663375738082));
#27243=CARTESIAN_POINT('Ctrl Pts',(-9.17414040953262,1.07661978399751,28.0140595972632));
#27244=CARTESIAN_POINT('Ctrl Pts',(-9.76925935148402,0.0156346666823883,
28.061781620718));
#27245=CARTESIAN_POINT('Ctrl Pts',(-9.20045532592656,-1.05968758954737,
28.1095036441729));
#27246=CARTESIAN_POINT('Ctrl Pts',(-7.98589880216476,-1.16169332864071,
28.1572256676277));
#27247=CARTESIAN_POINT('Ctrl Pts',(-7.37058564730116,-0.35742558256636,
28.1969940205068));
#27248=CARTESIAN_POINT('Ctrl Pts',(-7.44929649627935,0.376760220734205,
28.22880870281));
#27249=CARTESIAN_POINT('Ctrl Pts',(-7.85506071766296,0.993671549987,28.2606233851133));
#27250=CARTESIAN_POINT('Ctrl Pts',(-8.84124247215261,1.22367683912963,28.3003917379923));
#27251=CARTESIAN_POINT('Ctrl Pts',(-9.71423056098527,0.37312142237029,28.3481137614471));
#27252=CARTESIAN_POINT('Ctrl Pts',(-9.4701110321357,-0.818625878810101,
28.3958357849021));
#27253=CARTESIAN_POINT('Ctrl Pts',(-8.33639040638821,-1.25968541784629,
28.4435578083568));
#27254=CARTESIAN_POINT('Ctrl Pts',(-7.35113779671057,-0.542168856810177,
28.4912798318118));
#27255=CARTESIAN_POINT('Ctrl Pts',(-7.4120206186405,0.468647727901989,28.5310481846908));
#27256=CARTESIAN_POINT('Ctrl Pts',(-7.95190825959645,0.972379329670431,
28.5628628669941));
#27257=CARTESIAN_POINT('Ctrl Pts',(-8.66240088239154,1.1734375912628,28.5946775492973));
#27258=CARTESIAN_POINT('Ctrl Pts',(-9.55869172269085,0.702141914089626,
28.6344459021764));
#27259=CARTESIAN_POINT('Ctrl Pts',(-9.66239137790161,-0.51227115470021,
28.6821679256312));
#27260=CARTESIAN_POINT('Ctrl Pts',(-8.69804002694774,-1.25381174500308,
28.7298899490861));
#27261=CARTESIAN_POINT('Ctrl Pts',(-7.55208407768074,-0.845594970502949,
28.7776119725409));
#27262=CARTESIAN_POINT('Ctrl Pts',(-7.27643948470255,0.341659331902066,
28.8253339959958));
#27263=CARTESIAN_POINT('Ctrl Pts',(-7.98383831473153,1.06625838374073,28.8651023488749));
#27264=CARTESIAN_POINT('Ctrl Pts',(-8.7217111041732,1.09396997251344,28.8969170311781));
#27265=CARTESIAN_POINT('Ctrl Pts',(-9.39057170098815,0.781160600976512,
28.9287317134813));
#27266=CARTESIAN_POINT('Ctrl Pts',(-9.76003577755879,-0.161682533818022,
28.9685000663604));
#27267=CARTESIAN_POINT('Ctrl Pts',(-9.04389413728366,-1.14793494130765,
29.0162220898153));
#27268=CARTESIAN_POINT('Ctrl Pts',(-7.82942578787744,-1.07777272054675,
29.0639441132701));
#27269=CARTESIAN_POINT('Ctrl Pts',(-7.22988053396106,-0.0192825748490968,
29.111666136725));
#27270=CARTESIAN_POINT('Ctrl Pts',(-7.79821866312692,1.05893083384072,29.1593881601798));
#27271=CARTESIAN_POINT('Ctrl Pts',(-8.80728164041408,1.14407521357788,29.1991565130589));
#27272=CARTESIAN_POINT('Ctrl Pts',(-9.38343094294497,0.682257445520128,
29.2309711953621));
#27273=CARTESIAN_POINT('Ctrl Pts',(-9.68459549643142,0.00807318411422593,
29.2627858776654));
#27274=CARTESIAN_POINT('Ctrl Pts',(-9.34711913065458,-0.946688199617532,
29.3025542305444));
#27275=CARTESIAN_POINT('Ctrl Pts',(-8.1602548489812,-1.22398743093969,29.3502762539993));
#27276=CARTESIAN_POINT('Ctrl Pts',(-7.2877070281187,-0.376327816437086,
29.3979982774541));
#27277=CARTESIAN_POINT('Ctrl Pts',(-7.52686125179537,0.816432151475763,
29.445720300909));
#27278=CARTESIAN_POINT('Ctrl Pts',(-8.66209281831706,1.25997621452946,29.4934423243638));
#27279=CARTESIAN_POINT('Ctrl Pts',(-9.48095999247722,0.664170613867274,
29.533210677243));
#27280=CARTESIAN_POINT('Ctrl Pts',(-9.61444029499092,-0.0620612536963943,
29.5650253595461));
#27281=CARTESIAN_POINT('Ctrl Pts',(-9.40124341722056,-0.768925025649959,
29.5968400418494));
#27282=CARTESIAN_POINT('Ctrl Pts',(-8.52101122107249,-1.27024239984106,
29.6366083947285));
#27283=CARTESIAN_POINT('Ctrl Pts',(-7.44261890700309,-0.703265592319027,
29.6843304181833));
#27284=CARTESIAN_POINT('Ctrl Pts',(-7.33627786239381,0.508411815248644,
29.7320524416382));
#27285=CARTESIAN_POINT('Ctrl Pts',(-8.2995618713472,1.25445422207268,29.779774465093));
#27286=CARTESIAN_POINT('Ctrl Pts',(-9.25349370071878,0.914194267159221,
29.8195428179721));
#27287=CARTESIAN_POINT('Ctrl Pts',(-9.58672570471092,0.255051675598665,
29.8513575002753));
#27288=CARTESIAN_POINT('Ctrl Pts',(-9.58134081666635,-0.482923354571183,
29.8831721825786));
#27289=CARTESIAN_POINT('Ctrl Pts',(-8.87961978715692,-1.21312531614331,
29.9229405354576));
#27290=CARTESIAN_POINT('Ctrl Pts',(-7.68284834089023,-0.972316947591664,
29.9706625589125));
#27291=CARTESIAN_POINT('Ctrl Pts',(-7.31615319782486,-0.031134755764136,
30.0104309117915));
#27292=CARTESIAN_POINT('Ctrl Pts',(-7.59495772883202,0.655650918756826,
30.0422455940948));
#27293=CARTESIAN_POINT('Ctrl Pts',(-7.87606563100468,0.891954634492901,
30.0581529352464));
#27294=CARTESIAN_POINT('Ctrl Pts',(-8.03748311344989,0.969001292713786,
30.0661066058222));
#27295=CARTESIAN_POINT('Ctrl Pts',(-7.90984029786111,-0.827606761449139,
1.8));
#27296=CARTESIAN_POINT('Ctrl Pts',(-7.77197649840879,-0.729297198731152,
1.80795367057581));
#27297=CARTESIAN_POINT('Ctrl Pts',(-7.54863701760608,-0.4628715196836,1.82386101172743));
#27298=CARTESIAN_POINT('Ctrl Pts',(-7.40132815197149,0.223190340066621,
1.85567569403067));
#27299=CARTESIAN_POINT('Ctrl Pts',(-7.8975843624851,1.04057513890883,1.89544404690973));
#27300=CARTESIAN_POINT('Ctrl Pts',(-9.05290778687487,1.06881550059125,1.94316607036458));
#27301=CARTESIAN_POINT('Ctrl Pts',(-9.58740885957362,0.272911730207072,
1.98293442324364));
#27302=CARTESIAN_POINT('Ctrl Pts',(-9.47139510427018,-0.416034089157043,
2.01474910554688));
#27303=CARTESIAN_POINT('Ctrl Pts',(-9.05259577107697,-0.975943072842501,
2.04656378785012));
#27304=CARTESIAN_POINT('Ctrl Pts',(-8.10737674978987,-1.1367365362355,2.08633214072917));
#27305=CARTESIAN_POINT('Ctrl Pts',(-7.33160128421964,-0.283165032011243,
2.13405416418404));
#27306=CARTESIAN_POINT('Ctrl Pts',(-7.62947585871493,0.829120622165689,
2.1817761876389));
#27307=CARTESIAN_POINT('Ctrl Pts',(-8.72792114609409,1.18088449447148,2.22949821109376));
#27308=CARTESIAN_POINT('Ctrl Pts',(-9.4663990177441,0.569107464161922,2.26926656397281));
#27309=CARTESIAN_POINT('Ctrl Pts',(-9.54924456809875,-0.124914290005348,
2.30108124627605));
#27310=CARTESIAN_POINT('Ctrl Pts',(-9.30568364649701,-0.780136065581114,
2.3328959285793));
#27311=CARTESIAN_POINT('Ctrl Pts',(-8.44448253610224,-1.20134333884891,
2.37266428145834));
#27312=CARTESIAN_POINT('Ctrl Pts',(-7.45877664796192,-0.601610010654219,
2.42038630491321));
#27313=CARTESIAN_POINT('Ctrl Pts',(-7.43142063634725,0.549701954261673,
2.46810832836807));
#27314=CARTESIAN_POINT('Ctrl Pts',(-8.38397803243201,1.19692518514985,2.51583035182294));
#27315=CARTESIAN_POINT('Ctrl Pts',(-9.44509012097467,0.743724623326929,
2.56355237527779));
#27316=CARTESIAN_POINT('Ctrl Pts',(-9.60315220690443,-0.201811312771686,
2.60332072815685));
#27317=CARTESIAN_POINT('Ctrl Pts',(-9.21178449951522,-0.781003980273609,
2.63513541046009));
#27318=CARTESIAN_POINT('Ctrl Pts',(-8.5988604131823,-1.11709346661785,2.66695009276333));
#27319=CARTESIAN_POINT('Ctrl Pts',(-7.67200907556847,-0.872212497622945,
2.70671844564238));
#27320=CARTESIAN_POINT('Ctrl Pts',(-7.31894661150667,0.226289253311605,
2.75444046909725));
#27321=CARTESIAN_POINT('Ctrl Pts',(-8.05154383597101,1.11485849141834,2.80216249255211));
#27322=CARTESIAN_POINT('Ctrl Pts',(-9.19537976741075,0.981091778944714,
2.84988451600697));
#27323=CARTESIAN_POINT('Ctrl Pts',(-9.70133158308663,-0.0559097679809395,
2.89760653946183));
#27324=CARTESIAN_POINT('Ctrl Pts',(-9.20222130442427,-0.874389043558423,
2.93737489234089));
#27325=CARTESIAN_POINT('Ctrl Pts',(-8.52729507837894,-1.05634272967533,
2.96918957464412));
#27326=CARTESIAN_POINT('Ctrl Pts',(-7.84387270007337,-0.90948772098803,
3.00100425694737));
#27327=CARTESIAN_POINT('Ctrl Pts',(-7.3031589137604,-0.117876702228567,
3.04077260982642));
#27328=CARTESIAN_POINT('Ctrl Pts',(-7.75488071429994,0.943870403632135,
3.08849463328128));
#27329=CARTESIAN_POINT('Ctrl Pts',(-8.89028197036155,1.13653082253155,3.13621665673614));
#27330=CARTESIAN_POINT('Ctrl Pts',(-9.66779092684549,0.286981604349885,
3.18393868019101));
#27331=CARTESIAN_POINT('Ctrl Pts',(-9.37193042071709,-0.828287897935989,
3.23166070364586));
#27332=CARTESIAN_POINT('Ctrl Pts',(-8.45896286510886,-1.12070821481404,
3.27142905652493));
#27333=CARTESIAN_POINT('Ctrl Pts',(-7.82949920621424,-0.816721293551666,
3.30324373882816));
#27334=CARTESIAN_POINT('Ctrl Pts',(-7.4087428992097,-0.258512841293276,
3.33505842113141));
#27335=CARTESIAN_POINT('Ctrl Pts',(-7.51776071245581,0.693923254147438,
3.37482677401045));
#27336=CARTESIAN_POINT('Ctrl Pts',(-8.55405558131559,1.20132097455938,3.42254879746531));
#27337=CARTESIAN_POINT('Ctrl Pts',(-9.53876020395445,0.604151939157171,
3.47027082092018));
#27338=CARTESIAN_POINT('Ctrl Pts',(-9.57091178241385,-0.547030203992542,
3.51799284437504));
#27339=CARTESIAN_POINT('Ctrl Pts',(-8.61746895833269,-1.19688117390714,
3.5657148678299));
#27340=CARTESIAN_POINT('Ctrl Pts',(-7.73570976145469,-0.820689576164182,
3.60548322070896));
#27341=CARTESIAN_POINT('Ctrl Pts',(-7.4585680161445,-0.178953649869286,
3.6372979030122));
#27342=CARTESIAN_POINT('Ctrl Pts',(-7.50559368937304,0.518485331080344,
3.66911258531544));
#27343=CARTESIAN_POINT('Ctrl Pts',(-8.21119763983049,1.1674402328969,3.70888093819449));
#27344=CARTESIAN_POINT('Ctrl Pts',(-9.32687871186513,0.873135548271195,
3.75660296164935));
#27345=CARTESIAN_POINT('Ctrl Pts',(-9.68084973637808,-0.222747002236243,
3.80432498510421));
#27346=CARTESIAN_POINT('Ctrl Pts',(-8.95197025619296,-1.11436842081398,
3.85204700855908));
#27347=CARTESIAN_POINT('Ctrl Pts',(-7.80574215880651,-0.982002826150276,
3.89976903201393));
#27348=CARTESIAN_POINT('Ctrl Pts',(-7.38504307341408,-0.120590219414704,
3.939537384893));
#27349=CARTESIAN_POINT('Ctrl Pts',(-7.59532800195641,0.546052709685047,
3.97135206719623));
#27350=CARTESIAN_POINT('Ctrl Pts',(-8.08721095204589,1.0427253478503,4.00316674949948));
#27351=CARTESIAN_POINT('Ctrl Pts',(-9.04542379982193,1.071837851176,4.04293510237852));
#27352=CARTESIAN_POINT('Ctrl Pts',(-9.69660396175139,0.119302340762661,
4.09065712583339));
#27353=CARTESIAN_POINT('Ctrl Pts',(-9.24728286443354,-0.941058259319486,
4.13837914928825));
#27354=CARTESIAN_POINT('Ctrl Pts',(-8.11269623164964,-1.13845943309904,
4.18610117274311));
#27355=CARTESIAN_POINT('Ctrl Pts',(-7.3324614462396,-0.288404622204439,
4.23382319619797));
#27356=CARTESIAN_POINT('Ctrl Pts',(-7.57791048256601,0.638296068450016,
4.27359154907703));
#27357=CARTESIAN_POINT('Ctrl Pts',(-8.17310957881519,1.0048619996478,4.30540623138027));
#27358=CARTESIAN_POINT('Ctrl Pts',(-8.87006013423126,1.05864368236586,4.33722091368351));
#27359=CARTESIAN_POINT('Ctrl Pts',(-9.61375947960335,0.453721635167941,
4.37698926656257));
#27360=CARTESIAN_POINT('Ctrl Pts',(-9.48299272702672,-0.692689965571268,
4.42471129001742));
#27361=CARTESIAN_POINT('Ctrl Pts',(-8.44942055884309,-1.20060986462784,
4.4724333134723));
#27362=CARTESIAN_POINT('Ctrl Pts',(-7.46223022206171,-0.607559032348711,
4.52015533692714));
#27363=CARTESIAN_POINT('Ctrl Pts',(-7.42834802491375,0.545788919747837,
4.56787736038202));
#27364=CARTESIAN_POINT('Ctrl Pts',(-8.22029040779656,1.08601726192072,4.60764571326106));
#27365=CARTESIAN_POINT('Ctrl Pts',(-8.91024806509605,0.973807738151371,
4.6394603955643));
#27366=CARTESIAN_POINT('Ctrl Pts',(-9.47250745857794,0.558480252265651,
4.67127507786755));
#27367=CARTESIAN_POINT('Ctrl Pts',(-9.63914480964413,-0.385580864782726,
4.71104343074659));
#27368=CARTESIAN_POINT('Ctrl Pts',(-8.79017906601008,-1.16700051389882,
4.75876545420146));
#27369=CARTESIAN_POINT('Ctrl Pts',(-7.6762153949145,-0.874872134276515,
4.80648747765633));
#27370=CARTESIAN_POINT('Ctrl Pts',(-7.3176700873064,0.219522361823356,4.85420950111118));
#27371=CARTESIAN_POINT('Ctrl Pts',(-8.04665782451571,1.11391398795103,4.90193152456605));
#27372=CARTESIAN_POINT('Ctrl Pts',(-8.99902690165246,1.00431225253282,4.9416998774451));
#27373=CARTESIAN_POINT('Ctrl Pts',(-9.4473933441329,0.468028671441437,4.97351455974835));
#27374=CARTESIAN_POINT('Ctrl Pts',(-9.60086385536787,-0.213938591901918,
5.00532924205157));
#27375=CARTESIAN_POINT('Ctrl Pts',(-9.10920461013546,-1.03691525382525,
5.04509759493064));
#27376=CARTESIAN_POINT('Ctrl Pts',(-7.95590503741594,-1.07240606184469,
5.09281961838549));
#27377=CARTESIAN_POINT('Ctrl Pts',(-7.30459975514546,-0.122640048561389,
5.14054164184036));
#27378=CARTESIAN_POINT('Ctrl Pts',(-7.74948793304144,0.939588062472147,
5.18826366529521));
#27379=CARTESIAN_POINT('Ctrl Pts',(-8.88596892398453,1.13901338462022,5.23598568875008));
#27380=CARTESIAN_POINT('Ctrl Pts',(-9.53449109503047,0.433011689753366,
5.27575404162913));
#27381=CARTESIAN_POINT('Ctrl Pts',(-9.52269065962012,-0.265911264380261,
5.30756872393238));
#27382=CARTESIAN_POINT('Ctrl Pts',(-9.19255643359114,-0.882063793300652,
5.33938340623562));
#27383=CARTESIAN_POINT('Ctrl Pts',(-8.2822812089624,-1.18276034286533,5.37915175911467));
#27384=CARTESIAN_POINT('Ctrl Pts',(-7.38687368970327,-0.455020776575932,
5.42687378256953));
#27385=CARTESIAN_POINT('Ctrl Pts',(-7.51573379599412,0.689378246365011,
5.47459580602439));
#27386=CARTESIAN_POINT('Ctrl Pts',(-8.54717542720796,1.20161082254544,5.52231782947927));
#27387=CARTESIAN_POINT('Ctrl Pts',(-9.53712273626146,0.608851320566278,
5.57003985293409));
#27388=CARTESIAN_POINT('Ctrl Pts',(-9.56564774971944,-0.349379196115496,
5.60980820581319));
#27389=CARTESIAN_POINT('Ctrl Pts',(-9.09943307031321,-0.870221224754611,
5.6416228881164));
#27390=CARTESIAN_POINT('Ctrl Pts',(-8.44663234976153,-1.1201887533217,5.67343757041967));
#27391=CARTESIAN_POINT('Ctrl Pts',(-7.56149427253223,-0.752017619564837,
5.7132059232987));
#27392=CARTESIAN_POINT('Ctrl Pts',(-7.36048402589915,0.384184115444124,
5.76092794675357));
#27393=CARTESIAN_POINT('Ctrl Pts',(-8.20669107470487,1.16532922440469,5.80864997020842));
#27394=CARTESIAN_POINT('Ctrl Pts',(-9.32186521390639,0.87785628662166,5.8563719936633));
#27395=CARTESIAN_POINT('Ctrl Pts',(-9.6826861022262,-0.218121718833277,
5.90409401711814));
#27396=CARTESIAN_POINT('Ctrl Pts',(-9.07730820347234,-0.961450044133312,
5.94386236999722));
#27397=CARTESIAN_POINT('Ctrl Pts',(-8.3839558401117,-1.05030411727003,5.97567705230044));
#27398=CARTESIAN_POINT('Ctrl Pts',(-7.72672464100434,-0.812229135361763,
6.00749173460371));
#27399=CARTESIAN_POINT('Ctrl Pts',(-7.29822264555078,0.0453286990641955,
6.04726008748272));
#27400=CARTESIAN_POINT('Ctrl Pts',(-7.88960083185226,1.03610180258269,6.09498211093762));
#27401=CARTESIAN_POINT('Ctrl Pts',(-9.04063450660887,1.07318994459191,6.14270413439245));
#27402=CARTESIAN_POINT('Ctrl Pts',(-9.69590116689828,0.126152640883819,
6.19042615784734));
#27403=CARTESIAN_POINT('Ctrl Pts',(-9.25169784766887,-0.938761868865437,
6.23814818130218));
#27404=CARTESIAN_POINT('Ctrl Pts',(-8.30753474198256,-1.10482038070298,
6.27791653418125));
#27405=CARTESIAN_POINT('Ctrl Pts',(-7.72504936719716,-0.718370727770171,
6.30973121648449));
#27406=CARTESIAN_POINT('Ctrl Pts',(-7.38378353437386,-0.10831320799179,
6.34154589878772));
#27407=CARTESIAN_POINT('Ctrl Pts',(-7.62080949776357,0.820577577930954,
6.38131425166678));
#27408=CARTESIAN_POINT('Ctrl Pts',(-8.71628317856752,1.18292674179735,6.42903627512163));
#27409=CARTESIAN_POINT('Ctrl Pts',(-9.61102220693821,0.457877693931059,
6.4767582985765));
#27410=CARTESIAN_POINT('Ctrl Pts',(-9.48694324310275,-0.687049579495082,
6.52448032203136));
#27411=CARTESIAN_POINT('Ctrl Pts',(-8.45426188445871,-1.20176184221855,
6.57220234548622));
#27412=CARTESIAN_POINT('Ctrl Pts',(-7.63158681559905,-0.709598118880692,
6.61197069836528));
#27413=CARTESIAN_POINT('Ctrl Pts',(-7.44392618126472,-0.0362363792399661,
6.64378538066852));
#27414=CARTESIAN_POINT('Ctrl Pts',(-7.58499054185306,0.648404688957481,
6.67560006297176));
#27415=CARTESIAN_POINT('Ctrl Pts',(-8.37199588104198,1.19580033707788,6.71536841585081));
#27416=CARTESIAN_POINT('Ctrl Pts',(-9.43752891208507,0.75308275029716,6.76309043930567));
#27417=CARTESIAN_POINT('Ctrl Pts',(-9.6397939597727,-0.380646891718703,
6.81081246276053));
#27418=CARTESIAN_POINT('Ctrl Pts',(-8.7968570426639,-1.16531969262148,6.85853448621541));
#27419=CARTESIAN_POINT('Ctrl Pts',(-7.67912294882438,-0.878910898486879,
6.90625650967025));
#27420=CARTESIAN_POINT('Ctrl Pts',(-7.37898454940943,0.0315485133979244,
6.94602486254932));
#27421=CARTESIAN_POINT('Ctrl Pts',(-7.67763196849479,0.663562963521021,
6.97783954485255));
#27422=CARTESIAN_POINT('Ctrl Pts',(-8.23225858352771,1.08902960614752,7.0096542271558));
#27423=CARTESIAN_POINT('Ctrl Pts',(-9.18558342222681,0.988078373305267,
7.04942258003485));
#27424=CARTESIAN_POINT('Ctrl Pts',(-9.70173552716583,-0.0438840806899642,
7.09714460348971));
#27425=CARTESIAN_POINT('Ctrl Pts',(-9.1129237266811,-1.03360864556213,7.14486662694457));
#27426=CARTESIAN_POINT('Ctrl Pts',(-7.96205500537781,-1.07550419457644,
7.19258865039944));
#27427=CARTESIAN_POINT('Ctrl Pts',(-7.30415612412785,-0.127596728660616,
7.24031067385429));
#27428=CARTESIAN_POINT('Ctrl Pts',(-7.67286987062921,0.757315454911259,
7.28007902673335));
#27429=CARTESIAN_POINT('Ctrl Pts',(-8.31223670967161,1.03987976834036,7.31189370903659));
#27430=CARTESIAN_POINT('Ctrl Pts',(-9.0100487876404,0.998759822673581,7.34370839133983));
#27431=CARTESIAN_POINT('Ctrl Pts',(-9.66495359809054,0.298674764454046,
7.38347674421889));
#27432=CARTESIAN_POINT('Ctrl Pts',(-9.38010405357526,-0.819457713778441,
7.43119876767374));
#27433=CARTESIAN_POINT('Ctrl Pts',(-8.28725724730808,-1.18269304897191,
7.47892079112861));
#27434=CARTESIAN_POINT('Ctrl Pts',(-7.38949758043417,-0.461387544184974,
7.52664281458347));
#27435=CARTESIAN_POINT('Ctrl Pts',(-7.51215524722395,0.685919999007586,
7.57436483803833));
#27436=CARTESIAN_POINT('Ctrl Pts',(-8.3699756368797,1.11389614154802,7.61413319091739));
#27437=CARTESIAN_POINT('Ctrl Pts',(-9.03837480793247,0.909262092018708,
7.64594787322062));
#27438=CARTESIAN_POINT('Ctrl Pts',(-9.53919359505327,0.421601258490334,
7.67776255552388));
#27439=CARTESIAN_POINT('Ctrl Pts',(-9.57641663143542,-0.536330808545463,
7.71753090840291));
#27440=CARTESIAN_POINT('Ctrl Pts',(-8.62942769870831,-1.1955511534843,7.76525293185779));
#27441=CARTESIAN_POINT('Ctrl Pts',(-7.56530144703071,-0.755222445367275,
7.81297495531264));
#27442=CARTESIAN_POINT('Ctrl Pts',(-7.35830271009327,0.377652469884987,
7.86069697876751));
#27443=CARTESIAN_POINT('Ctrl Pts',(-8.20172212694212,1.16505528240931,7.90841900222237));
#27444=CARTESIAN_POINT('Ctrl Pts',(-9.13046741664916,0.927459856653719,
7.94818735510142));
#27445=CARTESIAN_POINT('Ctrl Pts',(-9.50205876271649,0.335385184320401,
7.98000203740466));
#27446=CARTESIAN_POINT('Ctrl Pts',(-9.56173842624569,-0.361085119319172,
8.01181671970791));
#27447=CARTESIAN_POINT('Ctrl Pts',(-8.96313370552467,-1.10987867419497,
8.05158507258695));
#27448=CARTESIAN_POINT('Ctrl Pts',(-7.8156562002608,-0.988821345617644,
8.09930709604182));
#27449=CARTESIAN_POINT('Ctrl Pts',(-7.29900498391781,0.0404140848611043,
8.14702911949668));
#27450=CARTESIAN_POINT('Ctrl Pts',(-7.88367768647865,1.03258941290634,8.19475114295154));
#27451=CARTESIAN_POINT('Ctrl Pts',(-9.03669748888875,1.07623385286206,8.24247316640641));
#27452=CARTESIAN_POINT('Ctrl Pts',(-9.58361051778681,0.288893050976006,
8.28224151928546));
#27453=CARTESIAN_POINT('Ctrl Pts',(-9.47724572542883,-0.401989773414212,
8.3140562015887));
#27454=CARTESIAN_POINT('Ctrl Pts',(-9.06669282573335,-0.967744899455822,
8.34587088389194));
#27455=CARTESIAN_POINT('Ctrl Pts',(-8.12407617387874,-1.14236805696769,
8.385639236771));
#27456=CARTESIAN_POINT('Ctrl Pts',(-7.3354977594041,-0.300047698604244,
8.43336126022585));
#27457=CARTESIAN_POINT('Ctrl Pts',(-7.61818561524077,0.816349017112872,
8.48108328368072));
#27458=CARTESIAN_POINT('Ctrl Pts',(-8.70950569765978,1.18414587464495,8.52880530713558));
#27459=CARTESIAN_POINT('Ctrl Pts',(-9.61003638925317,0.462755567399852,
8.57652733059045));
#27460=CARTESIAN_POINT('Ctrl Pts',(-9.50850068784772,-0.490507198490582,
8.61629568346948));
#27461=CARTESIAN_POINT('Ctrl Pts',(-8.97603188696186,-0.943397386255697,
8.64811036577274));
#27462=CARTESIAN_POINT('Ctrl Pts',(-8.2953882361285,-1.10263546797924,8.67992504807597));
#27463=CARTESIAN_POINT('Ctrl Pts',(-7.46827901092664,-0.617960598526543,
8.71969340095504));
#27464=CARTESIAN_POINT('Ctrl Pts',(-7.42302642728513,0.53499720883791,8.76741542440988));
#27465=CARTESIAN_POINT('Ctrl Pts',(-8.36724490293383,1.19431922496139,8.81513744786476));
#27466=CARTESIAN_POINT('Ctrl Pts',(-9.43320107257588,0.758439086501866,
8.86285947131961));
#27467=CARTESIAN_POINT('Ctrl Pts',(-9.64223992169735,-0.376312983972933,
8.91058149477448));
#27468=CARTESIAN_POINT('Ctrl Pts',(-8.94175347011682,-1.03078844619066,
8.95034984765353));
#27469=CARTESIAN_POINT('Ctrl Pts',(-8.24275566496688,-1.02490503847523,
8.98216452995676));
#27470=CARTESIAN_POINT('Ctrl Pts',(-7.62383052256787,-0.699998568553337,
9.01397921226003));
#27471=CARTESIAN_POINT('Ctrl Pts',(-7.315438978406,0.207698547770401,9.05374756513905));
#27472=CARTESIAN_POINT('Ctrl Pts',(-8.03557255959679,1.10923452993093,9.10146958859394));
#27473=CARTESIAN_POINT('Ctrl Pts',(-9.18102141880938,0.990066742210993,
9.14919161204878));
#27474=CARTESIAN_POINT('Ctrl Pts',(-9.70196712207443,-0.0370017194560962,
9.19691363550366));
#27475=CARTESIAN_POINT('Ctrl Pts',(-9.11760907802098,-1.03193145478362,
9.24463565895851));
#27476=CARTESIAN_POINT('Ctrl Pts',(-8.15965436942419,-1.06856717192152,
9.28440401183757));
#27477=CARTESIAN_POINT('Ctrl Pts',(-7.63488434792032,-0.606778290914648,
9.3162186941408));
#27478=CARTESIAN_POINT('Ctrl Pts',(-7.37939961054365,0.0438829842956811,
9.34803337644406));
#27479=CARTESIAN_POINT('Ctrl Pts',(-7.74006457714768,0.932106031371996,
9.38780172932309));
#27480=CARTESIAN_POINT('Ctrl Pts',(-8.87452398480516,1.1427273841981,9.43552375277797));
#27481=CARTESIAN_POINT('Ctrl Pts',(-9.66280451573322,0.303163297745353,
9.48324577623282));
#27482=CARTESIAN_POINT('Ctrl Pts',(-9.38478218192171,-0.814404432910586,
9.53096779968769));
#27483=CARTESIAN_POINT('Ctrl Pts',(-8.29189791040081,-1.18449019452684,
9.57868982314254));
#27484=CARTESIAN_POINT('Ctrl Pts',(-7.54347150337463,-0.585426497780913,
9.61845817602161));
#27485=CARTESIAN_POINT('Ctrl Pts',(-7.44875116596018,0.10714884380356,9.65027285832483));
#27486=CARTESIAN_POINT('Ctrl Pts',(-7.68125394638234,0.766371873730981,
9.6820875406281));
#27487=CARTESIAN_POINT('Ctrl Pts',(-8.5351536477378,1.20211801487063,9.72185589350713));
#27488=CARTESIAN_POINT('Ctrl Pts',(-9.5308974546648,0.619148227612896,9.769577916962));
#27489=CARTESIAN_POINT('Ctrl Pts',(-9.57772813351517,-0.531530241039361,
9.81729994041686));
#27490=CARTESIAN_POINT('Ctrl Pts',(-8.63627180399159,-1.19479039384633,
9.86502196387173));
#27491=CARTESIAN_POINT('Ctrl Pts',(-7.56763512943757,-0.759617830732582,
9.91274398732659));
#27492=CARTESIAN_POINT('Ctrl Pts',(-7.3935899270475,0.183105706163565,9.95251234020563));
#27493=CARTESIAN_POINT('Ctrl Pts',(-7.77509480916662,0.768841628751572,
9.98432702250888));
#27494=CARTESIAN_POINT('Ctrl Pts',(-8.38224154600145,1.11525956425949,10.0161417048121));
#27495=CARTESIAN_POINT('Ctrl Pts',(-9.31310554851392,0.886105449481985,
10.0559100576912));
#27496=CARTESIAN_POINT('Ctrl Pts',(-9.68471526164804,-0.206261578120577,
10.103632081146));
#27497=CARTESIAN_POINT('Ctrl Pts',(-8.96726644348741,-1.10710631725235,
10.1513541046009));
#27498=CARTESIAN_POINT('Ctrl Pts',(-7.82132982660755,-0.992723972480789,
10.1990761280558));
#27499=CARTESIAN_POINT('Ctrl Pts',(-7.29789403096364,0.0355631808608681,
10.2467981515106));
#27500=CARTESIAN_POINT('Ctrl Pts',(-7.7830759135267,0.862375094372996,10.2865665043897));
#27501=CARTESIAN_POINT('Ctrl Pts',(-8.45482491875085,1.05572922562212,10.3183811866929));
#27502=CARTESIAN_POINT('Ctrl Pts',(-9.14063560990152,0.920465623739701,
10.3501958689962));
#27503=CARTESIAN_POINT('Ctrl Pts',(-9.69467389428866,0.138122362168207,
10.3899642218752));
#27504=CARTESIAN_POINT('Ctrl Pts',(-9.2609922463669,-0.931120234319938,
10.4376862453301));
#27505=CARTESIAN_POINT('Ctrl Pts',(-8.12901546541348,-1.14297541618665,
10.4854082687849));
#27506=CARTESIAN_POINT('Ctrl Pts',(-7.33723505164926,-0.306711207290376,
10.5331302922398));
#27507=CARTESIAN_POINT('Ctrl Pts',(-7.61417160911282,0.813407377962594,
10.5808523156946));
#27508=CARTESIAN_POINT('Ctrl Pts',(-8.52205763101126,1.12124235117773,10.6206206685737));
#27509=CARTESIAN_POINT('Ctrl Pts',(-9.1565775804327,0.82795583618433,10.6524353508769));
#27510=CARTESIAN_POINT('Ctrl Pts',(-9.58672406848702,0.276950804532839,
10.6842500331802));
#27511=CARTESIAN_POINT('Ctrl Pts',(-9.49384665052284,-0.677194459420877,
10.7240183860592));
#27512=CARTESIAN_POINT('Ctrl Pts',(-8.46629056479243,-1.20206395993249,
10.7717404095141));
#27513=CARTESIAN_POINT('Ctrl Pts',(-7.47161698421242,-0.621651590321344,
10.819462432969));
#27514=CARTESIAN_POINT('Ctrl Pts',(-7.41998046699672,0.528821234560362,
10.8671844564238));
#27515=CARTESIAN_POINT('Ctrl Pts',(-8.36228464496208,1.19472088021117,10.9149064798787));
#27516=CARTESIAN_POINT('Ctrl Pts',(-9.25028639986432,0.833511408043712,
10.9546748327577));
#27517=CARTESIAN_POINT('Ctrl Pts',(-9.53825303203799,0.196559475127789,
10.986489515061));
#27518=CARTESIAN_POINT('Ctrl Pts',(-9.50304176070681,-0.501575692631294,
11.0183041973642));
#27519=CARTESIAN_POINT('Ctrl Pts',(-8.80852576484242,-1.162383479345,11.0580725502433));
#27520=CARTESIAN_POINT('Ctrl Pts',(-7.68802200901459,-0.88700948808109,
11.1057945736981));
#27521=CARTESIAN_POINT('Ctrl Pts',(-7.31554839363375,0.202723257387539,
11.153516597153));
#27522=CARTESIAN_POINT('Ctrl Pts',(-8.02922823218693,1.10655683650717,11.2012386206079));
#27523=CARTESIAN_POINT('Ctrl Pts',(-9.17753300181366,0.993615887593974,
11.2489606440627));
#27524=CARTESIAN_POINT('Ctrl Pts',(-9.6127555314957,0.139449188904468,11.2887289969418));
#27525=CARTESIAN_POINT('Ctrl Pts',(-9.41378702564638,-0.530658324686323,
11.320543679245));
#27526=CARTESIAN_POINT('Ctrl Pts',(-8.9303832558628,-1.03558737064206,11.3523583615483));
#27527=CARTESIAN_POINT('Ctrl Pts',(-7.97280061774567,-1.08091827257034,
11.3921267144273));
#27528=CARTESIAN_POINT('Ctrl Pts',(-7.30558733143117,-0.139543781491302,
11.4398487378822));
#27529=CARTESIAN_POINT('Ctrl Pts',(-7.73689209512053,0.928271863421417,
11.487570761337));
#27530=CARTESIAN_POINT('Ctrl Pts',(-8.86797410775294,1.1448533293894,11.5352927847919));
#27531=CARTESIAN_POINT('Ctrl Pts',(-9.66248851983205,0.308129748457519,
11.5830148082468));
#27532=CARTESIAN_POINT('Ctrl Pts',(-9.43276373142163,-0.622593583732446,
11.6227831611258));
#27533=CARTESIAN_POINT('Ctrl Pts',(-8.84385591278509,-0.999183715360338,
11.6545978434291));
#27534=CARTESIAN_POINT('Ctrl Pts',(-8.14791577199536,-1.06475708288359,
11.6864125257323));
#27535=CARTESIAN_POINT('Ctrl Pts',(-7.39408166832453,-0.472512586382552,
11.7261808786113));
#27536=CARTESIAN_POINT('Ctrl Pts',(-7.50542089758475,0.675948591854042,
11.7739029020662));
#27537=CARTESIAN_POINT('Ctrl Pts',(-8.53024583237525,1.20129410076524,11.8216249255211));
#27538=CARTESIAN_POINT('Ctrl Pts',(-9.52733504953497,0.625041427257073,
11.8693469489759));
#27539=CARTESIAN_POINT('Ctrl Pts',(-9.5807386046118,-0.527567596737633,
11.9170689724308));
#27540=CARTESIAN_POINT('Ctrl Pts',(-8.79805580683824,-1.08112611899371,
11.9568373253098));
#27541=CARTESIAN_POINT('Ctrl Pts',(-8.10629732601575,-0.980613680455361,
11.9886520076131));
#27542=CARTESIAN_POINT('Ctrl Pts',(-7.53708701106063,-0.574864788356556,
12.0204666899163));
#27543=CARTESIAN_POINT('Ctrl Pts',(-7.35449056110284,0.366239847672738,
12.0602350427954));
#27544=CARTESIAN_POINT('Ctrl Pts',(-8.19010517108621,1.16192051569936,12.1079570662502));
#27545=CARTESIAN_POINT('Ctrl Pts',(-9.30885492721204,0.888693441876452,
12.1556790897051));
#27546=CARTESIAN_POINT('Ctrl Pts',(-9.68587697728314,-0.199474019712831,
12.20340111316));
#27547=CARTESIAN_POINT('Ctrl Pts',(-8.97213579691505,-1.10607924214188,
12.2511231366148));
#27548=CARTESIAN_POINT('Ctrl Pts',(-8.01804765583374,-1.0126168510908,12.2908914894939));
#27549=CARTESIAN_POINT('Ctrl Pts',(-7.56066617820273,-0.484000988662495,
12.3227061717971));
#27550=CARTESIAN_POINT('Ctrl Pts',(-7.39567193745142,0.195270272771156,
12.3545208541003));
#27551=CARTESIAN_POINT('Ctrl Pts',(-7.87332769792352,1.02645278821577,12.3942892069794));
#27552=CARTESIAN_POINT('Ctrl Pts',(-9.02586111564668,1.08146390454855,12.4420112304343));
#27553=CARTESIAN_POINT('Ctrl Pts',(-9.6931526167034,0.142860631957331,12.4897332538892));
#27554=CARTESIAN_POINT('Ctrl Pts',(-9.26631175410989,-0.926747206795693,
12.537455277344));
#27555=CARTESIAN_POINT('Ctrl Pts',(-8.13336992371389,-1.14538460256293,
12.5851773007989));
#27556=CARTESIAN_POINT('Ctrl Pts',(-7.47298807192611,-0.450463593150824,
12.6249456536779));
#27557=CARTESIAN_POINT('Ctrl Pts',(-7.47295403032462,0.248558970813969,
12.6567603359812));
#27558=CARTESIAN_POINT('Ctrl Pts',(-7.79260946040346,0.87021237272846,12.6885750182844));
#27559=CARTESIAN_POINT('Ctrl Pts',(-8.69766342022542,1.1862768112589,12.7283433711635));
#27560=CARTESIAN_POINT('Ctrl Pts',(-9.60526325861529,0.473800822018835,
12.7760653946183));
#27561=CARTESIAN_POINT('Ctrl Pts',(-9.49579632937404,-0.672615787292102,
12.8237874180732));
#27562=CARTESIAN_POINT('Ctrl Pts',(-8.47317463994588,-1.20223728516817,
12.871509441528));
#27563=CARTESIAN_POINT('Ctrl Pts',(-7.47333377788248,-0.626322575825536,
12.9192314649829));
#27564=CARTESIAN_POINT('Ctrl Pts',(-7.42858998248594,0.331287674885324,
12.958999817862));
#27565=CARTESIAN_POINT('Ctrl Pts',(-7.88591997196862,0.859948082718679,
12.9908145001652));
#27566=CARTESIAN_POINT('Ctrl Pts',(-8.53439517357149,1.1209317201308,13.0226291824684));
#27567=CARTESIAN_POINT('Ctrl Pts',(-9.42563953786609,0.767798766972735,
13.0623975353475));
#27568=CARTESIAN_POINT('Ctrl Pts',(-9.64585690315083,-0.3648370146958,13.1101195588024));
#27569=CARTESIAN_POINT('Ctrl Pts',(-8.81299594463815,-1.16019647713199,
13.1578415822572));
#27570=CARTESIAN_POINT('Ctrl Pts',(-7.69311471065889,-0.891644671175397,
13.2055636057121));
#27571=CARTESIAN_POINT('Ctrl Pts',(-7.31379059716063,0.198067547168361,
13.2532856291669));
#27572=CARTESIAN_POINT('Ctrl Pts',(-7.90649716126405,0.951538401522895,
13.293053982046));
#27573=CARTESIAN_POINT('Ctrl Pts',(-8.59824584912319,1.0521182152822,13.3248686643492));
#27574=CARTESIAN_POINT('Ctrl Pts',(-9.25941346804454,0.82520429816681,13.3566833466525));
#27575=CARTESIAN_POINT('Ctrl Pts',(-9.70237252804341,-0.0249760771994319,
13.3964516995315));
#27576=CARTESIAN_POINT('Ctrl Pts',(-9.12785291712797,-1.0256192296581,13.4441737229864));
#27577=CARTESIAN_POINT('Ctrl Pts',(-7.97761211552232,-1.0821890893279,13.4918957464413));
#27578=CARTESIAN_POINT('Ctrl Pts',(-7.30640600133578,-0.146381201468398,
13.5396177698961));
#27579=CARTESIAN_POINT('Ctrl Pts',(-7.7325166226112,0.92590105630011,13.587339793351));
#27580=CARTESIAN_POINT('Ctrl Pts',(-8.67373303242592,1.10792047666089,13.62710814623));
#27581=CARTESIAN_POINT('Ctrl Pts',(-9.26267752728879,0.731387705097111,
13.6589228285333));
#27582=CARTESIAN_POINT('Ctrl Pts',(-9.61422274017161,0.127195261094417,
13.6907375108365));
#27583=CARTESIAN_POINT('Ctrl Pts',(-9.39295689585196,-0.805575249605032,
13.7305058637156));
#27584=CARTESIAN_POINT('Ctrl Pts',(-8.30377480362676,-1.18641888138164,
13.7782278871704));
#27585=CARTESIAN_POINT('Ctrl Pts',(-7.39688891086951,-0.476621707380971,
13.8259499106253));
#27586=CARTESIAN_POINT('Ctrl Pts',(-7.501566439608,0.670242131825176,13.8736719340801));
#27587=CARTESIAN_POINT('Ctrl Pts',(-8.52538569762017,1.20236394946876,13.921393957535));
#27588=CARTESIAN_POINT('Ctrl Pts',(-9.35627520405521,0.724198677215438,
13.9611623104141));
#27589=CARTESIAN_POINT('Ctrl Pts',(-9.55530897590372,0.0541105458815738,
13.9929769927173));
#27590=CARTESIAN_POINT('Ctrl Pts',(-9.42585582610759,-0.632820621047547,
14.0247916750206));
#27591=CARTESIAN_POINT('Ctrl Pts',(-8.64823070713109,-1.19346183771799,
14.0645600278996));
#27592=CARTESIAN_POINT('Ctrl Pts',(-7.57535517021029,-0.768847207534589,
14.1122820513545));
#27593=CARTESIAN_POINT('Ctrl Pts',(-7.35392503631861,0.361295591631145,
14.1600040748093));
#27594=CARTESIAN_POINT('Ctrl Pts',(-8.18345660789396,1.16012687698571,14.2077260982642));
#27595=CARTESIAN_POINT('Ctrl Pts',(-9.30587941362775,0.892682402266787,
14.2554481217191));
#27596=CARTESIAN_POINT('Ctrl Pts',(-9.62138890029986,-0.0125651679110466,
14.2952164745981));
#27597=CARTESIAN_POINT('Ctrl Pts',(-9.33348430715714,-0.649545145098795,
14.3270311569014));
#27598=CARTESIAN_POINT('Ctrl Pts',(-8.78614034549885,-1.08434065304129,
14.3588458392046));
#27599=CARTESIAN_POINT('Ctrl Pts',(-7.83124303309593,-0.99954370581937,
14.3986141920837));
#27600=CARTESIAN_POINT('Ctrl Pts',(-7.2976937506755,0.0235323740098842,
14.4463362155385));
#27601=CARTESIAN_POINT('Ctrl Pts',(-7.86966509538718,1.02308368911568,14.4940582389934));
#27602=CARTESIAN_POINT('Ctrl Pts',(-9.01965957764054,1.0844574741122,14.5417802624482));
#27603=CARTESIAN_POINT('Ctrl Pts',(-9.69351226740367,0.147824112333504,
14.5895022859031));
#27604=CARTESIAN_POINT('Ctrl Pts',(-9.33983295487833,-0.743203577124169,
14.6292706387821));
#27605=CARTESIAN_POINT('Ctrl Pts',(-8.7053415739125,-1.0365518915288,14.6610853210854));
#27606=CARTESIAN_POINT('Ctrl Pts',(-8.00693334672862,-1.00725181786108,
14.6929000033886));
#27607=CARTESIAN_POINT('Ctrl Pts',(-7.34026993918294,-0.318354655404035,
14.7326683562677));
#27608=CARTESIAN_POINT('Ctrl Pts',(-7.60614864303216,0.804440079539016,
14.7803903797225));
#27609=CARTESIAN_POINT('Ctrl Pts',(-8.69268923442672,1.18612528247478,14.8281124031774));
#27610=CARTESIAN_POINT('Ctrl Pts',(-9.60253195424284,0.480122254696041,
14.8758344266322));
#27611=CARTESIAN_POINT('Ctrl Pts',(-9.49931581731957,-0.669097450884765,
14.9235564500871));
#27612=CARTESIAN_POINT('Ctrl Pts',(-8.64886402084744,-1.11153517775476,
14.9633248029661));
#27613=CARTESIAN_POINT('Ctrl Pts',(-7.97709618774838,-0.918246475208985,
14.9951394852694));
#27614=CARTESIAN_POINT('Ctrl Pts',(-7.46809306529431,-0.439134409383918,
15.0269541675726));
#27615=CARTESIAN_POINT('Ctrl Pts',(-7.4146575515378,0.518030172478034,15.0667225204517));
#27616=CARTESIAN_POINT('Ctrl Pts',(-8.35035012993273,1.19318859338258,15.1144445439066));
#27617=CARTESIAN_POINT('Ctrl Pts',(-9.42177866202504,0.770938669116064,
15.1621665673614));
#27618=CARTESIAN_POINT('Ctrl Pts',(-9.64792730494328,-0.358269358952444,
15.2098885908163));
#27619=CARTESIAN_POINT('Ctrl Pts',(-8.81795958293278,-1.15983848287083,
15.2576106142711));
#27620=CARTESIAN_POINT('Ctrl Pts',(-7.88532479520075,-0.938000704162233,
15.2973789671502));
#27621=CARTESIAN_POINT('Ctrl Pts',(-7.50376303095584,-0.352302076284569,
15.3291936494535));
#27622=CARTESIAN_POINT('Ctrl Pts',(-7.43230033380396,0.343058292157666,
15.3610083317567));
#27623=CARTESIAN_POINT('Ctrl Pts',(-8.01814288331926,1.10187833907963,15.4007766846357));
#27624=CARTESIAN_POINT('Ctrl Pts',(-9.16750412307632,1.00026625060447,15.4484987080906));
#27625=CARTESIAN_POINT('Ctrl Pts',(-9.70150859744452,-0.0200766297906168,
15.4962207315455));
#27626=CARTESIAN_POINT('Ctrl Pts',(-9.13371290888423,-1.02200475985614,
15.5439427550003));
#27627=CARTESIAN_POINT('Ctrl Pts',(-7.98160573727265,-1.08517048015587,
15.5916647784552));
#27628=CARTESIAN_POINT('Ctrl Pts',(-7.4214259111463,-0.307189213773918,
15.6314331313343));
#27629=CARTESIAN_POINT('Ctrl Pts',(-7.51610178164494,0.385376694787397,
15.6632478136375));
#27630=CARTESIAN_POINT('Ctrl Pts',(-7.91697244650555,0.958038040322487,
15.6950624959408));
#27631=CARTESIAN_POINT('Ctrl Pts',(-8.85659756807664,1.14851359334971,15.7348308488197));
#27632=CARTESIAN_POINT('Ctrl Pts',(-9.65914155738177,0.319812236207544,
15.7825528722747));
#27633=CARTESIAN_POINT('Ctrl Pts',(-9.39571682675819,-0.801471685911283,
15.8302748957295));
#27634=CARTESIAN_POINT('Ctrl Pts',(-8.31018119647929,-1.18720590861515,
15.8779969191844));
#27635=CARTESIAN_POINT('Ctrl Pts',(-7.39870825395651,-0.482092567814215,
15.9257189426392));
#27636=CARTESIAN_POINT('Ctrl Pts',(-7.49888207502137,0.665597216138805,
15.9734409660941));
#27637=CARTESIAN_POINT('Ctrl Pts',(-8.51873041814767,1.20213901819083,16.0211629895489));
#27638=CARTESIAN_POINT('Ctrl Pts',(-9.52102419768294,0.634172756274771,
16.0688850130038));
#27639=CARTESIAN_POINT('Ctrl Pts',(-9.58620741064431,-0.5157930568929,16.1166070364587));
#27640=CARTESIAN_POINT('Ctrl Pts',(-8.65222970570018,-1.19292557033944,
16.1643290599136));
#27641=CARTESIAN_POINT('Ctrl Pts',(-7.75981223837764,-0.842543822233083,
16.2040974127926));
#27642=CARTESIAN_POINT('Ctrl Pts',(-7.46421470806744,-0.209092634934189,
16.2359120950958));
#27643=CARTESIAN_POINT('Ctrl Pts',(-7.49095487068437,0.48940290682626,16.2677267773991));
#27644=CARTESIAN_POINT('Ctrl Pts',(-8.17744624771311,1.15857095575367,16.3074951302781));
#27645=CARTESIAN_POINT('Ctrl Pts',(-9.30118867072826,0.896762228214262,
16.355217153733));
#27646=CARTESIAN_POINT('Ctrl Pts',(-9.6868182467658,-0.18838373056243,16.4029391771878));
#27647=CARTESIAN_POINT('Ctrl Pts',(-8.9841181888876,-1.1007833145585,16.4506612006427));
#27648=CARTESIAN_POINT('Ctrl Pts',(-7.83453304963084,-1.00173643888757,
16.4983832240976));
#27649=CARTESIAN_POINT('Ctrl Pts',(-7.38901196100714,-0.152895867269504,
16.5381515769766));
#27650=CARTESIAN_POINT('Ctrl Pts',(-7.5798625650184,0.519569006187027,16.5699662592799));
#27651=CARTESIAN_POINT('Ctrl Pts',(-8.05712461167899,1.03030690516145,16.6017809415831));
#27652=CARTESIAN_POINT('Ctrl Pts',(-9.01408915809622,1.08721476271011,16.6415492944621));
#27653=CARTESIAN_POINT('Ctrl Pts',(-9.69263777884286,0.15397778890258,16.6892713179171));
#27654=CARTESIAN_POINT('Ctrl Pts',(-9.27427785561657,-0.918975590320485,
16.7369933413719));
#27655=CARTESIAN_POINT('Ctrl Pts',(-8.14589768896835,-1.14921958576742,
16.7847153648267));
#27656=CARTESIAN_POINT('Ctrl Pts',(-7.34132275359406,-0.322165374757602,
16.8324373882816));
#27657=CARTESIAN_POINT('Ctrl Pts',(-7.55977535075367,0.611267993885054,
16.8722057411606));
#27658=CARTESIAN_POINT('Ctrl Pts',(-8.14408594319423,0.994952345727702,
16.9040204234639));
#27659=CARTESIAN_POINT('Ctrl Pts',(-8.83918220279198,1.0689370334114,16.9358351057671));
#27660=CARTESIAN_POINT('Ctrl Pts',(-9.60012329115488,0.485852082206321,
16.9756034586462));
#27661=CARTESIAN_POINT('Ctrl Pts',(-9.50268072865149,-0.663871558339279,
17.023325482101));
#27662=CARTESIAN_POINT('Ctrl Pts',(-8.48428382203488,-1.20157202386707,
17.0710475055559));
#27663=CARTESIAN_POINT('Ctrl Pts',(-7.480298800651,-0.637419449003703,17.1187695290108));
#27664=CARTESIAN_POINT('Ctrl Pts',(-7.41296046464096,0.514459472793085,
17.1664915524657));
#27665=CARTESIAN_POINT('Ctrl Pts',(-8.18889175657724,1.07744262493511,17.2062599053447));
#27666=CARTESIAN_POINT('Ctrl Pts',(-8.881815165691,0.985303082841596,17.2380745876479));
#27667=CARTESIAN_POINT('Ctrl Pts',(-9.45589064371805,0.586467412907256,
17.2698892699512));
#27668=CARTESIAN_POINT('Ctrl Pts',(-9.64985467091836,-0.352360236686092,
17.3096576228302));
#27669=CARTESIAN_POINT('Ctrl Pts',(-8.82392345937827,-1.15808794236697,
17.3573796462851));
#27670=CARTESIAN_POINT('Ctrl Pts',(-7.70195133285558,-0.898410068830963,
17.4051016697399));
#27671=CARTESIAN_POINT('Ctrl Pts',(-7.31179746852686,0.185118432340318,
17.4528236931948));
#27672=CARTESIAN_POINT('Ctrl Pts',(-8.01452273397517,1.10028874610208,17.5005457166497));
#27673=CARTESIAN_POINT('Ctrl Pts',(-8.96967136313036,1.01837113068638,17.5403140695287));
#27674=CARTESIAN_POINT('Ctrl Pts',(-9.43341203133604,0.495325110968304,
17.572128751832));
#27675=CARTESIAN_POINT('Ctrl Pts',(-9.60660874341056,-0.181901176927666,
17.6039434341352));
#27676=CARTESIAN_POINT('Ctrl Pts',(-9.13903953521102,-1.01879928006603,
17.6437117870143));
#27677=CARTESIAN_POINT('Ctrl Pts',(-7.98725565469605,-1.08774414553672,
17.6914338104691));
#27678=CARTESIAN_POINT('Ctrl Pts',(-7.30866226909047,-0.157279171604971,
17.739155833924));
#27679=CARTESIAN_POINT('Ctrl Pts',(-7.72253697950026,0.917412307278465,
17.7868778573789));
#27680=CARTESIAN_POINT('Ctrl Pts',(-8.85275194643118,1.14973456280779,17.8345998808337));
#27681=CARTESIAN_POINT('Ctrl Pts',(-9.52148929926934,0.462850473305008,
17.8743682337128));
#27682=CARTESIAN_POINT('Ctrl Pts',(-9.52997673057435,-0.236120563005232,
17.906182916016));
#27683=CARTESIAN_POINT('Ctrl Pts',(-9.21786242976372,-0.86159415103292,
17.9379975983193));
#27684=CARTESIAN_POINT('Ctrl Pts',(-8.31669687000343,-1.18858044034017,
17.9777659511983));
#27685=CARTESIAN_POINT('Ctrl Pts',(-7.40054731317204,-0.487132301554058,
18.0254879746532));
#27686=CARTESIAN_POINT('Ctrl Pts',(-7.49614243737496,0.660524277275207,
18.073209998108));
#27687=CARTESIAN_POINT('Ctrl Pts',(-8.51228454977271,1.2024737750269,18.1209320215629));
#27688=CARTESIAN_POINT('Ctrl Pts',(-9.51901692765617,0.638692415624239,
18.1686540450178));
#27689=CARTESIAN_POINT('Ctrl Pts',(-9.57533798580677,-0.318306715985504,
18.2084223978968));
#27690=CARTESIAN_POINT('Ctrl Pts',(-9.12443461381578,-0.852459030609261,
18.2402370802));
#27691=CARTESIAN_POINT('Ctrl Pts',(-8.47916294898904,-1.12126569842547,
18.2720517625033));
#27692=CARTESIAN_POINT('Ctrl Pts',(-7.5837132633384,-0.778936529406515,
18.3118201153824));
#27693=CARTESIAN_POINT('Ctrl Pts',(-7.3498148549232,0.350953304351522,18.3595421388372));
#27694=CARTESIAN_POINT('Ctrl Pts',(-8.17299650074059,1.1563265275784,18.4072641622921));
#27695=CARTESIAN_POINT('Ctrl Pts',(-9.29604348361364,0.901337263174473,
18.4549861857469));
#27696=CARTESIAN_POINT('Ctrl Pts',(-9.68851792402192,-0.183708042568584,
18.5027082092018));
#27697=CARTESIAN_POINT('Ctrl Pts',(-9.10496654566918,-0.944291495133526,
18.5424765620808));
#27698=CARTESIAN_POINT('Ctrl Pts',(-8.41448476974234,-1.05322938204008,
18.5742912443841));
#27699=CARTESIAN_POINT('Ctrl Pts',(-7.75062139220164,-0.834327664251033,
18.6061059266873));
#27700=CARTESIAN_POINT('Ctrl Pts',(-7.29741335566221,0.0104337666328781,
18.6458742795664));
#27701=CARTESIAN_POINT('Ctrl Pts',(-7.85979001642749,1.01795150509475,18.6935963030212));
#27702=CARTESIAN_POINT('Ctrl Pts',(-9.00926259833872,1.08842727494434,18.7413183264761));
#27703=CARTESIAN_POINT('Ctrl Pts',(-9.69173650578151,0.160804821377532,
18.789040349931));
#27704=CARTESIAN_POINT('Ctrl Pts',(-9.2786243254698,-0.91655205002906,18.8367623733858));
#27705=CARTESIAN_POINT('Ctrl Pts',(-8.33967793214922,-1.10994044151948,
18.8765307262649));
#27706=CARTESIAN_POINT('Ctrl Pts',(-7.746223032506,-0.740557404307124,18.9083454085681));
#27707=CARTESIAN_POINT('Ctrl Pts',(-7.38739693003254,-0.140660434591127,
18.9401600908714));
#27708=CARTESIAN_POINT('Ctrl Pts',(-7.59736645062633,0.79471767073023,18.9799284437504));
#27709=CARTESIAN_POINT('Ctrl Pts',(-8.68186329323757,1.1887051074019,19.0276504672053));
#27710=CARTESIAN_POINT('Ctrl Pts',(-9.59726656130047,0.489926954107713,
19.0753724906601));
#27711=CARTESIAN_POINT('Ctrl Pts',(-9.50646589579862,-0.658118902923217,
19.123094514115));
#27712=CARTESIAN_POINT('Ctrl Pts',(-8.48915653915779,-1.20258301999602,
19.1708165375699));
#27713=CARTESIAN_POINT('Ctrl Pts',(-7.65254526199483,-0.734500793868192,
19.2105848904489));
#27714=CARTESIAN_POINT('Ctrl Pts',(-7.44542256102972,-0.0668686100755817,
19.2423995727522));
#27715=CARTESIAN_POINT('Ctrl Pts',(-7.56655907558636,0.621577822794718,
19.2742142550554));
#27716=CARTESIAN_POINT('Ctrl Pts',(-8.33734740644836,1.19158198813036,19.3139826079345));
#27717=CARTESIAN_POINT('Ctrl Pts',(-9.41527942236304,0.779972864136537,
19.3617046313893));
#27718=CARTESIAN_POINT('Ctrl Pts',(-9.65036036266347,-0.347409503212236,
19.4094266548442));
#27719=CARTESIAN_POINT('Ctrl Pts',(-8.83054984563462,-1.15621403266934,
19.457148678299));
#27720=CARTESIAN_POINT('Ctrl Pts',(-7.704974867994,-0.902362754165209,19.5048707017539));
#27721=CARTESIAN_POINT('Ctrl Pts',(-7.37854114860306,-0.000996887084833204,
19.5446390546329));
#27722=CARTESIAN_POINT('Ctrl Pts',(-7.65872158751808,0.639418187488004,
19.5764537369362));
#27723=CARTESIAN_POINT('Ctrl Pts',(-8.20076747273577,1.0808010195163,19.6082684192394));
#27724=CARTESIAN_POINT('Ctrl Pts',(-9.15662042143786,1.00755799970849,19.6480367721185));
#27725=CARTESIAN_POINT('Ctrl Pts',(-9.70250291153056,-0.00899097053304161,
19.6957587955733));
#27726=CARTESIAN_POINT('Ctrl Pts',(-9.14266112686343,-1.01538613489058,
19.7434808190282));
#27727=CARTESIAN_POINT('Ctrl Pts',(-7.99349294093177,-1.09066249999925,
19.7912028424831));
#27728=CARTESIAN_POINT('Ctrl Pts',(-7.3083626688575,-0.162246638342256,
19.8389248659379));
#27729=CARTESIAN_POINT('Ctrl Pts',(-7.65124077756914,0.732992995531986,
19.878693218817));
#27730=CARTESIAN_POINT('Ctrl Pts',(-8.28213825309398,1.03399286507868,19.9105079011202));
#27731=CARTESIAN_POINT('Ctrl Pts',(-8.9808497396993,1.01314089690995,19.9423225834235));
#27732=CARTESIAN_POINT('Ctrl Pts',(-9.65579534164531,0.332356177702199,
19.9820909363025));
#27733=CARTESIAN_POINT('Ctrl Pts',(-9.40351421724518,-0.793571766777498,
20.0298129597574));
#27734=CARTESIAN_POINT('Ctrl Pts',(-8.32166885968162,-1.18836876907051,
20.0775349832122));
#27735=CARTESIAN_POINT('Ctrl Pts',(-7.40335486377068,-0.493420241756677,
20.1252570066671));
#27736=CARTESIAN_POINT('Ctrl Pts',(-7.49266575489391,0.656963636179604,
20.1729790301219));
#27737=CARTESIAN_POINT('Ctrl Pts',(-8.33770489079221,1.10965366069221,20.2127473830011));
#27738=CARTESIAN_POINT('Ctrl Pts',(-9.01176107344925,0.924502887773008,
20.2445620653043));
#27739=CARTESIAN_POINT('Ctrl Pts',(-9.52652095192111,0.451581315409929,
20.2763767476075));
#27740=CARTESIAN_POINT('Ctrl Pts',(-9.59152770853021,-0.504867073729894,
20.3161451004866));
#27741=CARTESIAN_POINT('Ctrl Pts',(-8.66406834236317,-1.1912915968917,20.3638671239414));
#27742=CARTESIAN_POINT('Ctrl Pts',(-7.58761183909353,-0.782029520380867,
20.4115891473963));
#27743=CARTESIAN_POINT('Ctrl Pts',(-7.34782400761312,0.344361107498901,
20.4593111708512));
#27744=CARTESIAN_POINT('Ctrl Pts',(-8.16803759563199,1.15590850101208,20.507033194306));
#27745=CARTESIAN_POINT('Ctrl Pts',(-9.10328679193923,0.945365535563934,
20.546801547185));
#27746=CARTESIAN_POINT('Ctrl Pts',(-9.49190376914431,0.364323892375815,
20.5786162294883));
#27747=CARTESIAN_POINT('Ctrl Pts',(-9.57177001728932,-0.330121158364715,
20.6104309117915));
#27748=CARTESIAN_POINT('Ctrl Pts',(-8.99514756642966,-1.09597097958138,
20.6501992646706));
#27749=CARTESIAN_POINT('Ctrl Pts',(-7.84464024017011,-1.0082646849842,20.6979212881254));
#27750=CARTESIAN_POINT('Ctrl Pts',(-7.29833798770444,0.0055439259737052,
20.7456433115803));
#27751=CARTESIAN_POINT('Ctrl Pts',(-7.85397129605098,1.0142687037785,20.7933653350352));
#27752=CARTESIAN_POINT('Ctrl Pts',(-9.00523890391058,1.09135564808224,20.8410873584901));
#27753=CARTESIAN_POINT('Ctrl Pts',(-9.57477038849185,0.320217990096556,
20.8808557113691));
#27754=CARTESIAN_POINT('Ctrl Pts',(-9.48849996469401,-0.373460581050405,
20.9126703936724));
#27755=CARTESIAN_POINT('Ctrl Pts',(-9.0945383169396,-0.950891759797607,
20.9444850759755));
#27756=CARTESIAN_POINT('Ctrl Pts',(-8.1573862740094,-1.15279631131811,20.9842534288547));
#27757=CARTESIAN_POINT('Ctrl Pts',(-7.34469566859739,-0.333715435113531,
21.0319754523094));
#27758=CARTESIAN_POINT('Ctrl Pts',(-7.59486638697568,0.790414745233752,
21.0796974757644));
#27759=CARTESIAN_POINT('Ctrl Pts',(-8.67505328733558,1.18972704280586,21.1274194992192));
#27760=CARTESIAN_POINT('Ctrl Pts',(-9.59613960186481,0.494774164492666,
21.1751415226741));
#27761=CARTESIAN_POINT('Ctrl Pts',(-9.52231055829104,-0.461033698949551,
21.2149098755531));
#27762=CARTESIAN_POINT('Ctrl Pts',(-9.00320899216289,-0.929185501396226,
21.2467245578564));
#27763=CARTESIAN_POINT('Ctrl Pts',(-8.32747313545848,-1.10810894327763,
21.2785392401596));
#27764=CARTESIAN_POINT('Ctrl Pts',(-7.48664689768428,-0.647641097100003,
21.3183075930387));
#27765=CARTESIAN_POINT('Ctrl Pts',(-7.40795428611476,0.503517873143993,
21.3660296164935));
#27766=CARTESIAN_POINT('Ctrl Pts',(-8.3326414115313,1.18996362540003,21.4137516399484));
#27767=CARTESIAN_POINT('Ctrl Pts',(-9.41079796358698,0.785201349538081,
21.4614736634033));
#27768=CARTESIAN_POINT('Ctrl Pts',(-9.65267952346093,-0.343006438452175,
21.5091956868581));
#27769=CARTESIAN_POINT('Ctrl Pts',(-8.97148112016971,-1.01753452151951,
21.5489640397372));
#27770=CARTESIAN_POINT('Ctrl Pts',(-8.27260697780362,-1.0319386606068,21.5807787220404));
#27771=CARTESIAN_POINT('Ctrl Pts',(-7.6445136546766,-0.725130375950133,
21.6125934043437));
#27772=CARTESIAN_POINT('Ctrl Pts',(-7.30991042897887,0.173234850917899,
21.6523617572227));
#27773=CARTESIAN_POINT('Ctrl Pts',(-8.00357793678801,1.09528956214643,21.7000837806776));
#27774=CARTESIAN_POINT('Ctrl Pts',(-9.15200263652367,1.00941314082768,21.7478058041324));
#27775=CARTESIAN_POINT('Ctrl Pts',(-9.70253468127204,-0.00210478704439917,
21.7955278275873));
#27776=CARTESIAN_POINT('Ctrl Pts',(-9.14729583240704,-1.01357368058483,
21.8432498510421));
#27777=CARTESIAN_POINT('Ctrl Pts',(-8.19080776710961,-1.07799402237706,
21.8830182039212));
#27778=CARTESIAN_POINT('Ctrl Pts',(-7.65285755162984,-0.63162857595897,
21.9148328862244));
#27779=CARTESIAN_POINT('Ctrl Pts',(-7.37859808588644,0.0113444340040694,
21.9466475685277));
#27780=CARTESIAN_POINT('Ctrl Pts',(-7.71333472266603,0.909659959579857,
21.9864159214067));
#27781=CARTESIAN_POINT('Ctrl Pts',(-8.84120404649836,1.15311486350827,22.0341379448616));
#27782=CARTESIAN_POINT('Ctrl Pts',(-9.65351690621254,0.336780453695434,
22.0818599683164));
#27783=CARTESIAN_POINT('Ctrl Pts',(-9.40804372796624,-0.788384853920802,
22.1295819917713));
#27784=CARTESIAN_POINT('Ctrl Pts',(-8.3263597217982,-1.1900304846565,22.1773040152262));
#27785=CARTESIAN_POINT('Ctrl Pts',(-7.56086357421315,-0.61293859637056,
22.2170723681052));
#27786=CARTESIAN_POINT('Ctrl Pts',(-7.44608444309555,0.076596244772818,
22.2488870504085));
#27787=CARTESIAN_POINT('Ctrl Pts',(-7.65935850290658,0.742288907720554,
22.2807017327117));
#27788=CARTESIAN_POINT('Ctrl Pts',(-8.50025311474624,1.20263187907136,22.3204700855908));
#27789=CARTESIAN_POINT('Ctrl Pts',(-9.5124954495042,0.648804326838139,22.3681921090456));
#27790=CARTESIAN_POINT('Ctrl Pts',(-9.59269934472105,-0.500030468027331,
22.4159141325005));
#27791=CARTESIAN_POINT('Ctrl Pts',(-8.67088748766811,-1.19033254023784,
22.4636361559554));
#27792=CARTESIAN_POINT('Ctrl Pts',(-7.59007209365373,-0.786355330545981,
22.5113581794102));
#27793=CARTESIAN_POINT('Ctrl Pts',(-7.38874215200747,0.150920324792225,
22.5511265322893));
#27794=CARTESIAN_POINT('Ctrl Pts',(-7.75308816941443,0.747480904859688,
22.5829412145925));
#27795=CARTESIAN_POINT('Ctrl Pts',(-8.3499260669922,1.11137246852348,22.6147558968957));
#27796=CARTESIAN_POINT('Ctrl Pts',(-9.28704811506866,0.909328744290342,
22.6545242497748));
#27797=CARTESIAN_POINT('Ctrl Pts',(-9.69020204494021,-0.171794010404042,
22.7022462732297));
#27798=CARTESIAN_POINT('Ctrl Pts',(-8.99919810938205,-1.09307985732919,
22.7499682966845));
#27799=CARTESIAN_POINT('Ctrl Pts',(-7.8504247320093,-1.01200101828279,22.7976903201394));
#27800=CARTESIAN_POINT('Ctrl Pts',(-7.29736827694888,0.000662824956886309,
22.8454123435943));
#27801=CARTESIAN_POINT('Ctrl Pts',(-7.75835155074568,0.841206589892776,
22.8851806964733));
#27802=CARTESIAN_POINT('Ctrl Pts',(-8.42420645284244,1.05397358790808,22.9169953787766));
#27803=CARTESIAN_POINT('Ctrl Pts',(-9.11365367676609,0.938669331634874,
22.9488100610797));
#27804=CARTESIAN_POINT('Ctrl Pts',(-9.69016238614474,0.172733885592879,
22.9885784139589));
#27805=CARTESIAN_POINT('Ctrl Pts',(-9.2876930476951,-0.908643908472059,
23.0363004374137));
#27806=CARTESIAN_POINT('Ctrl Pts',(-8.16234111093395,-1.15326007541409,
23.0840224608686));
#27807=CARTESIAN_POINT('Ctrl Pts',(-7.34662560561449,-0.340325720694794,
23.1317444843235));
#27808=CARTESIAN_POINT('Ctrl Pts',(-7.59093943845774,0.787357857695122,
23.1794665077782));
#27809=CARTESIAN_POINT('Ctrl Pts',(-8.48950964314851,1.12141022894101,23.2192348606574));
#27810=CARTESIAN_POINT('Ctrl Pts',(-9.13227358715871,0.846661146374397,
23.2510495429606));
#27811=CARTESIAN_POINT('Ctrl Pts',(-9.57822919443977,0.308371129352578,
23.2828642252638));
#27812=CARTESIAN_POINT('Ctrl Pts',(-9.51308039793912,-0.64806759519152,
23.3226325781429));
#27813=CARTESIAN_POINT('Ctrl Pts',(-8.5011889208313,-1.20253593553699,23.3703546015977));
#27814=CARTESIAN_POINT('Ctrl Pts',(-7.49009057848581,-0.651233665627234,
23.4180766250526));
#27815=CARTESIAN_POINT('Ctrl Pts',(-7.40508883683077,0.497256105601518,
23.4657986485074));
#27816=CARTESIAN_POINT('Ctrl Pts',(-8.32767158657437,1.1902211637137,23.5135206719624));
#27817=CARTESIAN_POINT('Ctrl Pts',(-9.22578171484917,0.854933828755763,
23.5532890248414));
#27818=CARTESIAN_POINT('Ctrl Pts',(-9.53211154671474,0.226607018727755,
23.5851037071447));
#27819=CARTESIAN_POINT('Ctrl Pts',(-9.51717514043059,-0.472255950571703,
23.6169183894479));
#27820=CARTESIAN_POINT('Ctrl Pts',(-8.84212844368635,-1.1529404271889,23.6566867423269));
#27821=CARTESIAN_POINT('Ctrl Pts',(-7.71410520295799,-0.91019968016524,
23.7044087657818));
#27822=CARTESIAN_POINT('Ctrl Pts',(-7.31016418213637,0.168264831257892,
23.7521307892367));
#27823=CARTESIAN_POINT('Ctrl Pts',(-7.99731398869925,1.09242888273476,23.7998528126915));
#27824=CARTESIAN_POINT('Ctrl Pts',(-9.14841269178917,1.01285955677601,23.8475748361464));
#27825=CARTESIAN_POINT('Ctrl Pts',(-9.60824002053544,0.171682864736176,
23.8873431890254));
#27826=CARTESIAN_POINT('Ctrl Pts',(-9.42880198158284,-0.503916525633289,
23.9191578713287));
#27827=CARTESIAN_POINT('Ctrl Pts',(-8.96025496060319,-1.02266139088192,
23.9509725536319));
#27828=CARTESIAN_POINT('Ctrl Pts',(-8.00439114523888,-1.09576245770156,
23.9907409065109));
#27829=CARTESIAN_POINT('Ctrl Pts',(-7.31013997945228,-0.174147125421988,
24.0384629299658));
#27830=CARTESIAN_POINT('Ctrl Pts',(-7.71027484520036,0.905735340365012,
24.0861849534207));
#27831=CARTESIAN_POINT('Ctrl Pts',(-8.83459523269867,1.15504983444261,24.1339069768756));
#27832=CARTESIAN_POINT('Ctrl Pts',(-9.65305691591741,0.34173564239159,24.1816290003304));
#27833=CARTESIAN_POINT('Ctrl Pts',(-9.45043867612152,-0.595262355682614,
24.2213973532095));
#27834=CARTESIAN_POINT('Ctrl Pts',(-8.87270761867775,-0.988784110298152,
24.2532120355127));
#27835=CARTESIAN_POINT('Ctrl Pts',(-8.17896354407182,-1.07452619471349,
24.285026717816));
#27836=CARTESIAN_POINT('Ctrl Pts',(-7.40825987210933,-0.504407567131031,
24.324795070695));
#27837=CARTESIAN_POINT('Ctrl Pts',(-7.48622361400777,0.646800996439465,
24.3725170941499));
#27838=CARTESIAN_POINT('Ctrl Pts',(-8.49537127660111,1.20166588610525,24.4202391176047));
#27839=CARTESIAN_POINT('Ctrl Pts',(-9.50876352283132,0.654591662638275,
24.4679611410596));
#27840=CARTESIAN_POINT('Ctrl Pts',(-9.59559355107939,-0.495982128164943,
24.5156831645145));
#27841=CARTESIAN_POINT('Ctrl Pts',(-8.82930478903784,-1.07202113089114,
24.5554515173935));
#27842=CARTESIAN_POINT('Ctrl Pts',(-8.13492076684851,-0.991626007787244,
24.5872661996968));
#27843=CARTESIAN_POINT('Ctrl Pts',(-7.5541752677766,-0.602566614636904,
24.619080882));
#27844=CARTESIAN_POINT('Ctrl Pts',(-7.34434466099276,0.332842662604764,
24.658849234879));
#27845=CARTESIAN_POINT('Ctrl Pts',(-8.15651650416419,1.15243792799395,24.7065712583339));
#27846=CARTESIAN_POINT('Ctrl Pts',(-9.2827241799191,0.911792292728668,24.7542932817887));
#27847=CARTESIAN_POINT('Ctrl Pts',(-9.69116629486312,-0.16497559750651,
24.8020153052437));
#27848=CARTESIAN_POINT('Ctrl Pts',(-9.00403560601477,-1.09191190509816,
24.8497373286984));
#27849=CARTESIAN_POINT('Ctrl Pts',(-8.04763700423772,-1.02617672416858,
24.8895056815775));
#27850=CARTESIAN_POINT('Ctrl Pts',(-7.57510761666008,-0.511056811947901,
24.9213203638808));
#27851=CARTESIAN_POINT('Ctrl Pts',(-7.39047026714238,0.163140188381993,
24.953135046184));
#27852=CARTESIAN_POINT('Ctrl Pts',(-7.8438037528424,1.00783430475553,24.9929033990631));
#27853=CARTESIAN_POINT('Ctrl Pts',(-8.99425531743911,1.09626902308409,25.0406254225179));
#27854=CARTESIAN_POINT('Ctrl Pts',(-9.68850424366054,0.177426011932626,
25.0883474459728));
#27855=CARTESIAN_POINT('Ctrl Pts',(-9.29288340878006,-0.904118349483034,
25.1360694694276));
#27856=CARTESIAN_POINT('Ctrl Pts',(-8.16676365035883,-1.15554187977053,
25.1837914928825));
#27857=CARTESIAN_POINT('Ctrl Pts',(-7.48649317569277,-0.480077979335733,
25.2235598457615));
#27858=CARTESIAN_POINT('Ctrl Pts',(-7.4661733610654,0.218649185746783,25.2553745280648));
#27859=CARTESIAN_POINT('Ctrl Pts',(-7.76765364280032,0.849317232991748,
25.287189210368));
#27860=CARTESIAN_POINT('Ctrl Pts',(-8.6631541573295,1.19151341644644,25.3269575632471));
#27861=CARTESIAN_POINT('Ctrl Pts',(-9.59104794585171,0.505676249831224,
25.3746795867019));
#27862=CARTESIAN_POINT('Ctrl Pts',(-9.51489638156947,-0.643434271380218,
25.4224016101568));
#27863=CARTESIAN_POINT('Ctrl Pts',(-8.50807512651903,-1.20250941040903,
25.4701236336117));
#27864=CARTESIAN_POINT('Ctrl Pts',(-7.49194220210365,-0.655852862101074,
25.5178456570665));
#27865=CARTESIAN_POINT('Ctrl Pts',(-7.41942719321752,0.300055592186921,
25.5576140099456));
#27866=CARTESIAN_POINT('Ctrl Pts',(-7.86122272622574,0.841765157456683,
25.5894286922488));
#27867=CARTESIAN_POINT('Ctrl Pts',(-8.50185100402222,1.12145776690186,25.6212433745521));
#27868=CARTESIAN_POINT('Ctrl Pts',(-9.40296799363835,0.794337650555834,
25.6610117274311));
#27869=CARTESIAN_POINT('Ctrl Pts',(-9.65596194639845,-0.331430336977873,
25.708733750886));
#27870=CARTESIAN_POINT('Ctrl Pts',(-8.84653327347151,-1.15062462049382,
25.7564557743408));
#27871=CARTESIAN_POINT('Ctrl Pts',(-7.71933027370747,-0.91468511972205,
25.8041777977958));
#27872=CARTESIAN_POINT('Ctrl Pts',(-7.30854223573027,0.163560070271257,
25.8518998212506));
#27873=CARTESIAN_POINT('Ctrl Pts',(-7.87913327787808,0.933914055211717,
25.8916681741297));
#27874=CARTESIAN_POINT('Ctrl Pts',(-8.56767177017992,1.05452620513634,25.9234828564328));
#27875=CARTESIAN_POINT('Ctrl Pts',(-9.23514601307596,0.846895087138279,
25.9552975387362));
#27876=CARTESIAN_POINT('Ctrl Pts',(-9.70259092973129,0.00992755527928493,
25.9950658916151));
#27877=CARTESIAN_POINT('Ctrl Pts',(-9.15735217491194,-1.00696683556567,
26.04278791507));
#27878=CARTESIAN_POINT('Ctrl Pts',(-8.00923749591142,-1.096893108507,26.0905099385249));
#27879=CARTESIAN_POINT('Ctrl Pts',(-7.31115672797335,-0.180957907667782,
26.1382319619798));
#27880=CARTESIAN_POINT('Ctrl Pts',(-7.70597001687183,0.903238554601866,
26.1859539854346));
#27881=CARTESIAN_POINT('Ctrl Pts',(-8.64150776634741,1.11249561851891,26.2257223383137));
#27882=CARTESIAN_POINT('Ctrl Pts',(-9.24113127558509,0.753212731005102,
26.2575370206169));
#27883=CARTESIAN_POINT('Ctrl Pts',(-9.61006222291879,0.159476676692902,
26.2893517029202));
#27884=CARTESIAN_POINT('Ctrl Pts',(-9.415958774083,-0.77932215726626,26.3291200557992));
#27885=CARTESIAN_POINT('Ctrl Pts',(-8.33828758368432,-1.19161368916269,
26.3768420792541));
#27886=CARTESIAN_POINT('Ctrl Pts',(-7.41118517990141,-0.508433490678091,
26.4245641027089));
#27887=CARTESIAN_POINT('Ctrl Pts',(-7.48253638214871,0.640985082618556,
26.4722861261638));
#27888=CARTESIAN_POINT('Ctrl Pts',(-8.49048214157161,1.20259424204372,26.5200081496186));
#27889=CARTESIAN_POINT('Ctrl Pts',(-9.33489815848678,0.748742955970736,
26.5597765024977));
#27890=CARTESIAN_POINT('Ctrl Pts',(-9.5532942060547,0.0847130526550384,
26.5915911848009));
#27891=CARTESIAN_POINT('Ctrl Pts',(-9.44383047110093,-0.605685554542794,
26.6234058671042));
#27892=CARTESIAN_POINT('Ctrl Pts',(-8.68280279902496,-1.18865749368541,
26.6631742199832));
#27893=CARTESIAN_POINT('Ctrl Pts',(-7.59805672146549,-0.795356782894942,
26.7108962434381));
#27894=CARTESIAN_POINT('Ctrl Pts',(-7.34392285778294,0.327884077308811,
26.758618266893));
#27895=CARTESIAN_POINT('Ctrl Pts',(-8.14992279296913,1.15045210196167,26.8063402903478));
#27896=CARTESIAN_POINT('Ctrl Pts',(-9.27963415904636,0.915693223014039,
26.8540623138027));
#27897=CARTESIAN_POINT('Ctrl Pts',(-9.62128124298946,0.0199830748488219,
26.8938306666817));
#27898=CARTESIAN_POINT('Ctrl Pts',(-9.35198320608394,-0.625083676278201,
26.925645348985));
#27899=CARTESIAN_POINT('Ctrl Pts',(-8.81748763267519,-1.07558010034525,
26.9574600312882));
#27900=CARTESIAN_POINT('Ctrl Pts',(-7.8605316734503,-1.01853019590265,26.9972283841673));
#27901=CARTESIAN_POINT('Ctrl Pts',(-7.2975172176546,-0.0113687269941268,
27.0449504076221));
#27902=CARTESIAN_POINT('Ctrl Pts',(-7.84024046489426,1.00436033511211,27.092672431077));
#27903=CARTESIAN_POINT('Ctrl Pts',(-8.98796951732628,1.09908136184312,27.1403944545319));
#27904=CARTESIAN_POINT('Ctrl Pts',(-9.68871970159898,0.18239783895712,27.1881164779867));
#27905=CARTESIAN_POINT('Ctrl Pts',(-9.36104716805341,-0.71851842255269,
27.2278848308658));
#27906=CARTESIAN_POINT('Ctrl Pts',(-8.73533605123604,-1.03015626425663,
27.259699513169));
#27907=CARTESIAN_POINT('Ctrl Pts',(-8.03637168178112,-1.02113649024308,
27.2915141954723));
#27908=CARTESIAN_POINT('Ctrl Pts',(-7.34999711030817,-0.351876191758067,
27.3312825483513));
#27909=CARTESIAN_POINT('Ctrl Pts',(-7.58318008445249,0.778161507815739,
27.3790045718062));
#27910=CARTESIAN_POINT('Ctrl Pts',(-8.65818646385365,1.19121759958578,27.426726595261));
#27911=CARTESIAN_POINT('Ctrl Pts',(-9.58813434263154,0.511915756913528,
27.4744486187159));
#27912=CARTESIAN_POINT('Ctrl Pts',(-9.51831228400498,-0.639815280272654,
27.5221706421708));
#27913=CARTESIAN_POINT('Ctrl Pts',(-8.68105831697462,-1.1067469606982,27.5619389950498));
#27914=CARTESIAN_POINT('Ctrl Pts',(-8.00396413429619,-0.933034514760314,
27.5937536773531));
#27915=CARTESIAN_POINT('Ctrl Pts',(-7.48127145702591,-0.468895622596703,
27.6255683596563));
#27916=CARTESIAN_POINT('Ctrl Pts',(-7.40008131862942,0.486315119030573,
27.6653367125354));
#27917=CARTESIAN_POINT('Ctrl Pts',(-8.31578657140523,1.18834317539839,27.7130587359902));
#27918=CARTESIAN_POINT('Ctrl Pts',(-9.39901761221339,0.797364195233005,
27.7607807594451));
#27919=CARTESIAN_POINT('Ctrl Pts',(-9.65784090229139,-0.324805379837842,
27.8085027828999));
#27920=CARTESIAN_POINT('Ctrl Pts',(-8.85148439065207,-1.15012269943416,
27.8562248063548));
#27921=CARTESIAN_POINT('Ctrl Pts',(-7.9128047387935,-0.955443705498678,
27.8959931592339));
#27922=CARTESIAN_POINT('Ctrl Pts',(-7.51440640767294,-0.381064635675364,
27.9278078415371));
#27923=CARTESIAN_POINT('Ctrl Pts',(-7.42279463151268,0.311928747092104,
27.9596225238404));
#27924=CARTESIAN_POINT('Ctrl Pts',(-7.9863685794706,1.08743103894948,27.9993908767193));
#27925=CARTESIAN_POINT('Ctrl Pts',(-9.13819588142177,1.01921543685667,28.0471129001743));
#27926=CARTESIAN_POINT('Ctrl Pts',(-9.70158364506713,0.0148010410636816,
28.0948349236291));
#27927=CARTESIAN_POINT('Ctrl Pts',(-9.16310771139847,-1.00318605097683,
28.142556947084));
#27928=CARTESIAN_POINT('Ctrl Pts',(-8.01331019109225,-1.09975294067858,
28.1902789705388));
#27929=CARTESIAN_POINT('Ctrl Pts',(-7.43080495083982,-0.338367989046775,
28.2300473234179));
#27930=CARTESIAN_POINT('Ctrl Pts',(-7.50531901190296,0.356671722620504,
28.2618620057211));
#27931=CARTESIAN_POINT('Ctrl Pts',(-7.88944826933002,0.940689924117418,
28.2936766880244));
#27932=CARTESIAN_POINT('Ctrl Pts',(-8.8230477467519,1.15843154909714,28.3334450409034));
#27933=CARTESIAN_POINT('Ctrl Pts',(-9.64948893755617,0.353226941538994,
28.3811670643583));
#27934=CARTESIAN_POINT('Ctrl Pts',(-9.41838563076225,-0.774977522329652,
28.4288890878132));
#27935=CARTESIAN_POINT('Ctrl Pts',(-8.34511391495364,-1.19252018450285,
28.476611111268));
#27936=CARTESIAN_POINT('Ctrl Pts',(-7.4123940412223,-0.513260926891183,
28.5243331347229));
#27937=CARTESIAN_POINT('Ctrl Pts',(-7.47003064875324,0.443659874939181,
28.5641014876019));
#27938=CARTESIAN_POINT('Ctrl Pts',(-7.98113199205868,0.920532984820785,
28.5959161699052));
#27939=CARTESIAN_POINT('Ctrl Pts',(-8.65374182116355,1.11087101034145,28.6277308522084));
#27940=CARTESIAN_POINT('Ctrl Pts',(-9.50224328279785,0.664704372278146,
28.6674992050875));
#27941=CARTESIAN_POINT('Ctrl Pts',(-9.60041377061406,-0.484957341939309,
28.7152212285423));
#27942=CARTESIAN_POINT('Ctrl Pts',(-8.68748072028854,-1.18695969033224,
28.7629432519972));
#27943=CARTESIAN_POINT('Ctrl Pts',(-7.60262605682145,-0.800508647597918,
28.810665275452));
#27944=CARTESIAN_POINT('Ctrl Pts',(-7.34167857245849,0.323442379934373,
28.8583872989069));
#27945=CARTESIAN_POINT('Ctrl Pts',(-8.01135956689715,1.00940649664747,28.8981556517859));
#27946=CARTESIAN_POINT('Ctrl Pts',(-8.70988967809667,1.03564052975447,28.9299703340892));
#27947=CARTESIAN_POINT('Ctrl Pts',(-9.3430872614141,0.739509857624331,28.9617850163924));
#27948=CARTESIAN_POINT('Ctrl Pts',(-9.69285186336733,-0.153061774255562,
29.0015533692715));
#27949=CARTESIAN_POINT('Ctrl Pts',(-9.01489421704395,-1.0867281375265,29.0492753927263));
#27950=CARTESIAN_POINT('Ctrl Pts',(-7.8651801697202,-1.02030689992113,29.0969974161812));
#27951=CARTESIAN_POINT('Ctrl Pts',(-7.29760210087134,-0.0182544462221305,
29.1447194396361));
#27952=CARTESIAN_POINT('Ctrl Pts',(-7.83563697930274,1.00246964476768,29.192441463091));
#27953=CARTESIAN_POINT('Ctrl Pts',(-8.79089767439502,1.08307420682354,29.23220981597));
#27954=CARTESIAN_POINT('Ctrl Pts',(-9.33632724182628,0.645880124738788,
29.2640244982732));
#27955=CARTESIAN_POINT('Ctrl Pts',(-9.62143398657489,0.00764272958403749,
29.2958391805765));
#27956=CARTESIAN_POINT('Ctrl Pts',(-9.3019515409739,-0.896211681488417,
29.3356075334555));
#27957=CARTESIAN_POINT('Ctrl Pts',(-8.17836973863726,-1.15872558044607,
29.3833295569104));
#27958=CARTESIAN_POINT('Ctrl Pts',(-7.35234534113202,-0.356262373711148,
29.4310515803652));
#27959=CARTESIAN_POINT('Ctrl Pts',(-7.57874808812184,0.772900762458947,
29.4787736038201));
#27960=CARTESIAN_POINT('Ctrl Pts',(-8.65345018277372,1.19279547618231,29.526495627275));
#27961=CARTESIAN_POINT('Ctrl Pts',(-9.42865613481405,0.628757665818371,
29.566263980154));
#27962=CARTESIAN_POINT('Ctrl Pts',(-9.55501939402632,-0.0587522064317555,
29.5980786624573));
#27963=CARTESIAN_POINT('Ctrl Pts',(-9.35318997184504,-0.727926671584861,
29.6298933447605));
#27964=CARTESIAN_POINT('Ctrl Pts',(-8.51989092266622,-1.2025142782169,29.6696616976397));
#27965=CARTESIAN_POINT('Ctrl Pts',(-7.4989974653622,-0.66576813704867,29.7173837210943));
#27966=CARTESIAN_POINT('Ctrl Pts',(-7.39832642452834,0.48130377881185,29.7651057445494));
#27967=CARTESIAN_POINT('Ctrl Pts',(-8.3102490425179,1.18756791113303,29.8128277680041));
#27968=CARTESIAN_POINT('Ctrl Pts',(-9.21331813028293,0.865450294731648,
29.8525961208832));
#27969=CARTESIAN_POINT('Ctrl Pts',(-9.52878251944959,0.241452561833112,
29.8844108031864));
#27970=CARTESIAN_POINT('Ctrl Pts',(-9.52368474853521,-0.457174338715818,
29.9162254854897));
#27971=CARTESIAN_POINT('Ctrl Pts',(-8.85937881967026,-1.1484426233223,29.9559938383687));
#27972=CARTESIAN_POINT('Ctrl Pts',(-7.72641809337258,-0.920473928895496,
30.0037158618236));
#27973=CARTESIAN_POINT('Ctrl Pts',(-7.3792747880128,-0.0294746800767998,
30.0434842147026));
#27974=CARTESIAN_POINT('Ctrl Pts',(-7.64321372550183,0.620692232781446,
30.0752988970059));
#27975=CARTESIAN_POINT('Ctrl Pts',(-7.90933322058758,0.844396458214266,
30.0912062381575));
#27976=CARTESIAN_POINT('Ctrl Pts',(-8.06214407575858,0.917335061595102,
30.0991599087333));
#27977=CARTESIAN_POINT('',(-7.9881611888325,1.07233375495115,30.));
#27978=CARTESIAN_POINT('Ctrl Pts',(-7.90984029786115,-0.827606761449162,
30.));
#27979=CARTESIAN_POINT('Ctrl Pts',(-7.79482765977711,-0.758933651579334,
30.));
#27980=CARTESIAN_POINT('Ctrl Pts',(-7.69456529374308,-0.668153006100937,
30.));
#27981=CARTESIAN_POINT('Ctrl Pts',(-7.53132804516273,-0.450356182128115,
30.));
#27982=CARTESIAN_POINT('Ctrl Pts',(-7.47119836686902,-0.324509106703349,
30.));
#27983=CARTESIAN_POINT('Ctrl Pts',(-7.40075075771614,-0.05295558696816,
30.));
#27984=CARTESIAN_POINT('Ctrl Pts',(-7.3926420328952,0.0905106217809897,
30.));
#27985=CARTESIAN_POINT('Ctrl Pts',(-7.43167638457232,0.376768385136799,
30.));
#27986=CARTESIAN_POINT('Ctrl Pts',(-7.48000224762515,0.516568235233513,
30.));
#27987=CARTESIAN_POINT('Ctrl Pts',(-7.60465705262832,0.731837239747291,
30.));
#27988=CARTESIAN_POINT('Ctrl Pts',(-7.66748861751526,0.812979534738878,
30.));
#27989=CARTESIAN_POINT('Ctrl Pts',(-7.81408314327503,0.958099062268137,
30.));
#27990=CARTESIAN_POINT('Ctrl Pts',(-7.89754686751452,1.02107277613379,30.));
#27991=CARTESIAN_POINT('Ctrl Pts',(-7.98816118883251,1.07233375495116,30.));
#27992=CARTESIAN_POINT('Ctrl Pts',(-7.98816118883246,1.07233375495113,30.));
#27993=CARTESIAN_POINT('Ctrl Pts',(-7.7185827492918,0.943660468883421,29.9879968132107));
#27994=CARTESIAN_POINT('Ctrl Pts',(-7.5011118191916,0.709457822903462,29.9759936264214));
#27995=CARTESIAN_POINT('Ctrl Pts',(-7.39273625402487,0.431098187741625,
29.9639904396321));
#27996=CARTESIAN_POINT('Ctrl Pts',(-7.28436068885813,0.152738552579788,
29.9519872528427));
#27997=CARTESIAN_POINT('Ctrl Pts',(-7.28621794011163,-0.166856559148227,
29.9399840660534));
#27998=CARTESIAN_POINT('Ctrl Pts',(-7.39782131852533,-0.443937838810512,
29.9279808792641));
#27999=CARTESIAN_POINT('Ctrl Pts',(-7.50942469693902,-0.721019118472796,
29.9159776924748));
#28000=CARTESIAN_POINT('Ctrl Pts',(-7.72960287363902,-0.952678470383577,
29.9039745056855));
#28001=CARTESIAN_POINT('Ctrl Pts',(-8.00065856416201,-1.07820998932502,
29.8919713188961));
#28002=CARTESIAN_POINT('Ctrl Pts',(-8.271714254685,-1.20374150826646,29.8799681321068));
#28003=CARTESIAN_POINT('Ctrl Pts',(-8.5908026046793,-1.22182768311292,29.8679649453175));
#28004=CARTESIAN_POINT('Ctrl Pts',(-8.87430710148917,-1.12772906515695,
29.8559617585282));
#28005=CARTESIAN_POINT('Ctrl Pts',(-9.15781159829903,-1.03363044720099,
29.8439585717389));
#28006=CARTESIAN_POINT('Ctrl Pts',(-9.40275673161545,-0.828334644790751,
29.8319553849496));
#28007=CARTESIAN_POINT('Ctrl Pts',(-9.54495508174642,-0.565639043699543,
29.8199521981602));
#28008=CARTESIAN_POINT('Ctrl Pts',(-9.63850099762682,-0.39282339162483,
29.8120558400052));
#28009=CARTESIAN_POINT('Ctrl Pts',(-9.68822500000028,-0.196509765607819,
29.8041594818502));
#28010=CARTESIAN_POINT('Ctrl Pts',(-9.688225,1.70996550252767E-12,29.7962631236951));
#28011=CARTESIAN_POINT('Origin',(-8.5,0.,30.));
#28012=CARTESIAN_POINT('Origin',(-8.5,0.,30.));
#28013=CARTESIAN_POINT('Origin',(-8.5,0.,1.8));
#34379=UNCERTAINTY_MEASURE_WITH_UNIT(LENGTH_MEASURE(0.001),#34434,
'DISTANCE_ACCURACY_VALUE',
'Maximum model space distance between geometric entities at asserted c
onnectivities');
#34404=UNCERTAINTY_MEASURE_WITH_UNIT(LENGTH_MEASURE(0.001),#34434,
'DISTANCE_ACCURACY_VALUE',
'Maximum model space distance between geometric entities at asserted c
onnectivities');
#34408=(
GEOMETRIC_REPRESENTATION_CONTEXT(3)
GLOBAL_UNCERTAINTY_ASSIGNED_CONTEXT((#34379))
GLOBAL_UNIT_ASSIGNED_CONTEXT((#34434,#34436,#34437))
REPRESENTATION_CONTEXT('','3D')
);
#34433=(
GEOMETRIC_REPRESENTATION_CONTEXT(3)
GLOBAL_UNCERTAINTY_ASSIGNED_CONTEXT((#34404))
GLOBAL_UNIT_ASSIGNED_CONTEXT((#34434,#34436,#34437))
REPRESENTATION_CONTEXT('','3D')
);
#34434=(
LENGTH_UNIT()
NAMED_UNIT(*)
SI_UNIT(.CENTI.,.METRE.)
);
#34436=(
NAMED_UNIT(*)
PLANE_ANGLE_UNIT()
SI_UNIT($,.RADIAN.)
);
#34437=(
NAMED_UNIT(*)
SI_UNIT($,.STERADIAN.)
SOLID_ANGLE_UNIT()
);
#34441=SHAPE_DEFINITION_REPRESENTATION(#34469,#34540);
#34469=PRODUCT_DEFINITION_SHAPE('',$,#34569);
#34540=SHAPE_REPRESENTATION('',(#9072),#34408);
#34565=PRODUCT_DEFINITION_CONTEXT('part definition',#34651,'design');
#34569=PRODUCT_DEFINITION('Threaded column','Threaded column',#34597,#34565);
#34597=PRODUCT_DEFINITION_FORMATION('',$,#34656);
#34651=APPLICATION_CONTEXT(
'Core Data for Automotive Mechanical Design Process');
#34652=PRODUCT_CONTEXT('part definition',#34651,'mechanical');
#34656=PRODUCT('Threaded column','Threaded column','Threaded column',(#34652));
#34751=COLOUR_RGB('Off White',0.89,0.88,0.83);
#34752=FILL_AREA_STYLE_COLOUR('',#34751);
#34753=FILL_AREA_STYLE('',(#34752));
#34754=SURFACE_STYLE_FILL_AREA(#34753);
#34755=SURFACE_SIDE_STYLE('',(#34754));
#34756=SURFACE_STYLE_USAGE(.BOTH.,#34755);
#34757=PRESENTATION_STYLE_ASSIGNMENT((#34756));
ENDSEC;
END-ISO-10303-21;
